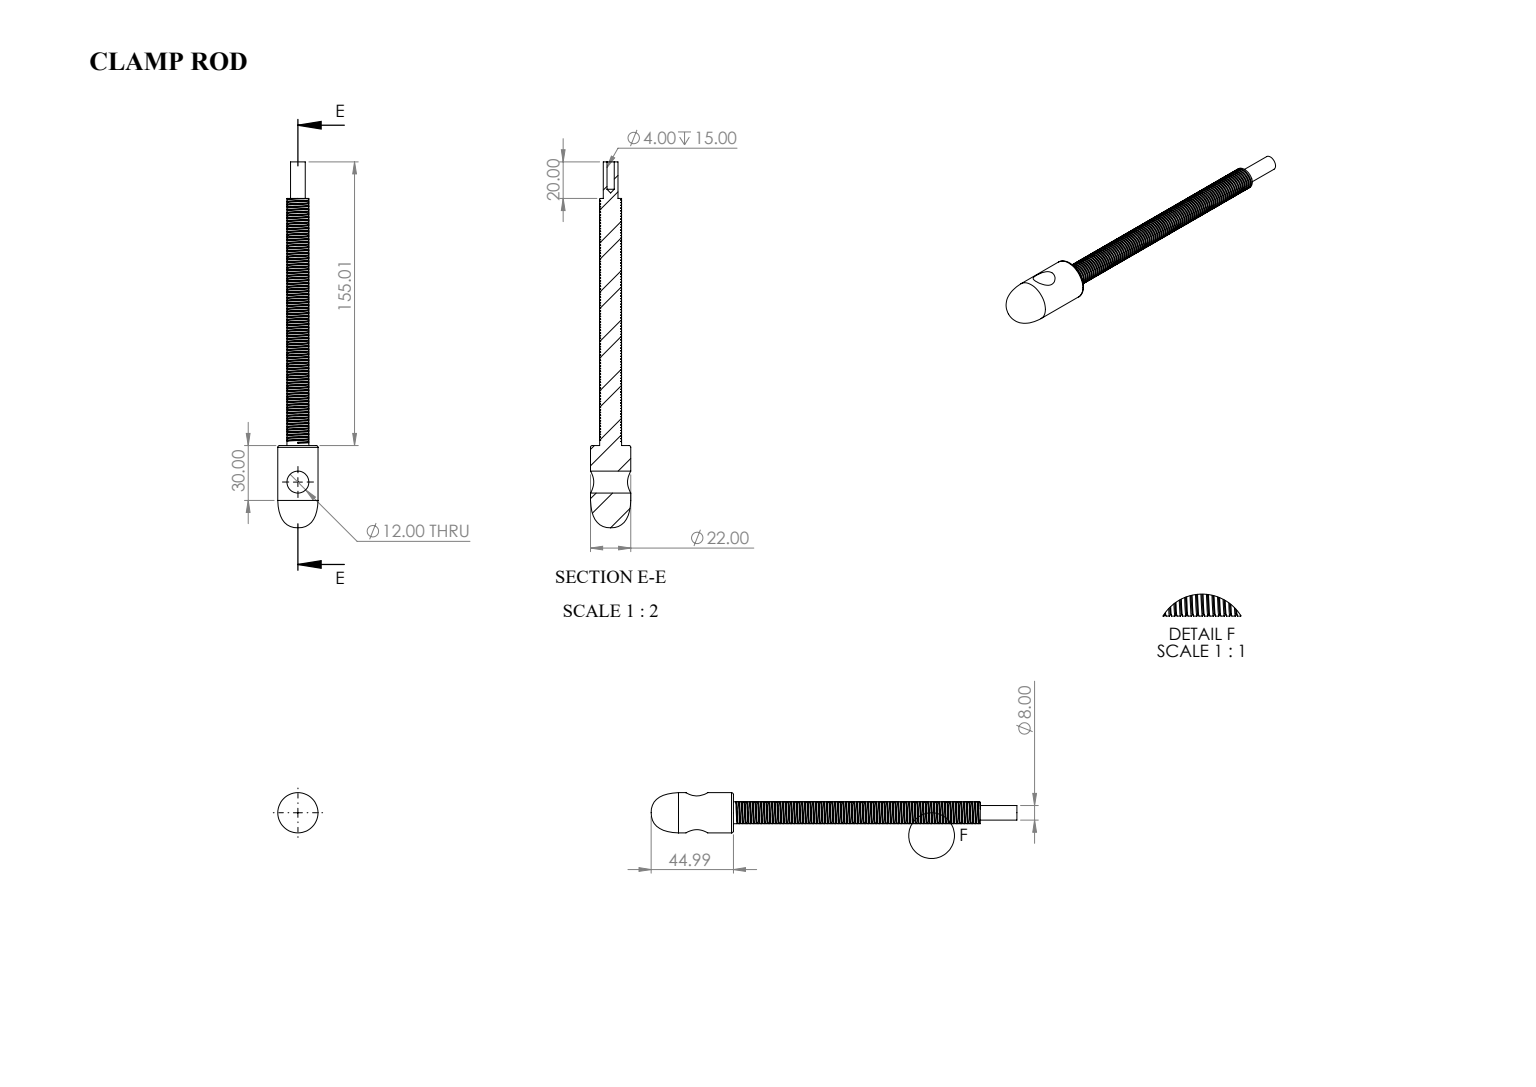
ISO-10303-21;
HEADER;
FILE_DESCRIPTION (('STEP AP214'),
    '1' );
FILE_NAME ('Clamp rod.step',
    '2026-10-07T06:38:26',
    ( '' ),
    ( '' ),
    'SwSTEP 2.0',
    'SolidWorks 2021',
    '' );
FILE_SCHEMA (( 'AUTOMOTIVE_DESIGN' ));
ENDSEC;

DATA;
#1=VERTEX_POINT ( 'NONE', #13580 ) ;
#5=ORIENTED_EDGE ( 'NONE', *, *, #19399, .F. ) ;
#6=CARTESIAN_POINT ( 'NONE',  ( -5.412658773652684552, -3.125000000000099920, -143.0669872981078470 ) ) ;
#10=CARTESIAN_POINT ( 'NONE',  ( 5.999999999999999112, 2.951592740943527306E-14, -151.5863248654052029 ) ) ;
#13=CARTESIAN_POINT ( 'NONE',  ( 3.464101615137757051, -5.999999999999979572, -171.3363248654052029 ) ) ;
#15=CARTESIAN_POINT ( 'NONE',  ( -5.412658773652739619, 3.124999999999975131, -63.18301270189225249 ) ) ;
#16=CARTESIAN_POINT ( 'NONE',  ( -5.999999999999963585, 1.780251999655701777E-13, -110.9136751345948255 ) ) ;
#18=DIRECTION ( 'NONE',  ( 1.000000000000000000, -5.551115123125774074E-17, 0.000000000000000000 ) ) ;
#21=CYLINDRICAL_SURFACE ( 'NONE', #16144, 11.00000000000001599 ) ;
#23=EDGE_CURVE ( 'NONE', #18475, #14303, #3726, .T. ) ;
#26=EDGE_LOOP ( 'NONE', ( #21447, #18277, #20127, #3460 ) ) ;
#27=CARTESIAN_POINT ( 'NONE',  ( -6.350852961085760029, -1.281975124255709124E-13, -55.12500000000003553 ) ) ;
#29=CARTESIAN_POINT ( 'NONE',  ( 6.000000000000000888, -1.859271017917181981E-14, -167.1636751345948255 ) ) ;
#30=CARTESIAN_POINT ( 'NONE',  ( -3.464101615137757051, -5.999999999999979572, -179.0863248654052313 ) ) ;
#34=CARTESIAN_POINT ( 'NONE',  ( -3.608439182435052128, -6.250000000000110134, -103.9419872981078328 ) ) ;
#36=CARTESIAN_POINT ( 'NONE',  ( -3.464101615137725076, 5.999999999999979572, -176.5863248654052313 ) ) ;
#37=VECTOR ( 'NONE', #4562, 1000.000000000000000 ) ;
#40=CARTESIAN_POINT ( 'NONE',  ( 3.175426480543072749, -5.500000000000105693, -138.6250000000000568 ) ) ;
#47=CARTESIAN_POINT ( 'NONE',  ( -3.175426480542816510, -5.500000000000057732, -66.87500000000002842 ) ) ;
#48=CARTESIAN_POINT ( 'NONE',  ( 0.000000000000000000, -5.999999999999991118, -81.46132486540524553 ) ) ;
#50=CARTESIAN_POINT ( 'NONE',  ( 3.608439182435180470, 6.249999999999982236, -80.05801270189219565 ) ) ;
#51=CARTESIAN_POINT ( 'NONE',  ( 5.196152422706629359, 3.000000000000002665, -140.0386751345948255 ) ) ;
#58=( BOUNDED_CURVE ( )  B_SPLINE_CURVE ( 2, ( #3111, #10057, #5114, #12242, #12386, #512, #17135, #26164, #2819 ),
 .UNSPECIFIED., .F., .T. ) 
 B_SPLINE_CURVE_WITH_KNOTS ( ( 3, 2, 2, 2, 3 ),
 ( 0.05277777777777781232, 0.05370370370370369795, 0.05555555555555558023, 0.05740740740740746251, 0.05833333333333334814 ),
 .UNSPECIFIED. ) 
 CURVE ( )  GEOMETRIC_REPRESENTATION_ITEM ( )  RATIONAL_B_SPLINE_CURVE ( ( 0.9330127018922194093, 0.9330127018922234061, 1.000000000000000000, 0.8660254037844388186, 1.000000000000000000, 0.8660254037844388186, 1.000000000000000000, 0.9330127018922194093, 0.9330127018922194093 ) ) 
 REPRESENTATION_ITEM ( '' )  );
#59=CARTESIAN_POINT ( 'NONE',  ( 4.763139720814407951, -2.749999999999988454, -149.0000000000000284 ) ) ;
#61=CARTESIAN_POINT ( 'NONE',  ( 3.175426480543072749, -5.500000000000105693, -138.6250000000000568 ) ) ;
#62=CARTESIAN_POINT ( 'NONE',  ( 3.608439182435180470, 6.249999999999982236, -164.0580127018922383 ) ) ;
#63=CARTESIAN_POINT ( 'NONE',  ( 0.000000000000000000, -5.999999999999991118, -148.9613248654052597 ) ) ;
#65=CARTESIAN_POINT ( 'NONE',  ( 6.350852961086080661, -9.614813431917819062E-14, -76.87500000000002842 ) ) ;
#67=CARTESIAN_POINT ( 'NONE',  ( -4.763139720814407951, 2.749999999999946709, -62.75000000000002842 ) ) ;
#68=CARTESIAN_POINT ( 'NONE',  ( -5.196152422706601826, 2.999999999999975131, -154.5386751345948539 ) ) ;
#70=CARTESIAN_POINT ( 'NONE',  ( 3.464101615137757051, -5.999999999999979572, -114.3363248654051745 ) ) ;
#71=CARTESIAN_POINT ( 'NONE',  ( -5.196152422706573404, -3.000000000000002665, -144.7113248654052313 ) ) ;
#74=CARTESIAN_POINT ( 'NONE',  ( -3.464101615137757051, -5.999999999999979572, -50.08632486540522422 ) ) ;
#75=CARTESIAN_POINT ( 'NONE',  ( 6.000000000000000888, -3.330669073875464691E-16, -7.560779664488942560E-35 ) ) ;
#78=ORIENTED_EDGE ( 'NONE', *, *, #7844, .T. ) ;
#82=CARTESIAN_POINT ( 'NONE',  ( -3.464101615137757051, -5.999999999999979572, -85.16367513459481131 ) ) ;
#84=VERTEX_POINT ( 'NONE', #7829 ) ;
#86=VECTOR ( 'NONE', #24008, 1000.000000000000114 ) ;
#87=VERTEX_POINT ( 'NONE', #29166 ) ;
#89=CARTESIAN_POINT ( 'NONE',  ( -6.350852961085760029, -1.281975124255709124E-13, -91.12500000000001421 ) ) ;
#90=CARTESIAN_POINT ( 'NONE',  ( -7.216878364870328078, 0.000000000000000000, -106.5580127018922525 ) ) ;
#91=VERTEX_POINT ( 'NONE', #21836 ) ;
#92=CARTESIAN_POINT ( 'NONE',  ( 5.959413262067462469, 9.246315551493085039, -24.19612909832622449 ) ) ;
#94=CIRCLE ( 'NONE', #6471, 2.000000000000003109 ) ;
#95=CARTESIAN_POINT ( 'NONE',  ( 3.464101615137757051, -5.999999999999979572, -63.33632486540521711 ) ) ;
#97=ADVANCED_FACE ( 'NONE', ( #784 ), #22288, .T. ) ;
#99=CARTESIAN_POINT ( 'NONE',  ( 4.763139720814407951, 2.750000000000002665, -169.7500000000000000 ) ) ;
#102=CARTESIAN_POINT ( 'NONE',  ( -4.763139720814407951, 2.749999999999946709, -151.2500000000000000 ) ) ;
#106=CARTESIAN_POINT ( 'NONE',  ( -2.775557561562891351E-14, -5.500000000000115463, -101.2500000000000000 ) ) ;
#109=CARTESIAN_POINT ( 'NONE',  ( 3.175426480543072749, 5.499999999999865885, -154.6250000000000853 ) ) ;
#110=CARTESIAN_POINT ( 'NONE',  ( -3.175426480542816510, 5.499999999999865885, -86.87500000000007105 ) ) ;
#113=ORIENTED_EDGE ( 'NONE', *, *, #22581, .F. ) ;
#120=ORIENTED_EDGE ( 'NONE', *, *, #127, .F. ) ;
#122=DIRECTION ( 'NONE',  ( -7.147005652999508048E-36, 5.642372883946980038E-36, 1.000000000000000000 ) ) ;
#124=VERTEX_POINT ( 'NONE', #14929 ) ;
#127=EDGE_CURVE ( 'NONE', #21812, #1827, #10033, .T. ) ;
#128=CARTESIAN_POINT ( 'NONE',  ( 4.763139720814407951, -2.749999999999988454, -109.9999999999999858 ) ) ;
#130=CARTESIAN_POINT ( 'NONE',  ( 3.175426480543072749, -5.500000000000105693, -150.6250000000000284 ) ) ;
#131=CARTESIAN_POINT ( 'NONE',  ( -5.412658773652684552, -3.125000000000099920, -130.4330127018922383 ) ) ;
#132=ORIENTED_EDGE ( 'NONE', *, *, #22296, .F. ) ;
#133=CARTESIAN_POINT ( 'NONE',  ( 0.000000000000000000, 0.000000000000000000, 0.000000000000000000 ) ) ;
#134=CARTESIAN_POINT ( 'NONE',  ( 3.608439182435180470, -6.249999999999997335, -171.1919872981078470 ) ) ;
#137=VERTEX_POINT ( 'NONE', #1215 ) ;
#141=CARTESIAN_POINT ( 'NONE',  ( -3.464101615137725076, 5.999999999999979572, -95.58632486540524553 ) ) ;
#143=CARTESIAN_POINT ( 'NONE',  ( -2.775557561562891351E-14, -5.500000000000115463, -180.7500000000000284 ) ) ;
#145=CARTESIAN_POINT ( 'NONE',  ( -5.412658773652739619, 3.124999999999975131, -178.6830127018922383 ) ) ;
#149=CARTESIAN_POINT ( 'NONE',  ( -6.350852961085760029, -1.281975124255709124E-13, -113.6249999999999858 ) ) ;
#152=VERTEX_POINT ( 'NONE', #29328 ) ;
#154=DIRECTION ( 'NONE',  ( -7.147005652999508048E-36, 5.642372883946980038E-36, 1.000000000000000000 ) ) ;
#155=CARTESIAN_POINT ( 'NONE',  ( 6.000000000000000888, 1.607695154586715303, -168.5966878364870354 ) ) ;
#156=CARTESIAN_POINT ( 'NONE',  ( 5.196152422706629359, 3.000000000000002665, -131.9613248654052313 ) ) ;
#157=( BOUNDED_CURVE ( )  B_SPLINE_CURVE ( 2, ( #10782, #15865, #1831, #11235, #29931, #22280, #26855, #27319, #5814 ),
 .UNSPECIFIED., .F., .T. ) 
 B_SPLINE_CURVE_WITH_KNOTS ( ( 3, 2, 2, 2, 3 ),
 ( 0.6750000000000000444, 0.6759259259259259300, 0.6777777777777778123, 0.6796296296296295836, 0.6805555555555554692 ),
 .UNSPECIFIED. ) 
 CURVE ( )  GEOMETRIC_REPRESENTATION_ITEM ( )  RATIONAL_B_SPLINE_CURVE ( ( 0.9330127018922194093, 0.9330127018922234061, 1.000000000000000000, 0.8660254037844388186, 1.000000000000000000, 0.8660254037844388186, 1.000000000000000000, 0.9330127018922234061, 0.9330127018922194093 ) ) 
 REPRESENTATION_ITEM ( '' )  );
#159=EDGE_LOOP ( 'NONE', ( #11290, #9356, #28132, #17982 ) ) ;
#170=CARTESIAN_POINT ( 'NONE',  ( 3.608439182435180470, -6.249999999999997335, -141.1919872981078186 ) ) ;
#177=CYLINDRICAL_SURFACE ( 'NONE', #16338, 6.000000000000000888 ) ;
#179=CARTESIAN_POINT ( 'NONE',  ( 3.464101615137852974, 5.999999999999884537, -146.8363248654052313 ) ) ;
#184=CARTESIAN_POINT ( 'NONE',  ( -4.763139720814407951, -2.750000000000016431, -58.00000000000004974 ) ) ;
#186=CYLINDRICAL_SURFACE ( 'NONE', #12466, 6.000000000000000888 ) ;
#190=CARTESIAN_POINT ( 'NONE',  ( -7.216878364870328078, 0.000000000000000000, -99.69198729810781856 ) ) ;
#194=CARTESIAN_POINT ( 'NONE',  ( -4.763139720814407951, 2.749999999999946709, -128.7500000000000284 ) ) ;
#197=EDGE_LOOP ( 'NONE', ( #23745, #2064, #9008, #12960 ) ) ;
#198=CARTESIAN_POINT ( 'NONE',  ( 6.000000000000052403, 1.607695154586625819, -163.5193375672974128 ) ) ;
#199=CARTESIAN_POINT ( 'NONE',  ( 0.000000000000000000, 5.499999999999991118, -67.50000000000000000 ) ) ;
#201=CARTESIAN_POINT ( 'NONE',  ( 2.775557561562891351E-14, 6.250000000000033751, -84.43301270189223828 ) ) ;
#202=CARTESIAN_POINT ( 'NONE',  ( 6.000000000000000888, -3.330669073875464691E-16, -7.560779664488942560E-35 ) ) ;
#203=CARTESIAN_POINT ( 'NONE',  ( 6.000000000000000888, 1.743066579297358182E-13, -113.1636751345948397 ) ) ;
#205=FACE_OUTER_BOUND ( 'NONE', #29290, .T. ) ;
#208=CARTESIAN_POINT ( 'NONE',  ( -3.175426480542816066, -5.500000000000057732, -144.8750000000000853 ) ) ;
#209=CARTESIAN_POINT ( 'NONE',  ( 5.196152422706629359, -2.999999999999988898, -105.2113248654052455 ) ) ;
#210=CARTESIAN_POINT ( 'NONE',  ( 3.608439182435180470, -6.249999999999997335, -155.5580127018922383 ) ) ;
#211=DIRECTION ( 'NONE',  ( 1.000000000000000000, -5.551115123125773458E-17, -1.260129944081490338E-35 ) ) ;
#212=DIRECTION ( 'NONE',  ( 1.000000000000000000, -5.551115123125774074E-17, 0.000000000000000000 ) ) ;
#213=CARTESIAN_POINT ( 'NONE',  ( -4.763139720814407951, 2.749999999999946709, -82.25000000000004263 ) ) ;
#214=CARTESIAN_POINT ( 'NONE',  ( 5.999999999999974243, 1.607695154586759934, -132.5966878364870354 ) ) ;
#215=CARTESIAN_POINT ( 'NONE',  ( -6.350852961085760029, -1.281975124255709124E-13, -67.12500000000002842 ) ) ;
#216=CARTESIAN_POINT ( 'NONE',  ( -5.999999999999971578, 1.607695154586715303, -154.4806624327026157 ) ) ;
#218=CARTESIAN_POINT ( 'NONE',  ( 0.000000000000000000, 0.000000000000000000, 0.000000000000000000 ) ) ;
#221=EDGE_CURVE ( 'NONE', #23969, #26551, #13207, .T. ) ;
#222=CARTESIAN_POINT ( 'NONE',  ( 6.000000000000000888, 1.743066579297358182E-13, -49.58632486540520290 ) ) ;
#225=DIRECTION ( 'NONE',  ( -7.147005652999508048E-36, 5.642372883946980038E-36, 1.000000000000000000 ) ) ;
#226=VERTEX_POINT ( 'NONE', #20904 ) ;
#229=CARTESIAN_POINT ( 'NONE',  ( -5.999999999999963585, 1.780251999655701777E-13, -62.91367513459483973 ) ) ;
#230=( BOUNDED_CURVE ( )  B_SPLINE_CURVE ( 2, ( #16660, #4488, #23098, #2488, #25984, #326, #16513, #12052, #16065 ),
 .UNSPECIFIED., .F., .T. ) 
 B_SPLINE_CURVE_WITH_KNOTS ( ( 3, 2, 2, 2, 3 ),
 ( 0.5083333333333334147, 0.5092592592592593004, 0.5111111111111110716, 0.5129629629629629539, 0.5138888888888888395 ),
 .UNSPECIFIED. ) 
 CURVE ( )  GEOMETRIC_REPRESENTATION_ITEM ( )  RATIONAL_B_SPLINE_CURVE ( ( 0.9330127018922194093, 0.9330127018922234061, 1.000000000000000000, 0.8660254037844388186, 1.000000000000000000, 0.8660254037844388186, 1.000000000000000000, 0.9330127018922234061, 0.9330127018922194093 ) ) 
 REPRESENTATION_ITEM ( '' )  );
#231=ADVANCED_FACE ( 'NONE', ( #13556 ), #6599, .F. ) ;
#233=CARTESIAN_POINT ( 'NONE',  ( 2.775557561562891351E-14, -6.250000000000061284, -151.8169872981078186 ) ) ;
#235=CARTESIAN_POINT ( 'NONE',  ( -2.775557561562891351E-14, -5.500000000000115463, -87.75000000000000000 ) ) ;
#236=CARTESIAN_POINT ( 'NONE',  ( -5.412658773652684552, -3.125000000000099920, -100.4330127018922525 ) ) ;
#237=( BOUNDED_CURVE ( )  B_SPLINE_CURVE ( 2, ( #7992, #5676, #24577, #27183, #10633, #12799, #20145, #15086, #3680 ),
 .UNSPECIFIED., .F., .F. ) 
 B_SPLINE_CURVE_WITH_KNOTS ( ( 3, 2, 2, 2, 3 ),
 ( 0.5416666666666667407, 0.5425925925925925153, 0.5444444444444445086, 0.5462962962962962798, 0.5472222222222222765 ),
 .UNSPECIFIED. ) 
 CURVE ( )  GEOMETRIC_REPRESENTATION_ITEM ( )  RATIONAL_B_SPLINE_CURVE ( ( 0.9330127018922194093, 0.9330127018922274029, 1.000000000000000000, 0.8660254037844388186, 1.000000000000000000, 0.8660254037844388186, 1.000000000000000000, 0.9330127018922154125, 0.9330127018922194093 ) ) 
 REPRESENTATION_ITEM ( '' )  );
#238=ORIENTED_EDGE ( 'NONE', *, *, #23310, .F. ) ;
#240=CARTESIAN_POINT ( 'NONE',  ( 3.175426480543072749, -5.500000000000105693, -167.1250000000000000 ) ) ;
#241=CARTESIAN_POINT ( 'NONE',  ( -5.999999999999962697, 3.323446944526963891E-14, -155.3363248654052313 ) ) ;
#243=CARTESIAN_POINT ( 'NONE',  ( -5.999999999999963585, 1.780251999655701777E-13, -68.33632486540521711 ) ) ;
#244=CARTESIAN_POINT ( 'NONE',  ( 6.350852961086080661, -9.614813431917819062E-14, -175.8750000000000284 ) ) ;
#247=CARTESIAN_POINT ( 'NONE',  ( -6.350852961085760029, -1.281975124255709124E-13, -158.6250000000000284 ) ) ;
#249=CARTESIAN_POINT ( 'NONE',  ( 0.000000000000000000, -5.999999999999991118, -103.9613248654052171 ) ) ;
#251=CARTESIAN_POINT ( 'NONE',  ( 6.350852961086080661, -9.614813431917819062E-14, -100.8749999999999858 ) ) ;
#254=CARTESIAN_POINT ( 'NONE',  ( 0.000000000000000000, 5.499999999999991118, -156.0000000000000284 ) ) ;
#255=CARTESIAN_POINT ( 'NONE',  ( 0.000000000000000000, 5.499999999999991118, -87.00000000000002842 ) ) ;
#264=LINE ( 'NONE', #7761, #2214 ) ;
#265=ORIENTED_EDGE ( 'NONE', *, *, #5075, .F. ) ;
#266=VECTOR ( 'NONE', #18330, 1000.000000000000000 ) ;
#267=FACE_OUTER_BOUND ( 'NONE', #28986, .T. ) ;
#268=DIRECTION ( 'NONE',  ( 1.000000000000000000, -5.551115123125773458E-17, -1.260129944081490338E-35 ) ) ;
#269=VERTEX_POINT ( 'NONE', #30248 ) ;
#270=EDGE_CURVE ( 'NONE', #5714, #18702, #21431, .T. ) ;
#271=EDGE_CURVE ( 'NONE', #137, #4894, #411, .T. ) ;
#272=ORIENTED_EDGE ( 'NONE', *, *, #28675, .F. ) ;
#275=CARTESIAN_POINT ( 'NONE',  ( 4.763139720814407951, -2.749999999999988454, -111.5000000000000426 ) ) ;
#277=CARTESIAN_POINT ( 'NONE',  ( -7.216878364870328078, 0.000000000000000000, -123.0580127018922667 ) ) ;
#280=CARTESIAN_POINT ( 'NONE',  ( 5.412658773652712085, -3.125000000000086153, -171.0669872981078186 ) ) ;
#282=CARTESIAN_POINT ( 'NONE',  ( -5.999999999999963585, 1.780251999655701777E-13, -95.91367513459483973 ) ) ;
#284=CARTESIAN_POINT ( 'NONE',  ( 1.170107792545981740, 5.489964307952348577, -180.0000000000000000 ) ) ;
#285=CARTESIAN_POINT ( 'NONE',  ( 6.000000000000052403, 1.607695154586625819, -138.0193375672974128 ) ) ;
#286=CARTESIAN_POINT ( 'NONE',  ( 3.175426480543072749, -5.500000000000105693, -176.1250000000000284 ) ) ;
#288=CARTESIAN_POINT ( 'NONE',  ( 5.412658773652712085, -3.125000000000086153, -173.4330127018922667 ) ) ;
#290=CARTESIAN_POINT ( 'NONE',  ( 6.000000000000000888, -1.859271017917181981E-14, -159.6636751345948539 ) ) ;
#291=CARTESIAN_POINT ( 'NONE',  ( 0.000000000000000000, 5.499999999999991118, -113.9999999999999858 ) ) ;
#293=CARTESIAN_POINT ( 'NONE',  ( 5.196152422706629359, 3.000000000000002665, -89.03867513459485394 ) ) ;
#297=FACE_OUTER_BOUND ( 'NONE', #159, .T. ) ;
#298=ADVANCED_FACE ( 'NONE', ( #18607 ), #22898, .T. ) ;
#300=FACE_OUTER_BOUND ( 'NONE', #4802, .T. ) ;
#301=ORIENTED_EDGE ( 'NONE', *, *, #25346, .T. ) ;
#303=CARTESIAN_POINT ( 'NONE',  ( -2.775557561562891351E-14, -5.500000000000115463, -177.7500000000000284 ) ) ;
#304=CARTESIAN_POINT ( 'NONE',  ( -5.999999999999919176, 1.607695154586804565, -109.4806624327025872 ) ) ;
#306=ADVANCED_FACE ( 'NONE', ( #6902 ), #3947, .F. ) ;
#309=ORIENTED_EDGE ( 'NONE', *, *, #13878, .F. ) ;
#310=CARTESIAN_POINT ( 'NONE',  ( 6.000000000000000888, 1.607695154586715303, -141.5966878364870354 ) ) ;
#312=AXIS2_PLACEMENT_3D ( 'NONE', #25231, #13938, #2374 ) ;
#313=CARTESIAN_POINT ( 'NONE',  ( 3.608439182435180470, -6.249999999999997335, -139.6919872981078470 ) ) ;
#316=CARTESIAN_POINT ( 'NONE',  ( 0.000000000000000000, -5.999999999999991118, -116.5386751345948113 ) ) ;
#320=CARTESIAN_POINT ( 'NONE',  ( -6.000000000000007105, -1.607695154586655129, -56.84668783648705670 ) ) ;
#321=CARTESIAN_POINT ( 'NONE',  ( -5.196152422706601826, 2.999999999999975131, -92.46132486540520290 ) ) ;
#322=CARTESIAN_POINT ( 'NONE',  ( -5.196152422706601826, 2.999999999999975131, -60.03867513459481842 ) ) ;
#323=CYLINDRICAL_SURFACE ( 'NONE', #17586, 6.000000000000000888 ) ;
#325=( BOUNDED_CURVE ( )  B_SPLINE_CURVE ( 2, ( #10202, #24450, #15442, #15117, #22321, #16023, #7867, #17427, #1256 ),
 .UNSPECIFIED., .F., .T. ) 
 B_SPLINE_CURVE_WITH_KNOTS ( ( 3, 2, 2, 2, 3 ),
 ( 0.9694444444444444420, 0.9703703703703703276, 0.9722222222222222099, 0.9740740740740740922, 0.9749999999999999778 ),
 .UNSPECIFIED. ) 
 CURVE ( )  GEOMETRIC_REPRESENTATION_ITEM ( )  RATIONAL_B_SPLINE_CURVE ( ( 0.9330127018922194093, 0.9330127018922194093, 1.000000000000000000, 0.8660254037844388186, 1.000000000000000000, 0.8660254037844388186, 1.000000000000000000, 0.9330127018922234061, 0.9330127018922194093 ) ) 
 REPRESENTATION_ITEM ( '' )  );
#326=CARTESIAN_POINT ( 'NONE',  ( -3.464101615137725076, 5.999999999999979572, -112.6636751345948113 ) ) ;
#330=CARTESIAN_POINT ( 'NONE',  ( 5.196152422706629359, 3.000000000000002665, -88.46132486540525974 ) ) ;
#331=DIRECTION ( 'NONE',  ( 1.000000000000000000, -5.551115123125773458E-17, -1.260129944081490338E-35 ) ) ;
#336=CARTESIAN_POINT ( 'NONE',  ( -5.412658773652684552, -3.125000000000099920, -107.0669872981078186 ) ) ;
#340=CARTESIAN_POINT ( 'NONE',  ( -2.775557561562891351E-14, -5.500000000000115463, -126.7500000000000284 ) ) ;
#341=VERTEX_POINT ( 'NONE', #2733 ) ;
#342=ORIENTED_EDGE ( 'NONE', *, *, #4463, .F. ) ;
#343=CARTESIAN_POINT ( 'NONE',  ( 0.000000000000000000, 5.999999999999977796, -163.2113248654052313 ) ) ;
#344=CARTESIAN_POINT ( 'NONE',  ( 6.350852961086080661, -9.614813431917819062E-14, -58.87500000000005684 ) ) ;
#345=CARTESIAN_POINT ( 'NONE',  ( 3.464101615137852974, 5.999999999999884537, -115.9136751345948255 ) ) ;
#347=CARTESIAN_POINT ( 'NONE',  ( -3.608439182435052128, -6.250000000000110134, -83.80801270189228092 ) ) ;
#353=CARTESIAN_POINT ( 'NONE',  ( 4.763139720814407951, 2.750000000000002665, -141.2500000000000000 ) ) ;
#356=CARTESIAN_POINT ( 'NONE',  ( -5.999999999999919176, 1.607695154586804565, -89.40331216351302146 ) ) ;
#357=CARTESIAN_POINT ( 'NONE',  ( -4.763139720814407951, -2.750000000000016431, -70.00000000000000000 ) ) ;
#361=CARTESIAN_POINT ( 'NONE',  ( 4.763139720814407951, -2.749999999999988454, -68.00000000000000000 ) ) ;
#375=CARTESIAN_POINT ( 'NONE',  ( 5.196152422706629359, -2.999999999999988898, -158.2886751345948824 ) ) ;
#376=CARTESIAN_POINT ( 'NONE',  ( 5.412658773652739619, 3.124999999999988898, -46.31698729810784698 ) ) ;
#378=CARTESIAN_POINT ( 'NONE',  ( -3.608439182435115633, 6.249999999999965361, -152.4419872981078186 ) ) ;
#380=CARTESIAN_POINT ( 'NONE',  ( 6.350852961086080661, -9.614813431917819062E-14, -93.37500000000001421 ) ) ;
#382=CARTESIAN_POINT ( 'NONE',  ( -5.999999999999963585, 8.134310703387671600E-14, -146.9136751345948255 ) ) ;
#384=EDGE_CURVE ( 'NONE', #3266, #22196, #14318, .T. ) ;
#385=CARTESIAN_POINT ( 'NONE',  ( 3.464101615137852974, 5.999999999999884537, -54.41367513459480421 ) ) ;
#388=CARTESIAN_POINT ( 'NONE',  ( 6.000000000000000888, -1.859271017917181981E-14, -58.58632486540521001 ) ) ;
#390=CARTESIAN_POINT ( 'NONE',  ( -6.350852961085760029, -1.281975124255709124E-13, -161.6250000000000284 ) ) ;
#391=CARTESIAN_POINT ( 'NONE',  ( 3.464101615137852974, 5.999999999999884537, -58.33632486540519579 ) ) ;
#393=CARTESIAN_POINT ( 'NONE',  ( 3.175426480543072749, 5.499999999999865885, -157.6250000000000000 ) ) ;
#395=CARTESIAN_POINT ( 'NONE',  ( -5.999999999999963585, 1.780251999655701777E-13, -52.41367513459481842 ) ) ;
#396=CARTESIAN_POINT ( 'NONE',  ( 4.763139720814407951, -2.749999999999988454, -104.0000000000000426 ) ) ;
#398=CARTESIAN_POINT ( 'NONE',  ( 4.763139720814407951, 2.750000000000002665, -85.75000000000000000 ) ) ;
#399=EDGE_CURVE ( 'NONE', #13073, #10035, #3539, .T. ) ;
#403=CARTESIAN_POINT ( 'NONE',  ( 6.000000000000000888, 1.743066579297358182E-13, -66.08632486540521711 ) ) ;
#405=DIRECTION ( 'NONE',  ( -7.147005652999508048E-36, 5.642372883946980038E-36, 1.000000000000000000 ) ) ;
#406=( BOUNDED_CURVE ( )  B_SPLINE_CURVE ( 2, ( #1039, #17971, #8566, #24843, #3636, #27284, #29442, #15202, #10435 ),
 .UNSPECIFIED., .F., .T. ) 
 B_SPLINE_CURVE_WITH_KNOTS ( ( 3, 2, 2, 2, 3 ),
 ( 0.7305555555555556246, 0.7314814814814813992, 0.7333333333333333925, 0.7351851851851851638, 0.7361111111111111605 ),
 .UNSPECIFIED. ) 
 CURVE ( )  GEOMETRIC_REPRESENTATION_ITEM ( )  RATIONAL_B_SPLINE_CURVE ( ( 0.9330127018922194093, 0.9330127018922274029, 1.000000000000000000, 0.8660254037844388186, 1.000000000000000000, 0.8660254037844388186, 1.000000000000000000, 0.9330127018922154125, 0.9330127018922194093 ) ) 
 REPRESENTATION_ITEM ( '' )  );
#407=VERTEX_POINT ( 'NONE', #16470 ) ;
#411=( BOUNDED_CURVE ( )  B_SPLINE_CURVE ( 2, ( #22599, #27778, #25320, #13714, #3980, #25172, #11559, #20749, #13403 ),
 .UNSPECIFIED., .F., .T. ) 
 B_SPLINE_CURVE_WITH_KNOTS ( ( 3, 2, 2, 2, 3 ),
 ( 0.7916666666666666297, 0.7925925925925926263, 0.7944444444444445086, 0.7962962962962962798, 0.7972222222222222765 ),
 .UNSPECIFIED. ) 
 CURVE ( )  GEOMETRIC_REPRESENTATION_ITEM ( )  RATIONAL_B_SPLINE_CURVE ( ( 0.9330127018922194093, 0.9330127018922154125, 1.000000000000000000, 0.8660254037844388186, 1.000000000000000000, 0.8660254037844388186, 1.000000000000000000, 0.9330127018922154125, 0.9330127018922194093 ) ) 
 REPRESENTATION_ITEM ( '' )  );
#415=CARTESIAN_POINT ( 'NONE',  ( -6.350852961085760029, -1.281975124255709124E-13, -116.6250000000000000 ) ) ;
#417=CARTESIAN_POINT ( 'NONE',  ( -7.216878364870328078, 0.000000000000000000, -126.0580127018922383 ) ) ;
#419=ORIENTED_EDGE ( 'NONE', *, *, #27844, .T. ) ;
#420=DIRECTION ( 'NONE',  ( -7.147005652999508048E-36, 5.642372883946980038E-36, 1.000000000000000000 ) ) ;
#421=CARTESIAN_POINT ( 'NONE',  ( -5.412658773652739619, 3.124999999999975131, -164.3169872981078470 ) ) ;
#424=EDGE_CURVE ( 'NONE', #5958, #13461, #21610, .T. ) ;
#425=ORIENTED_EDGE ( 'NONE', *, *, #2357, .T. ) ;
#429=CARTESIAN_POINT ( 'NONE',  ( -6.350852961085760029, -1.281975124255709124E-13, -178.1250000000000568 ) ) ;
#432=CARTESIAN_POINT ( 'NONE',  ( 5.412658773652712085, -3.125000000000086153, -180.9330127018922099 ) ) ;
#433=CARTESIAN_POINT ( 'NONE',  ( 3.464101615137852974, 5.999999999999884537, -76.33632486540521711 ) ) ;
#434=CARTESIAN_POINT ( 'NONE',  ( 6.000000000000000888, -1.859271017917181981E-14, -101.1636751345948397 ) ) ;
#435=CARTESIAN_POINT ( 'NONE',  ( 3.175426480543072749, 5.499999999999865885, -123.1250000000000426 ) ) ;
#437=CARTESIAN_POINT ( 'NONE',  ( 4.763139720814407951, -2.749999999999988454, -115.9999999999999858 ) ) ;
#442=CARTESIAN_POINT ( 'NONE',  ( -6.000000000000007105, -1.607695154586655129, -137.2693375672974412 ) ) ;
#445=CARTESIAN_POINT ( 'NONE',  ( -3.175426480542816066, -5.500000000000057732, -176.3750000000000284 ) ) ;
#447=CARTESIAN_POINT ( 'NONE',  ( 6.000000000000000888, -1.859271017917181981E-14, -110.1636751345948397 ) ) ;
#448=VERTEX_POINT ( 'NONE', #25798 ) ;
#449=CARTESIAN_POINT ( 'NONE',  ( 6.000000000000000888, 1.743066579297358182E-13, -77.16367513459482552 ) ) ;
#451=ORIENTED_EDGE ( 'NONE', *, *, #28247, .T. ) ;
#453=CARTESIAN_POINT ( 'NONE',  ( -5.999999999999919176, 1.607695154586804565, -84.90331216351302146 ) ) ;
#457=CARTESIAN_POINT ( 'NONE',  ( -7.216878364870328078, 0.000000000000000000, -131.1919872981078754 ) ) ;
#467=LINE ( 'NONE', #14635, #3548 ) ;
#469=PRESENTATION_STYLE_ASSIGNMENT (( #21238 ) ) ;
#471=DIRECTION ( 'NONE',  ( 1.000000000000000000, -5.551115123125773458E-17, -1.260129944081490338E-35 ) ) ;
#472=AXIS2_PLACEMENT_3D ( 'NONE', #8835, #8361, #29233 ) ;
#474=AXIS2_PLACEMENT_3D ( 'NONE', #15433, #6176, #10653 ) ;
#478=CARTESIAN_POINT ( 'NONE',  ( -5.196152422706601826, 2.999999999999975131, -62.46132486540523132 ) ) ;
#483=CARTESIAN_POINT ( 'NONE',  ( -5.412658773652739619, 3.124999999999975131, -107.3169872981078470 ) ) ;
#484=CARTESIAN_POINT ( 'NONE',  ( 0.000000000000000000, -5.999999999999991118, -50.53867513459481131 ) ) ;
#488=CARTESIAN_POINT ( 'NONE',  ( -4.763139720814407951, -2.750000000000016431, -128.5000000000000000 ) ) ;
#490=ORIENTED_EDGE ( 'NONE', *, *, #27090, .F. ) ;
#492=CARTESIAN_POINT ( 'NONE',  ( -4.763139720814407951, -2.750000000000016431, -58.00000000000004974 ) ) ;
#494=CARTESIAN_POINT ( 'NONE',  ( 3.464101615137757051, -5.999999999999979572, -179.4136751345948255 ) ) ;
#495=ADVANCED_FACE ( 'NONE', ( #14745 ), #24385, .T. ) ;
#496=CARTESIAN_POINT ( 'NONE',  ( -5.412658773652739619, 3.124999999999975131, -85.68301270189226670 ) ) ;
#497=( BOUNDED_CURVE ( )  B_SPLINE_CURVE ( 2, ( #1610, #24805, #8523, #10863, #3898, #11012, #30329, #18684, #16396 ),
 .UNSPECIFIED., .F., .T. ) 
 B_SPLINE_CURVE_WITH_KNOTS ( ( 3, 2, 2, 2, 3 ),
 ( 0.3027777777777777568, 0.3037037037037036979, 0.3055555555555555802, 0.3074074074074074070, 0.3083333333333333481 ),
 .UNSPECIFIED. ) 
 CURVE ( )  GEOMETRIC_REPRESENTATION_ITEM ( )  RATIONAL_B_SPLINE_CURVE ( ( 0.9330127018922194093, 0.9330127018922174109, 1.000000000000000000, 0.8660254037844388186, 1.000000000000000000, 0.8660254037844388186, 1.000000000000000000, 0.9330127018922174109, 0.9330127018922194093 ) ) 
 REPRESENTATION_ITEM ( '' )  );
#499=LINE ( 'NONE', #202, #6440 ) ;
#504=CARTESIAN_POINT ( 'NONE',  ( -3.175426480542816066, 5.499999999999865885, -137.8750000000000568 ) ) ;
#505=CARTESIAN_POINT ( 'NONE',  ( -5.999999999999963585, 1.780251999655701777E-13, -68.33632486540521711 ) ) ;
#506=CARTESIAN_POINT ( 'NONE',  ( 3.608439182435180470, 6.249999999999982236, -156.5580127018922383 ) ) ;
#509=CARTESIAN_POINT ( 'NONE',  ( 3.175426480543072749, -5.500000000000105693, -68.12500000000002842 ) ) ;
#510=CARTESIAN_POINT ( 'NONE',  ( 6.000000000000000888, 1.607695154586715303, -114.5966878364870496 ) ) ;
#511=CARTESIAN_POINT ( 'NONE',  ( 4.763139720814407951, -2.749999999999988454, -66.50000000000000000 ) ) ;
#512=CARTESIAN_POINT ( 'NONE',  ( 3.464101615137852974, 5.999999999999884537, -53.83632486540516737 ) ) ;
#514=CARTESIAN_POINT ( 'NONE',  ( 6.000000000000000888, -1.607695154586752384, -144.1533121635130215 ) ) ;
#516=CARTESIAN_POINT ( 'NONE',  ( 0.000000000000000000, 5.999999999999977796, -133.7886751345947971 ) ) ;
#518=DIRECTION ( 'NONE',  ( 1.000000000000000000, -5.551115123125773458E-17, -1.260129944081490338E-35 ) ) ;
#525=CARTESIAN_POINT ( 'NONE',  ( -4.763139720814407951, 2.749999999999946709, -176.7500000000000284 ) ) ;
#528=CARTESIAN_POINT ( 'NONE',  ( 5.412658773652712085, -3.125000000000086153, -151.5669872981077901 ) ) ;
#529=ORIENTED_EDGE ( 'NONE', *, *, #11929, .F. ) ;
#530=CARTESIAN_POINT ( 'NONE',  ( 0.000000000000000000, 5.499999999999991118, -79.50000000000001421 ) ) ;
#533=EDGE_CURVE ( 'NONE', #16758, #856, #5098, .T. ) ;
#534=CARTESIAN_POINT ( 'NONE',  ( 2.775557561562891351E-14, -6.250000000000061284, -98.68301270189222407 ) ) ;
#536=AXIS2_PLACEMENT_3D ( 'NONE', #24063, #9950, #268 ) ;
#537=CARTESIAN_POINT ( 'NONE',  ( 6.000000000000000888, 1.743066579297358182E-13, -99.08632486540518869 ) ) ;
#542=CARTESIAN_POINT ( 'NONE',  ( -6.350852961085760029, -1.281975124255709124E-13, -167.6249999999999716 ) ) ;
#544=CARTESIAN_POINT ( 'NONE',  ( -3.175426480542816510, -5.500000000000057732, -155.3750000000000000 ) ) ;
#545=CARTESIAN_POINT ( 'NONE',  ( -5.999999999999971578, 1.607695154586715303, -76.48066243270260145 ) ) ;
#546=CARTESIAN_POINT ( 'NONE',  ( -3.464101615137757051, -5.999999999999979572, -104.0863248654052171 ) ) ;
#548=CARTESIAN_POINT ( 'NONE',  ( -4.763139720814407951, 2.749999999999946709, -91.25000000000005684 ) ) ;
#549=CARTESIAN_POINT ( 'NONE',  ( -5.999999999999963585, 8.134310703387671600E-14, -125.3363248654052171 ) ) ;
#551=CARTESIAN_POINT ( 'NONE',  ( -4.763139720814407951, -2.750000000000016431, -89.50000000000002842 ) ) ;
#553=DIRECTION ( 'NONE',  ( -7.147005652999508048E-36, 5.642372883946980038E-36, 1.000000000000000000 ) ) ;
#559=FACE_OUTER_BOUND ( 'NONE', #25739, .T. ) ;
#561=CARTESIAN_POINT ( 'NONE',  ( 2.775557561562895769E-14, 11.00000000000000000, -14.99152654425661702 ) ) ;
#562=LINE ( 'NONE', #14722, #2515 ) ;
#563=VECTOR ( 'NONE', #154, 1000.000000000000000 ) ;
#565=EDGE_CURVE ( 'NONE', #10035, #23969, #28298, .T. ) ;
#567=VERTEX_POINT ( 'NONE', #2802 ) ;
#568=CARTESIAN_POINT ( 'NONE',  ( 6.350852961086080661, -9.614813431917819062E-14, -108.3750000000000426 ) ) ;
#570=EDGE_CURVE ( 'NONE', #16363, #15998, #499, .T. ) ;
#571=CARTESIAN_POINT ( 'NONE',  ( -5.412658773652739619, 3.124999999999975131, -124.6830127018922525 ) ) ;
#572=ORIENTED_EDGE ( 'NONE', *, *, #9855, .F. ) ;
#574=CARTESIAN_POINT ( 'NONE',  ( -3.608439182435115633, 6.249999999999965361, -164.4419872981078186 ) ) ;
#578=VECTOR ( 'NONE', #10743, 1000.000000000000000 ) ;
#579=CARTESIAN_POINT ( 'NONE',  ( -5.412658773652739619, 3.124999999999975131, -57.18301270189224539 ) ) ;
#580=ORIENTED_EDGE ( 'NONE', *, *, #270, .T. ) ;
#583=CARTESIAN_POINT ( 'NONE',  ( -4.763139720814407951, -2.750000000000016431, -175.0000000000000568 ) ) ;
#585=CARTESIAN_POINT ( 'NONE',  ( 0.000000000000000000, -5.999999999999991118, -112.9613248654052171 ) ) ;
#586=CARTESIAN_POINT ( 'NONE',  ( 2.775557561562891351E-14, 6.250000000000033751, -177.4330127018922667 ) ) ;
#589=CARTESIAN_POINT ( 'NONE',  ( 3.175426480543072749, 5.499999999999865885, -118.6250000000000284 ) ) ;
#590=CARTESIAN_POINT ( 'NONE',  ( -5.999999999999963585, 1.780251999655701777E-13, -48.83632486540521711 ) ) ;
#592=CARTESIAN_POINT ( 'NONE',  ( -4.763139720814407951, -2.750000000000016431, -113.5000000000000426 ) ) ;
#594=CARTESIAN_POINT ( 'NONE',  ( 0.000000000000000000, 5.999999999999977796, -88.78867513459486815 ) ) ;
#596=AXIS2_PLACEMENT_3D ( 'NONE', #27372, #17745, #27220 ) ;
#597=CARTESIAN_POINT ( 'NONE',  ( 6.000000000000000888, -1.859271017917181981E-14, -171.6636751345948539 ) ) ;
#602=CARTESIAN_POINT ( 'NONE',  ( 0.000000000000000000, 5.499999999999991118, -177.0000000000000568 ) ) ;
#603=EDGE_CURVE ( 'NONE', #26278, #3013, #9857, .T. ) ;
#606=CARTESIAN_POINT ( 'NONE',  ( -5.196152422706573404, -3.000000000000002665, -125.7886751345948539 ) ) ;
#607=ORIENTED_EDGE ( 'NONE', *, *, #14978, .T. ) ;
#614=CARTESIAN_POINT ( 'NONE',  ( 2.775557561562891351E-14, 6.250000000000033751, -134.5669872981078470 ) ) ;
#616=CARTESIAN_POINT ( 'NONE',  ( 3.464101615137852974, 5.999999999999884537, -130.9136751345948539 ) ) ;
#621=CARTESIAN_POINT ( 'NONE',  ( 6.000000000000000888, -1.859271017917181981E-14, -135.6636751345948255 ) ) ;
#629=LINE ( 'NONE', #14357, #14784 ) ;
#630=CARTESIAN_POINT ( 'NONE',  ( 4.763139720814407951, 2.750000000000002665, -139.7500000000000284 ) ) ;
#633=EDGE_LOOP ( 'NONE', ( #16313, #27975, #1968, #14002 ) ) ;
#634=CARTESIAN_POINT ( 'NONE',  ( 3.175426480543072749, -5.500000000000105693, -48.62500000000000711 ) ) ;
#635=CARTESIAN_POINT ( 'NONE',  ( -3.464101615137725076, 5.999999999999979572, -88.08632486540520290 ) ) ;
#636=CARTESIAN_POINT ( 'NONE',  ( -3.464101615137757051, -5.999999999999979572, -100.1636751345948113 ) ) ;
#637=STYLED_ITEM ( 'NONE', ( #9932 ), #15129 ) ;
#643=CARTESIAN_POINT ( 'NONE',  ( 7.216878364870455975, -6.409875621278545621E-14, -95.94198729810780435 ) ) ;
#646=CARTESIAN_POINT ( 'NONE',  ( 0.000000000000000000, 0.000000000000000000, 0.000000000000000000 ) ) ;
#648=CARTESIAN_POINT ( 'NONE',  ( -6.350852961085760029, -1.281975124255709124E-13, -130.1250000000000284 ) ) ;
#649=VECTOR ( 'NONE', #7995, 1000.000000000000000 ) ;
#650=ADVANCED_FACE ( 'NONE', ( #5702 ), #17888, .T. ) ;
#651=VERTEX_POINT ( 'NONE', #19847 ) ;
#655=CARTESIAN_POINT ( 'NONE',  ( 4.763139720814407951, -2.749999999999988454, -56.00000000000004974 ) ) ;
#656=DIRECTION ( 'NONE',  ( -7.147005652999508048E-36, 5.642372883946980038E-36, 1.000000000000000000 ) ) ;
#658=CARTESIAN_POINT ( 'NONE',  ( -7.216878364870328078, 0.000000000000000000, -82.55801270189220986 ) ) ;
#659=CARTESIAN_POINT ( 'NONE',  ( -6.000000000000000888, 1.067854986875958443E-15, 7.560779664488942560E-35 ) ) ;
#661=CARTESIAN_POINT ( 'NONE',  ( -5.196152422706601826, 2.999999999999975131, -79.53867513459483973 ) ) ;
#664=CARTESIAN_POINT ( 'NONE',  ( -4.763139720814407951, 2.749999999999946709, -136.2499999999999716 ) ) ;
#666=DIRECTION ( 'NONE',  ( -7.147005652999508048E-36, 5.642372883946980038E-36, 1.000000000000000000 ) ) ;
#667=CARTESIAN_POINT ( 'NONE',  ( 6.000000000000000888, 1.743066579297358182E-13, -51.66367513459483263 ) ) ;
#668=CARTESIAN_POINT ( 'NONE',  ( -2.775557561562891351E-14, -5.500000000000115463, -71.25000000000002842 ) ) ;
#669=CARTESIAN_POINT ( 'NONE',  ( 0.000000000000000000, 5.999999999999977796, -114.2886751345948397 ) ) ;
#670=CARTESIAN_POINT ( 'NONE',  ( 3.175426480543072749, 5.499999999999865885, -58.62499999999998579 ) ) ;
#671=LINE ( 'NONE', #12834, #5698 ) ;
#674=DIRECTION ( 'NONE',  ( 1.260129944081490070E-35, 5.642372883946978702E-36, 1.000000000000000000 ) ) ;
#677=CARTESIAN_POINT ( 'NONE',  ( -5.196152422706573404, -3.000000000000002665, -58.28867513459484684 ) ) ;
#681=DIRECTION ( 'NONE',  ( -7.147005652999508048E-36, 5.642372883946980038E-36, 1.000000000000000000 ) ) ;
#685=( BOUNDED_CURVE ( )  B_SPLINE_CURVE ( 2, ( #21379, #16796, #14490, #23827, #19664, #24717, #8270, #12486, #26695 ),
 .UNSPECIFIED., .F., .T. ) 
 B_SPLINE_CURVE_WITH_KNOTS ( ( 3, 2, 2, 2, 3 ),
 ( 0.9527777777777778345, 0.9537037037037037202, 0.9555555555555556024, 0.9574074074074073737, 0.9583333333333333703 ),
 .UNSPECIFIED. ) 
 CURVE ( )  GEOMETRIC_REPRESENTATION_ITEM ( )  RATIONAL_B_SPLINE_CURVE ( ( 0.9330127018922194093, 0.9330127018922234061, 1.000000000000000000, 0.8660254037844388186, 1.000000000000000000, 0.8660254037844388186, 1.000000000000000000, 0.9330127018922154125, 0.9330127018922194093 ) ) 
 REPRESENTATION_ITEM ( '' )  );
#686=CARTESIAN_POINT ( 'NONE',  ( 3.175426480543072749, -5.500000000000105693, -180.6250000000000284 ) ) ;
#688=VERTEX_POINT ( 'NONE', #17572 ) ;
#689=CARTESIAN_POINT ( 'NONE',  ( -6.350852961085760029, -1.281975124255709124E-13, -79.12500000000001421 ) ) ;
#690=CARTESIAN_POINT ( 'NONE',  ( 5.412658773652739619, 3.124999999999988898, -101.1830127018922241 ) ) ;
#693=CARTESIAN_POINT ( 'NONE',  ( -4.763139720814407951, 2.749999999999946709, -167.7500000000000000 ) ) ;
#697=CARTESIAN_POINT ( 'NONE',  ( -5.999999999999956479, -1.607695154586745057, -59.26933756729745539 ) ) ;
#700=CARTESIAN_POINT ( 'NONE',  ( 4.763139720814407951, -2.749999999999988454, -167.0000000000000284 ) ) ;
#701=CARTESIAN_POINT ( 'NONE',  ( 0.000000000000000000, -5.999999999999991118, -60.46132486540523132 ) ) ;
#702=CARTESIAN_POINT ( 'NONE',  ( -2.775557561562891351E-14, -5.500000000000115463, -150.7500000000000568 ) ) ;
#704=CARTESIAN_POINT ( 'NONE',  ( -5.196152422706573404, -3.000000000000002665, -52.28867513459483973 ) ) ;
#705=CARTESIAN_POINT ( 'NONE',  ( 3.175426480543072749, -5.500000000000105693, -98.12500000000004263 ) ) ;
#706=CARTESIAN_POINT ( 'NONE',  ( -3.175426480542816510, 5.499999999999865885, -89.87500000000001421 ) ) ;
#709=CARTESIAN_POINT ( 'NONE',  ( 0.000000000000000000, -5.999999999999991118, -136.0386751345948255 ) ) ;
#712=CARTESIAN_POINT ( 'NONE',  ( 6.000000000000000888, -1.859271017917181981E-14, -88.58632486540523132 ) ) ;
#713=EDGE_CURVE ( 'NONE', #28274, #9960, #8962, .T. ) ;
#716=EDGE_CURVE ( 'NONE', #15617, #21702, #27616, .T. ) ;
#718=CARTESIAN_POINT ( 'NONE',  ( 6.000000000000000888, -3.330669073875464691E-16, -7.560779664488942560E-35 ) ) ;
#719=CYLINDRICAL_SURFACE ( 'NONE', #14325, 4.000000000000004441 ) ;
#721=EDGE_LOOP ( 'NONE', ( #24132, #26615, #12517, #1556 ) ) ;
#723=ORIENTED_EDGE ( 'NONE', *, *, #24077, .F. ) ;
#724=CARTESIAN_POINT ( 'NONE',  ( -4.763139720814407951, 2.749999999999946709, -106.2500000000000142 ) ) ;
#726=CARTESIAN_POINT ( 'NONE',  ( 2.775557561562891351E-14, -6.250000000000061284, -122.6830127018922525 ) ) ;
#727=ORIENTED_EDGE ( 'NONE', *, *, #26320, .T. ) ;
#728=CARTESIAN_POINT ( 'NONE',  ( 6.000000000000000888, 1.743066579297358182E-13, -111.6636751345948255 ) ) ;
#729=CARTESIAN_POINT ( 'NONE',  ( 3.608439182435180470, 6.249999999999982236, -157.1919872981078470 ) ) ;
#733=VECTOR ( 'NONE', #24203, 1000.000000000000000 ) ;
#734=( BOUNDED_CURVE ( )  B_SPLINE_CURVE ( 2, ( #7930, #21493, #12589, #26656, #9808, #28516, #7487, #16897, #14586 ),
 .UNSPECIFIED., .F., .F. ) 
 B_SPLINE_CURVE_WITH_KNOTS ( ( 3, 2, 2, 2, 3 ),
 ( 0.8361111111111110272, 0.8370370370370370239, 0.8388888888888889062, 0.8407407407407407884, 0.8416666666666666741 ),
 .UNSPECIFIED. ) 
 CURVE ( )  GEOMETRIC_REPRESENTATION_ITEM ( )  RATIONAL_B_SPLINE_CURVE ( ( 0.9330127018922194093, 0.9330127018922154125, 1.000000000000000000, 0.8660254037844388186, 1.000000000000000000, 0.8660254037844388186, 1.000000000000000000, 0.9330127018922194093, 0.9330127018922194093 ) ) 
 REPRESENTATION_ITEM ( '' )  );
#735=CARTESIAN_POINT ( 'NONE',  ( 2.775557561562891351E-14, -6.250000000000061284, -61.18301270189224539 ) ) ;
#740=FACE_OUTER_BOUND ( 'NONE', #21778, .T. ) ;
#742=CARTESIAN_POINT ( 'NONE',  ( -5.999999999999963585, -1.487416814333745711E-14, -113.3363248654052029 ) ) ;
#743=CARTESIAN_POINT ( 'NONE',  ( -7.216878364870328078, 0.000000000000000000, -166.5580127018922383 ) ) ;
#744=CARTESIAN_POINT ( 'NONE',  ( 0.000000000000000000, 0.000000000000000000, 0.000000000000000000 ) ) ;
#747=CARTESIAN_POINT ( 'NONE',  ( 4.763139720814407951, 2.750000000000002665, -115.7500000000000142 ) ) ;
#748=CARTESIAN_POINT ( 'NONE',  ( -4.763139720814407951, -2.750000000000016431, -114.9999999999999858 ) ) ;
#749=CARTESIAN_POINT ( 'NONE',  ( -5.999999999999963585, -1.487416814333745711E-14, -88.41367513459482552 ) ) ;
#750=VERTEX_POINT ( 'NONE', #6178 ) ;
#753=CARTESIAN_POINT ( 'NONE',  ( 3.464101615137852974, 5.999999999999884537, -109.3363248654052313 ) ) ;
#754=ADVANCED_FACE ( 'NONE', ( #3547 ), #12979, .T. ) ;
#761=CARTESIAN_POINT ( 'NONE',  ( 5.196152422706629359, 3.000000000000002665, -144.5386751345948539 ) ) ;
#766=AXIS2_PLACEMENT_3D ( 'NONE', #22355, #13325, #29562 ) ;
#768=CARTESIAN_POINT ( 'NONE',  ( -3.608439182435115633, 6.249999999999965361, -131.4419872981078470 ) ) ;
#770=CARTESIAN_POINT ( 'NONE',  ( 6.000000000000000888, -1.859271017917181981E-14, -84.08632486540520290 ) ) ;
#771=CARTESIAN_POINT ( 'NONE',  ( -5.999999999999963585, 8.134310703387671600E-14, -116.9136751345948539 ) ) ;
#774=DIRECTION ( 'NONE',  ( -7.147005652999508048E-36, 5.642372883946980038E-36, 1.000000000000000000 ) ) ;
#776=( BOUNDED_CURVE ( )  B_SPLINE_CURVE ( 2, ( #18217, #4046, #8982, #16240, #3741, #13175, #17921, #22513, #27535 ),
 .UNSPECIFIED., .F., .T. ) 
 B_SPLINE_CURVE_WITH_KNOTS ( ( 3, 2, 2, 2, 3 ),
 ( 0.7249999999999999778, 0.7259259259259259744, 0.7277777777777777457, 0.7296296296296296280, 0.7305555555555556246 ),
 .UNSPECIFIED. ) 
 CURVE ( )  GEOMETRIC_REPRESENTATION_ITEM ( )  RATIONAL_B_SPLINE_CURVE ( ( 0.9330127018922194093, 0.9330127018922154125, 1.000000000000000000, 0.8660254037844388186, 1.000000000000000000, 0.8660254037844388186, 1.000000000000000000, 0.9330127018922154125, 0.9330127018922194093 ) ) 
 REPRESENTATION_ITEM ( '' )  );
#781=CARTESIAN_POINT ( 'NONE',  ( 6.000000000000052403, -1.607695154586662678, -162.1533121635129646 ) ) ;
#784=FACE_OUTER_BOUND ( 'NONE', #24987, .T. ) ;
#785=CARTESIAN_POINT ( 'NONE',  ( 6.350852961086080661, -9.614813431917819062E-14, -138.3750000000000568 ) ) ;
#787=ORIENTED_EDGE ( 'NONE', *, *, #30306, .T. ) ;
#788=CARTESIAN_POINT ( 'NONE',  ( -6.000000000000000888, 1.067854986875958443E-15, 7.560779664488942560E-35 ) ) ;
#793=DIRECTION ( 'NONE',  ( -7.147005652999508048E-36, 5.642372883946980038E-36, 1.000000000000000000 ) ) ;
#794=CARTESIAN_POINT ( 'NONE',  ( 2.775557561562891351E-14, -6.250000000000061284, -91.81698729810783277 ) ) ;
#798=CARTESIAN_POINT ( 'NONE',  ( -4.763139720814407951, -2.750000000000016431, -130.0000000000000000 ) ) ;
#799=VERTEX_POINT ( 'NONE', #16 ) ;
#803=CARTESIAN_POINT ( 'NONE',  ( -3.175426480542816510, 5.499999999999865885, -53.87500000000003553 ) ) ;
#804=CARTESIAN_POINT ( 'NONE',  ( -6.000000000000007105, -1.607695154586655129, -51.76933756729743408 ) ) ;
#805=CARTESIAN_POINT ( 'NONE',  ( 3.682280293032525798, 10.37087330740121516, -29.75307074678472219 ) ) ;
#806=CARTESIAN_POINT ( 'NONE',  ( -3.608439182435052128, -6.250000000000110134, -73.30801270189222407 ) ) ;
#808=CARTESIAN_POINT ( 'NONE',  ( 0.000000000000000000, 0.000000000000000000, -183.0000000000000000 ) ) ;
#810=CARTESIAN_POINT ( 'NONE',  ( 3.175426480543072749, -5.500000000000105693, -141.6250000000000000 ) ) ;
#812=CARTESIAN_POINT ( 'NONE',  ( -7.216878364870328078, 0.000000000000000000, -156.0580127018922383 ) ) ;
#813=CARTESIAN_POINT ( 'NONE',  ( 0.000000000000000000, 5.499999999999991118, -70.50000000000000000 ) ) ;
#814=ADVANCED_FACE ( 'NONE', ( #25673 ), #14053, .T. ) ;
#815=CARTESIAN_POINT ( 'NONE',  ( -6.350852961085760029, -1.281975124255709124E-13, -61.12500000000000711 ) ) ;
#819=CARTESIAN_POINT ( 'NONE',  ( 6.000000000000000888, 7.762456499804234384E-14, -127.5863248654052171 ) ) ;
#820=VECTOR ( 'NONE', #10037, 1000.000000000000000 ) ;
#823=ORIENTED_EDGE ( 'NONE', *, *, #13344, .F. ) ;
#828=CARTESIAN_POINT ( 'NONE',  ( 3.175426480543072749, -5.500000000000105693, -177.6250000000000284 ) ) ;
#830=CARTESIAN_POINT ( 'NONE',  ( 2.775557561562891351E-14, 6.250000000000033751, -155.5669872981078186 ) ) ;
#832=CARTESIAN_POINT ( 'NONE',  ( 3.175426480543072749, 5.499999999999865885, -79.62500000000002842 ) ) ;
#837=CARTESIAN_POINT ( 'NONE',  ( 2.676951800742168933E-14, -11.00000000000000000, -19.00000000000002132 ) ) ;
#839=CARTESIAN_POINT ( 'NONE',  ( -2.775557561562891351E-14, -5.500000000000115463, -162.7500000000000000 ) ) ;
#840=CARTESIAN_POINT ( 'NONE',  ( -5.999999999999963585, 1.780251999655701777E-13, -70.41367513459482552 ) ) ;
#841=CARTESIAN_POINT ( 'NONE',  ( 3.175426480543072749, -5.500000000000105693, -144.6250000000000000 ) ) ;
#843=CARTESIAN_POINT ( 'NONE',  ( 3.175426480543072749, 5.499999999999865885, -91.62500000000001421 ) ) ;
#844=LINE ( 'NONE', #12869, #23611 ) ;
#846=( BOUNDED_CURVE ( )  B_SPLINE_CURVE ( 2, ( #18304, #29786, #27617, #4440, #13865, #23205, #26380, #5028, #14738 ),
 .UNSPECIFIED., .F., .F. ) 
 B_SPLINE_CURVE_WITH_KNOTS ( ( 3, 2, 2, 2, 3 ),
 ( 0.7694444444444443754, 0.7703703703703703720, 0.7722222222222222543, 0.7740740740740741366, 0.7750000000000000222 ),
 .UNSPECIFIED. ) 
 CURVE ( )  GEOMETRIC_REPRESENTATION_ITEM ( )  RATIONAL_B_SPLINE_CURVE ( ( 0.9330127018922194093, 0.9330127018922154125, 1.000000000000000000, 0.8660254037844388186, 1.000000000000000000, 0.8660254037844388186, 1.000000000000000000, 0.9330127018922194093, 0.9330127018922194093 ) ) 
 REPRESENTATION_ITEM ( '' )  );
#847=CARTESIAN_POINT ( 'NONE',  ( -6.350852961085760029, -1.281975124255709124E-13, -82.12500000000004263 ) ) ;
#848=CARTESIAN_POINT ( 'NONE',  ( -3.464101615137725076, 5.999999999999979572, -143.5863248654052029 ) ) ;
#853=ORIENTED_EDGE ( 'NONE', *, *, #6435, .T. ) ;
#854=DIRECTION ( 'NONE',  ( -7.147005652999508048E-36, 5.642372883946980038E-36, 1.000000000000000000 ) ) ;
#855=CARTESIAN_POINT ( 'NONE',  ( 0.000000000000000000, 0.000000000000000000, 0.000000000000000000 ) ) ;
#856=VERTEX_POINT ( 'NONE', #23833 ) ;
#859=ORIENTED_EDGE ( 'NONE', *, *, #13108, .T. ) ;
#860=CARTESIAN_POINT ( 'NONE',  ( -6.350852961085760029, -1.281975124255709124E-13, -109.1250000000000426 ) ) ;
#862=CARTESIAN_POINT ( 'NONE',  ( 7.216878364870455975, -6.409875621278545621E-14, -123.8080127018922099 ) ) ;
#863=CARTESIAN_POINT ( 'NONE',  ( -3.464101615137725076, 5.999999999999979572, -111.1636751345948113 ) ) ;
#864=CARTESIAN_POINT ( 'NONE',  ( -5.412658773652684552, -3.125000000000099920, -158.0669872981078754 ) ) ;
#866=VECTOR ( 'NONE', #30376, 1000.000000000000000 ) ;
#869=ADVANCED_FACE ( 'NONE', ( #2769 ), #23688, .T. ) ;
#870=CARTESIAN_POINT ( 'NONE',  ( 3.608439182435180470, 6.249999999999982236, -56.05801270189221697 ) ) ;
#873=EDGE_CURVE ( 'NONE', #26117, #9617, #18488, .T. ) ;
#875=CARTESIAN_POINT ( 'NONE',  ( 0.000000000000000000, 5.999999999999977796, -137.7113248654052029 ) ) ;
#876=CARTESIAN_POINT ( 'NONE',  ( 3.175426480543072749, -5.500000000000105693, -173.1250000000000284 ) ) ;
#879=CARTESIAN_POINT ( 'NONE',  ( 7.216878364870455975, -6.409875621278545621E-14, -167.3080127018922951 ) ) ;
#882=CARTESIAN_POINT ( 'NONE',  ( -3.175426480542816066, 5.499999999999865885, -119.8750000000000284 ) ) ;
#884=CARTESIAN_POINT ( 'NONE',  ( -2.775557561562891351E-14, -5.500000000000115463, -105.7500000000000142 ) ) ;
#885=CARTESIAN_POINT ( 'NONE',  ( -5.196152422706601826, 2.999999999999975131, -100.5386751345947971 ) ) ;
#889=CARTESIAN_POINT ( 'NONE',  ( -5.999999999999963585, 1.780251999655701777E-13, -104.3363248654052313 ) ) ;
#890=CARTESIAN_POINT ( 'NONE',  ( 0.000000000000000000, 5.999999999999977796, -86.71132486540523132 ) ) ;
#891=VERTEX_POINT ( 'NONE', #3355 ) ;
#892=CARTESIAN_POINT ( 'NONE',  ( 5.196152422706629359, -2.999999999999988898, -126.7886751345948539 ) ) ;
#893=CARTESIAN_POINT ( 'NONE',  ( -7.216878364870328078, 0.000000000000000000, -84.69198729810781856 ) ) ;
#899=VERTEX_POINT ( 'NONE', #10460 ) ;
#900=CARTESIAN_POINT ( 'NONE',  ( 5.412658773652712085, -3.125000000000086153, -127.5669872981078328 ) ) ;
#904=EDGE_LOOP ( 'NONE', ( #7851, #19174, #4581, #7003 ) ) ;
#907=EDGE_CURVE ( 'NONE', #26173, #21329, #8122, .T. ) ;
#908=CYLINDRICAL_SURFACE ( 'NONE', #11806, 6.000000000000000888 ) ;
#911=CARTESIAN_POINT ( 'NONE',  ( -3.464101615137757051, -5.999999999999979572, -47.08632486540521001 ) ) ;
#912=CARTESIAN_POINT ( 'NONE',  ( 2.775557561562891351E-14, 6.250000000000033751, -68.56698729810784698 ) ) ;
#916=CARTESIAN_POINT ( 'NONE',  ( -3.175426480542816510, -5.500000000000057732, -135.8750000000000284 ) ) ;
#921=CARTESIAN_POINT ( 'NONE',  ( -4.763139720814407951, 2.749999999999946709, -47.75000000000001421 ) ) ;
#923=CARTESIAN_POINT ( 'NONE',  ( -6.000000000000000888, 1.067854986875958443E-15, 7.560779664488942560E-35 ) ) ;
#928=CARTESIAN_POINT ( 'NONE',  ( -7.216878364870328078, 0.000000000000000000, -95.19198729810780435 ) ) ;
#933=EDGE_CURVE ( 'NONE', #5714, #6341, #12785, .T. ) ;
#934=( BOUNDED_CURVE ( )  B_SPLINE_CURVE ( 2, ( #21772, #10103, #29104, #3305, #19474, #12731, #22070, #10405, #17478 ),
 .UNSPECIFIED., .F., .T. ) 
 B_SPLINE_CURVE_WITH_KNOTS ( ( 3, 2, 2, 2, 3 ),
 ( 0.7305555555555556246, 0.7314814814814815103, 0.7333333333333332815, 0.7351851851851851638, 0.7361111111111110494 ),
 .UNSPECIFIED. ) 
 CURVE ( )  GEOMETRIC_REPRESENTATION_ITEM ( )  RATIONAL_B_SPLINE_CURVE ( ( 0.9330127018922194093, 0.9330127018922234061, 1.000000000000000000, 0.8660254037844388186, 1.000000000000000000, 0.8660254037844388186, 1.000000000000000000, 0.9330127018922234061, 0.9330127018922194093 ) ) 
 REPRESENTATION_ITEM ( '' )  );
#936=ORIENTED_EDGE ( 'NONE', *, *, #2428, .F. ) ;
#938=CARTESIAN_POINT ( 'NONE',  ( -4.763139720814407951, -2.750000000000016431, -56.49999999999999289 ) ) ;
#939=AXIS2_PLACEMENT_3D ( 'NONE', #2581, #2142, #18442 ) ;
#941=FACE_OUTER_BOUND ( 'NONE', #3694, .T. ) ;
#942=CARTESIAN_POINT ( 'NONE',  ( -5.412658773652739619, 3.124999999999975131, -78.18301270189220986 ) ) ;
#946=DIRECTION ( 'NONE',  ( -7.147005652999508048E-36, 5.642372883946980038E-36, 1.000000000000000000 ) ) ;
#947=CARTESIAN_POINT ( 'NONE',  ( 0.000000000000000000, 5.999999999999977796, -104.7113248654052455 ) ) ;
#948=CARTESIAN_POINT ( 'NONE',  ( 3.175426480543072749, -5.500000000000105693, -129.6250000000000284 ) ) ;
#951=CARTESIAN_POINT ( 'NONE',  ( 5.196152422706629359, 3.000000000000002665, -51.53867513459481131 ) ) ;
#952=CARTESIAN_POINT ( 'NONE',  ( -3.175426480542816066, 5.499999999999865885, -71.87500000000000000 ) ) ;
#954=CARTESIAN_POINT ( 'NONE',  ( 6.350852961086080661, -9.614813431917819062E-14, -55.87500000000003553 ) ) ;
#956=VERTEX_POINT ( 'NONE', #3206 ) ;
#959=CARTESIAN_POINT ( 'NONE',  ( 0.000000000000000000, 5.999999999999977796, -97.78867513459482552 ) ) ;
#961=CARTESIAN_POINT ( 'NONE',  ( -5.999999999999963585, -1.487416814333745711E-14, -167.9136751345948255 ) ) ;
#967=AXIS2_PLACEMENT_3D ( 'NONE', #10942, #18012, #27929 ) ;
#968=ADVANCED_FACE ( 'NONE', ( #1786 ), #908, .T. ) ;
#969=CYLINDRICAL_SURFACE ( 'NONE', #5964, 6.000000000000000888 ) ;
#970=CARTESIAN_POINT ( 'NONE',  ( -3.175426480542816510, -5.500000000000057732, -176.3750000000000284 ) ) ;
#972=CARTESIAN_POINT ( 'NONE',  ( -5.412658773652739619, 3.124999999999975131, -147.8169872981078186 ) ) ;
#974=CARTESIAN_POINT ( 'NONE',  ( 4.763139720814407951, 2.750000000000002665, -82.74999999999998579 ) ) ;
#975=ADVANCED_FACE ( 'NONE', ( #5513 ), #10306, .T. ) ;
#976=CARTESIAN_POINT ( 'NONE',  ( 2.775557561562891351E-14, 6.250000000000033751, -91.93301270189225249 ) ) ;
#982=DIRECTION ( 'NONE',  ( 1.000000000000000000, -5.551115123125773458E-17, -1.260129944081490338E-35 ) ) ;
#985=CARTESIAN_POINT ( 'NONE',  ( 4.763139720814407951, -2.749999999999988454, -165.4999999999999716 ) ) ;
#987=CARTESIAN_POINT ( 'NONE',  ( 3.175426480543072749, 5.499999999999865885, -145.6250000000000284 ) ) ;
#989=CARTESIAN_POINT ( 'NONE',  ( 0.000000000000000000, 0.000000000000000000, 0.000000000000000000 ) ) ;
#990=CARTESIAN_POINT ( 'NONE',  ( -3.175426480542816066, 5.499999999999865885, -94.37500000000002842 ) ) ;
#992=CARTESIAN_POINT ( 'NONE',  ( 0.000000000000000000, 5.499999999999991118, -78.00000000000001421 ) ) ;
#993=CARTESIAN_POINT ( 'NONE',  ( 0.000000000000000000, 0.000000000000000000, 0.000000000000000000 ) ) ;
#994=CARTESIAN_POINT ( 'NONE',  ( 6.000000000000000888, -1.607695154586752384, -72.15331216351299304 ) ) ;
#995=CARTESIAN_POINT ( 'NONE',  ( 6.000000000000052403, -1.607695154586662678, -108.1533121635129362 ) ) ;
#1002=CARTESIAN_POINT ( 'NONE',  ( 6.000000000000000888, 1.743066579297358182E-13, -78.66367513459482552 ) ) ;
#1010=CARTESIAN_POINT ( 'NONE',  ( -2.775557561562891351E-14, -5.500000000000115463, -102.7500000000000142 ) ) ;
#1012=CARTESIAN_POINT ( 'NONE',  ( 7.216878364870455975, -6.409875621278545621E-14, -116.3080127018922383 ) ) ;
#1015=CARTESIAN_POINT ( 'NONE',  ( 3.464101615137852974, 5.999999999999884537, -111.4136751345948113 ) ) ;
#1016=CARTESIAN_POINT ( 'NONE',  ( -3.608439182435115633, 6.249999999999965361, -158.4419872981077901 ) ) ;
#1018=CARTESIAN_POINT ( 'NONE',  ( -5.196152422706601826, 2.999999999999975131, -63.03867513459482552 ) ) ;
#1019=CARTESIAN_POINT ( 'NONE',  ( -3.608439182435115633, 6.249999999999965361, -60.30801270189223118 ) ) ;
#1021=DIRECTION ( 'NONE',  ( -7.147005652999508048E-36, 5.642372883946980038E-36, 1.000000000000000000 ) ) ;
#1022=( BOUNDED_CURVE ( )  B_SPLINE_CURVE ( 2, ( #24795, #13319, #10381, #3742, #29082, #17457, #26771, #1446, #29558 ),
 .UNSPECIFIED., .F., .F. ) 
 B_SPLINE_CURVE_WITH_KNOTS ( ( 3, 2, 2, 2, 3 ),
 ( 0.2249999999999999778, 0.2259259259259259189, 0.2277777777777777735, 0.2296296296296296280, 0.2305555555555555691 ),
 .UNSPECIFIED. ) 
 CURVE ( )  GEOMETRIC_REPRESENTATION_ITEM ( )  RATIONAL_B_SPLINE_CURVE ( ( 0.9330127018922196314, 0.9330127018922185211, 1.000000000000000000, 0.8660254037844388186, 1.000000000000000000, 0.8660254037844388186, 1.000000000000000000, 0.9330127018922184101, 0.9330127018922194093 ) ) 
 REPRESENTATION_ITEM ( '' )  );
#1023=CARTESIAN_POINT ( 'NONE',  ( -5.196152422706573404, -3.000000000000002665, -56.78867513459484684 ) ) ;
#1024=CARTESIAN_POINT ( 'NONE',  ( -5.999999999999963585, 1.780251999655701777E-13, -62.33632486540522422 ) ) ;
#1026=CARTESIAN_POINT ( 'NONE',  ( 4.763139720814407951, -2.749999999999988454, -174.5000000000000000 ) ) ;
#1029=CARTESIAN_POINT ( 'NONE',  ( -3.608439182435115633, 6.249999999999965361, -165.3080127018922667 ) ) ;
#1030=CARTESIAN_POINT ( 'NONE',  ( 6.000000000000000888, -3.330669073875464691E-16, -7.560779664488942560E-35 ) ) ;
#1032=CARTESIAN_POINT ( 'NONE',  ( 6.350852961086080661, -9.614813431917819062E-14, -112.8750000000000568 ) ) ;
#1034=CARTESIAN_POINT ( 'NONE',  ( 3.175426480543072749, -5.500000000000105693, -102.6250000000000000 ) ) ;
#1037=CARTESIAN_POINT ( 'NONE',  ( -5.999999999999963585, 1.780251999655701777E-13, -112.4136751345948255 ) ) ;
#1039=CARTESIAN_POINT ( 'NONE',  ( -5.999999999999963585, 8.134310703387671600E-14, -144.8363248654052029 ) ) ;
#1041=ORIENTED_EDGE ( 'NONE', *, *, #16511, .T. ) ;
#1043=DIRECTION ( 'NONE',  ( -7.147005652999508048E-36, 5.642372883946980038E-36, 1.000000000000000000 ) ) ;
#1046=CARTESIAN_POINT ( 'NONE',  ( -3.175426480542816510, 5.499999999999865885, -160.3750000000000000 ) ) ;
#1047=CARTESIAN_POINT ( 'NONE',  ( -3.464101615137725076, 5.999999999999979572, -65.58632486540523132 ) ) ;
#1050=CARTESIAN_POINT ( 'NONE',  ( 2.775557561562891351E-14, 6.250000000000033751, -85.06698729810780435 ) ) ;
#1052=CARTESIAN_POINT ( 'NONE',  ( 6.000000000000052403, -1.607695154586662678, -102.7306624327026014 ) ) ;
#1060=CARTESIAN_POINT ( 'NONE',  ( 5.412658773652712085, -3.125000000000086153, -141.9330127018922383 ) ) ;
#1061=ORIENTED_EDGE ( 'NONE', *, *, #15386, .T. ) ;
#1063=CARTESIAN_POINT ( 'NONE',  ( 2.775557561562891351E-14, -6.250000000000061284, -130.8169872981078186 ) ) ;
#1064=CARTESIAN_POINT ( 'NONE',  ( 6.000000000000000888, -1.607695154586752384, -135.1533121635129646 ) ) ;
#1065=CARTESIAN_POINT ( 'NONE',  ( 6.000000000000000888, 1.743066579297358182E-13, -50.16367513459482552 ) ) ;
#1072=CARTESIAN_POINT ( 'NONE',  ( 3.464101615137852974, 5.999999999999884537, -46.33632486540520290 ) ) ;
#1073=CARTESIAN_POINT ( 'NONE',  ( -5.412658773652739619, 3.124999999999975131, -65.31698729810780435 ) ) ;
#1074=VECTOR ( 'NONE', #6895, 1000.000000000000000 ) ;
#1075=CARTESIAN_POINT ( 'NONE',  ( 3.608439182435180470, 6.249999999999982236, -55.19198729810779724 ) ) ;
#1078=DIRECTION ( 'NONE',  ( -7.147005652999508048E-36, 5.642372883946980038E-36, 1.000000000000000000 ) ) ;
#1079=CARTESIAN_POINT ( 'NONE',  ( -3.175426480542816510, -5.500000000000057732, -131.3750000000000000 ) ) ;
#1081=ORIENTED_EDGE ( 'NONE', *, *, #14582, .F. ) ;
#1085=CARTESIAN_POINT ( 'NONE',  ( 6.000000000000000888, 7.762456499804235646E-14, -128.1636751345948539 ) ) ;
#1086=VERTEX_POINT ( 'NONE', #10382 ) ;
#1088=LINE ( 'NONE', #8141, #5633 ) ;
#1091=LINE ( 'NONE', #16959, #11184 ) ;
#1095=FACE_OUTER_BOUND ( 'NONE', #24456, .T. ) ;
#1098=CARTESIAN_POINT ( 'NONE',  ( -4.763139720814407951, -2.750000000000016431, -50.49999999999998579 ) ) ;
#1100=FACE_OUTER_BOUND ( 'NONE', #19908, .T. ) ;
#1102=CARTESIAN_POINT ( 'NONE',  ( 0.000000000000000000, 5.999999999999977796, -169.2113248654052313 ) ) ;
#1105=CARTESIAN_POINT ( 'NONE',  ( -4.763139720814407951, -2.750000000000016431, -128.5000000000000000 ) ) ;
#1108=CARTESIAN_POINT ( 'NONE',  ( 4.763139720814407951, 2.750000000000002665, -60.25000000000002842 ) ) ;
#1109=CARTESIAN_POINT ( 'NONE',  ( -6.350852961085760029, -1.281975124255709124E-13, -53.62500000000002842 ) ) ;
#1110=ORIENTED_EDGE ( 'NONE', *, *, #6647, .T. ) ;
#1114=CARTESIAN_POINT ( 'NONE',  ( 6.000000000000052403, -1.607695154586662678, -98.23066243270257303 ) ) ;
#1117=EDGE_CURVE ( 'NONE', #22297, #28019, #20626, .T. ) ;
#1122=EDGE_LOOP ( 'NONE', ( #29042, #12206, #2437, #3414 ) ) ;
#1123=CARTESIAN_POINT ( 'NONE',  ( 6.350852961086080661, -9.614813431917819062E-14, -147.3750000000000284 ) ) ;
#1124=CARTESIAN_POINT ( 'NONE',  ( -5.412658773652684552, -3.125000000000099920, -50.06698729810782567 ) ) ;
#1126=EDGE_LOOP ( 'NONE', ( #23177, #6889, #6796, #29307 ) ) ;
#1127=CARTESIAN_POINT ( 'NONE',  ( -5.412658773652739619, 3.124999999999975131, -150.8169872981078186 ) ) ;
#1128=CARTESIAN_POINT ( 'NONE',  ( -4.763139720814407951, -2.750000000000016431, -71.50000000000001421 ) ) ;
#1129=CARTESIAN_POINT ( 'NONE',  ( 3.608439182435180470, -6.249999999999997335, -97.05801270189228092 ) ) ;
#1131=CARTESIAN_POINT ( 'NONE',  ( -3.464101615137757051, -5.999999999999979572, -96.58632486540517448 ) ) ;
#1132=LINE ( 'NONE', #5889, #21951 ) ;
#1133=CARTESIAN_POINT ( 'NONE',  ( -5.999999999999963585, 1.780251999655701777E-13, -98.33632486540520290 ) ) ;
#1135=CARTESIAN_POINT ( 'NONE',  ( 3.175426480543072749, 5.499999999999865885, -157.6250000000000284 ) ) ;
#1136=CARTESIAN_POINT ( 'NONE',  ( 0.000000000000000000, 0.000000000000000000, -185.0000000000000000 ) ) ;
#1137=CARTESIAN_POINT ( 'NONE',  ( 6.350852961086080661, -9.614813431917819062E-14, -150.3749999999999716 ) ) ;
#1138=DIRECTION ( 'NONE',  ( -7.147005652999508048E-36, 5.642372883946980038E-36, 1.000000000000000000 ) ) ;
#1142=CARTESIAN_POINT ( 'NONE',  ( 3.175426480543072749, -5.500000000000105693, -92.12500000000002842 ) ) ;
#1144=CARTESIAN_POINT ( 'NONE',  ( -4.763139720814407951, 2.749999999999946709, -77.74999999999998579 ) ) ;
#1145=CARTESIAN_POINT ( 'NONE',  ( -3.464101615137725076, 5.999999999999979572, -164.5863248654051745 ) ) ;
#1146=CARTESIAN_POINT ( 'NONE',  ( 6.000000000000000888, 1.743066579297358182E-13, -108.0863248654051745 ) ) ;
#1147=CYLINDRICAL_SURFACE ( 'NONE', #12388, 6.000000000000000888 ) ;
#1149=CARTESIAN_POINT ( 'NONE',  ( 5.196152422706629359, 3.000000000000002665, -134.9613248654052313 ) ) ;
#1150=CARTESIAN_POINT ( 'NONE',  ( 5.999999999999993783, 1.607695154586726627, -174.5966878364870638 ) ) ;
#1151=EDGE_CURVE ( 'NONE', #14341, #27647, #10219, .T. ) ;
#1152=ORIENTED_EDGE ( 'NONE', *, *, #25660, .T. ) ;
#1154=VERTEX_POINT ( 'NONE', #12860 ) ;
#1157=CARTESIAN_POINT ( 'NONE',  ( -3.175426480542816510, -5.500000000000057732, -102.8750000000000142 ) ) ;
#1158=DIRECTION ( 'NONE',  ( -7.147005652999508048E-36, 5.642372883946980038E-36, 1.000000000000000000 ) ) ;
#1159=CARTESIAN_POINT ( 'NONE',  ( -7.216878364870328078, 0.000000000000000000, -117.0580127018922383 ) ) ;
#1161=DIRECTION ( 'NONE',  ( 1.000000000000000000, -5.551115123125773458E-17, -1.260129944081490338E-35 ) ) ;
#1164=CARTESIAN_POINT ( 'NONE',  ( -5.412658773652739619, 3.124999999999975131, -52.68301270189223828 ) ) ;
#1166=CARTESIAN_POINT ( 'NONE',  ( -5.999999999999919176, 1.607695154586804565, -167.4033121635129930 ) ) ;
#1167=CARTESIAN_POINT ( 'NONE',  ( 6.000000000000000000, 2.951592740943527306E-14, -162.0863248654052029 ) ) ;
#1169=CARTESIAN_POINT ( 'NONE',  ( 4.763139720814407951, -2.749999999999988454, -167.0000000000000284 ) ) ;
#1172=CARTESIAN_POINT ( 'NONE',  ( 3.608439182435180470, 6.249999999999982236, -167.0580127018922383 ) ) ;
#1173=CARTESIAN_POINT ( 'NONE',  ( 5.196152422706629359, 3.000000000000002665, -48.53867513459481131 ) ) ;
#1174=EDGE_CURVE ( 'NONE', #6115, #21171, #17488, .T. ) ;
#1175=CARTESIAN_POINT ( 'NONE',  ( -3.175426480542816066, 5.499999999999865885, -116.8750000000000000 ) ) ;
#1177=CARTESIAN_POINT ( 'NONE',  ( -6.350852961085760029, -1.281975124255709124E-13, -104.6250000000000142 ) ) ;
#1179=CARTESIAN_POINT ( 'NONE',  ( 6.000000000000052403, -1.607695154586662678, -87.15331216351297883 ) ) ;
#1181=ORIENTED_EDGE ( 'NONE', *, *, #24077, .T. ) ;
#1183=CARTESIAN_POINT ( 'NONE',  ( -6.000000000000000888, 1.067854986875958443E-15, 7.560779664488942560E-35 ) ) ;
#1186=ADVANCED_FACE ( 'NONE', ( #6969 ), #23283, .T. ) ;
#1187=EDGE_LOOP ( 'NONE', ( #5977, #17515, #27970, #21972 ) ) ;
#1188=CARTESIAN_POINT ( 'NONE',  ( 4.763139720814407951, 2.750000000000002665, -160.7500000000000568 ) ) ;
#1189=CARTESIAN_POINT ( 'NONE',  ( -5.999999999999962697, 3.323446944526963891E-14, -155.9136751345948255 ) ) ;
#1190=CARTESIAN_POINT ( 'NONE',  ( 2.775557561562891351E-14, 6.250000000000033751, -80.56698729810784698 ) ) ;
#1191=CARTESIAN_POINT ( 'NONE',  ( 5.196152422706629359, -2.999999999999988898, -129.2113248654052029 ) ) ;
#1198=ORIENTED_EDGE ( 'NONE', *, *, #12923, .F. ) ;
#1199=CARTESIAN_POINT ( 'NONE',  ( -7.216878364870328078, 0.000000000000000000, -126.6919872981078186 ) ) ;
#1200=CARTESIAN_POINT ( 'NONE',  ( 6.350852961086080661, -9.614813431917819062E-14, -169.8750000000000568 ) ) ;
#1201=ORIENTED_EDGE ( 'NONE', *, *, #28205, .T. ) ;
#1205=( BOUNDED_CURVE ( )  B_SPLINE_CURVE ( 2, ( #1262, #8493, #17587, #15285, #1422, #13444, #20183, #10673, #29680 ),
 .UNSPECIFIED., .F., .T. ) 
 B_SPLINE_CURVE_WITH_KNOTS ( ( 3, 2, 2, 2, 3 ),
 ( 0.9472222222222221877, 0.9481481481481481843, 0.9499999999999999556, 0.9518518518518518379, 0.9527777777777778345 ),
 .UNSPECIFIED. ) 
 CURVE ( )  GEOMETRIC_REPRESENTATION_ITEM ( )  RATIONAL_B_SPLINE_CURVE ( ( 0.9330127018922194093, 0.9330127018922154125, 1.000000000000000000, 0.8660254037844388186, 1.000000000000000000, 0.8660254037844388186, 1.000000000000000000, 0.9330127018922154125, 0.9330127018922194093 ) ) 
 REPRESENTATION_ITEM ( '' )  );
#1211=CARTESIAN_POINT ( 'NONE',  ( -3.608439182435115633, 6.249999999999965361, -66.94198729810787540 ) ) ;
#1212=CARTESIAN_POINT ( 'NONE',  ( 2.775557561562891351E-14, 6.250000000000033751, -56.56698729810783277 ) ) ;
#1214=ADVANCED_FACE ( 'NONE', ( #11475 ), #20499, .T. ) ;
#1215=CARTESIAN_POINT ( 'NONE',  ( 6.000000000000000000, 2.951592740943527306E-14, -153.0863248654052029 ) ) ;
#1216=CARTESIAN_POINT ( 'NONE',  ( -3.175426480542816510, 5.499999999999865885, -125.8749999999999858 ) ) ;
#1218=CARTESIAN_POINT ( 'NONE',  ( -5.196152422706601826, 2.999999999999975131, -166.5386751345948539 ) ) ;
#1222=AXIS2_PLACEMENT_3D ( 'NONE', #19173, #2861, #23774 ) ;
#1223=CARTESIAN_POINT ( 'NONE',  ( -5.999999999999963585, 1.780251999655701777E-13, -68.33632486540521711 ) ) ;
#1227=CARTESIAN_POINT ( 'NONE',  ( 3.464101615137757051, -5.999999999999979572, -147.9136751345947971 ) ) ;
#1228=EDGE_LOOP ( 'NONE', ( #5885, #18243, #10727, #28847 ) ) ;
#1230=CYLINDRICAL_SURFACE ( 'NONE', #23312, 6.000000000000000888 ) ;
#1231=CARTESIAN_POINT ( 'NONE',  ( 7.216878364870455975, -6.409875621278545621E-14, -94.44198729810780435 ) ) ;
#1235=VERTEX_POINT ( 'NONE', #8834 ) ;
#1240=VECTOR ( 'NONE', #11493, 1000.000000000000000 ) ;
#1241=CARTESIAN_POINT ( 'NONE',  ( -2.775557561562891351E-14, -5.500000000000115463, -50.25000000000001421 ) ) ;
#1243=CARTESIAN_POINT ( 'NONE',  ( -5.999999999999963585, -1.487416814333745711E-14, -134.9136751345948255 ) ) ;
#1245=CARTESIAN_POINT ( 'NONE',  ( -5.412658773652684552, -3.125000000000099920, -71.93301270189222407 ) ) ;
#1246=DIRECTION ( 'NONE',  ( 1.000000000000000000, -5.551115123125773458E-17, -1.260129944081490338E-35 ) ) ;
#1250=( BOUNDED_CURVE ( )  B_SPLINE_CURVE ( 2, ( #18450, #23048, #27922, #4439, #25639, #4288, #22892, #16464, #25793 ),
 .UNSPECIFIED., .F., .F. ) 
 B_SPLINE_CURVE_WITH_KNOTS ( ( 3, 2, 2, 2, 3 ),
 ( 0.6416666666666666075, 0.6425925925925926041, 0.6444444444444443754, 0.6462962962962963687, 0.6472222222222221433 ),
 .UNSPECIFIED. ) 
 CURVE ( )  GEOMETRIC_REPRESENTATION_ITEM ( )  RATIONAL_B_SPLINE_CURVE ( ( 0.9330127018922194093, 0.9330127018922154125, 1.000000000000000000, 0.8660254037844388186, 1.000000000000000000, 0.8660254037844388186, 1.000000000000000000, 0.9330127018922274029, 0.9330127018922194093 ) ) 
 REPRESENTATION_ITEM ( '' )  );
#1251=CARTESIAN_POINT ( 'NONE',  ( 3.464101615137757051, -5.999999999999979572, -152.4136751345947971 ) ) ;
#1252=ADVANCED_FACE ( 'NONE', ( #6513 ), #13620, .T. ) ;
#1253=CARTESIAN_POINT ( 'NONE',  ( -5.999999999999963585, 1.780251999655701777E-13, -104.3363248654052313 ) ) ;
#1255=CARTESIAN_POINT ( 'NONE',  ( -4.763139720814407951, 2.749999999999946709, -128.7500000000000284 ) ) ;
#1256=CARTESIAN_POINT ( 'NONE',  ( -5.999999999999963585, 3.021315404115421074E-15, -177.8363248654052029 ) ) ;
#1257=CARTESIAN_POINT ( 'NONE',  ( -6.000000000000000888, 1.067854986875958443E-15, 7.560779664488942560E-35 ) ) ;
#1259=VECTOR ( 'NONE', #23001, 1000.000000000000000 ) ;
#1260=CARTESIAN_POINT ( 'NONE',  ( -4.763139720814407951, -2.750000000000016431, -67.00000000000000000 ) ) ;
#1261=CARTESIAN_POINT ( 'NONE',  ( -3.175426480542816510, 5.499999999999865885, -58.37500000000004974 ) ) ;
#1262=CARTESIAN_POINT ( 'NONE',  ( 6.000000000000001776, 5.345404176511898156E-15, -174.0863248654052597 ) ) ;
#1263=ORIENTED_EDGE ( 'NONE', *, *, #10873, .F. ) ;
#1266=CARTESIAN_POINT ( 'NONE',  ( 0.000000000000000000, 0.000000000000000000, 0.000000000000000000 ) ) ;
#1273=CARTESIAN_POINT ( 'NONE',  ( 5.999999999999949374, -1.607695154586841868, -121.6533121635130215 ) ) ;
#1274=ORIENTED_EDGE ( 'NONE', *, *, #7037, .T. ) ;
#1276=CARTESIAN_POINT ( 'NONE',  ( 0.000000000000000000, 5.499999999999991118, -145.5000000000000284 ) ) ;
#1277=CARTESIAN_POINT ( 'NONE',  ( 2.775557561562891351E-14, -6.250000000000061284, -48.31698729810784698 ) ) ;
#1280=CARTESIAN_POINT ( 'NONE',  ( 2.775557561562891351E-14, 6.250000000000033751, -146.5669872981077901 ) ) ;
#1281=CARTESIAN_POINT ( 'NONE',  ( -3.175426480542816510, -5.500000000000057732, -71.37499999999997158 ) ) ;
#1282=CARTESIAN_POINT ( 'NONE',  ( -5.412658773652684552, -3.125000000000099920, -91.43301270189225249 ) ) ;
#1283=CARTESIAN_POINT ( 'NONE',  ( -3.035671606378273601, -10.57820549248702413, -19.81012201018820207 ) ) ;
#1285=DIRECTION ( 'NONE',  ( -7.147005652999508048E-36, 5.642372883946980038E-36, 1.000000000000000000 ) ) ;
#1287=CARTESIAN_POINT ( 'NONE',  ( 6.000000000000000888, 1.743066579297358182E-13, -64.58632486540520290 ) ) ;
#1290=CARTESIAN_POINT ( 'NONE',  ( 4.763139720814407951, 2.750000000000002665, -154.7500000000000568 ) ) ;
#1292=CARTESIAN_POINT ( 'NONE',  ( -2.775557561562891351E-14, -5.500000000000115463, -147.7500000000000568 ) ) ;
#1293=CARTESIAN_POINT ( 'NONE',  ( -2.846577545692754452, 4.964493094582011601, -180.0000000000000568 ) ) ;
#1294=CARTESIAN_POINT ( 'NONE',  ( 4.763139720814407951, -2.749999999999988454, -83.00000000000001421 ) ) ;
#1297=CARTESIAN_POINT ( 'NONE',  ( -2.775557561562891351E-14, -5.500000000000115463, -84.74999999999998579 ) ) ;
#1299=CARTESIAN_POINT ( 'NONE',  ( 0.000000000000000000, 0.000000000000000000, 0.000000000000000000 ) ) ;
#1304=CARTESIAN_POINT ( 'NONE',  ( -5.999999999999962697, 3.323446944526963891E-14, -149.9136751345948255 ) ) ;
#1307=CARTESIAN_POINT ( 'NONE',  ( 0.000000000000000000, 0.000000000000000000, 0.000000000000000000 ) ) ;
#1308=ORIENTED_EDGE ( 'NONE', *, *, #3958, .T. ) ;
#1311=CARTESIAN_POINT ( 'NONE',  ( 5.196152422706629359, 3.000000000000002665, -80.96132486540518869 ) ) ;
#1313=ORIENTED_EDGE ( 'NONE', *, *, #1406, .F. ) ;
#1315=EDGE_LOOP ( 'NONE', ( #26283, #787, #24719, #15620 ) ) ;
#1316=ADVANCED_FACE ( 'NONE', ( #205 ), #7283, .T. ) ;
#1317=CARTESIAN_POINT ( 'NONE',  ( 3.175426480543072749, -5.500000000000105693, -99.62500000000007105 ) ) ;
#1318=AXIS2_PLACEMENT_3D ( 'NONE', #14407, #23448, #7138 ) ;
#1320=CARTESIAN_POINT ( 'NONE',  ( 3.608439182435180470, -6.249999999999997335, -112.0580127018922241 ) ) ;
#1321=ORIENTED_EDGE ( 'NONE', *, *, #25861, .F. ) ;
#1322=CARTESIAN_POINT ( 'NONE',  ( -5.196152422706601826, 2.999999999999975131, -140.4613248654052029 ) ) ;
#1324=CARTESIAN_POINT ( 'NONE',  ( -7.216878364870328078, 0.000000000000000000, -52.55801270189219565 ) ) ;
#1328=EDGE_CURVE ( 'NONE', #891, #6568, #7854, .T. ) ;
#1329=DIRECTION ( 'NONE',  ( -7.147005652999508048E-36, 5.642372883946980038E-36, 1.000000000000000000 ) ) ;
#1332=CARTESIAN_POINT ( 'NONE',  ( -4.763139720814407951, -2.750000000000016431, -172.0000000000000284 ) ) ;
#1334=CARTESIAN_POINT ( 'NONE',  ( -3.464101615137757051, -5.999999999999979572, -158.0863248654051461 ) ) ;
#1335=CARTESIAN_POINT ( 'NONE',  ( -3.608439182435052128, -6.250000000000110134, -169.3080127018922383 ) ) ;
#1337=CARTESIAN_POINT ( 'NONE',  ( 3.175426480543072749, -5.500000000000105693, -108.6250000000000426 ) ) ;
#1339=CARTESIAN_POINT ( 'NONE',  ( 6.350852961086080661, -9.614813431917819062E-14, -105.3750000000000142 ) ) ;
#1342=AXIS2_PLACEMENT_3D ( 'NONE', #6536, #15958, #2095 ) ;
#1343=ORIENTED_EDGE ( 'NONE', *, *, #17804, .T. ) ;
#1345=CARTESIAN_POINT ( 'NONE',  ( -5.196152422706573404, -3.000000000000002665, -90.71132486540523132 ) ) ;
#1350=CARTESIAN_POINT ( 'NONE',  ( -5.412658773652739619, 3.124999999999975131, -84.81698729810783277 ) ) ;
#1353=EDGE_LOOP ( 'NONE', ( #22306, #16440, #26957, #9386 ) ) ;
#1354=LINE ( 'NONE', #15056, #20895 ) ;
#1355=VECTOR ( 'NONE', #18169, 1000.000000000000000 ) ;
#1356=EDGE_LOOP ( 'NONE', ( #20099, #18143, #1741, #23491 ) ) ;
#1357=VERTEX_POINT ( 'NONE', #28452 ) ;
#1360=CARTESIAN_POINT ( 'NONE',  ( -6.350852961085760029, -1.281975124255709124E-13, -119.6250000000000142 ) ) ;
#1361=CARTESIAN_POINT ( 'NONE',  ( 5.412658773652739619, 3.124999999999988898, -138.6830127018922099 ) ) ;
#1364=CARTESIAN_POINT ( 'NONE',  ( 3.608439182435180470, -6.249999999999997335, -120.1919872981077901 ) ) ;
#1366=CARTESIAN_POINT ( 'NONE',  ( 3.175426480543072749, 5.499999999999865885, -175.6250000000000284 ) ) ;
#1371=EDGE_CURVE ( 'NONE', #2905, #26686, #29456, .T. ) ;
#1372=CARTESIAN_POINT ( 'NONE',  ( -3.464101615137725076, 5.999999999999979572, -148.0863248654052029 ) ) ;
#1374=CARTESIAN_POINT ( 'NONE',  ( 6.000000000000000888, -1.607695154586752384, -54.73066243270260856 ) ) ;
#1376=CARTESIAN_POINT ( 'NONE',  ( 5.412658773652739619, 3.124999999999988898, -68.81698729810781856 ) ) ;
#1377=CARTESIAN_POINT ( 'NONE',  ( -5.412658773652684552, -3.125000000000099920, -57.56698729810783277 ) ) ;
#1378=CARTESIAN_POINT ( 'NONE',  ( 6.000000000000000888, -1.859271017917181981E-14, -120.6636751345948255 ) ) ;
#1379=CARTESIAN_POINT ( 'NONE',  ( -5.196152422706573404, -3.000000000000002665, -64.28867513459479710 ) ) ;
#1380=CARTESIAN_POINT ( 'NONE',  ( 0.000000000000000000, 5.999999999999977796, -55.78867513459484684 ) ) ;
#1382=CARTESIAN_POINT ( 'NONE',  ( -4.763139720814407951, -2.750000000000016431, -128.5000000000000000 ) ) ;
#1383=ORIENTED_EDGE ( 'NONE', *, *, #1753, .T. ) ;
#1387=CARTESIAN_POINT ( 'NONE',  ( 5.196152422706629359, 3.000000000000002665, -130.4613248654051745 ) ) ;
#1388=CARTESIAN_POINT ( 'NONE',  ( 6.000000000000000888, -3.330669073875464691E-16, -7.560779664488942560E-35 ) ) ;
#1392=CARTESIAN_POINT ( 'NONE',  ( 2.775557561562891351E-14, -6.250000000000061284, -112.8169872981078470 ) ) ;
#1394=( BOUNDED_CURVE ( )  B_SPLINE_CURVE ( 2, ( #16594, #11373, #23336, #27901, #20870, #28206, #23487, #25288, #6875 ),
 .UNSPECIFIED., .F., .T. ) 
 B_SPLINE_CURVE_WITH_KNOTS ( ( 3, 2, 2, 2, 3 ),
 ( 0.2916666666666666297, 0.2925925925925926263, 0.2944444444444443976, 0.2962962962962962798, 0.2972222222222222765 ),
 .UNSPECIFIED. ) 
 CURVE ( )  GEOMETRIC_REPRESENTATION_ITEM ( )  RATIONAL_B_SPLINE_CURVE ( ( 0.9330127018922194093, 0.9330127018922154125, 1.000000000000000000, 0.8660254037844388186, 1.000000000000000000, 0.8660254037844388186, 1.000000000000000000, 0.9330127018922154125, 0.9330127018922194093 ) ) 
 REPRESENTATION_ITEM ( '' )  );
#1397=EDGE_LOOP ( 'NONE', ( #6849, #11106, #18173, #7701 ) ) ;
#1398=CYLINDRICAL_SURFACE ( 'NONE', #13043, 6.000000000000000888 ) ;
#1402=CARTESIAN_POINT ( 'NONE',  ( -5.999999999999971578, 1.607695154586715303, -80.98066243270260145 ) ) ;
#1403=CARTESIAN_POINT ( 'NONE',  ( -2.775557561562891351E-14, -5.500000000000115463, -48.75000000000001421 ) ) ;
#1404=CARTESIAN_POINT ( 'NONE',  ( 6.000000000000000888, 1.743066579297358182E-13, -90.08632486540521711 ) ) ;
#1406=EDGE_CURVE ( 'NONE', #15772, #19941, #28840, .T. ) ;
#1408=CARTESIAN_POINT ( 'NONE',  ( 5.412658773652712085, -3.125000000000086153, -75.93301270189223828 ) ) ;
#1413=CARTESIAN_POINT ( 'NONE',  ( -5.999999999999963585, 1.780251999655701777E-13, -83.33632486540520290 ) ) ;
#1416=CARTESIAN_POINT ( 'NONE',  ( 3.175426480543072749, 5.499999999999865885, -135.1250000000000284 ) ) ;
#1418=CARTESIAN_POINT ( 'NONE',  ( -5.412658773652739619, 3.124999999999975131, -148.6830127018922099 ) ) ;
#1420=ORIENTED_EDGE ( 'NONE', *, *, #26541, .T. ) ;
#1421=CARTESIAN_POINT ( 'NONE',  ( 3.175426480543072749, 5.499999999999865885, -60.12500000000000000 ) ) ;
#1422=CARTESIAN_POINT ( 'NONE',  ( 0.000000000000000000, -5.999999999999991118, -174.4613248654052313 ) ) ;
#1423=ORIENTED_EDGE ( 'NONE', *, *, #29948, .F. ) ;
#1426=CARTESIAN_POINT ( 'NONE',  ( -5.999999999999956479, -1.607695154586745057, -118.3466878364870496 ) ) ;
#1434=EDGE_CURVE ( 'NONE', #2600, #448, #13380, .T. ) ;
#1435=CARTESIAN_POINT ( 'NONE',  ( -4.763139720814407951, -2.750000000000016431, -142.0000000000000284 ) ) ;
#1438=CARTESIAN_POINT ( 'NONE',  ( -3.608439182435052128, -6.250000000000110134, -48.44198729810783277 ) ) ;
#1441=CARTESIAN_POINT ( 'NONE',  ( -4.763139720814407951, 2.749999999999946709, -73.25000000000004263 ) ) ;
#1443=CARTESIAN_POINT ( 'NONE',  ( 2.775557561562891351E-14, -6.250000000000061284, -97.18301270189222407 ) ) ;
#1444=CARTESIAN_POINT ( 'NONE',  ( -3.979146954363663724, -10.25926384964412641, -20.49296196285819249 ) ) ;
#1445=CARTESIAN_POINT ( 'NONE',  ( 0.000000000000000000, 5.999999999999977796, -106.7886751345948397 ) ) ;
#1446=CARTESIAN_POINT ( 'NONE',  ( 6.000000000000014211, -1.607695154586730180, -150.7306624327026157 ) ) ;
#1447=CARTESIAN_POINT ( 'NONE',  ( 3.464101615137757051, -5.999999999999979572, -86.41367513459481131 ) ) ;
#1449=CARTESIAN_POINT ( 'NONE',  ( 4.763139720814407951, 2.750000000000002665, -153.2500000000000000 ) ) ;
#1451=DIRECTION ( 'NONE',  ( -7.147005652999508048E-36, 5.642372883946980038E-36, 1.000000000000000000 ) ) ;
#1453=AXIS2_PLACEMENT_3D ( 'NONE', #14881, #1021, #3029 ) ;
#1454=CARTESIAN_POINT ( 'NONE',  ( -6.350852961085760029, -1.281975124255709124E-13, -86.62500000000000000 ) ) ;
#1455=DIRECTION ( 'NONE',  ( 1.000000000000000000, -5.551115123125773458E-17, -1.260129944081490338E-35 ) ) ;
#1456=CARTESIAN_POINT ( 'NONE',  ( 3.175426480543072749, -5.500000000000105693, -84.62499999999998579 ) ) ;
#1457=CARTESIAN_POINT ( 'NONE',  ( 6.000000000000000888, 1.743066579297358182E-13, -74.16367513459483973 ) ) ;
#1463=EDGE_LOOP ( 'NONE', ( #15726, #20603, #7769, #24062 ) ) ;
#1467=EDGE_CURVE ( 'NONE', #28105, #1357, #29526, .T. ) ;
#1471=CARTESIAN_POINT ( 'NONE',  ( -4.763139720814407951, 2.749999999999946709, -97.25000000000000000 ) ) ;
#1472=AXIS2_PLACEMENT_3D ( 'NONE', #1633, #30044, #4389 ) ;
#1473=CARTESIAN_POINT ( 'NONE',  ( 5.196152422706629359, 3.000000000000002665, -96.53867513459479710 ) ) ;
#1474=CARTESIAN_POINT ( 'NONE',  ( 5.412658773652712085, -3.125000000000086153, -114.9330127018922667 ) ) ;
#1476=CARTESIAN_POINT ( 'NONE',  ( 6.000000000000000888, 7.762456499804235646E-14, -117.0863248654052171 ) ) ;
#1479=DIRECTION ( 'NONE',  ( -7.147005652999508048E-36, 5.642372883946980038E-36, 1.000000000000000000 ) ) ;
#1480=CARTESIAN_POINT ( 'NONE',  ( -5.412658773652684552, -3.125000000000099920, -52.43301270189226670 ) ) ;
#1482=CARTESIAN_POINT ( 'NONE',  ( 5.196152422706629359, 3.000000000000002665, -160.4613248654052029 ) ) ;
#1483=( BOUNDED_CURVE ( )  B_SPLINE_CURVE ( 2, ( #26051, #4994, #14427, #23764, #21461, #391, #9782, #2846, #28786 ),
 .UNSPECIFIED., .F., .T. ) 
 B_SPLINE_CURVE_WITH_KNOTS ( ( 3, 2, 2, 2, 3 ),
 ( 0.08611111111111113825, 0.08703703703703702388, 0.08888888888888890616, 0.09074074074074078844, 0.09166666666666667407 ),
 .UNSPECIFIED. ) 
 CURVE ( )  GEOMETRIC_REPRESENTATION_ITEM ( )  RATIONAL_B_SPLINE_CURVE ( ( 0.9330127018922194093, 0.9330127018922234061, 1.000000000000000000, 0.8660254037844388186, 1.000000000000000000, 0.8660254037844388186, 1.000000000000000000, 0.9330127018922194093, 0.9330127018922194093 ) ) 
 REPRESENTATION_ITEM ( '' )  );
#1486=CARTESIAN_POINT ( 'NONE',  ( 0.000000000000000000, 5.499999999999991118, -166.4999999999999716 ) ) ;
#1488=CARTESIAN_POINT ( 'NONE',  ( -6.350852961085760029, -1.281975124255709124E-13, -110.6249999999999716 ) ) ;
#1490=CARTESIAN_POINT ( 'NONE',  ( 0.000000000000000000, 5.499999999999991118, -106.5000000000000426 ) ) ;
#1496=VECTOR ( 'NONE', #7971, 1000.000000000000000 ) ;
#1498=DIRECTION ( 'NONE',  ( 1.000000000000000000, -5.551115123125773458E-17, -1.260129944081490338E-35 ) ) ;
#1500=CARTESIAN_POINT ( 'NONE',  ( 4.763139720814407951, -2.749999999999988454, -158.0000000000000284 ) ) ;
#1502=CARTESIAN_POINT ( 'NONE',  ( 2.775557561562891351E-14, -6.250000000000061284, -79.81698729810781856 ) ) ;
#1504=ORIENTED_EDGE ( 'NONE', *, *, #4500, .T. ) ;
#1505=FACE_OUTER_BOUND ( 'NONE', #16602, .T. ) ;
#1508=EDGE_LOOP ( 'NONE', ( #12148, #15683, #3081, #29216 ) ) ;
#1510=CARTESIAN_POINT ( 'NONE',  ( 3.175426480543072749, -5.500000000000105693, -119.1250000000000142 ) ) ;
#1511=CARTESIAN_POINT ( 'NONE',  ( 3.608439182435180470, -6.249999999999997335, -137.5580127018922099 ) ) ;
#1512=ORIENTED_EDGE ( 'NONE', *, *, #19591, .F. ) ;
#1514=CARTESIAN_POINT ( 'NONE',  ( -5.412658773652739619, 3.124999999999975131, -123.8169872981078612 ) ) ;
#1515=CARTESIAN_POINT ( 'NONE',  ( 2.775557561562891351E-14, -6.250000000000061284, -175.8169872981077901 ) ) ;
#1516=CARTESIAN_POINT ( 'NONE',  ( -3.175426480542816510, 5.499999999999865885, -169.3750000000000853 ) ) ;
#1519=ORIENTED_EDGE ( 'NONE', *, *, #17212, .T. ) ;
#1525=CARTESIAN_POINT ( 'NONE',  ( 6.000000000000000888, -1.859271017917181981E-14, -46.58632486540520290 ) ) ;
#1527=CARTESIAN_POINT ( 'NONE',  ( 5.412658773652739619, 3.124999999999988898, -65.81698729810780435 ) ) ;
#1528=CARTESIAN_POINT ( 'NONE',  ( -5.412658773652739619, 3.124999999999975131, -54.81698729810779724 ) ) ;
#1530=CARTESIAN_POINT ( 'NONE',  ( -4.763139720814407951, -2.750000000000016431, -52.00000000000004263 ) ) ;
#1531=CARTESIAN_POINT ( 'NONE',  ( -5.999999999999971578, 1.607695154586715303, -55.48066243270262987 ) ) ;
#1533=CARTESIAN_POINT ( 'NONE',  ( -6.350852961085760029, -1.281975124255709124E-13, -133.1250000000000284 ) ) ;
#1538=EDGE_CURVE ( 'NONE', #9651, #18552, #14062, .T. ) ;
#1539=( BOUNDED_CURVE ( )  B_SPLINE_CURVE ( 2, ( #28814, #7630, #26217, #3313, #14875, #22080, #10113, #21930, #17040 ),
 .UNSPECIFIED., .F., .F. ) 
 B_SPLINE_CURVE_WITH_KNOTS ( ( 3, 2, 2, 2, 3 ),
 ( 0.8916666666666666075, 0.8925925925925926041, 0.8944444444444444864, 0.8962962962962962576, 0.8972222222222222543 ),
 .UNSPECIFIED. ) 
 CURVE ( )  GEOMETRIC_REPRESENTATION_ITEM ( )  RATIONAL_B_SPLINE_CURVE ( ( 0.9330127018922194093, 0.9330127018922154125, 1.000000000000000000, 0.8660254037844388186, 1.000000000000000000, 0.8660254037844388186, 1.000000000000000000, 0.9330127018922154125, 0.9330127018922194093 ) ) 
 REPRESENTATION_ITEM ( '' )  );
#1540=CARTESIAN_POINT ( 'NONE',  ( 6.000000000000000888, -1.859271017917181981E-14, -58.58632486540521001 ) ) ;
#1541=DIRECTION ( 'NONE',  ( 1.000000000000000000, -5.551115123125773458E-17, -1.260129944081490338E-35 ) ) ;
#1543=ORIENTED_EDGE ( 'NONE', *, *, #25275, .T. ) ;
#1545=CARTESIAN_POINT ( 'NONE',  ( -5.999999999999963585, -1.487416814333745711E-14, -71.33632486540521711 ) ) ;
#1547=CARTESIAN_POINT ( 'NONE',  ( -5.412658773652739619, 3.124999999999975131, -119.3169872981078043 ) ) ;
#1551=EDGE_CURVE ( 'NONE', #30268, #2318, #19624, .T. ) ;
#1554=DIRECTION ( 'NONE',  ( 1.000000000000000000, -5.551115123125773458E-17, -1.260129944081490338E-35 ) ) ;
#1556=ORIENTED_EDGE ( 'NONE', *, *, #13694, .F. ) ;
#1558=ORIENTED_EDGE ( 'NONE', *, *, #20639, .T. ) ;
#1560=CARTESIAN_POINT ( 'NONE',  ( -6.350852961085760029, -1.281975124255709124E-13, -50.62500000000001421 ) ) ;
#1563=CARTESIAN_POINT ( 'NONE',  ( -5.999999999999956479, -1.607695154586745057, -80.26933756729744118 ) ) ;
#1564=CARTESIAN_POINT ( 'NONE',  ( 5.412658773652712085, -3.125000000000086153, -65.43301270189222407 ) ) ;
#1570=CARTESIAN_POINT ( 'NONE',  ( 6.000000000000000888, -1.859271017917181981E-14, -93.66367513459481131 ) ) ;
#1571=CARTESIAN_POINT ( 'NONE',  ( 3.175426480543072749, -5.500000000000105693, -134.1250000000000284 ) ) ;
#1572=CARTESIAN_POINT ( 'NONE',  ( 2.775557561562891351E-14, 6.250000000000033751, -148.9330127018922383 ) ) ;
#1576=CARTESIAN_POINT ( 'NONE',  ( 3.175426480543072749, 5.499999999999865885, -61.62500000000001421 ) ) ;
#1577=CARTESIAN_POINT ( 'NONE',  ( 0.000000000000000000, -5.999999999999991118, -76.96132486540518869 ) ) ;
#1579=ORIENTED_EDGE ( 'NONE', *, *, #3648, .F. ) ;
#1585=ADVANCED_FACE ( 'NONE', ( #6941 ), #16360, .T. ) ;
#1586=( BOUNDED_CURVE ( )  B_SPLINE_CURVE ( 2, ( #26131, #21396, #7254, #25986, #4931, #14362, #2634, #12054, #7541 ),
 .UNSPECIFIED., .F., .T. ) 
 B_SPLINE_CURVE_WITH_KNOTS ( ( 3, 2, 2, 2, 3 ),
 ( 0.4472222222222221877, 0.4481481481481481843, 0.4499999999999999556, 0.4518518518518518379, 0.4527777777777778345 ),
 .UNSPECIFIED. ) 
 CURVE ( )  GEOMETRIC_REPRESENTATION_ITEM ( )  RATIONAL_B_SPLINE_CURVE ( ( 0.9330127018922194093, 0.9330127018922154125, 1.000000000000000000, 0.8660254037844388186, 1.000000000000000000, 0.8660254037844388186, 1.000000000000000000, 0.9330127018922154125, 0.9330127018922194093 ) ) 
 REPRESENTATION_ITEM ( '' )  );
#1587=EDGE_CURVE ( 'NONE', #23232, #688, #22775, .T. ) ;
#1591=ORIENTED_EDGE ( 'NONE', *, *, #11046, .F. ) ;
#1592=CARTESIAN_POINT ( 'NONE',  ( -2.775557561562891351E-14, -5.500000000000115463, -149.2500000000000000 ) ) ;
#1593=ORIENTED_EDGE ( 'NONE', *, *, #12719, .F. ) ;
#1596=CARTESIAN_POINT ( 'NONE',  ( -4.763139720814407951, 2.749999999999946709, -76.25000000000004263 ) ) ;
#1598=CARTESIAN_POINT ( 'NONE',  ( -5.412658773652739619, 3.124999999999975131, -90.18301270189222407 ) ) ;
#1599=( GEOMETRIC_REPRESENTATION_CONTEXT ( 3 ) GLOBAL_UNCERTAINTY_ASSIGNED_CONTEXT ( ( #9739 ) ) GLOBAL_UNIT_ASSIGNED_CONTEXT ( ( #1638, #26049, #7009 ) ) REPRESENTATION_CONTEXT ( 'NONE', 'WORKASPACE' ) );
#1600=DIRECTION ( 'NONE',  ( -7.147005652999508048E-36, 5.642372883946980038E-36, 1.000000000000000000 ) ) ;
#1605=CARTESIAN_POINT ( 'NONE',  ( 4.763139720814407951, 2.750000000000002665, -156.2500000000000000 ) ) ;
#1607=CARTESIAN_POINT ( 'NONE',  ( -3.847734726282651341, 4.353436196510543255, -179.9999999999999716 ) ) ;
#1608=EDGE_CURVE ( 'NONE', #11104, #7154, #629, .T. ) ;
#1609=CARTESIAN_POINT ( 'NONE',  ( 4.763139720814407951, -2.749999999999988454, -84.50000000000001421 ) ) ;
#1610=CARTESIAN_POINT ( 'NONE',  ( -5.999999999999963585, 8.134310703387671600E-14, -140.9136751345947971 ) ) ;
#1611=CARTESIAN_POINT ( 'NONE',  ( -3.175426480542816510, -5.500000000000057732, -74.37500000000000000 ) ) ;
#1613=CARTESIAN_POINT ( 'NONE',  ( 0.000000000000000000, -5.999999999999991118, -120.4613248654052313 ) ) ;
#1615=CARTESIAN_POINT ( 'NONE',  ( -5.196152422706573404, -3.000000000000002665, -108.7113248654052455 ) ) ;
#1616=CARTESIAN_POINT ( 'NONE',  ( 0.000000000000000000, -5.999999999999991118, -149.5386751345948539 ) ) ;
#1620=EDGE_CURVE ( 'NONE', #1154, #14874, #25896, .T. ) ;
#1621=CARTESIAN_POINT ( 'NONE',  ( 5.999999999999949374, 1.607695154586804565, -75.59668783648704959 ) ) ;
#1625=ORIENTED_EDGE ( 'NONE', *, *, #20597, .F. ) ;
#1627=CARTESIAN_POINT ( 'NONE',  ( -3.175426480542816510, -5.500000000000057732, -101.3750000000000000 ) ) ;
#1629=CARTESIAN_POINT ( 'NONE',  ( 5.999999999999949374, 1.607695154586804565, -96.59668783648702117 ) ) ;
#1630=CARTESIAN_POINT ( 'NONE',  ( 7.216878364870455975, -6.409875621278545621E-14, -113.3080127018922241 ) ) ;
#1631=AXIS2_PLACEMENT_3D ( 'NONE', #14570, #21174, #9946 ) ;
#1632=CARTESIAN_POINT ( 'NONE',  ( 5.196152422706629359, 3.000000000000002665, -140.9613248654052597 ) ) ;
#1633=CARTESIAN_POINT ( 'NONE',  ( 5.551115123125782702E-14, 1.999999999999890754, -200.0000000000000000 ) ) ;
#1634=CARTESIAN_POINT ( 'NONE',  ( 3.464101615137757051, -5.999999999999979572, -143.4136751345948255 ) ) ;
#1635=CARTESIAN_POINT ( 'NONE',  ( 5.412658773652712085, -3.125000000000086153, -51.93301270189220986 ) ) ;
#1638=( LENGTH_UNIT ( ) NAMED_UNIT ( * ) SI_UNIT ( .MILLI., .METRE. ) );
#1640=CARTESIAN_POINT ( 'NONE',  ( 5.196152422706629359, 3.000000000000002665, -136.4613248654051745 ) ) ;
#1641=CARTESIAN_POINT ( 'NONE',  ( -3.175426480542816510, 5.499999999999865885, -161.8750000000000568 ) ) ;
#1644=ADVANCED_FACE ( 'NONE', ( #11569 ), #25657, .T. ) ;
#1645=CARTESIAN_POINT ( 'NONE',  ( 6.350852961086080661, -9.614813431917819062E-14, -109.8750000000000426 ) ) ;
#1647=CARTESIAN_POINT ( 'NONE',  ( 6.000000000000026645, -1.607695154586707753, -122.2306624327026014 ) ) ;
#1649=CARTESIAN_POINT ( 'NONE',  ( 0.000000000000000000, 5.499999999999991118, -99.00000000000002842 ) ) ;
#1650=CARTESIAN_POINT ( 'NONE',  ( -5.999999999999962697, 3.323446944526963891E-14, -151.4136751345948255 ) ) ;
#1658=EDGE_LOOP ( 'NONE', ( #28483, #28368, #823, #7689 ) ) ;
#1659=LINE ( 'NONE', #27591, #6925 ) ;
#1662=CARTESIAN_POINT ( 'NONE',  ( 3.608439182435180470, 6.249999999999982236, -89.69198729810783277 ) ) ;
#1663=CARTESIAN_POINT ( 'NONE',  ( 6.000000000000000888, 7.762456499804234384E-14, -129.0863248654052029 ) ) ;
#1665=CARTESIAN_POINT ( 'NONE',  ( -3.978158145384737221, 10.25965056898454009, -29.50791791133369912 ) ) ;
#1666=CARTESIAN_POINT ( 'NONE',  ( 3.175426480543072749, 5.499999999999865885, -151.6250000000000284 ) ) ;
#1669=CARTESIAN_POINT ( 'NONE',  ( -2.775557561562891351E-14, -5.500000000000115463, -125.2500000000000284 ) ) ;
#1670=( BOUNDED_CURVE ( )  B_SPLINE_CURVE ( 2, ( #12028, #23816, #21367, #16488, #25814, #9694, #28398, #21524, #449 ),
 .UNSPECIFIED., .F., .T. ) 
 B_SPLINE_CURVE_WITH_KNOTS ( ( 3, 2, 2, 2, 3 ),
 ( 0.7694444444444443754, 0.7703703703703703720, 0.7722222222222222543, 0.7740740740740740256, 0.7750000000000000222 ),
 .UNSPECIFIED. ) 
 CURVE ( )  GEOMETRIC_REPRESENTATION_ITEM ( )  RATIONAL_B_SPLINE_CURVE ( ( 0.9330127018922194093, 0.9330127018922154125, 1.000000000000000000, 0.8660254037844388186, 1.000000000000000000, 0.8660254037844388186, 1.000000000000000000, 0.9330127018922154125, 0.9330127018922194093 ) ) 
 REPRESENTATION_ITEM ( '' )  );
#1671=CARTESIAN_POINT ( 'NONE',  ( 7.216878364870455975, -6.409875621278545621E-14, -138.8080127018922667 ) ) ;
#1672=VERTEX_POINT ( 'NONE', #27635 ) ;
#1673=CARTESIAN_POINT ( 'NONE',  ( 6.000000000000000000, 2.951592740943527306E-14, -156.6636751345948255 ) ) ;
#1674=CARTESIAN_POINT ( 'NONE',  ( -5.412658773652739619, 3.124999999999975131, -120.8169872981078612 ) ) ;
#1675=CARTESIAN_POINT ( 'NONE',  ( 7.216878364870455975, -6.409875621278545621E-14, -178.4419872981078470 ) ) ;
#1676=CARTESIAN_POINT ( 'NONE',  ( -4.763139720814407951, 2.749999999999946709, -172.2500000000000000 ) ) ;
#1678=LINE ( 'NONE', #14418, #25045 ) ;
#1683=CARTESIAN_POINT ( 'NONE',  ( -5.999999999999963585, -1.487416814333745711E-14, -128.3363248654052029 ) ) ;
#1684=DIRECTION ( 'NONE',  ( -7.147005652999508048E-36, 5.642372883946980038E-36, 1.000000000000000000 ) ) ;
#1685=CARTESIAN_POINT ( 'NONE',  ( 3.608439182435180470, -6.249999999999997335, -76.69198729810784698 ) ) ;
#1686=CARTESIAN_POINT ( 'NONE',  ( 5.412658773652712085, -3.125000000000086153, -60.06698729810783277 ) ) ;
#1687=CARTESIAN_POINT ( 'NONE',  ( -3.464101615137757051, -5.999999999999979572, -121.1636751345947829 ) ) ;
#1688=CARTESIAN_POINT ( 'NONE',  ( -6.350852961085760029, -1.281975124255709124E-13, -49.12500000000000711 ) ) ;
#1692=CARTESIAN_POINT ( 'NONE',  ( 4.763139720814407951, 2.750000000000002665, -127.7500000000000284 ) ) ;
#1693=CARTESIAN_POINT ( 'NONE',  ( -5.196152422706601826, 2.999999999999975131, -50.46132486540522422 ) ) ;
#1695=CARTESIAN_POINT ( 'NONE',  ( -6.000000000000060396, -1.607695154586566089, -119.2693375672974554 ) ) ;
#1698=CARTESIAN_POINT ( 'NONE',  ( 6.000000000000000888, -1.607695154586752384, -147.7306624327026157 ) ) ;
#1699=VERTEX_POINT ( 'NONE', #6614 ) ;
#1703=CARTESIAN_POINT ( 'NONE',  ( -5.412658773652739619, 3.124999999999975131, -116.3169872981078043 ) ) ;
#1705=CARTESIAN_POINT ( 'NONE',  ( 6.000000000000000888, -1.859271017917181981E-14, -135.6636751345948255 ) ) ;
#1707=DIRECTION ( 'NONE',  ( -7.147005652999508048E-36, 5.642372883946980038E-36, 1.000000000000000000 ) ) ;
#1712=EDGE_CURVE ( 'NONE', #16735, #152, #4458, .T. ) ;
#1713=CARTESIAN_POINT ( 'NONE',  ( 4.763139720814407951, -2.749999999999988454, -47.00000000000004263 ) ) ;
#1717=CARTESIAN_POINT ( 'NONE',  ( 5.412658773652712085, -3.125000000000086153, -66.93301270189222407 ) ) ;
#1719=CARTESIAN_POINT ( 'NONE',  ( 0.000000000000000000, 0.000000000000000000, 0.000000000000000000 ) ) ;
#1726=CARTESIAN_POINT ( 'NONE',  ( -6.350852961085760029, -1.281975124255709124E-13, -124.1250000000000426 ) ) ;
#1728=ORIENTED_EDGE ( 'NONE', *, *, #3030, .F. ) ;
#1729=CARTESIAN_POINT ( 'NONE',  ( 6.350852961086080661, -9.614813431917819062E-14, -64.87500000000001421 ) ) ;
#1730=CARTESIAN_POINT ( 'NONE',  ( 0.000000000000000000, 5.999999999999977796, -124.2113248654052029 ) ) ;
#1731=CYLINDRICAL_SURFACE ( 'NONE', #14058, 6.000000000000000888 ) ;
#1733=VECTOR ( 'NONE', #1707, 1000.000000000000000 ) ;
#1736=CARTESIAN_POINT ( 'NONE',  ( 6.000000000000000888, 7.762456499804235646E-14, -119.1636751345948113 ) ) ;
#1740=CARTESIAN_POINT ( 'NONE',  ( 6.350852961086080661, -9.614813431917819062E-14, -144.3750000000000568 ) ) ;
#1741=ORIENTED_EDGE ( 'NONE', *, *, #4930, .T. ) ;
#1743=ORIENTED_EDGE ( 'NONE', *, *, #5754, .F. ) ;
#1745=CARTESIAN_POINT ( 'NONE',  ( 4.763139720814407951, -2.749999999999988454, -72.50000000000001421 ) ) ;
#1747=CARTESIAN_POINT ( 'NONE',  ( -7.216878364870328078, 0.000000000000000000, -88.55801270189223828 ) ) ;
#1749=CARTESIAN_POINT ( 'NONE',  ( -3.677985992802528692, -10.37237449091587038, -20.24368265486285168 ) ) ;
#1750=CARTESIAN_POINT ( 'NONE',  ( 6.000000000000000888, 1.743066579297358182E-13, -107.1636751345948539 ) ) ;
#1753=EDGE_CURVE ( 'NONE', #6341, #1235, #24733, .T. ) ;
#1755=( BOUNDED_CURVE ( )  B_SPLINE_CURVE ( 2, ( #27471, #3832, #22448, #22601, #16026, #4300, #10791, #6447, #13718 ),
 .UNSPECIFIED., .F., .T. ) 
 B_SPLINE_CURVE_WITH_KNOTS ( ( 3, 2, 2, 2, 3 ),
 ( 0.3194444444444444753, 0.3203703703703703609, 0.3222222222222222432, 0.3240740740740740700, 0.3250000000000000111 ),
 .UNSPECIFIED. ) 
 CURVE ( )  GEOMETRIC_REPRESENTATION_ITEM ( )  RATIONAL_B_SPLINE_CURVE ( ( 0.9330127018922194093, 0.9330127018922214077, 1.000000000000000000, 0.8660254037844388186, 1.000000000000000000, 0.8660254037844388186, 1.000000000000000000, 0.9330127018922194093, 0.9330127018922194093 ) ) 
 REPRESENTATION_ITEM ( '' )  );
#1756=CARTESIAN_POINT ( 'NONE',  ( 3.175426480543072749, 5.499999999999865885, -153.1250000000000853 ) ) ;
#1760=CARTESIAN_POINT ( 'NONE',  ( -4.763139720814407951, -2.750000000000016431, -88.00000000000002842 ) ) ;
#1761=CARTESIAN_POINT ( 'NONE',  ( -4.763139720814407951, 2.749999999999946709, -74.75000000000004263 ) ) ;
#1763=CARTESIAN_POINT ( 'NONE',  ( -5.999999999999963585, 1.780251999655701777E-13, -51.83632486540522422 ) ) ;
#1765=CARTESIAN_POINT ( 'NONE',  ( -5.999999999999956479, -1.607695154586745057, -76.34668783648700696 ) ) ;
#1768=CARTESIAN_POINT ( 'NONE',  ( 5.999999999999974243, 1.607695154586759934, -119.0966878364870354 ) ) ;
#1769=CARTESIAN_POINT ( 'NONE',  ( -5.196152422706601826, 2.999999999999975131, -134.4613248654051745 ) ) ;
#1770=CARTESIAN_POINT ( 'NONE',  ( 6.000000000000000888, -3.330669073875464691E-16, -7.560779664488942560E-35 ) ) ;
#1775=CARTESIAN_POINT ( 'NONE',  ( -3.464101615137725076, 5.999999999999979572, -157.0863248654051745 ) ) ;
#1780=CARTESIAN_POINT ( 'NONE',  ( 4.763139720814407951, -2.749999999999988454, -101.0000000000000284 ) ) ;
#1781=LINE ( 'NONE', #29587, #20442 ) ;
#1782=CARTESIAN_POINT ( 'NONE',  ( 3.608439182435180470, 6.249999999999982236, -104.0580127018922383 ) ) ;
#1784=CARTESIAN_POINT ( 'NONE',  ( -3.175426480542816510, 5.499999999999865885, -163.3750000000000568 ) ) ;
#1785=CARTESIAN_POINT ( 'NONE',  ( 5.412658773652712085, -3.125000000000086153, -53.43301270189226670 ) ) ;
#1786=FACE_OUTER_BOUND ( 'NONE', #8972, .T. ) ;
#1787=ORIENTED_EDGE ( 'NONE', *, *, #19661, .F. ) ;
#1788=EDGE_CURVE ( 'NONE', #688, #9162, #25493, .T. ) ;
#1789=CARTESIAN_POINT ( 'NONE',  ( 0.000000000000000000, 0.000000000000000000, 0.000000000000000000 ) ) ;
#1790=CARTESIAN_POINT ( 'NONE',  ( 6.350852961086080661, -9.614813431917819062E-14, -159.3750000000000284 ) ) ;
#1794=CARTESIAN_POINT ( 'NONE',  ( 4.763139720814407951, -2.749999999999988454, -105.5000000000000426 ) ) ;
#1797=CARTESIAN_POINT ( 'NONE',  ( 3.175426480543072749, -5.500000000000105693, -101.1250000000000000 ) ) ;
#1799=CARTESIAN_POINT ( 'NONE',  ( -3.464101615137725076, 5.999999999999979572, -162.1636751345948824 ) ) ;
#1801=VERTEX_POINT ( 'NONE', #30414 ) ;
#1809=CARTESIAN_POINT ( 'NONE',  ( -3.608439182435115633, 6.249999999999965361, -89.44198729810784698 ) ) ;
#1812=CARTESIAN_POINT ( 'NONE',  ( 5.196152422706629359, -2.999999999999988898, -65.28867513459479710 ) ) ;
#1814=ORIENTED_EDGE ( 'NONE', *, *, #25969, .F. ) ;
#1816=ORIENTED_EDGE ( 'NONE', *, *, #5303, .T. ) ;
#1818=CARTESIAN_POINT ( 'NONE',  ( -2.775557561562891351E-14, -5.500000000000115463, -117.7500000000000284 ) ) ;
#1821=CARTESIAN_POINT ( 'NONE',  ( 2.775557561562891351E-14, -6.250000000000061284, -128.6830127018922383 ) ) ;
#1822=ORIENTED_EDGE ( 'NONE', *, *, #29117, .T. ) ;
#1824=CARTESIAN_POINT ( 'NONE',  ( -5.412658773652684552, -3.125000000000099920, -126.5669872981078328 ) ) ;
#1825=CARTESIAN_POINT ( 'NONE',  ( -5.412658773652684552, -3.125000000000099920, -176.0669872981078186 ) ) ;
#1827=VERTEX_POINT ( 'NONE', #9692 ) ;
#1830=DIRECTION ( 'NONE',  ( -7.147005652999508048E-36, 5.642372883946980038E-36, 1.000000000000000000 ) ) ;
#1831=CARTESIAN_POINT ( 'NONE',  ( 5.196152422706629359, 3.000000000000002665, -90.53867513459485394 ) ) ;
#1836=CARTESIAN_POINT ( 'NONE',  ( -3.608439182435052128, -6.250000000000110134, -72.44198729810781856 ) ) ;
#1837=CARTESIAN_POINT ( 'NONE',  ( 3.608439182435180470, -6.249999999999997335, -58.69198729810781856 ) ) ;
#1839=CARTESIAN_POINT ( 'NONE',  ( -3.175426480542816510, -5.500000000000057732, -48.87500000000001421 ) ) ;
#1841=DIRECTION ( 'NONE',  ( -1.000000000000000000, 5.551115123125774690E-17, 0.000000000000000000 ) ) ;
#1843=CARTESIAN_POINT ( 'NONE',  ( 0.000000000000000000, 5.499999999999991118, -118.5000000000000568 ) ) ;
#1845=ORIENTED_EDGE ( 'NONE', *, *, #4106, .T. ) ;
#1847=CARTESIAN_POINT ( 'NONE',  ( 6.000000000000000888, 7.762456499804234384E-14, -123.0863248654052313 ) ) ;
#1849=ORIENTED_EDGE ( 'NONE', *, *, #13796, .T. ) ;
#1852=CARTESIAN_POINT ( 'NONE',  ( -3.608439182435052128, -6.250000000000110134, -117.4419872981078328 ) ) ;
#1853=CARTESIAN_POINT ( 'NONE',  ( -6.000000000000007105, -1.607695154586655129, -110.2693375672973986 ) ) ;
#1861=EDGE_CURVE ( 'NONE', #21664, #269, #5048, .T. ) ;
#1862=CARTESIAN_POINT ( 'NONE',  ( 5.412658773652739619, 3.124999999999988898, -149.8169872981078186 ) ) ;
#1863=ORIENTED_EDGE ( 'NONE', *, *, #20873, .T. ) ;
#1869=CARTESIAN_POINT ( 'NONE',  ( -3.608439182435115633, 6.249999999999965361, -67.80801270189226670 ) ) ;
#1871=CARTESIAN_POINT ( 'NONE',  ( 3.464101615137852974, 5.999999999999884537, -177.4136751345947971 ) ) ;
#1872=CYLINDRICAL_SURFACE ( 'NONE', #16767, 6.000000000000000888 ) ;
#1873=CARTESIAN_POINT ( 'NONE',  ( 3.464101615137757051, -5.999999999999979572, -155.4136751345947687 ) ) ;
#1877=CARTESIAN_POINT ( 'NONE',  ( 4.763139720814407951, 2.750000000000002665, -126.2500000000000284 ) ) ;
#1880=ORIENTED_EDGE ( 'NONE', *, *, #14063, .T. ) ;
#1881=CARTESIAN_POINT ( 'NONE',  ( 6.350852961086080661, -9.614813431917819062E-14, -58.87500000000004974 ) ) ;
#1882=CARTESIAN_POINT ( 'NONE',  ( 3.464101615137757051, -5.999999999999979572, -153.9136751345947971 ) ) ;
#1883=CARTESIAN_POINT ( 'NONE',  ( 6.000000000000000888, 1.743066579297358182E-13, -70.58632486540523132 ) ) ;
#1884=CARTESIAN_POINT ( 'NONE',  ( 6.000000000000014211, -1.607695154586730180, -162.7306624327026725 ) ) ;
#1885=EDGE_LOOP ( 'NONE', ( #8262, #17030, #26038, #26441 ) ) ;
#1894=CARTESIAN_POINT ( 'NONE',  ( 6.350852961086080661, -9.614813431917819062E-14, -139.8750000000000568 ) ) ;
#1895=EDGE_CURVE ( 'NONE', #29849, #22223, #25723, .T. ) ;
#1899=CARTESIAN_POINT ( 'NONE',  ( 0.000000000000000000, 5.499999999999991118, -69.00000000000000000 ) ) ;
#1900=CARTESIAN_POINT ( 'NONE',  ( -5.196152422706573404, -3.000000000000002665, -164.7886751345948255 ) ) ;
#1901=CARTESIAN_POINT ( 'NONE',  ( 7.216878364870455975, -6.409875621278545621E-14, -90.80801270189223828 ) ) ;
#1904=CARTESIAN_POINT ( 'NONE',  ( -3.464101615137725076, 5.999999999999979572, -106.6636751345948397 ) ) ;
#1906=CARTESIAN_POINT ( 'NONE',  ( 0.000000000000000000, 0.000000000000000000, 0.000000000000000000 ) ) ;
#1909=CARTESIAN_POINT ( 'NONE',  ( 3.175426480543072749, -5.500000000000105693, -144.6250000000000000 ) ) ;
#1911=CARTESIAN_POINT ( 'NONE',  ( -6.350852961085760029, -1.281975124255709124E-13, -142.1250000000000000 ) ) ;
#1912=CARTESIAN_POINT ( 'NONE',  ( 5.412658773652739619, 3.124999999999988898, -159.6830127018922099 ) ) ;
#1913=DIRECTION ( 'NONE',  ( 1.000000000000000000, -5.551115123125773458E-17, -1.260129944081490338E-35 ) ) ;
#1914=CYLINDRICAL_SURFACE ( 'NONE', #18404, 6.000000000000000888 ) ;
#1915=CARTESIAN_POINT ( 'NONE',  ( 4.763139720814407951, -2.749999999999988454, -77.00000000000001421 ) ) ;
#1917=CARTESIAN_POINT ( 'NONE',  ( -3.175426480542816510, 5.499999999999865885, -73.37500000000000000 ) ) ;
#1918=CARTESIAN_POINT ( 'NONE',  ( 0.000000000000000000, 0.000000000000000000, 0.000000000000000000 ) ) ;
#1919=DIRECTION ( 'NONE',  ( -7.147005652999508048E-36, 5.642372883946980038E-36, 1.000000000000000000 ) ) ;
#1920=DIRECTION ( 'NONE',  ( -7.147005652999508048E-36, 5.642372883946980038E-36, 1.000000000000000000 ) ) ;
#1921=EDGE_CURVE ( 'NONE', #12335, #28542, #1586, .T. ) ;
#1925=EDGE_CURVE ( 'NONE', #28690, #12627, #5379, .T. ) ;
#1926=CARTESIAN_POINT ( 'NONE',  ( 5.196152422706629359, 3.000000000000002665, -55.46132486540522422 ) ) ;
#1932=CARTESIAN_POINT ( 'NONE',  ( -3.464101615137757051, -5.999999999999979572, -157.1636751345947971 ) ) ;
#1933=CARTESIAN_POINT ( 'NONE',  ( -5.999999999999963585, 0.000000000000000000, -179.3363248654052313 ) ) ;
#1939=CARTESIAN_POINT ( 'NONE',  ( -4.763139720814407951, 2.749999999999946709, -95.75000000000000000 ) ) ;
#1941=CARTESIAN_POINT ( 'NONE',  ( 7.216878364870455975, -6.409875621278545621E-14, -105.8080127018922525 ) ) ;
#1944=CARTESIAN_POINT ( 'NONE',  ( -2.775557561562891351E-14, -5.500000000000115463, -162.7500000000000000 ) ) ;
#1945=CARTESIAN_POINT ( 'NONE',  ( 1.581364418632522639, -10.89278420593270447, -30.80148057605385503 ) ) ;
#1946=AXIS2_PLACEMENT_3D ( 'NONE', #13470, #19888, #10701 ) ;
#1948=CYLINDRICAL_SURFACE ( 'NONE', #24486, 6.000000000000000888 ) ;
#1949=CYLINDRICAL_SURFACE ( 'NONE', #13935, 6.000000000000000888 ) ;
#1951=CARTESIAN_POINT ( 'NONE',  ( -2.775557561562891351E-14, -5.500000000000115463, -174.7500000000000284 ) ) ;
#1953=CARTESIAN_POINT ( 'NONE',  ( 4.763139720814407951, 2.750000000000002665, -159.2500000000000000 ) ) ;
#1956=CARTESIAN_POINT ( 'NONE',  ( -4.763139720814407951, 2.749999999999946709, -112.2500000000000142 ) ) ;
#1957=CYLINDRICAL_SURFACE ( 'NONE', #10992, 6.000000000000000888 ) ;
#1959=CARTESIAN_POINT ( 'NONE',  ( 3.175426480543072749, 5.499999999999865885, -96.12500000000004263 ) ) ;
#1962=ORIENTED_EDGE ( 'NONE', *, *, #10188, .T. ) ;
#1965=EDGE_CURVE ( 'NONE', #20877, #1086, #237, .T. ) ;
#1968=ORIENTED_EDGE ( 'NONE', *, *, #5524, .F. ) ;
#1970=CARTESIAN_POINT ( 'NONE',  ( 3.608439182435180470, -6.249999999999997335, -90.19198729810784698 ) ) ;
#1976=CARTESIAN_POINT ( 'NONE',  ( 6.350852961086080661, -9.614813431917819062E-14, -120.3750000000000142 ) ) ;
#1978=CARTESIAN_POINT ( 'NONE',  ( -5.412658773652684552, -3.125000000000099920, -131.9330127018922383 ) ) ;
#1981=CARTESIAN_POINT ( 'NONE',  ( 5.412658773652712085, -3.125000000000086153, -166.5669872981078186 ) ) ;
#1982=CARTESIAN_POINT ( 'NONE',  ( -5.412658773652739619, 3.124999999999975131, -177.8169872981077901 ) ) ;
#1983=CARTESIAN_POINT ( 'NONE',  ( 5.196152422706629359, 3.000000000000002665, -147.5386751345948539 ) ) ;
#1984=VERTEX_POINT ( 'NONE', #1540 ) ;
#1990=CARTESIAN_POINT ( 'NONE',  ( 7.216878364870455975, -6.409875621278545621E-14, -74.94198729810783277 ) ) ;
#1991=CARTESIAN_POINT ( 'NONE',  ( 5.412658773652712085, -3.125000000000086153, -61.56698729810783277 ) ) ;
#1992=CARTESIAN_POINT ( 'NONE',  ( 5.999999999999949374, 1.607695154586804565, -111.0193375672974270 ) ) ;
#1993=CARTESIAN_POINT ( 'NONE',  ( 3.175426480543072749, -5.500000000000105693, -50.12500000000001421 ) ) ;
#1994=CARTESIAN_POINT ( 'NONE',  ( 5.196152422706629359, 3.000000000000002665, -103.4613248654052171 ) ) ;
#1998=CARTESIAN_POINT ( 'NONE',  ( 3.175426480543072749, 5.499999999999865885, -124.6250000000000426 ) ) ;
#1999=CARTESIAN_POINT ( 'NONE',  ( -3.175426480542816510, 5.499999999999865885, -155.8750000000000000 ) ) ;
#2004=EDGE_CURVE ( 'NONE', #15491, #16271, #6300, .T. ) ;
#2007=VECTOR ( 'NONE', #20605, 1000.000000000000000 ) ;
#2010=CARTESIAN_POINT ( 'NONE',  ( 5.196152422706629359, -2.999999999999988898, -114.7886751345948397 ) ) ;
#2012=CARTESIAN_POINT ( 'NONE',  ( -5.412658773652684552, -3.125000000000099920, -119.0669872981078328 ) ) ;
#2013=CARTESIAN_POINT ( 'NONE',  ( 0.000000000000000000, -5.999999999999991118, -176.5386751345948824 ) ) ;
#2014=ADVANCED_FACE ( 'NONE', ( #5994 ), #15569, .T. ) ;
#2016=EDGE_LOOP ( 'NONE', ( #10257, #16667, #23258, #28613 ) ) ;
#2017=ORIENTED_EDGE ( 'NONE', *, *, #19492, .F. ) ;
#2018=CYLINDRICAL_SURFACE ( 'NONE', #13549, 6.000000000000000888 ) ;
#2022=CARTESIAN_POINT ( 'NONE',  ( 5.412658773652712085, -3.125000000000086153, -150.0669872981078470 ) ) ;
#2028=CARTESIAN_POINT ( 'NONE',  ( -5.196152422706573404, -3.000000000000002665, -137.7886751345947971 ) ) ;
#2029=CARTESIAN_POINT ( 'NONE',  ( 5.412658773652712085, -3.125000000000086153, -71.43301270189222407 ) ) ;
#2033=CARTESIAN_POINT ( 'NONE',  ( -3.464101615137757051, -5.999999999999979572, -161.0863248654052313 ) ) ;
#2034=CARTESIAN_POINT ( 'NONE',  ( 5.196152422706629359, -2.999999999999988898, -146.2886751345948824 ) ) ;
#2036=CARTESIAN_POINT ( 'NONE',  ( 6.000000000000000888, -3.330669073875464691E-16, -7.560779664488942560E-35 ) ) ;
#2038=CARTESIAN_POINT ( 'NONE',  ( 6.000000000000000888, -3.330669073875464691E-16, -7.560779664488942560E-35 ) ) ;
#2039=( BOUNDED_CURVE ( )  B_SPLINE_CURVE ( 2, ( #2859, #12280, #17173, #23772, #5304, #24059, #4862, #5450, #14858 ),
 .UNSPECIFIED., .F., .T. ) 
 B_SPLINE_CURVE_WITH_KNOTS ( ( 3, 2, 2, 2, 3 ),
 ( 0.4083333333333333259, 0.4092592592592592671, 0.4111111111111110938, 0.4129629629629629761, 0.4138888888888888618 ),
 .UNSPECIFIED. ) 
 CURVE ( )  GEOMETRIC_REPRESENTATION_ITEM ( )  RATIONAL_B_SPLINE_CURVE ( ( 0.9330127018922194093, 0.9330127018922194093, 1.000000000000000000, 0.8660254037844388186, 1.000000000000000000, 0.8660254037844388186, 1.000000000000000000, 0.9330127018922214077, 0.9330127018922194093 ) ) 
 REPRESENTATION_ITEM ( '' )  );
#2040=CARTESIAN_POINT ( 'NONE',  ( 6.350852961086080661, -9.614813431917819062E-14, -120.3750000000000426 ) ) ;
#2042=CARTESIAN_POINT ( 'NONE',  ( 2.775557561562891351E-14, 6.250000000000033751, -142.9330127018922383 ) ) ;
#2047=CARTESIAN_POINT ( 'NONE',  ( 3.175426480543072749, 5.499999999999865885, -58.62499999999999289 ) ) ;
#2048=DIRECTION ( 'NONE',  ( -7.147005652999508048E-36, 5.642372883946980038E-36, 1.000000000000000000 ) ) ;
#2050=EDGE_CURVE ( 'NONE', #30268, #19941, #19982, .T. ) ;
#2052=ORIENTED_EDGE ( 'NONE', *, *, #20488, .F. ) ;
#2061=VERTEX_POINT ( 'NONE', #13408 ) ;
#2063=CARTESIAN_POINT ( 'NONE',  ( -6.350852961085760029, -1.281975124255709124E-13, -136.1250000000000568 ) ) ;
#2064=ORIENTED_EDGE ( 'NONE', *, *, #12820, .T. ) ;
#2067=CARTESIAN_POINT ( 'NONE',  ( -3.175426480542816510, -5.500000000000057732, -63.87500000000001421 ) ) ;
#2075=CARTESIAN_POINT ( 'NONE',  ( 3.175426480543072749, 5.499999999999865885, -147.1250000000000284 ) ) ;
#2077=CARTESIAN_POINT ( 'NONE',  ( -7.216878364870328078, 0.000000000000000000, -157.5580127018922383 ) ) ;
#2078=CARTESIAN_POINT ( 'NONE',  ( -4.763139720814407951, 2.749999999999946709, -76.25000000000004263 ) ) ;
#2080=CARTESIAN_POINT ( 'NONE',  ( 3.175426480543072749, 5.499999999999865885, -76.62500000000001421 ) ) ;
#2082=CARTESIAN_POINT ( 'NONE',  ( -5.999999999999963585, -1.487416814333745711E-14, -154.4136751345947971 ) ) ;
#2084=CARTESIAN_POINT ( 'NONE',  ( -5.999999999999963585, -1.487416814333745711E-14, -88.41367513459482552 ) ) ;
#2085=DIRECTION ( 'NONE',  ( -7.147005652999508048E-36, 5.642372883946980038E-36, 1.000000000000000000 ) ) ;
#2088=CARTESIAN_POINT ( 'NONE',  ( 3.464101615137852974, 5.999999999999884537, -55.33632486540524553 ) ) ;
#2090=CARTESIAN_POINT ( 'NONE',  ( 6.000000000000000888, 1.743066579297358182E-13, -86.16367513459481131 ) ) ;
#2091=ORIENTED_EDGE ( 'NONE', *, *, #27334, .F. ) ;
#2095=DIRECTION ( 'NONE',  ( 1.000000000000000000, -5.551115123125773458E-17, -1.260129944081490338E-35 ) ) ;
#2096=VERTEX_POINT ( 'NONE', #1223 ) ;
#2097=ORIENTED_EDGE ( 'NONE', *, *, #10762, .T. ) ;
#2098=VERTEX_POINT ( 'NONE', #29334 ) ;
#2099=CARTESIAN_POINT ( 'NONE',  ( -3.175426480542816510, 5.499999999999865885, -89.87500000000001421 ) ) ;
#2100=CARTESIAN_POINT ( 'NONE',  ( 5.412658773652739619, 3.124999999999988898, -107.1830127018922383 ) ) ;
#2101=CARTESIAN_POINT ( 'NONE',  ( -6.000000000000000888, 1.067854986875958443E-15, 7.560779664488942560E-35 ) ) ;
#2102=CARTESIAN_POINT ( 'NONE',  ( -5.999999999999919176, 1.607695154586804565, -51.90331216351300725 ) ) ;
#2104=CARTESIAN_POINT ( 'NONE',  ( 3.175426480543072749, -5.500000000000105693, -165.6250000000000000 ) ) ;
#2105=CARTESIAN_POINT ( 'NONE',  ( 5.380679364423385458, -9.595766763449143255, -27.68326114948592931 ) ) ;
#2106=ORIENTED_EDGE ( 'NONE', *, *, #26530, .F. ) ;
#2108=DIRECTION ( 'NONE',  ( -7.147005652999508048E-36, 5.642372883946980038E-36, 1.000000000000000000 ) ) ;
#2110=CARTESIAN_POINT ( 'NONE',  ( 3.175426480543072749, -5.500000000000105693, -174.6250000000000284 ) ) ;
#2112=CARTESIAN_POINT ( 'NONE',  ( 3.175426480543072749, -5.500000000000105693, -162.6250000000000284 ) ) ;
#2114=CARTESIAN_POINT ( 'NONE',  ( 3.175426480543072749, 5.499999999999865885, -100.6250000000000000 ) ) ;
#2115=DIRECTION ( 'NONE',  ( -7.147005652999508048E-36, 5.642372883946980038E-36, 1.000000000000000000 ) ) ;
#2117=CARTESIAN_POINT ( 'NONE',  ( -3.175426480542816510, -5.500000000000057732, -99.87500000000000000 ) ) ;
#2124=DIRECTION ( 'NONE',  ( -7.147005652999508048E-36, 5.642372883946980038E-36, 1.000000000000000000 ) ) ;
#2128=CARTESIAN_POINT ( 'NONE',  ( -5.999999999999963585, 1.780251999655701777E-13, -111.8363248654052313 ) ) ;
#2137=CARTESIAN_POINT ( 'NONE',  ( 3.175426480543072749, 5.499999999999865885, -115.6250000000000142 ) ) ;
#2140=CARTESIAN_POINT ( 'NONE',  ( 3.608439182435180470, 6.249999999999982236, -134.0580127018922667 ) ) ;
#2141=ORIENTED_EDGE ( 'NONE', *, *, #8869, .T. ) ;
#2142=DIRECTION ( 'NONE',  ( -7.147005652999508048E-36, 5.642372883946980038E-36, 1.000000000000000000 ) ) ;
#2143=CARTESIAN_POINT ( 'NONE',  ( -3.608439182435115633, 6.249999999999965361, -165.9419872981078186 ) ) ;
#2144=CARTESIAN_POINT ( 'NONE',  ( -5.412658773652684552, -3.125000000000099920, -180.5669872981078186 ) ) ;
#2150=CARTESIAN_POINT ( 'NONE',  ( 5.511802646651305260, 2.338480655312030976, -180.0000000000001705 ) ) ;
#2153=CARTESIAN_POINT ( 'NONE',  ( -3.608439182435052128, -6.250000000000110134, -73.94198729810781856 ) ) ;
#2154=CARTESIAN_POINT ( 'NONE',  ( 3.608439182435180470, -6.249999999999997335, -60.19198729810783277 ) ) ;
#2155=CARTESIAN_POINT ( 'NONE',  ( -3.175426480542816510, 5.499999999999865885, -47.87500000000000000 ) ) ;
#2157=CARTESIAN_POINT ( 'NONE',  ( -3.464101615137757051, -5.999999999999979572, -123.5863248654051745 ) ) ;
#2158=CARTESIAN_POINT ( 'NONE',  ( 0.000000000000000000, -5.999999999999991118, -53.53867513459481842 ) ) ;
#2160=CARTESIAN_POINT ( 'NONE',  ( 4.763139720814407951, -2.749999999999988454, -119.0000000000000000 ) ) ;
#2164=VECTOR ( 'NONE', #17817, 1000.000000000000000 ) ;
#2166=CARTESIAN_POINT ( 'NONE',  ( -5.999999999999963585, 1.780251999655701777E-13, -95.33632486540520290 ) ) ;
#2169=CARTESIAN_POINT ( 'NONE',  ( -6.000000000000000888, 1.067854986875958443E-15, 7.560779664488942560E-35 ) ) ;
#2171=CARTESIAN_POINT ( 'NONE',  ( 7.216878364870455975, -6.409875621278545621E-14, -109.4419872981078043 ) ) ;
#2173=ORIENTED_EDGE ( 'NONE', *, *, #8544, .T. ) ;
#2174=CARTESIAN_POINT ( 'NONE',  ( -5.999999999999982236, -1.607695154586700426, -142.3466878364870354 ) ) ;
#2176=CARTESIAN_POINT ( 'NONE',  ( 3.608439182435180470, 6.249999999999982236, -136.1919872981078470 ) ) ;
#2183=CARTESIAN_POINT ( 'NONE',  ( -5.412658773652739619, 3.124999999999975131, -70.68301270189225249 ) ) ;
#2185=CARTESIAN_POINT ( 'NONE',  ( 5.196152422706629359, -2.999999999999988898, -124.7113248654052597 ) ) ;
#2186=CARTESIAN_POINT ( 'NONE',  ( 5.196152422706629359, -2.999999999999988898, -69.78867513459485394 ) ) ;
#2191=EDGE_CURVE ( 'NONE', #28056, #407, #21075, .T. ) ;
#2192=CARTESIAN_POINT ( 'NONE',  ( 6.350852961086080661, -9.614813431917819062E-14, -123.3750000000000000 ) ) ;
#2194=CARTESIAN_POINT ( 'NONE',  ( 5.412658773652712085, -3.125000000000086153, -144.9330127018922383 ) ) ;
#2196=CYLINDRICAL_SURFACE ( 'NONE', #4313, 6.000000000000000888 ) ;
#2198=CARTESIAN_POINT ( 'NONE',  ( 4.763139720814407951, -2.749999999999988454, -56.00000000000004974 ) ) ;
#2199=CARTESIAN_POINT ( 'NONE',  ( 3.464101615137852974, 5.999999999999884537, -124.3363248654051603 ) ) ;
#2200=CARTESIAN_POINT ( 'NONE',  ( 6.000000000000000888, 1.607695154586715303, -63.01933756729744829 ) ) ;
#2202=ORIENTED_EDGE ( 'NONE', *, *, #12275, .F. ) ;
#2205=AXIS2_PLACEMENT_3D ( 'NONE', #28868, #27023, #14927 ) ;
#2206=CARTESIAN_POINT ( 'NONE',  ( 5.412658773652739619, 3.124999999999988898, -103.3169872981078470 ) ) ;
#2211=CARTESIAN_POINT ( 'NONE',  ( -6.350852961085760029, -1.281975124255709124E-13, -134.6250000000000284 ) ) ;
#2214=VECTOR ( 'NONE', #405, 1000.000000000000000 ) ;
#2215=CARTESIAN_POINT ( 'NONE',  ( -4.763139720814407951, -2.750000000000016431, -62.50000000000000000 ) ) ;
#2226=( BOUNDED_CURVE ( )  B_SPLINE_CURVE ( 2, ( #19868, #5871, #8175, #28611, #3261, #17140, #17593, #7579, #15292 ),
 .UNSPECIFIED., .F., .T. ) 
 B_SPLINE_CURVE_WITH_KNOTS ( ( 3, 2, 2, 2, 3 ),
 ( 0.3138888888888888840, 0.3148148148148147696, 0.3166666666666666519, 0.3185185185185185341, 0.3194444444444445308 ),
 .UNSPECIFIED. ) 
 CURVE ( )  GEOMETRIC_REPRESENTATION_ITEM ( )  RATIONAL_B_SPLINE_CURVE ( ( 0.9330127018922194093, 0.9330127018922194093, 1.000000000000000000, 0.8660254037844388186, 1.000000000000000000, 0.8660254037844388186, 1.000000000000000000, 0.9330127018922154125, 0.9330127018922194093 ) ) 
 REPRESENTATION_ITEM ( '' )  );
#2227=CARTESIAN_POINT ( 'NONE',  ( 3.175426480543072749, -5.500000000000105693, -152.1250000000000284 ) ) ;
#2229=CIRCLE ( 'NONE', #11578, 4.000000000000003553 ) ;
#2230=CARTESIAN_POINT ( 'NONE',  ( -3.175426480542816510, 5.499999999999865885, -134.8750000000000000 ) ) ;
#2231=CARTESIAN_POINT ( 'NONE',  ( -5.412658773652684552, -3.125000000000099920, -164.9330127018922667 ) ) ;
#2232=FACE_OUTER_BOUND ( 'NONE', #13224, .T. ) ;
#2233=CARTESIAN_POINT ( 'NONE',  ( 3.175426480543072749, -5.500000000000105693, -80.12500000000002842 ) ) ;
#2234=CARTESIAN_POINT ( 'NONE',  ( -3.999999999999997335, 7.119033245839719993E-16, -180.0000000000000568 ) ) ;
#2235=CARTESIAN_POINT ( 'NONE',  ( 6.350852961086080661, -9.614813431917819062E-14, -76.87500000000000000 ) ) ;
#2236=CARTESIAN_POINT ( 'NONE',  ( -3.464101615137757051, -5.999999999999979572, -156.5863248654052313 ) ) ;
#2238=CARTESIAN_POINT ( 'NONE',  ( -3.464101615137757051, -5.999999999999979572, -88.16367513459482552 ) ) ;
#2251=VERTEX_POINT ( 'NONE', #8774 ) ;
#2255=CARTESIAN_POINT ( 'NONE',  ( 4.763139720814407951, -2.749999999999988454, -87.50000000000002842 ) ) ;
#2257=CARTESIAN_POINT ( 'NONE',  ( 3.608439182435180470, -6.249999999999997335, -109.0580127018921957 ) ) ;
#2258=ORIENTED_EDGE ( 'NONE', *, *, #21716, .F. ) ;
#2261=CARTESIAN_POINT ( 'NONE',  ( -6.000000000000007105, -1.607695154586655129, -63.76933756729744118 ) ) ;
#2263=CARTESIAN_POINT ( 'NONE',  ( 5.196152422706629359, 3.000000000000002665, -93.53867513459479710 ) ) ;
#2264=CARTESIAN_POINT ( 'NONE',  ( -4.763139720814407951, -2.750000000000016431, -169.0000000000000284 ) ) ;
#2265=CARTESIAN_POINT ( 'NONE',  ( 3.175426480543072749, -5.500000000000105693, -156.6250000000000000 ) ) ;
#2269=CARTESIAN_POINT ( 'NONE',  ( -3.175426480542816066, -5.500000000000057732, -104.3750000000000142 ) ) ;
#2270=CARTESIAN_POINT ( 'NONE',  ( -5.196152422706601826, 2.999999999999975131, -87.03867513459483973 ) ) ;
#2271=CARTESIAN_POINT ( 'NONE',  ( -2.775557561562891351E-14, -5.500000000000115463, -101.2500000000000000 ) ) ;
#2277=CARTESIAN_POINT ( 'NONE',  ( -3.464101615137757051, -5.999999999999979572, -161.6636751345947687 ) ) ;
#2283=CARTESIAN_POINT ( 'NONE',  ( -5.999999999999919176, 1.607695154586804565, -111.9033121635129930 ) ) ;
#2286=CARTESIAN_POINT ( 'NONE',  ( 6.000000000000000888, -3.330669073875464691E-16, -7.560779664488942560E-35 ) ) ;
#2290=CARTESIAN_POINT ( 'NONE',  ( 0.000000000000000000, 5.499999999999991118, -115.5000000000000426 ) ) ;
#2293=CARTESIAN_POINT ( 'NONE',  ( -3.608439182435115633, 6.249999999999965361, -130.8080127018922383 ) ) ;
#2296=CARTESIAN_POINT ( 'NONE',  ( 3.608439182435180470, -6.249999999999997335, -172.6919872981078470 ) ) ;
#2302=CARTESIAN_POINT ( 'NONE',  ( 2.846577545700131662, 4.964493094578525501, -180.0000000000000000 ) ) ;
#2303=DIRECTION ( 'NONE',  ( 1.000000000000000000, -5.551115123125774690E-17, 0.000000000000000000 ) ) ;
#2306=CARTESIAN_POINT ( 'NONE',  ( 5.412658773652739619, 3.124999999999988898, -176.1830127018922383 ) ) ;
#2308=CARTESIAN_POINT ( 'NONE',  ( -6.000000000000007105, -1.607695154586655129, -48.76933756729741987 ) ) ;
#2309=LINE ( 'NONE', #21350, #4504 ) ;
#2310=CARTESIAN_POINT ( 'NONE',  ( 4.763139720814407951, 2.750000000000002665, -124.7500000000000284 ) ) ;
#2311=CARTESIAN_POINT ( 'NONE',  ( 6.000000000000000888, -1.859271017917181981E-14, -146.1636751345948255 ) ) ;
#2315=LINE ( 'NONE', #28389, #563 ) ;
#2316=CARTESIAN_POINT ( 'NONE',  ( 5.196152422706629359, 3.000000000000002665, -105.5386751345948113 ) ) ;
#2317=( BOUNDED_CURVE ( )  B_SPLINE_CURVE ( 2, ( #20901, #19496, #28826, #7787, #585, #12753, #3178, #9820, #742 ),
 .UNSPECIFIED., .F., .T. ) 
 B_SPLINE_CURVE_WITH_KNOTS ( ( 3, 2, 2, 2, 3 ),
 ( 0.4916666666666665853, 0.4925925925925925819, 0.4944444444444444642, 0.4962962962962963465, 0.4972222222222222321 ),
 .UNSPECIFIED. ) 
 CURVE ( )  GEOMETRIC_REPRESENTATION_ITEM ( )  RATIONAL_B_SPLINE_CURVE ( ( 0.9330127018922194093, 0.9330127018922154125, 1.000000000000000000, 0.8660254037844388186, 1.000000000000000000, 0.8660254037844388186, 1.000000000000000000, 0.9330127018922194093, 0.9330127018922194093 ) ) 
 REPRESENTATION_ITEM ( '' )  );
#2318=VERTEX_POINT ( 'NONE', #2166 ) ;
#2321=CARTESIAN_POINT ( 'NONE',  ( 5.196152422706629359, 3.000000000000002665, -122.0386751345948824 ) ) ;
#2322=EDGE_CURVE ( 'NONE', #91, #5714, #22225, .T. ) ;
#2323=CARTESIAN_POINT ( 'NONE',  ( 2.775557561562891351E-14, -6.250000000000061284, -108.3169872981077901 ) ) ;
#2325=ORIENTED_EDGE ( 'NONE', *, *, #17767, .F. ) ;
#2326=CYLINDRICAL_SURFACE ( 'NONE', #16772, 6.000000000000000888 ) ;
#2331=EDGE_CURVE ( 'NONE', #3077, #26117, #7501, .T. ) ;
#2333=CARTESIAN_POINT ( 'NONE',  ( 7.216878364870455975, -6.409875621278545621E-14, -136.4419872981077901 ) ) ;
#2334=CARTESIAN_POINT ( 'NONE',  ( -5.999999999999963585, 8.134310703387671600E-14, -146.9136751345948255 ) ) ;
#2337=CARTESIAN_POINT ( 'NONE',  ( 5.196152422706629359, -2.999999999999988898, -171.2113248654052313 ) ) ;
#2338=CARTESIAN_POINT ( 'NONE',  ( 5.412658773652739619, 3.124999999999988898, -57.68301270189224539 ) ) ;
#2341=CARTESIAN_POINT ( 'NONE',  ( 3.464101615137757051, -5.999999999999979572, -124.8363248654051745 ) ) ;
#2345=CARTESIAN_POINT ( 'NONE',  ( 0.000000000000000000, 5.999999999999977796, -115.2113248654052029 ) ) ;
#2348=CARTESIAN_POINT ( 'NONE',  ( 6.000000000000000888, 1.743066579297358182E-13, -75.08632486540521711 ) ) ;
#2351=CARTESIAN_POINT ( 'NONE',  ( 4.763139720814407951, 2.750000000000002665, -55.75000000000002132 ) ) ;
#2353=CARTESIAN_POINT ( 'NONE',  ( 5.196152422706629359, 3.000000000000002665, -121.4613248654052313 ) ) ;
#2357=EDGE_CURVE ( 'NONE', #28820, #11352, #22041, .T. ) ;
#2358=CARTESIAN_POINT ( 'NONE',  ( -5.412658773652684552, -3.125000000000099920, -104.0669872981078186 ) ) ;
#2362=EDGE_LOOP ( 'NONE', ( #28718, #15523, #16232, #7841 ) ) ;
#2363=( BOUNDED_CURVE ( )  B_SPLINE_CURVE ( 2, ( #10930, #20279, #29469, #24718, #15225, #15066, #3351, #19809, #15549 ),
 .UNSPECIFIED., .F., .F. ) 
 B_SPLINE_CURVE_WITH_KNOTS ( ( 3, 2, 2, 2, 3 ),
 ( 0.008333333333333414750, 0.009259259259259300379, 0.01111111111111107164, 0.01296296296296295392, 0.01388888888888883955 ),
 .UNSPECIFIED. ) 
 CURVE ( )  GEOMETRIC_REPRESENTATION_ITEM ( )  RATIONAL_B_SPLINE_CURVE ( ( 0.9330127018922194093, 0.9330127018922234061, 1.000000000000000000, 0.8660254037844388186, 1.000000000000000000, 0.8660254037844388186, 1.000000000000000000, 0.9330127018922234061, 0.9330127018922194093 ) ) 
 REPRESENTATION_ITEM ( '' )  );
#2365=CARTESIAN_POINT ( 'NONE',  ( -4.763139720814407951, -2.750000000000016431, -139.0000000000000000 ) ) ;
#2369=CARTESIAN_POINT ( 'NONE',  ( 4.763139720814407951, 2.750000000000002665, -67.75000000000002842 ) ) ;
#2371=CARTESIAN_POINT ( 'NONE',  ( -3.608439182435052128, -6.250000000000110134, -80.80801270189226670 ) ) ;
#2374=DIRECTION ( 'NONE',  ( 1.000000000000000000, -5.551115123125773458E-17, -1.260129944081490338E-35 ) ) ;
#2376=CARTESIAN_POINT ( 'NONE',  ( -3.175426480542816066, -5.500000000000057732, -146.3750000000000284 ) ) ;
#2378=CARTESIAN_POINT ( 'NONE',  ( 0.000000000000000000, 5.499999999999991118, -133.5000000000000000 ) ) ;
#2379=CARTESIAN_POINT ( 'NONE',  ( -3.608439182435115633, 6.249999999999965361, -162.3080127018922667 ) ) ;
#2380=CARTESIAN_POINT ( 'NONE',  ( 3.464101615137757051, -5.999999999999979572, -148.8363248654051176 ) ) ;
#2381=CARTESIAN_POINT ( 'NONE',  ( 3.175426480543072749, 5.499999999999865885, -75.12500000000000000 ) ) ;
#2382=CARTESIAN_POINT ( 'NONE',  ( -6.350852961085760029, -1.281975124255709124E-13, -62.62500000000001421 ) ) ;
#2385=EDGE_CURVE ( 'NONE', #22196, #4423, #17948, .T. ) ;
#2388=CARTESIAN_POINT ( 'NONE',  ( -3.464101615137757051, -5.999999999999979572, -98.08632486540524553 ) ) ;
#2389=EDGE_CURVE ( 'NONE', #15666, #14341, #19074, .T. ) ;
#2393=DIRECTION ( 'NONE',  ( -7.147005652999508048E-36, 5.642372883946980038E-36, 1.000000000000000000 ) ) ;
#2395=ORIENTED_EDGE ( 'NONE', *, *, #10585, .T. ) ;
#2396=( BOUNDED_CURVE ( )  B_SPLINE_CURVE ( 2, ( #17510, #29751, #3936, #6257, #20394, #8728, #27433, #13223, #6402 ),
 .UNSPECIFIED., .F., .T. ) 
 B_SPLINE_CURVE_WITH_KNOTS ( ( 3, 2, 2, 2, 3 ),
 ( 0.7361111111111110494, 0.7370370370370370461, 0.7388888888888889284, 0.7407407407407406996, 0.7416666666666666963 ),
 .UNSPECIFIED. ) 
 CURVE ( )  GEOMETRIC_REPRESENTATION_ITEM ( )  RATIONAL_B_SPLINE_CURVE ( ( 0.9330127018922194093, 0.9330127018922154125, 1.000000000000000000, 0.8660254037844388186, 1.000000000000000000, 0.8660254037844388186, 1.000000000000000000, 0.9330127018922154125, 0.9330127018922194093 ) ) 
 REPRESENTATION_ITEM ( '' )  );
#2399=VERTEX_POINT ( 'NONE', #14897 ) ;
#2400=CARTESIAN_POINT ( 'NONE',  ( -3.175426480542816510, 5.499999999999865885, -88.37500000000000000 ) ) ;
#2401=CARTESIAN_POINT ( 'NONE',  ( 7.216878364870455975, -6.409875621278545621E-14, -107.3080127018922525 ) ) ;
#2402=( BOUNDED_CURVE ( )  B_SPLINE_CURVE ( 2, ( #16114, #4073, #22834, #1775, #11179, #29879, #8858, #13806, #18241 ),
 .UNSPECIFIED., .F., .T. ) 
 B_SPLINE_CURVE_WITH_KNOTS ( ( 3, 2, 2, 2, 3 ),
 ( 0.8194444444444444198, 0.8203703703703704164, 0.8222222222222221877, 0.8240740740740740700, 0.8249999999999999556 ),
 .UNSPECIFIED. ) 
 CURVE ( )  GEOMETRIC_REPRESENTATION_ITEM ( )  RATIONAL_B_SPLINE_CURVE ( ( 0.9330127018922194093, 0.9330127018922154125, 1.000000000000000000, 0.8660254037844388186, 1.000000000000000000, 0.8660254037844388186, 1.000000000000000000, 0.9330127018922234061, 0.9330127018922194093 ) ) 
 REPRESENTATION_ITEM ( '' )  );
#2403=ORIENTED_EDGE ( 'NONE', *, *, #30161, .F. ) ;
#2406=CARTESIAN_POINT ( 'NONE',  ( -6.350852961085760029, -1.281975124255709124E-13, -163.1249999999999716 ) ) ;
#2407=CARTESIAN_POINT ( 'NONE',  ( -5.412658773652739619, 3.124999999999975131, -48.18301270189223828 ) ) ;
#2409=SURFACE_SIDE_STYLE ('',( #14424 ) ) ;
#2410=CARTESIAN_POINT ( 'NONE',  ( -3.175426480542816066, -5.500000000000057732, -170.3750000000000853 ) ) ;
#2412=CARTESIAN_POINT ( 'NONE',  ( 4.763139720814407951, 2.750000000000002665, -151.7500000000000568 ) ) ;
#2414=CARTESIAN_POINT ( 'NONE',  ( 0.000000000000000000, 5.499999999999991118, -103.5000000000000426 ) ) ;
#2417=CARTESIAN_POINT ( 'NONE',  ( 4.763139720814407951, 2.750000000000002665, -87.25000000000005684 ) ) ;
#2424=DIRECTION ( 'NONE',  ( -7.147005652999508048E-36, 5.642372883946980038E-36, 1.000000000000000000 ) ) ;
#2428=EDGE_CURVE ( 'NONE', #1801, #26144, #4898, .T. ) ;
#2431=CARTESIAN_POINT ( 'NONE',  ( 0.000000000000000000, 0.000000000000000000, 0.000000000000000000 ) ) ;
#2433=ORIENTED_EDGE ( 'NONE', *, *, #19492, .T. ) ;
#2434=LINE ( 'NONE', #2286, #3664 ) ;
#2435=ORIENTED_EDGE ( 'NONE', *, *, #25003, .T. ) ;
#2437=ORIENTED_EDGE ( 'NONE', *, *, #24781, .F. ) ;
#2438=CARTESIAN_POINT ( 'NONE',  ( 3.175426480543072749, -5.500000000000105693, -110.1249999999999858 ) ) ;
#2439=AXIS2_PLACEMENT_3D ( 'NONE', #3544, #5700, #21859 ) ;
#2441=CARTESIAN_POINT ( 'NONE',  ( -7.216878364870328078, 0.000000000000000000, -129.0580127018922383 ) ) ;
#2442=ORIENTED_EDGE ( 'NONE', *, *, #8844, .T. ) ;
#2445=CARTESIAN_POINT ( 'NONE',  ( 7.216878364870455975, -6.409875621278545621E-14, -167.9419872981078186 ) ) ;
#2449=CARTESIAN_POINT ( 'NONE',  ( 3.106370373199874635, 4.832402510089593761, -180.0000000000001421 ) ) ;
#2451=CARTESIAN_POINT ( 'NONE',  ( 6.350852961086080661, -9.614813431917819062E-14, -178.8750000000000284 ) ) ;
#2453=CARTESIAN_POINT ( 'NONE',  ( -3.608439182435115633, 6.249999999999965361, -177.3080127018922383 ) ) ;
#2455=CARTESIAN_POINT ( 'NONE',  ( -4.763139720814407951, -2.750000000000016431, -111.9999999999999858 ) ) ;
#2457=CARTESIAN_POINT ( 'NONE',  ( 6.000000000000052403, 1.607695154586625819, -154.5193375672974128 ) ) ;
#2458=VERTEX_POINT ( 'NONE', #21359 ) ;
#2463=EDGE_CURVE ( 'NONE', #15491, #21222, #25343, .T. ) ;
#2467=CARTESIAN_POINT ( 'NONE',  ( -5.196152422706573404, -3.000000000000002665, -176.7886751345948539 ) ) ;
#2468=CARTESIAN_POINT ( 'NONE',  ( -5.196152422706573404, -3.000000000000002665, -95.78867513459482552 ) ) ;
#2469=LINE ( 'NONE', #25959, #11347 ) ;
#2470=ORIENTED_EDGE ( 'NONE', *, *, #27046, .F. ) ;
#2471=ORIENTED_EDGE ( 'NONE', *, *, #25251, .T. ) ;
#2472=LINE ( 'NONE', #4467, #26239 ) ;
#2474=CARTESIAN_POINT ( 'NONE',  ( 2.775557561562891351E-14, 6.250000000000033751, -137.5669872981077901 ) ) ;
#2477=CARTESIAN_POINT ( 'NONE',  ( -5.196152422706573404, -3.000000000000002665, -171.7113248654052029 ) ) ;
#2480=CARTESIAN_POINT ( 'NONE',  ( -5.999999999999963585, 8.134310703387671600E-14, -125.3363248654052171 ) ) ;
#2482=CARTESIAN_POINT ( 'NONE',  ( 0.000000000000000000, -5.999999999999991118, -139.9613248654052313 ) ) ;
#2483=ADVANCED_FACE ( 'NONE', ( #14608 ), #23961, .T. ) ;
#2485=SURFACE_SIDE_STYLE ('',( #2629 ) ) ;
#2487=( BOUNDED_CURVE ( )  B_SPLINE_CURVE ( 2, ( #15246, #5831, #13114, #3837, #29493, #13265, #24578, #7839, #12957 ),
 .UNSPECIFIED., .F., .T. ) 
 B_SPLINE_CURVE_WITH_KNOTS ( ( 3, 2, 2, 2, 3 ),
 ( 0.3750000000000000000, 0.3759259259259258856, 0.3777777777777777679, 0.3796296296296296502, 0.3805555555555555358 ),
 .UNSPECIFIED. ) 
 CURVE ( )  GEOMETRIC_REPRESENTATION_ITEM ( )  RATIONAL_B_SPLINE_CURVE ( ( 0.9330127018922194093, 0.9330127018922194093, 1.000000000000000000, 0.8660254037844388186, 1.000000000000000000, 0.8660254037844388186, 1.000000000000000000, 0.9330127018922234061, 0.9330127018922194093 ) ) 
 REPRESENTATION_ITEM ( '' )  );
#2488=CARTESIAN_POINT ( 'NONE',  ( 3.464101615137852974, 5.999999999999884537, -112.9136751345948255 ) ) ;
#2489=ORIENTED_EDGE ( 'NONE', *, *, #4182, .T. ) ;
#2490=CARTESIAN_POINT ( 'NONE',  ( 0.000000000000000000, 5.499999999999991118, -52.49999999999999289 ) ) ;
#2491=CARTESIAN_POINT ( 'NONE',  ( -5.999999999999971578, 1.607695154586715303, -87.90331216351300725 ) ) ;
#2495=CARTESIAN_POINT ( 'NONE',  ( 2.775557561562891351E-14, 6.250000000000033751, -100.0669872981078186 ) ) ;
#2497=CARTESIAN_POINT ( 'NONE',  ( 6.000000000000000888, 1.743066579297358182E-13, -77.16367513459483973 ) ) ;
#2499=CARTESIAN_POINT ( 'NONE',  ( -3.175426480542816510, 5.499999999999865885, -139.3750000000000568 ) ) ;
#2502=CARTESIAN_POINT ( 'NONE',  ( 5.196152422706629359, 3.000000000000002665, -163.4613248654052029 ) ) ;
#2503=CARTESIAN_POINT ( 'NONE',  ( 4.763139720814407951, -2.749999999999988454, -69.50000000000000000 ) ) ;
#2505=CARTESIAN_POINT ( 'NONE',  ( -5.999999999999919176, 1.607695154586804565, -65.98066243270258724 ) ) ;
#2506=CARTESIAN_POINT ( 'NONE',  ( -7.216878364870328078, 0.000000000000000000, -84.05801270189220986 ) ) ;
#2510=CARTESIAN_POINT ( 'NONE',  ( 5.999999999999949374, -1.607695154586841868, -175.6533121635130215 ) ) ;
#2511=VECTOR ( 'NONE', #12672, 1000.000000000000114 ) ;
#2513=CARTESIAN_POINT ( 'NONE',  ( -3.175426480542816066, 5.499999999999865885, -149.8750000000000000 ) ) ;
#2515=VECTOR ( 'NONE', #21031, 1000.000000000000000 ) ;
#2516=CARTESIAN_POINT ( 'NONE',  ( -5.412658773652739619, 3.124999999999975131, -162.1830127018922951 ) ) ;
#2517=CARTESIAN_POINT ( 'NONE',  ( -5.999999999999962697, 3.323446944526963260E-14, -149.3363248654052313 ) ) ;
#2518=VECTOR ( 'NONE', #14237, 1000.000000000000000 ) ;
#2519=CARTESIAN_POINT ( 'NONE',  ( -3.175426480542816066, 5.499999999999865885, -82.37500000000002842 ) ) ;
#2520=CARTESIAN_POINT ( 'NONE',  ( 3.464101615137852974, 5.999999999999884537, -85.91367513459482552 ) ) ;
#2522=CARTESIAN_POINT ( 'NONE',  ( -2.775557561562891351E-14, -5.500000000000115463, -63.75000000000002842 ) ) ;
#2530=( BOUNDED_CURVE ( )  B_SPLINE_CURVE ( 2, ( #10038, #19415, #14235, #28146, #14088, #25860, #4806, #2505, #15109 ),
 .UNSPECIFIED., .F., .F. ) 
 B_SPLINE_CURVE_WITH_KNOTS ( ( 3, 2, 2, 2, 3 ),
 ( 0.8527777777777778567, 0.8537037037037037424, 0.8555555555555555136, 0.8574074074074073959, 0.8583333333333332815 ),
 .UNSPECIFIED. ) 
 CURVE ( )  GEOMETRIC_REPRESENTATION_ITEM ( )  RATIONAL_B_SPLINE_CURVE ( ( 0.9330127018922194093, 0.9330127018922234061, 1.000000000000000000, 0.8660254037844388186, 1.000000000000000000, 0.8660254037844388186, 1.000000000000000000, 0.9330127018922234061, 0.9330127018922194093 ) ) 
 REPRESENTATION_ITEM ( '' )  );
#2533=CARTESIAN_POINT ( 'NONE',  ( 6.000000000000000888, -3.330669073875464691E-16, -7.560779664488942560E-35 ) ) ;
#2534=VERTEX_POINT ( 'NONE', #18231 ) ;
#2536=CARTESIAN_POINT ( 'NONE',  ( 6.000000000000000888, -1.859271017917181981E-14, -141.0863248654052029 ) ) ;
#2537=B_SPLINE_CURVE_WITH_KNOTS ( 'NONE', 3,
 ( #11703, #25638, #284, #14312, #27770, #2302, #2449, #6590, #6747, #16463, #21200, #18302, #7052, #16318, #2150, #16013 ),
 .UNSPECIFIED., .F., .F.,
 ( 4, 2, 2, 2, 2, 2, 2, 4 ),
 ( 0.000000000000000000, 0.001747794382755240477, 0.002621691574132859522, 0.003495588765510479218, 0.004369485956888098481, 0.005243383148265719045, 0.006117280339643340475, 0.006991177531020960172 ),
 .UNSPECIFIED. ) ;
#2539=CARTESIAN_POINT ( 'NONE',  ( 6.350852961086080661, -9.614813431917819062E-14, -153.3750000000000000 ) ) ;
#2540=DIRECTION ( 'NONE',  ( -7.147005652999508048E-36, 5.642372883946980038E-36, 1.000000000000000000 ) ) ;
#2543=ORIENTED_EDGE ( 'NONE', *, *, #603, .T. ) ;
#2544=CARTESIAN_POINT ( 'NONE',  ( 4.763139720814407951, -2.749999999999988454, -89.00000000000002842 ) ) ;
#2545=CARTESIAN_POINT ( 'NONE',  ( 7.216878364870455975, -6.409875621278545621E-14, -101.3080127018922525 ) ) ;
#2547=EDGE_CURVE ( 'NONE', #226, #17900, #28486, .T. ) ;
#2549=CARTESIAN_POINT ( 'NONE',  ( -3.464101615137757051, -5.999999999999979572, -68.08632486540523132 ) ) ;
#2550=CARTESIAN_POINT ( 'NONE',  ( 4.763139720814407951, 2.750000000000002665, -171.2500000000000000 ) ) ;
#2551=CARTESIAN_POINT ( 'NONE',  ( 5.196152422706629359, -2.999999999999988898, -80.28867513459481131 ) ) ;
#2552=CARTESIAN_POINT ( 'NONE',  ( -6.350852961085760029, -1.281975124255709124E-13, -154.1250000000000568 ) ) ;
#2554=CARTESIAN_POINT ( 'NONE',  ( 4.763139720814407951, -2.749999999999988454, -99.50000000000002842 ) ) ;
#2556=CARTESIAN_POINT ( 'NONE',  ( 0.000000000000000000, 5.999999999999977796, -59.71132486540520290 ) ) ;
#2557=EDGE_CURVE ( 'NONE', #84, #21073, #12765, .T. ) ;
#2558=CARTESIAN_POINT ( 'NONE',  ( -4.763139720814407951, -2.750000000000016431, -155.5000000000000284 ) ) ;
#2559=CARTESIAN_POINT ( 'NONE',  ( -3.175426480542816510, 5.499999999999865885, -91.37500000000001421 ) ) ;
#2564=UNCERTAINTY_MEASURE_WITH_UNIT (LENGTH_MEASURE( 1.000000000000000082E-05 ), #28419, 'distance_accuracy_value', 'NONE');
#2566=CARTESIAN_POINT ( 'NONE',  ( 5.196152422706629359, -2.999999999999988898, -66.21132486540520290 ) ) ;
#2574=CARTESIAN_POINT ( 'NONE',  ( -3.464101615137757051, -5.999999999999979572, -141.5863248654052029 ) ) ;
#2576=ORIENTED_EDGE ( 'NONE', *, *, #30089, .T. ) ;
#2577=CARTESIAN_POINT ( 'NONE',  ( 4.763139720814407951, -2.749999999999988454, -117.5000000000000426 ) ) ;
#2579=CARTESIAN_POINT ( 'NONE',  ( 7.216878364870455975, -6.409875621278545621E-14, -120.8080127018921957 ) ) ;
#2581=CARTESIAN_POINT ( 'NONE',  ( 0.000000000000000000, 0.000000000000000000, 0.000000000000000000 ) ) ;
#2582=CARTESIAN_POINT ( 'NONE',  ( 3.608439182435180470, 6.249999999999982236, -169.1919872981078186 ) ) ;
#2586=ORIENTED_EDGE ( 'NONE', *, *, #28158, .F. ) ;
#2588=EDGE_CURVE ( 'NONE', #14973, #8441, #16177, .T. ) ;
#2589=DIRECTION ( 'NONE',  ( -7.147005652999508048E-36, 5.642372883946980038E-36, 1.000000000000000000 ) ) ;
#2590=LINE ( 'NONE', #28666, #30003 ) ;
#2591=CARTESIAN_POINT ( 'NONE',  ( -4.763139720814407951, 2.749999999999946709, -176.7500000000000284 ) ) ;
#2593=CARTESIAN_POINT ( 'NONE',  ( -7.216878364870328078, 0.000000000000000000, -174.0580127018922667 ) ) ;
#2597=CARTESIAN_POINT ( 'NONE',  ( -2.775557561562891351E-14, -5.500000000000115463, -113.2500000000000142 ) ) ;
#2598=CARTESIAN_POINT ( 'NONE',  ( 5.630955349231442142, 2.071796769705314123, -180.0000000000000568 ) ) ;
#2599=CARTESIAN_POINT ( 'NONE',  ( 6.000000000000000888, 1.607695154586715303, -101.0966878364870638 ) ) ;
#2600=VERTEX_POINT ( 'NONE', #889 ) ;
#2604=CARTESIAN_POINT ( 'NONE',  ( -6.000000000000023093, 1.607695154586625819, -131.4033121635129930 ) ) ;
#2606=ORIENTED_EDGE ( 'NONE', *, *, #11414, .F. ) ;
#2608=CARTESIAN_POINT ( 'NONE',  ( 6.000000000000000888, -3.330669073875464691E-16, -7.560779664488942560E-35 ) ) ;
#2609=CARTESIAN_POINT ( 'NONE',  ( 5.196152422706629359, 3.000000000000002665, -108.5386751345948113 ) ) ;
#2612=CARTESIAN_POINT ( 'NONE',  ( -5.999999999999963585, -1.487416814333745711E-14, -80.33632486540523132 ) ) ;
#2614=ORIENTED_EDGE ( 'NONE', *, *, #3229, .F. ) ;
#2616=( BOUNDED_SURFACE ( )  B_SPLINE_SURFACE ( 2, 3, ( 
 ( #15747, #13432, #6483, #25204 ),
 ( #4167, #13591, #8159, #26892 ),
 ( #15273, #24601, #3551, #10658 ) ),
 .UNSPECIFIED., .F., .F., .F. ) 
 B_SPLINE_SURFACE_WITH_KNOTS ( ( 3, 3 ),
 ( 4, 4 ),
 ( 0.000000000000000000, 1.000000000000000000 ),
 ( 0.000000000000000000, 1.000000000000000000 ),
 .UNSPECIFIED. ) 
 GEOMETRIC_REPRESENTATION_ITEM ( )  RATIONAL_B_SPLINE_SURFACE ( (
 ( 1.000000000000000000, 0.3333333333333334259, 0.3333333333333334259, 1.000000000000000000),
 ( 1.000000000000000000, 0.3333333333333334259, 0.3333333333333334259, 1.000000000000000000),
 ( 1.000000000000000000, 0.3333333333333334259, 0.3333333333333334259, 1.000000000000000000) ) ) 
 REPRESENTATION_ITEM ( '' )  SURFACE ( )  );
#2618=CARTESIAN_POINT ( 'NONE',  ( -3.608439182435052128, -6.250000000000110134, -141.4419872981078186 ) ) ;
#2619=CARTESIAN_POINT ( 'NONE',  ( 6.000000000000001776, 5.345404176511898156E-15, -174.6636751345948539 ) ) ;
#2621=CARTESIAN_POINT ( 'NONE',  ( 0.000000000000000000, 5.999999999999977796, -129.2886751345947971 ) ) ;
#2628=CARTESIAN_POINT ( 'NONE',  ( 5.999999999999949374, 1.607695154586804565, -60.59668783648704249 ) ) ;
#2629=SURFACE_STYLE_FILL_AREA ( #23545 ) ;
#2632=CARTESIAN_POINT ( 'NONE',  ( 5.999999999999988454, 1.607695154586737729, -149.0966878364870922 ) ) ;
#2634=CARTESIAN_POINT ( 'NONE',  ( -5.196152422706573404, -3.000000000000002665, -107.2113248654052455 ) ) ;
#2635=CARTESIAN_POINT ( 'NONE',  ( 6.000000000000000888, 7.762456499804234384E-14, -132.6636751345948539 ) ) ;
#2636=CARTESIAN_POINT ( 'NONE',  ( -5.999999999999919176, 1.607695154586804565, -120.9033121635129930 ) ) ;
#2642=CARTESIAN_POINT ( 'NONE',  ( -5.412658773652739619, 3.124999999999975131, -101.3169872981078470 ) ) ;
#2643=CARTESIAN_POINT ( 'NONE',  ( 0.000000000000000000, 5.999999999999977796, -176.7113248654052029 ) ) ;
#2647=CARTESIAN_POINT ( 'NONE',  ( -6.350852961085760029, -1.281975124255709124E-13, -131.6250000000000284 ) ) ;
#2649=CARTESIAN_POINT ( 'NONE',  ( 6.350852961086080661, -9.614813431917819062E-14, -57.37500000000004974 ) ) ;
#2650=CARTESIAN_POINT ( 'NONE',  ( 6.000000000000000888, -1.859271017917181981E-14, -116.1636751345948255 ) ) ;
#2651=DIRECTION ( 'NONE',  ( -7.147005652999508048E-36, 5.642372883946980038E-36, 1.000000000000000000 ) ) ;
#2652=CARTESIAN_POINT ( 'NONE',  ( 5.412658773652739619, 3.124999999999988898, -86.18301270189220986 ) ) ;
#2653=( BOUNDED_CURVE ( )  B_SPLINE_CURVE ( 2, ( #2904, #7662, #2468, #11884, #9384, #28547, #28252, #4905, #4762 ),
 .UNSPECIFIED., .F., .T. ) 
 B_SPLINE_CURVE_WITH_KNOTS ( ( 3, 2, 2, 2, 3 ),
 ( 0.6361111111111110716, 0.6370370370370370683, 0.6388888888888888395, 0.6407407407407407218, 0.6416666666666667185 ),
 .UNSPECIFIED. ) 
 CURVE ( )  GEOMETRIC_REPRESENTATION_ITEM ( )  RATIONAL_B_SPLINE_CURVE ( ( 0.9330127018922194093, 0.9330127018922154125, 1.000000000000000000, 0.8660254037844388186, 1.000000000000000000, 0.8660254037844388186, 1.000000000000000000, 0.9330127018922154125, 0.9330127018922194093 ) ) 
 REPRESENTATION_ITEM ( '' )  );
#2656=CARTESIAN_POINT ( 'NONE',  ( -3.464101615137725076, 5.999999999999979572, -139.6636751345947971 ) ) ;
#2659=CARTESIAN_POINT ( 'NONE',  ( 3.175426480543072749, 5.499999999999865885, -144.1250000000000000 ) ) ;
#2661=CARTESIAN_POINT ( 'NONE',  ( -5.412658773652684552, -3.125000000000099920, -154.4330127018922383 ) ) ;
#2662=CARTESIAN_POINT ( 'NONE',  ( 0.000000000000000000, 5.999999999999977796, -116.7113248654052597 ) ) ;
#2664=CARTESIAN_POINT ( 'NONE',  ( 3.175426480543072749, 5.499999999999865885, -69.12500000000002842 ) ) ;
#2666=CARTESIAN_POINT ( 'NONE',  ( 3.175426480543072749, 5.499999999999865885, -61.62500000000000000 ) ) ;
#2667=CARTESIAN_POINT ( 'NONE',  ( 0.000000000000000000, -5.999999999999991118, -148.0386751345948539 ) ) ;
#2674=EDGE_LOOP ( 'NONE', ( #27119, #10105, #17595, #4465 ) ) ;
#2679=CARTESIAN_POINT ( 'NONE',  ( 5.999999999999949374, 1.607695154586804565, -64.51933756729744118 ) ) ;
#2680=CARTESIAN_POINT ( 'NONE',  ( 3.175426480543072749, -5.500000000000105693, -179.1250000000000568 ) ) ;
#2682=VERTEX_POINT ( 'NONE', #19250 ) ;
#2684=CARTESIAN_POINT ( 'NONE',  ( -6.350852961085760029, -1.281975124255709124E-13, -86.62499999999998579 ) ) ;
#2685=TOROIDAL_SURFACE ( 'NONE', #10053, 9.999999999999998224, 1.000000000000000000 ) ;
#2687=ORIENTED_EDGE ( 'NONE', *, *, #11577, .T. ) ;
#2691=CARTESIAN_POINT ( 'NONE',  ( -5.999999999999963585, 1.780251999655701777E-13, -94.41367513459482552 ) ) ;
#2692=CARTESIAN_POINT ( 'NONE',  ( 4.509628467067703816, -10.03401783428612326, -21.03762154299058906 ) ) ;
#2693=CARTESIAN_POINT ( 'NONE',  ( 5.196152422706629359, -2.999999999999988898, -67.71132486540520290 ) ) ;
#2694=CARTESIAN_POINT ( 'NONE',  ( -4.763139720814407951, -2.750000000000016431, -166.0000000000000284 ) ) ;
#2695=CARTESIAN_POINT ( 'NONE',  ( 6.000000000000000888, -1.607695154586752384, -80.23066243270258724 ) ) ;
#2696=CARTESIAN_POINT ( 'NONE',  ( -6.350852961085760029, -1.281975124255709124E-13, -152.6250000000000568 ) ) ;
#2698=CARTESIAN_POINT ( 'NONE',  ( -3.464101615137757051, -5.999999999999979572, -52.16367513459485394 ) ) ;
#2699=( BOUNDED_CURVE ( )  B_SPLINE_CURVE ( 2, ( #8153, #26887, #20000, #5400, #29352, #22310, #24759, #24594, #24440 ),
 .UNSPECIFIED., .F., .F. ) 
 B_SPLINE_CURVE_WITH_KNOTS ( ( 3, 2, 2, 2, 3 ),
 ( 0.9027777777777777901, 0.9037037037037036757, 0.9055555555555555580, 0.9074074074074074403, 0.9083333333333333259 ),
 .UNSPECIFIED. ) 
 CURVE ( )  GEOMETRIC_REPRESENTATION_ITEM ( )  RATIONAL_B_SPLINE_CURVE ( ( 0.9330127018922194093, 0.9330127018922194093, 1.000000000000000000, 0.8660254037844388186, 1.000000000000000000, 0.8660254037844388186, 1.000000000000000000, 0.9330127018922194093, 0.9330127018922194093 ) ) 
 REPRESENTATION_ITEM ( '' )  );
#2701=CARTESIAN_POINT ( 'NONE',  ( -2.775557561562891351E-14, -5.500000000000115463, -89.25000000000005684 ) ) ;
#2703=CARTESIAN_POINT ( 'NONE',  ( 0.000000000000000000, 0.000000000000000000, 0.000000000000000000 ) ) ;
#2707=CARTESIAN_POINT ( 'NONE',  ( 6.000000000000000888, 7.762456499804235646E-14, -129.6636751345948255 ) ) ;
#2708=VERTEX_POINT ( 'NONE', #12651 ) ;
#2709=AXIS2_PLACEMENT_3D ( 'NONE', #5352, #16637, #5203 ) ;
#2710=CARTESIAN_POINT ( 'NONE',  ( 6.000000000000000888, 7.762456499804235646E-14, -117.6636751345948255 ) ) ;
#2712=EDGE_CURVE ( 'NONE', #11265, #20245, #26137, .T. ) ;
#2713=ORIENTED_EDGE ( 'NONE', *, *, #3850, .T. ) ;
#2717=CARTESIAN_POINT ( 'NONE',  ( -3.175426480542816510, -5.500000000000057732, -110.3750000000000426 ) ) ;
#2720=CARTESIAN_POINT ( 'NONE',  ( -3.608439182435052128, -6.250000000000110134, -125.8080127018922383 ) ) ;
#2723=CARTESIAN_POINT ( 'NONE',  ( 2.775557561562891351E-14, 6.250000000000033751, -158.5669872981078186 ) ) ;
#2727=CARTESIAN_POINT ( 'NONE',  ( 2.799076333356274106E-14, 11.00000000000000000, -19.00000000000002132 ) ) ;
#2728=CARTESIAN_POINT ( 'NONE',  ( -4.763139720814407951, 2.749999999999946709, -181.2500000000000284 ) ) ;
#2731=CARTESIAN_POINT ( 'NONE',  ( 3.608439182435180470, 6.249999999999982236, -176.0580127018922667 ) ) ;
#2732=DIRECTION ( 'NONE',  ( 1.000000000000000000, -5.551115123125773458E-17, -1.260129944081490338E-35 ) ) ;
#2733=CARTESIAN_POINT ( 'NONE',  ( -5.999999999999962697, 3.323446944526963891E-14, -161.9136751345948539 ) ) ;
#2734=CARTESIAN_POINT ( 'NONE',  ( -2.775557561562891351E-14, -5.500000000000115463, -123.7500000000000284 ) ) ;
#2737=CARTESIAN_POINT ( 'NONE',  ( -3.175426480542816510, 5.499999999999865885, -113.8750000000000000 ) ) ;
#2739=CARTESIAN_POINT ( 'NONE',  ( 5.196152422706629359, 3.000000000000002665, -101.0386751345948539 ) ) ;
#2744=CARTESIAN_POINT ( 'NONE',  ( -3.464101615137725076, 5.999999999999979572, -168.1636751345948255 ) ) ;
#2746=PLANE ( 'NONE',  #8076 ) ;
#2748=CARTESIAN_POINT ( 'NONE',  ( 6.000000000000000888, 1.743066579297358182E-13, -87.08632486540520290 ) ) ;
#2751=CARTESIAN_POINT ( 'NONE',  ( -4.763139720814407951, 2.749999999999946709, -179.7500000000000284 ) ) ;
#2754=ORIENTED_EDGE ( 'NONE', *, *, #10445, .T. ) ;
#2757=ORIENTED_EDGE ( 'NONE', *, *, #23319, .T. ) ;
#2762=CARTESIAN_POINT ( 'NONE',  ( 5.412658773652712085, -3.125000000000086153, -129.0669872981078470 ) ) ;
#2765=VERTEX_POINT ( 'NONE', #24889 ) ;
#2769=FACE_OUTER_BOUND ( 'NONE', #17397, .T. ) ;
#2772=CARTESIAN_POINT ( 'NONE',  ( 6.000000000000052403, -1.607695154586662678, -99.15331216351297883 ) ) ;
#2773=CARTESIAN_POINT ( 'NONE',  ( 5.196152422706629359, 3.000000000000002665, -146.9613248654052597 ) ) ;
#2775=( NAMED_UNIT ( * ) PLANE_ANGLE_UNIT ( ) SI_UNIT ( $, .RADIAN. ) );
#2780=CARTESIAN_POINT ( 'NONE',  ( 3.175426480543072749, 5.499999999999865885, -48.12500000000000000 ) ) ;
#2783=EDGE_LOOP ( 'NONE', ( #3660, #529, #9080, #20842 ) ) ;
#2788=CARTESIAN_POINT ( 'NONE',  ( -3.608439182435052128, -6.250000000000110134, -100.9419872981078186 ) ) ;
#2789=CARTESIAN_POINT ( 'NONE',  ( -5.999999999999971578, 1.607695154586715303, -172.4806624327026157 ) ) ;
#2790=ADVANCED_FACE ( 'NONE', ( #26875 ), #1230, .T. ) ;
#2794=AXIS2_PLACEMENT_3D ( 'NONE', #3371, #24884, #24425 ) ;
#2795=CARTESIAN_POINT ( 'NONE',  ( 0.000000000000000000, 5.499999999999991118, -127.5000000000000568 ) ) ;
#2798=CARTESIAN_POINT ( 'NONE',  ( 0.000000000000000000, 5.499999999999991118, -60.00000000000005684 ) ) ;
#2799=CARTESIAN_POINT ( 'NONE',  ( 3.464101615137757051, -5.999999999999979572, -81.33632486540523132 ) ) ;
#2801=CARTESIAN_POINT ( 'NONE',  ( 2.775557561562891351E-14, 6.250000000000033751, -82.93301270189223828 ) ) ;
#2802=CARTESIAN_POINT ( 'NONE',  ( 2.775557561562891351E-14, 10.99999999999998224, -31.00000000000002842 ) ) ;
#2804=CARTESIAN_POINT ( 'NONE',  ( 5.999999999999999112, 2.951592740943527306E-14, -150.0863248654052313 ) ) ;
#2806=LINE ( 'NONE', #9896, #23463 ) ;
#2807=CARTESIAN_POINT ( 'NONE',  ( 5.999999999999949374, 1.607695154586804565, -61.51933756729744118 ) ) ;
#2809=CARTESIAN_POINT ( 'NONE',  ( -4.763139720814407951, 2.749999999999946709, -140.7500000000000284 ) ) ;
#2811=CARTESIAN_POINT ( 'NONE',  ( -5.412658773652739619, 3.124999999999975131, -150.1830127018922667 ) ) ;
#2812=CARTESIAN_POINT ( 'NONE',  ( -5.999999999999963585, -1.487416814333745711E-14, -101.3363248654052171 ) ) ;
#2813=VECTOR ( 'NONE', #2540, 1000.000000000000000 ) ;
#2815=EDGE_CURVE ( 'NONE', #2765, #25369, #27340, .T. ) ;
#2816=CARTESIAN_POINT ( 'NONE',  ( -4.763139720814407951, -2.750000000000016431, -68.50000000000000000 ) ) ;
#2817=CARTESIAN_POINT ( 'NONE',  ( -5.999999999999963585, 1.780251999655701777E-13, -85.41367513459483973 ) ) ;
#2818=CARTESIAN_POINT ( 'NONE',  ( -2.775557561562891351E-14, -5.500000000000115463, -68.25000000000002842 ) ) ;
#2819=CARTESIAN_POINT ( 'NONE',  ( 6.000000000000000888, -1.859271017917181981E-14, -54.08632486540521001 ) ) ;
#2823=CARTESIAN_POINT ( 'NONE',  ( -5.999999999999971578, 1.607695154586715303, -133.4806624327025872 ) ) ;
#2824=CARTESIAN_POINT ( 'NONE',  ( 6.000000000000000888, -1.607695154586752384, -147.1533121635130215 ) ) ;
#2826=ADVANCED_FACE ( 'NONE', ( #6159 ), #2685, .T. ) ;
#2829=VECTOR ( 'NONE', #21429, 1000.000000000000000 ) ;
#2833=CARTESIAN_POINT ( 'NONE',  ( -2.775557561562891351E-14, -5.500000000000115463, -177.7500000000000284 ) ) ;
#2836=CARTESIAN_POINT ( 'NONE',  ( -4.763139720814407951, 2.749999999999946709, -83.74999999999998579 ) ) ;
#2837=CARTESIAN_POINT ( 'NONE',  ( -5.412658773652684552, -3.125000000000099920, -98.93301270189225249 ) ) ;
#2839=MECHANICAL_DESIGN_GEOMETRIC_PRESENTATION_REPRESENTATION('',(#24414),#25396);
#2840=CARTESIAN_POINT ( 'NONE',  ( -5.999999999999963585, -1.487416814333745711E-14, -128.3363248654052029 ) ) ;
#2845=CARTESIAN_POINT ( 'NONE',  ( -3.175426480542816066, 5.499999999999865885, -166.3750000000000568 ) ) ;
#2846=CARTESIAN_POINT ( 'NONE',  ( 6.000000000000000888, 1.607695154586715303, -58.51933756729743408 ) ) ;
#2847=COLOUR_RGB ( '', 0.40784314, 0.44705882, 0.49803922) ;
#2848=CARTESIAN_POINT ( 'NONE',  ( 3.175426480543072749, 5.499999999999865885, -154.6250000000000853 ) ) ;
#2849=EDGE_CURVE ( 'NONE', #9948, #12840, #10858, .T. ) ;
#2850=CARTESIAN_POINT ( 'NONE',  ( -3.464101615137725076, 5.999999999999979572, -76.66367513459483973 ) ) ;
#2853=CARTESIAN_POINT ( 'NONE',  ( 0.000000000000000000, 5.499999999999991118, -96.00000000000002842 ) ) ;
#2855=CARTESIAN_POINT ( 'NONE',  ( -4.763139720814407951, 2.749999999999946709, -88.25000000000005684 ) ) ;
#2859=CARTESIAN_POINT ( 'NONE',  ( 6.000000000000000888, -1.859271017917181981E-14, -126.6636751345948397 ) ) ;
#2860=EDGE_CURVE ( 'NONE', #23232, #25957, #1088, .T. ) ;
#2861=DIRECTION ( 'NONE',  ( -7.147005652999508048E-36, 5.642372883946980038E-36, 1.000000000000000000 ) ) ;
#2862=ORIENTED_EDGE ( 'NONE', *, *, #14815, .T. ) ;
#2863=SURFACE_STYLE_USAGE ( .BOTH. , #14573 ) ;
#2869=CARTESIAN_POINT ( 'NONE',  ( 3.175426480543072749, 5.499999999999865885, -106.6250000000000284 ) ) ;
#2871=CARTESIAN_POINT ( 'NONE',  ( 6.350852961086080661, -9.614813431917819062E-14, -150.3749999999999716 ) ) ;
#2872=CARTESIAN_POINT ( 'NONE',  ( 5.412658773652739619, 3.124999999999988898, -122.1830127018922525 ) ) ;
#2875=CARTESIAN_POINT ( 'NONE',  ( -5.196152422706601826, 2.999999999999975131, -111.0386751345948113 ) ) ;
#2876=CARTESIAN_POINT ( 'NONE',  ( -3.608439182435115633, 6.249999999999965361, -159.9419872981077901 ) ) ;
#2879=CARTESIAN_POINT ( 'NONE',  ( 5.412658773652739619, 3.124999999999988898, -60.68301270189224539 ) ) ;
#2880=ORIENTED_EDGE ( 'NONE', *, *, #17113, .T. ) ;
#2881=CARTESIAN_POINT ( 'NONE',  ( 6.000000000000000888, -1.859271017917181981E-14, -168.0863248654052029 ) ) ;
#2882=CARTESIAN_POINT ( 'NONE',  ( -0.4007817556719547869, 11.00000000000000711, -19.00000000000001066 ) ) ;
#2884=CARTESIAN_POINT ( 'NONE',  ( -4.763139720814407951, 2.749999999999946709, -175.2500000000000284 ) ) ;
#2886=CARTESIAN_POINT ( 'NONE',  ( 5.196152422706629359, 3.000000000000002665, -100.4613248654052171 ) ) ;
#2887=CARTESIAN_POINT ( 'NONE',  ( -5.412658773652684552, -3.125000000000099920, -179.9330127018922099 ) ) ;
#2889=EDGE_CURVE ( 'NONE', #9651, #8975, #3687, .T. ) ;
#2890=CARTESIAN_POINT ( 'NONE',  ( -5.999999999999963585, 1.780251999655701777E-13, -48.83632486540521711 ) ) ;
#2891=CARTESIAN_POINT ( 'NONE',  ( 4.763139720814407951, 2.750000000000002665, -118.7500000000000284 ) ) ;
#2892=CARTESIAN_POINT ( 'NONE',  ( 0.000000000000000000, 5.999999999999977796, -84.28867513459481131 ) ) ;
#2893=CARTESIAN_POINT ( 'NONE',  ( -3.175426480542816510, 5.499999999999865885, -116.8750000000000142 ) ) ;
#2897=LINE ( 'NONE', #19205, #8416 ) ;
#2898=CARTESIAN_POINT ( 'NONE',  ( 3.464101615137757051, -5.999999999999979572, -55.83632486540525264 ) ) ;
#2901=CARTESIAN_POINT ( 'NONE',  ( -5.196152422706573404, -3.000000000000002665, -126.7113248654052597 ) ) ;
#2904=CARTESIAN_POINT ( 'NONE',  ( -5.999999999999963585, 1.780251999655701777E-13, -95.91367513459483973 ) ) ;
#2905=VERTEX_POINT ( 'NONE', #27261 ) ;
#2906=ORIENTED_EDGE ( 'NONE', *, *, #6480, .T. ) ;
#2910=CARTESIAN_POINT ( 'NONE',  ( -7.216878364870328078, 0.000000000000000000, -128.1919872981078186 ) ) ;
#2913=CARTESIAN_POINT ( 'NONE',  ( -3.464101615137757051, -5.999999999999979572, -116.6636751345947545 ) ) ;
#2918=( BOUNDED_CURVE ( )  B_SPLINE_CURVE ( 2, ( #18115, #17820, #13222, #24692, #15369, #1799, #6401, #8245, #8565 ),
 .UNSPECIFIED., .F., .T. ) 
 B_SPLINE_CURVE_WITH_KNOTS ( ( 3, 2, 2, 2, 3 ),
 ( 0.1416666666666666907, 0.1425925925925926041, 0.1444444444444444309, 0.1462962962962962854, 0.1472222222222221988 ),
 .UNSPECIFIED. ) 
 CURVE ( )  GEOMETRIC_REPRESENTATION_ITEM ( )  RATIONAL_B_SPLINE_CURVE ( ( 0.9330127018922194093, 0.9330127018922204085, 1.000000000000000000, 0.8660254037844388186, 1.000000000000000000, 0.8660254037844388186, 1.000000000000000000, 0.9330127018922205195, 0.9330127018922196314 ) ) 
 REPRESENTATION_ITEM ( '' )  );
#2921=CARTESIAN_POINT ( 'NONE',  ( 6.000000000000052403, -1.607695154586662678, -139.6533121635129930 ) ) ;
#2922=CARTESIAN_POINT ( 'NONE',  ( 5.196152422706629359, -2.999999999999988898, -69.21132486540521711 ) ) ;
#2925=CARTESIAN_POINT ( 'NONE',  ( -5.196152422706573404, -3.000000000000002665, -143.2113248654052313 ) ) ;
#2927=CARTESIAN_POINT ( 'NONE',  ( -6.350852961085760029, -1.281975124255709124E-13, -136.1250000000000568 ) ) ;
#2929=VERTEX_POINT ( 'NONE', #24959 ) ;
#2932=ADVANCED_FACE ( 'NONE', ( #29724 ), #12887, .T. ) ;
#2934=VERTEX_POINT ( 'NONE', #3608 ) ;
#2937=CARTESIAN_POINT ( 'NONE',  ( -3.608439182435115633, 6.249999999999965361, -95.44198729810779014 ) ) ;
#2938=CARTESIAN_POINT ( 'NONE',  ( 0.000000000000000000, 0.000000000000000000, 0.000000000000000000 ) ) ;
#2943=CARTESIAN_POINT ( 'NONE',  ( 0.000000000000000000, 5.499999999999991118, -126.0000000000000000 ) ) ;
#2947=CARTESIAN_POINT ( 'NONE',  ( -5.196152422706601826, 2.999999999999975131, -96.03867513459485394 ) ) ;
#2948=CARTESIAN_POINT ( 'NONE',  ( -4.763139720814407951, 2.749999999999946709, -55.25000000000002132 ) ) ;
#2951=CARTESIAN_POINT ( 'NONE',  ( 3.035671606378345100, 10.57820549248699926, -19.81012201018821273 ) ) ;
#2952=CARTESIAN_POINT ( 'NONE',  ( -5.412658773652739619, 3.124999999999975131, -81.18301270189220986 ) ) ;
#2953=CARTESIAN_POINT ( 'NONE',  ( -5.999999999999971578, 1.607695154586715303, -168.9033121635130215 ) ) ;
#2958=EDGE_CURVE ( 'NONE', #14503, #25740, #14966, .T. ) ;
#2959=CARTESIAN_POINT ( 'NONE',  ( 3.175426480543072749, 5.499999999999865885, -136.6250000000000568 ) ) ;
#2961=CARTESIAN_POINT ( 'NONE',  ( -3.608439182435115633, 6.249999999999965361, -151.8080127018922383 ) ) ;
#2963=CARTESIAN_POINT ( 'NONE',  ( 3.175426480543072749, 5.499999999999865885, -67.62500000000002842 ) ) ;
#2964=CARTESIAN_POINT ( 'NONE',  ( -4.763139720814407951, -2.750000000000016431, -61.00000000000000000 ) ) ;
#2971=AXIS2_PLACEMENT_3D ( 'NONE', #1906, #11313, #30010 ) ;
#2977=CARTESIAN_POINT ( 'NONE',  ( -3.175426480542816510, -5.500000000000057732, -179.3750000000000568 ) ) ;
#2979=CARTESIAN_POINT ( 'NONE',  ( -5.412658773652739619, 3.124999999999975131, -153.8169872981078186 ) ) ;
#2981=CARTESIAN_POINT ( 'NONE',  ( -3.175426480542816510, 5.499999999999865885, -83.87500000000004263 ) ) ;
#2983=CARTESIAN_POINT ( 'NONE',  ( 2.775557561562891351E-14, -6.250000000000061284, -100.1830127018922241 ) ) ;
#2987=CARTESIAN_POINT ( 'NONE',  ( 3.175426480543072749, 5.499999999999865885, -168.1250000000000000 ) ) ;
#2989=CARTESIAN_POINT ( 'NONE',  ( 4.754775042825850839, -9.920200456738756500, -21.33539821540183468 ) ) ;
#2992=CARTESIAN_POINT ( 'NONE',  ( 3.175426480543072749, -5.500000000000105693, -162.6250000000000568 ) ) ;
#2993=CARTESIAN_POINT ( 'NONE',  ( -3.464101615137725076, 5.999999999999979572, -161.5863248654051745 ) ) ;
#2994=CARTESIAN_POINT ( 'NONE',  ( 3.175426480543072749, -5.500000000000105693, -146.1250000000000000 ) ) ;
#2996=CARTESIAN_POINT ( 'NONE',  ( -3.175426480542816066, -5.500000000000057732, -96.87499999999997158 ) ) ;
#2997=CARTESIAN_POINT ( 'NONE',  ( 6.000000000000000888, -1.859271017917181981E-14, -126.0863248654052171 ) ) ;
#2998=( BOUNDED_CURVE ( )  B_SPLINE_CURVE ( 2, ( #16258, #9148, #11645, #11492, #25411, #13487, #27403, #9300, #13958 ),
 .UNSPECIFIED., .F., .F. ) 
 B_SPLINE_CURVE_WITH_KNOTS ( ( 3, 2, 2, 2, 3 ),
 ( 0.6416666666666667185, 0.6425925925925926041, 0.6444444444444444864, 0.6462962962962962576, 0.6472222222222221433 ),
 .UNSPECIFIED. ) 
 CURVE ( )  GEOMETRIC_REPRESENTATION_ITEM ( )  RATIONAL_B_SPLINE_CURVE ( ( 0.9330127018922194093, 0.9330127018922234061, 1.000000000000000000, 0.8660254037844388186, 1.000000000000000000, 0.8660254037844388186, 1.000000000000000000, 0.9330127018922234061, 0.9330127018922194093 ) ) 
 REPRESENTATION_ITEM ( '' )  );
#2999=CARTESIAN_POINT ( 'NONE',  ( -2.775557561562891351E-14, -5.500000000000115463, -92.25000000000000000 ) ) ;
#3001=CARTESIAN_POINT ( 'NONE',  ( -5.999999999999971578, 1.607695154586715303, -143.4033121635129930 ) ) ;
#3006=CARTESIAN_POINT ( 'NONE',  ( -6.000000000000000888, 1.067854986875958443E-15, 7.560779664488942560E-35 ) ) ;
#3008=ORIENTED_EDGE ( 'NONE', *, *, #7985, .T. ) ;
#3009=CARTESIAN_POINT ( 'NONE',  ( 5.196152422706629359, 3.000000000000002665, -179.0386751345948255 ) ) ;
#3013=VERTEX_POINT ( 'NONE', #26956 ) ;
#3014=ORIENTED_EDGE ( 'NONE', *, *, #8120, .T. ) ;
#3015=VECTOR ( 'NONE', #25712, 1000.000000000000000 ) ;
#3018=CARTESIAN_POINT ( 'NONE',  ( -2.775557561562891351E-14, -5.500000000000115463, -104.2500000000000142 ) ) ;
#3020=CARTESIAN_POINT ( 'NONE',  ( -3.608439182435052128, -6.250000000000110134, -121.3080127018921957 ) ) ;
#3022=CARTESIAN_POINT ( 'NONE',  ( -5.999999999999963585, -1.487416814333745711E-14, -118.4136751345948255 ) ) ;
#3023=CARTESIAN_POINT ( 'NONE',  ( 2.775557561562891351E-14, -6.250000000000061284, -157.8169872981078470 ) ) ;
#3027=CARTESIAN_POINT ( 'NONE',  ( -3.608439182435115633, 6.249999999999965361, -57.30801270189221697 ) ) ;
#3029=DIRECTION ( 'NONE',  ( 1.000000000000000000, -5.551115123125773458E-17, -1.260129944081490338E-35 ) ) ;
#3030=EDGE_CURVE ( 'NONE', #26278, #3569, #25738, .T. ) ;
#3031=CARTESIAN_POINT ( 'NONE',  ( -1.384933631640781648, 10.91424797897492560, -19.15860252534411146 ) ) ;
#3032=CARTESIAN_POINT ( 'NONE',  ( 6.000000000000000888, 7.762456499804234384E-14, -138.0863248654051745 ) ) ;
#3033=CARTESIAN_POINT ( 'NONE',  ( -3.175426480542816510, 5.499999999999865885, -178.3750000000000568 ) ) ;
#3036=CARTESIAN_POINT ( 'NONE',  ( 5.412658773652712085, -3.125000000000086153, -167.4330127018922667 ) ) ;
#3039=CARTESIAN_POINT ( 'NONE',  ( -4.763139720814407951, 2.749999999999946709, -119.7500000000000284 ) ) ;
#3040=CARTESIAN_POINT ( 'NONE',  ( -3.464101615137725076, 5.999999999999979572, -84.16367513459481131 ) ) ;
#3041=CARTESIAN_POINT ( 'NONE',  ( 4.763139720814407951, 2.750000000000002665, -112.7500000000000142 ) ) ;
#3043=CARTESIAN_POINT ( 'NONE',  ( -5.999999999999971578, 1.607695154586715303, -88.48066243270262987 ) ) ;
#3044=ORIENTED_EDGE ( 'NONE', *, *, #4067, .T. ) ;
#3048=ORIENTED_EDGE ( 'NONE', *, *, #16099, .T. ) ;
#3050=CARTESIAN_POINT ( 'NONE',  ( -3.175426480542816066, -5.500000000000057732, -179.3750000000000568 ) ) ;
#3051=EDGE_LOOP ( 'NONE', ( #14605, #23100, #26807, #9998 ) ) ;
#3053=VERTEX_POINT ( 'NONE', #28024 ) ;
#3055=CARTESIAN_POINT ( 'NONE',  ( 0.000000000000000000, 5.999999999999977796, -85.21132486540523132 ) ) ;
#3057=EDGE_CURVE ( 'NONE', #15338, #12734, #21000, .T. ) ;
#3058=ORIENTED_EDGE ( 'NONE', *, *, #22847, .F. ) ;
#3059=CARTESIAN_POINT ( 'NONE',  ( -3.608439182435052128, -6.250000000000110134, -130.9419872981078470 ) ) ;
#3060=LINE ( 'NONE', #26114, #29914 ) ;
#3061=CARTESIAN_POINT ( 'NONE',  ( 5.999999999999949374, 1.607695154586804565, -50.09668783648704249 ) ) ;
#3062=CYLINDRICAL_SURFACE ( 'NONE', #17718, 6.000000000000000888 ) ;
#3063=VERTEX_POINT ( 'NONE', #13495 ) ;
#3066=CARTESIAN_POINT ( 'NONE',  ( -5.196152422706573404, -3.000000000000002665, -92.21132486540523132 ) ) ;
#3067=CARTESIAN_POINT ( 'NONE',  ( 0.000000000000000000, 0.000000000000000000, 0.000000000000000000 ) ) ;
#3068=EDGE_CURVE ( 'NONE', #14517, #16677, #19282, .T. ) ;
#3070=CARTESIAN_POINT ( 'NONE',  ( -5.999999999999971578, 1.607695154586715303, -92.40331216351296462 ) ) ;
#3071=DIRECTION ( 'NONE',  ( -7.147005652999508048E-36, 5.642372883946980038E-36, 1.000000000000000000 ) ) ;
#3072=DIRECTION ( 'NONE',  ( -7.147005652999508048E-36, 5.642372883946980038E-36, 1.000000000000000000 ) ) ;
#3073=CARTESIAN_POINT ( 'NONE',  ( 6.000000000000000888, 1.743066579297358182E-13, -56.16367513459481842 ) ) ;
#3074=CARTESIAN_POINT ( 'NONE',  ( -5.999999999999956479, -1.607695154586745057, -143.2693375672974696 ) ) ;
#3075=CARTESIAN_POINT ( 'NONE',  ( 3.175426480543072749, 5.499999999999865885, -133.6250000000000284 ) ) ;
#3076=AXIS2_PLACEMENT_3D ( 'NONE', #3148, #19322, #7615 ) ;
#3077=VERTEX_POINT ( 'NONE', #27410 ) ;
#3078=CARTESIAN_POINT ( 'NONE',  ( 0.000000000000000000, 5.499999999999991118, -49.49999999999998579 ) ) ;
#3081=ORIENTED_EDGE ( 'NONE', *, *, #15845, .F. ) ;
#3083=CARTESIAN_POINT ( 'NONE',  ( -3.608439182435052128, -6.250000000000110134, -91.94198729810786119 ) ) ;
#3084=CARTESIAN_POINT ( 'NONE',  ( -3.464101615137757051, -5.999999999999979572, -78.58632486540523132 ) ) ;
#3086=ADVANCED_FACE ( 'NONE', ( #6376 ), #9310, .T. ) ;
#3087=CARTESIAN_POINT ( 'NONE',  ( -6.350852961085760029, -1.281975124255709124E-13, -133.1250000000000284 ) ) ;
#3088=( BOUNDED_CURVE ( )  B_SPLINE_CURVE ( 2, ( #25106, #6224, #13485, #15643, #18087, #15485, #5905, #20515, #3760 ),
 .UNSPECIFIED., .F., .T. ) 
 B_SPLINE_CURVE_WITH_KNOTS ( ( 3, 2, 2, 2, 3 ),
 ( 0.5750000000000000666, 0.5759259259259259522, 0.5777777777777777235, 0.5796296296296296058, 0.5805555555555554914 ),
 .UNSPECIFIED. ) 
 CURVE ( )  GEOMETRIC_REPRESENTATION_ITEM ( )  RATIONAL_B_SPLINE_CURVE ( ( 0.9330127018922194093, 0.9330127018922234061, 1.000000000000000000, 0.8660254037844388186, 1.000000000000000000, 0.8660254037844388186, 1.000000000000000000, 0.9330127018922234061, 0.9330127018922194093 ) ) 
 REPRESENTATION_ITEM ( '' )  );
#3092=CARTESIAN_POINT ( 'NONE',  ( 5.196152422706629359, -2.999999999999988898, -82.71132486540521711 ) ) ;
#3093=CARTESIAN_POINT ( 'NONE',  ( -3.175426480542816510, -5.500000000000057732, -59.37500000000005684 ) ) ;
#3094=CARTESIAN_POINT ( 'NONE',  ( -5.999999999999963585, -1.487416814333745711E-14, -101.9136751345948397 ) ) ;
#3095=CARTESIAN_POINT ( 'NONE',  ( 6.000000000000000888, 1.743066579297358182E-13, -62.16367513459481131 ) ) ;
#3096=EDGE_CURVE ( 'NONE', #2061, #14641, #6515, .T. ) ;
#3097=CARTESIAN_POINT ( 'NONE',  ( 5.412658773652739619, 3.124999999999988898, -74.18301270189225249 ) ) ;
#3098=PRODUCT_DEFINITION_FORMATION_WITH_SPECIFIED_SOURCE ( 'ANY', '', #30020, .NOT_KNOWN. ) ;
#3100=DIRECTION ( 'NONE',  ( -7.147005652999508048E-36, 5.642372883946980038E-36, 1.000000000000000000 ) ) ;
#3103=CARTESIAN_POINT ( 'NONE',  ( -4.763139720814407951, -2.750000000000016431, -142.0000000000000284 ) ) ;
#3105=CARTESIAN_POINT ( 'NONE',  ( -3.608439182435115633, 6.249999999999965361, -156.3080127018922383 ) ) ;
#3108=CARTESIAN_POINT ( 'NONE',  ( -4.763139720814407951, -2.750000000000016431, -71.50000000000001421 ) ) ;
#3109=CARTESIAN_POINT ( 'NONE',  ( 6.000000000000000888, 1.743066579297358182E-13, -104.1636751345948397 ) ) ;
#3110=CARTESIAN_POINT ( 'NONE',  ( -6.350852961085760029, -1.281975124255709124E-13, -59.62500000000000000 ) ) ;
#3111=CARTESIAN_POINT ( 'NONE',  ( -5.999999999999963585, 1.780251999655701777E-13, -53.33632486540522422 ) ) ;
#3114=VECTOR ( 'NONE', #27005, 1000.000000000000000 ) ;
#3121=ORIENTED_EDGE ( 'NONE', *, *, #22620, .F. ) ;
#3123=EDGE_CURVE ( 'NONE', #22623, #8626, #2402, .T. ) ;
#3124=ADVANCED_FACE ( 'NONE', ( #4380 ), #27557, .T. ) ;
#3125=CARTESIAN_POINT ( 'NONE',  ( -4.763139720814407951, -2.750000000000016431, -178.0000000000000568 ) ) ;
#3127=CARTESIAN_POINT ( 'NONE',  ( 5.412658773652712085, -3.125000000000086153, -153.0669872981078470 ) ) ;
#3129=CARTESIAN_POINT ( 'NONE',  ( 0.000000000000000000, 5.499999999999991118, -78.00000000000001421 ) ) ;
#3130=CARTESIAN_POINT ( 'NONE',  ( 3.608439182435180470, 6.249999999999982236, -102.5580127018922383 ) ) ;
#3131=VERTEX_POINT ( 'NONE', #25256 ) ;
#3134=CARTESIAN_POINT ( 'NONE',  ( 3.027755249632174461, -10.58056329815971175, -19.80527582512398155 ) ) ;
#3137=CARTESIAN_POINT ( 'NONE',  ( -3.175426480542816066, -5.500000000000057732, -165.8750000000000568 ) ) ;
#3139=CARTESIAN_POINT ( 'NONE',  ( -6.350852961085760029, -1.281975124255709124E-13, -146.6250000000000284 ) ) ;
#3142=CARTESIAN_POINT ( 'NONE',  ( 4.763139720814407951, -2.749999999999988454, -95.00000000000002842 ) ) ;
#3144=CARTESIAN_POINT ( 'NONE',  ( 6.350852961086080661, -9.614813431917819062E-14, -78.37500000000001421 ) ) ;
#3145=CARTESIAN_POINT ( 'NONE',  ( 3.464101615137852974, 5.999999999999884537, -143.8363248654052029 ) ) ;
#3148=CARTESIAN_POINT ( 'NONE',  ( 0.000000000000000000, 0.000000000000000000, 0.000000000000000000 ) ) ;
#3151=ORIENTED_EDGE ( 'NONE', *, *, #19399, .T. ) ;
#3157=ORIENTED_EDGE ( 'NONE', *, *, #5433, .T. ) ;
#3161=CARTESIAN_POINT ( 'NONE',  ( 4.763139720814407951, -2.749999999999988454, -102.5000000000000284 ) ) ;
#3163=CARTESIAN_POINT ( 'NONE',  ( -5.412658773652739619, 3.124999999999975131, -126.1830127018922525 ) ) ;
#3166=CARTESIAN_POINT ( 'NONE',  ( 7.216878364870455975, -6.409875621278545621E-14, -160.4419872981077901 ) ) ;
#3170=CARTESIAN_POINT ( 'NONE',  ( 3.608439182435180470, 6.249999999999982236, -62.05801270189223828 ) ) ;
#3171=ORIENTED_EDGE ( 'NONE', *, *, #23133, .F. ) ;
#3173=( BOUNDED_CURVE ( )  B_SPLINE_CURVE ( 2, ( #7581, #12249, #23744, #21285, #28322, #26027, #26317, #26172, #23882 ),
 .UNSPECIFIED., .F., .T. ) 
 B_SPLINE_CURVE_WITH_KNOTS ( ( 3, 2, 2, 2, 3 ),
 ( 0.2694444444444444309, 0.2703703703703703720, 0.2722222222222221988, 0.2740740740740740811, 0.2750000000000000222 ),
 .UNSPECIFIED. ) 
 CURVE ( )  GEOMETRIC_REPRESENTATION_ITEM ( )  RATIONAL_B_SPLINE_CURVE ( ( 0.9330127018922194093, 0.9330127018922174109, 1.000000000000000000, 0.8660254037844388186, 1.000000000000000000, 0.8660254037844388186, 1.000000000000000000, 0.9330127018922174109, 0.9330127018922194093 ) ) 
 REPRESENTATION_ITEM ( '' )  );
#3174=CARTESIAN_POINT ( 'NONE',  ( -5.999486246981926563, 9.219878802943876295, -25.40874315777524117 ) ) ;
#3176=CARTESIAN_POINT ( 'NONE',  ( -2.775557561562891351E-14, -5.500000000000115463, -168.7500000000000000 ) ) ;
#3178=CARTESIAN_POINT ( 'NONE',  ( -5.196152422706573404, -3.000000000000002665, -113.2113248654051887 ) ) ;
#3179=CARTESIAN_POINT ( 'NONE',  ( 5.412658773652712085, -3.125000000000086153, -168.9330127018922099 ) ) ;
#3182=CARTESIAN_POINT ( 'NONE',  ( 3.175426480543072749, -5.500000000000105693, -117.6250000000000284 ) ) ;
#3183=CARTESIAN_POINT ( 'NONE',  ( -6.350852961085760029, -1.281975124255709124E-13, -103.1250000000000000 ) ) ;
#3191=CARTESIAN_POINT ( 'NONE',  ( 0.000000000000000000, -5.999999999999991118, -127.0386751345948255 ) ) ;
#3192=CARTESIAN_POINT ( 'NONE',  ( 7.216878364870455975, -6.409875621278545621E-14, -83.94198729810781856 ) ) ;
#3195=EDGE_CURVE ( 'NONE', #25601, #18584, #29039, .T. ) ;
#3196=VERTEX_POINT ( 'NONE', #5539 ) ;
#3198=ORIENTED_EDGE ( 'NONE', *, *, #30089, .F. ) ;
#3200=CARTESIAN_POINT ( 'NONE',  ( -5.412658773652684552, -3.125000000000099920, -128.0669872981078470 ) ) ;
#3201=CARTESIAN_POINT ( 'NONE',  ( 0.000000000000000000, 5.999999999999977796, -49.78867513459483973 ) ) ;
#3205=CARTESIAN_POINT ( 'NONE',  ( 3.464101615137757051, -5.999999999999979572, -138.9136751345947971 ) ) ;
#3206=CARTESIAN_POINT ( 'NONE',  ( -5.999999999999963585, 8.134310703387671600E-14, -136.4136751345948255 ) ) ;
#3208=CARTESIAN_POINT ( 'NONE',  ( -3.464101615137757051, -5.999999999999979572, -99.58632486540520290 ) ) ;
#3214=CARTESIAN_POINT ( 'NONE',  ( 6.000000000000000888, 7.762456499804234384E-14, -128.1636751345948539 ) ) ;
#3215=DIRECTION ( 'NONE',  ( 1.000000000000000000, -5.551115123125773458E-17, -1.260129944081490338E-35 ) ) ;
#3217=CARTESIAN_POINT ( 'NONE',  ( 0.000000000000000000, 5.999999999999977796, -173.7113248654052029 ) ) ;
#3219=CARTESIAN_POINT ( 'NONE',  ( 6.350852961086080661, -9.614813431917819062E-14, -49.87500000000000711 ) ) ;
#3227=CARTESIAN_POINT ( 'NONE',  ( 3.608439182435180470, 6.249999999999982236, -97.19198729810780435 ) ) ;
#3228=CARTESIAN_POINT ( 'NONE',  ( 5.196152422706629359, -2.999999999999988898, -50.28867513459483973 ) ) ;
#3229=EDGE_CURVE ( 'NONE', #22623, #9072, #16562, .T. ) ;
#3233=AXIS2_PLACEMENT_3D ( 'NONE', #2703, #553, #16882 ) ;
#3237=CARTESIAN_POINT ( 'NONE',  ( -6.350852961085760029, -1.281975124255709124E-13, -58.12500000000005684 ) ) ;
#3240=CARTESIAN_POINT ( 'NONE',  ( 0.000000000000000000, 5.999999999999977796, -67.78867513459485394 ) ) ;
#3243=CARTESIAN_POINT ( 'NONE',  ( 0.000000000000000000, 0.000000000000000000, 0.000000000000000000 ) ) ;
#3245=CARTESIAN_POINT ( 'NONE',  ( -5.999999999999956479, -1.607695154586745057, -168.7693375672974128 ) ) ;
#3247=CARTESIAN_POINT ( 'NONE',  ( 4.763139720814407951, -2.749999999999988454, -143.0000000000000284 ) ) ;
#3249=CARTESIAN_POINT ( 'NONE',  ( 7.216878364870455975, -6.409875621278545621E-14, -153.8080127018922099 ) ) ;
#3251=CARTESIAN_POINT ( 'NONE',  ( 0.000000000000000000, 5.999999999999977796, -67.21132486540520290 ) ) ;
#3253=CARTESIAN_POINT ( 'NONE',  ( 4.763139720814407951, -2.749999999999988454, -74.00000000000001421 ) ) ;
#3254=CARTESIAN_POINT ( 'NONE',  ( -4.763139720814407951, 2.749999999999946709, -53.75000000000002132 ) ) ;
#3256=VERTEX_POINT ( 'NONE', #229 ) ;
#3261=CARTESIAN_POINT ( 'NONE',  ( 0.000000000000000000, -5.999999999999991118, -88.96132486540520290 ) ) ;
#3264=( BOUNDED_CURVE ( )  B_SPLINE_CURVE ( 2, ( #17857, #18151, #29937, #13553, #27621, #8283, #25317, #8602, #4134 ),
 .UNSPECIFIED., .F., .T. ) 
 B_SPLINE_CURVE_WITH_KNOTS ( ( 3, 2, 2, 2, 3 ),
 ( 0.08055555555555556080, 0.08148148148148148806, 0.08333333333333332871, 0.08518518518518518323, 0.08611111111111111049 ),
 .UNSPECIFIED. ) 
 CURVE ( )  GEOMETRIC_REPRESENTATION_ITEM ( )  RATIONAL_B_SPLINE_CURVE ( ( 0.9330127018922194093, 0.9330127018922194093, 1.000000000000000000, 0.8660254037844388186, 1.000000000000000000, 0.8660254037844388186, 1.000000000000000000, 0.9330127018922194093, 0.9330127018922194093 ) ) 
 REPRESENTATION_ITEM ( '' )  );
#3265=ADVANCED_FACE ( 'NONE', ( #25212 ), #2196, .T. ) ;
#3266=VERTEX_POINT ( 'NONE', #11600 ) ;
#3270=CARTESIAN_POINT ( 'NONE',  ( -3.464101615137757051, -5.999999999999979572, -102.5863248654052171 ) ) ;
#3271=CARTESIAN_POINT ( 'NONE',  ( -3.175426480542816510, -5.500000000000057732, -177.8750000000000568 ) ) ;
#3274=CARTESIAN_POINT ( 'NONE',  ( -5.412658773652684552, -3.125000000000099920, -147.5669872981077901 ) ) ;
#3275=ORIENTED_EDGE ( 'NONE', *, *, #6016, .T. ) ;
#3276=CARTESIAN_POINT ( 'NONE',  ( -6.350852961085760029, -1.281975124255709124E-13, -85.12499999999998579 ) ) ;
#3278=CARTESIAN_POINT ( 'NONE',  ( 5.412658773652739619, 3.124999999999988898, -92.18301270189222407 ) ) ;
#3279=CARTESIAN_POINT ( 'NONE',  ( -3.464101615137725076, 5.999999999999979572, -175.6636751345948539 ) ) ;
#3281=DIRECTION ( 'NONE',  ( 1.000000000000000000, -5.551115123125773458E-17, -1.260129944081490338E-35 ) ) ;
#3285=CARTESIAN_POINT ( 'NONE',  ( -4.763139720814407951, -2.750000000000016431, -167.4999999999999716 ) ) ;
#3286=LINE ( 'NONE', #12712, #12391 ) ;
#3287=CARTESIAN_POINT ( 'NONE',  ( 4.763139720814407951, 2.750000000000002665, -150.2500000000000000 ) ) ;
#3288=DIRECTION ( 'NONE',  ( 1.000000000000000000, -5.551115123125773458E-17, -1.260129944081490338E-35 ) ) ;
#3289=EDGE_CURVE ( 'NONE', #8702, #19684, #9255, .T. ) ;
#3290=CARTESIAN_POINT ( 'NONE',  ( -3.175426480542816066, 5.499999999999865885, -97.37499999999997158 ) ) ;
#3293=CARTESIAN_POINT ( 'NONE',  ( -3.175426480542816510, 5.499999999999865885, -80.87500000000002842 ) ) ;
#3296=CARTESIAN_POINT ( 'NONE',  ( 0.000000000000000000, 5.999999999999977796, -64.78867513459485394 ) ) ;
#3298=CARTESIAN_POINT ( 'NONE',  ( 0.000000000000000000, 0.000000000000000000, 0.000000000000000000 ) ) ;
#3299=CARTESIAN_POINT ( 'NONE',  ( -3.464101615137725076, 5.999999999999979572, -128.5863248654052029 ) ) ;
#3301=EDGE_CURVE ( 'NONE', #17475, #9162, #15810, .T. ) ;
#3302=CARTESIAN_POINT ( 'NONE',  ( 0.000000000000000000, 5.999999999999977796, -78.28867513459481131 ) ) ;
#3303=ORIENTED_EDGE ( 'NONE', *, *, #18154, .T. ) ;
#3304=CARTESIAN_POINT ( 'NONE',  ( 3.464101615137852974, 5.999999999999884537, -73.33632486540520290 ) ) ;
#3305=CARTESIAN_POINT ( 'NONE',  ( 3.464101615137852974, 5.999999999999884537, -82.91367513459479710 ) ) ;
#3306=CARTESIAN_POINT ( 'NONE',  ( 6.000000000000000888, -1.859271017917181981E-14, -115.5863248654052171 ) ) ;
#3308=ORIENTED_EDGE ( 'NONE', *, *, #5000, .T. ) ;
#3310=CARTESIAN_POINT ( 'NONE',  ( 3.175426480543072749, 5.499999999999865885, -102.1250000000000142 ) ) ;
#3311=CARTESIAN_POINT ( 'NONE',  ( 3.608439182435180470, 6.249999999999982236, -119.0580127018922667 ) ) ;
#3313=CARTESIAN_POINT ( 'NONE',  ( -3.464101615137757051, -5.999999999999979572, -61.16367513459483263 ) ) ;
#3314=CARTESIAN_POINT ( 'NONE',  ( -5.412658773652739619, 3.124999999999975131, -159.8169872981078470 ) ) ;
#3315=CARTESIAN_POINT ( 'NONE',  ( -6.000000000000000888, 1.067854986875958443E-15, 7.560779664488942560E-35 ) ) ;
#3317=CARTESIAN_POINT ( 'NONE',  ( 7.216878364870455975, -6.409875621278545621E-14, -62.30801270189223828 ) ) ;
#3319=CARTESIAN_POINT ( 'NONE',  ( -5.196152422706601826, 2.999999999999975131, -117.0386751345948682 ) ) ;
#3320=CARTESIAN_POINT ( 'NONE',  ( -5.999999999999963585, 1.780251999655701777E-13, -98.91367513459483973 ) ) ;
#3321=CARTESIAN_POINT ( 'NONE',  ( -5.801553858104669281, 9.346157964213334779, -26.58091173639826366 ) ) ;
#3322=LINE ( 'NONE', #22240, #578 ) ;
#3323=CARTESIAN_POINT ( 'NONE',  ( 6.350852961086080661, -9.614813431917819062E-14, -169.8750000000000568 ) ) ;
#3326=CARTESIAN_POINT ( 'NONE',  ( 2.775557561562891351E-14, 6.250000000000033751, -169.9330127018922099 ) ) ;
#3330=CARTESIAN_POINT ( 'NONE',  ( 3.175426480543072749, 5.499999999999865885, -117.1249999999999858 ) ) ;
#3332=ADVANCED_FACE ( 'NONE', ( #17656 ), #17361, .T. ) ;
#3333=CARTESIAN_POINT ( 'NONE',  ( 4.763139720814407951, -2.749999999999988454, -108.5000000000000426 ) ) ;
#3339=ORIENTED_EDGE ( 'NONE', *, *, #12241, .F. ) ;
#3340=CARTESIAN_POINT ( 'NONE',  ( 3.175426480543072749, -5.500000000000105693, -161.1250000000000284 ) ) ;
#3341=CARTESIAN_POINT ( 'NONE',  ( -5.196152422706601826, 2.999999999999975131, -156.0386751345948539 ) ) ;
#3342=CARTESIAN_POINT ( 'NONE',  ( -5.412658773652684552, -3.125000000000099920, -81.56698729810784698 ) ) ;
#3343=ORIENTED_EDGE ( 'NONE', *, *, #28060, .T. ) ;
#3344=DIRECTION ( 'NONE',  ( -7.147005652999508048E-36, 5.642372883946980038E-36, 1.000000000000000000 ) ) ;
#3347=( BOUNDED_CURVE ( )  B_SPLINE_CURVE ( 2, ( #2311, #14324, #30405, #9374, #16626, #9530, #4893, #29943, #8923 ),
 .UNSPECIFIED., .F., .T. ) 
 B_SPLINE_CURVE_WITH_KNOTS ( ( 3, 2, 2, 2, 3 ),
 ( 0.2638888888888888951, 0.2648148148148148362, 0.2666666666666666630, 0.2685185185185185452, 0.2694444444444444309 ),
 .UNSPECIFIED. ) 
 CURVE ( )  GEOMETRIC_REPRESENTATION_ITEM ( )  RATIONAL_B_SPLINE_CURVE ( ( 0.9330127018922194093, 0.9330127018922194093, 1.000000000000000000, 0.8660254037844388186, 1.000000000000000000, 0.8660254037844388186, 1.000000000000000000, 0.9330127018922214077, 0.9330127018922194093 ) ) 
 REPRESENTATION_ITEM ( '' )  );
#3349=CARTESIAN_POINT ( 'NONE',  ( 3.608439182435180470, -6.249999999999997335, -133.6919872981078470 ) ) ;
#3350=DIRECTION ( 'NONE',  ( -7.147005652999508048E-36, 5.642372883946980038E-36, 1.000000000000000000 ) ) ;
#3351=CARTESIAN_POINT ( 'NONE',  ( 5.196152422706629359, 3.000000000000002665, -47.96132486540521711 ) ) ;
#3355=CARTESIAN_POINT ( 'NONE',  ( -5.999999999999963585, 1.780251999655701777E-13, -60.83632486540522422 ) ) ;
#3358=CARTESIAN_POINT ( 'NONE',  ( 0.000000000000000000, -5.999999999999991118, -55.03867513459481842 ) ) ;
#3360=CARTESIAN_POINT ( 'NONE',  ( 3.608439182435180470, -6.249999999999997335, -69.19198729810781856 ) ) ;
#3361=CARTESIAN_POINT ( 'NONE',  ( -3.608439182435052128, -6.250000000000110134, -51.44198729810784698 ) ) ;
#3362=CARTESIAN_POINT ( 'NONE',  ( -5.999999999999956479, -1.607695154586745057, -128.8466878364870354 ) ) ;
#3366=CARTESIAN_POINT ( 'NONE',  ( 4.763139720814407951, -2.749999999999988454, -129.5000000000000000 ) ) ;
#3367=CARTESIAN_POINT ( 'NONE',  ( 0.000000000000000000, 0.000000000000000000, 0.000000000000000000 ) ) ;
#3369=CARTESIAN_POINT ( 'NONE',  ( 3.464101615137852974, 5.999999999999884537, -173.8363248654051461 ) ) ;
#3371=CARTESIAN_POINT ( 'NONE',  ( 0.000000000000000000, 0.000000000000000000, 0.000000000000000000 ) ) ;
#3376=ORIENTED_EDGE ( 'NONE', *, *, #22189, .F. ) ;
#3380=CARTESIAN_POINT ( 'NONE',  ( 2.775557561562891351E-14, 6.250000000000033751, -97.06698729810780435 ) ) ;
#3381=CARTESIAN_POINT ( 'NONE',  ( 3.464101615137757051, -5.999999999999979572, -50.41367513459484684 ) ) ;
#3387=CARTESIAN_POINT ( 'NONE',  ( 5.196152422706629359, 3.000000000000002665, -81.53867513459483973 ) ) ;
#3389=CARTESIAN_POINT ( 'NONE',  ( 6.350852961086080661, -9.614813431917819062E-14, -52.87500000000002132 ) ) ;
#3392=CARTESIAN_POINT ( 'NONE',  ( 0.000000000000000000, -5.999999999999991118, -51.46132486540522422 ) ) ;
#3393=CARTESIAN_POINT ( 'NONE',  ( -3.608439182435115633, 6.249999999999965361, -73.80801270189223828 ) ) ;
#3394=CARTESIAN_POINT ( 'NONE',  ( 0.000000000000000000, -5.999999999999991118, -172.9613248654052313 ) ) ;
#3397=( BOUNDED_CURVE ( )  B_SPLINE_CURVE ( 2, ( #3704, #20464, #10821, #22931, #8637, #18041, #13590, #13289, #20172 ),
 .UNSPECIFIED., .F., .F. ) 
 B_SPLINE_CURVE_WITH_KNOTS ( ( 3, 2, 2, 2, 3 ),
 ( 0.02499999999999999445, 0.02592592592592592518, 0.02777777777777777624, 0.02962962962962963076, 0.03055555555555556149 ),
 .UNSPECIFIED. ) 
 CURVE ( )  GEOMETRIC_REPRESENTATION_ITEM ( )  RATIONAL_B_SPLINE_CURVE ( ( 0.9330127018922195203, 0.9330127018922190762, 1.000000000000000000, 0.8660254037844388186, 1.000000000000000000, 0.8660254037844388186, 1.000000000000000000, 0.9330127018922189652, 0.9330127018922194093 ) ) 
 REPRESENTATION_ITEM ( '' )  );
#3398=VECTOR ( 'NONE', #15561, 1000.000000000000000 ) ;
#3399=CARTESIAN_POINT ( 'NONE',  ( -5.999999999999968026, -1.607695154586722186, -152.8466878364870070 ) ) ;
#3400=CARTESIAN_POINT ( 'NONE',  ( 0.000000000000000000, 0.000000000000000000, 0.000000000000000000 ) ) ;
#3401=CARTESIAN_POINT ( 'NONE',  ( 3.464101615137757051, -5.999999999999979572, -93.91367513459479710 ) ) ;
#3403=CARTESIAN_POINT ( 'NONE',  ( -3.175426480542816066, 5.499999999999865885, -134.8750000000000284 ) ) ;
#3405=CARTESIAN_POINT ( 'NONE',  ( -7.216878364870328078, 0.000000000000000000, -148.5580127018922667 ) ) ;
#3406=DIRECTION ( 'NONE',  ( 1.000000000000000000, -5.551115123125773458E-17, -1.260129944081490338E-35 ) ) ;
#3407=CARTESIAN_POINT ( 'NONE',  ( 4.763139720814407951, -2.749999999999988454, -62.00000000000000000 ) ) ;
#3408=CARTESIAN_POINT ( 'NONE',  ( 4.763139720814407951, -2.749999999999988454, -56.00000000000004974 ) ) ;
#3413=CARTESIAN_POINT ( 'NONE',  ( 6.000000000000000888, 1.743066579297358182E-13, -98.16367513459481131 ) ) ;
#3414=ORIENTED_EDGE ( 'NONE', *, *, #1861, .F. ) ;
#3418=CARTESIAN_POINT ( 'NONE',  ( 0.000000000000000000, 5.499999999999991118, -147.0000000000000284 ) ) ;
#3421=CARTESIAN_POINT ( 'NONE',  ( 5.412658773652739619, 3.124999999999988898, -151.3169872981078186 ) ) ;
#3423=CARTESIAN_POINT ( 'NONE',  ( -3.175426480542816510, 5.499999999999865885, -80.87500000000002842 ) ) ;
#3424=CARTESIAN_POINT ( 'NONE',  ( 7.216878364870455975, -6.409875621278545621E-14, -93.80801270189219565 ) ) ;
#3432=CARTESIAN_POINT ( 'NONE',  ( -3.175426480542816066, -5.500000000000057732, -152.3749999999999716 ) ) ;
#3433=LINE ( 'NONE', #19739, #6166 ) ;
#3434=CARTESIAN_POINT ( 'NONE',  ( 4.763139720814407951, -2.749999999999988454, -146.0000000000000284 ) ) ;
#3436=CARTESIAN_POINT ( 'NONE',  ( 4.763139720814407951, -2.749999999999988454, -96.50000000000002842 ) ) ;
#3437=CARTESIAN_POINT ( 'NONE',  ( -3.175426480542816510, 5.499999999999865885, -77.87500000000001421 ) ) ;
#3440=CYLINDRICAL_SURFACE ( 'NONE', #16706, 6.000000000000000888 ) ;
#3442=FACE_OUTER_BOUND ( 'NONE', #24095, .T. ) ;
#3445=DIRECTION ( 'NONE',  ( -7.147005652999508048E-36, 5.642372883946980038E-36, 1.000000000000000000 ) ) ;
#3455=ORIENTED_EDGE ( 'NONE', *, *, #271, .F. ) ;
#3457=CARTESIAN_POINT ( 'NONE',  ( 6.350852961086080661, -9.614813431917819062E-14, -103.8750000000000000 ) ) ;
#3458=CARTESIAN_POINT ( 'NONE',  ( -5.196152422706573404, -3.000000000000002665, -89.78867513459488237 ) ) ;
#3459=CARTESIAN_POINT ( 'NONE',  ( -5.412658773652684552, -3.125000000000099920, -115.4330127018922099 ) ) ;
#3460=ORIENTED_EDGE ( 'NONE', *, *, #8067, .F. ) ;
#3461=CARTESIAN_POINT ( 'NONE',  ( 0.000000000000000000, 0.000000000000000000, 0.000000000000000000 ) ) ;
#3464=CARTESIAN_POINT ( 'NONE',  ( 2.775557561562891351E-14, 6.250000000000033751, -52.93301270189220986 ) ) ;
#3466=CARTESIAN_POINT ( 'NONE',  ( 5.999999999999974243, 1.607695154586759934, -117.5966878364870354 ) ) ;
#3469=CARTESIAN_POINT ( 'NONE',  ( -5.999999999999963585, 8.134310703387671600E-14, -135.8363248654052597 ) ) ;
#3471=CARTESIAN_POINT ( 'NONE',  ( -3.175426480542816510, -5.500000000000057732, -167.3750000000000568 ) ) ;
#3473=CARTESIAN_POINT ( 'NONE',  ( -5.999999999999919176, 1.607695154586804565, -107.4033121635130072 ) ) ;
#3474=CARTESIAN_POINT ( 'NONE',  ( 5.412658773652739619, 3.124999999999988898, -170.1830127018922383 ) ) ;
#3476=VECTOR ( 'NONE', #12338, 1000.000000000000000 ) ;
#3477=CARTESIAN_POINT ( 'NONE',  ( 6.350852961086080661, -9.614813431917819062E-14, -117.3750000000000000 ) ) ;
#3478=CARTESIAN_POINT ( 'NONE',  ( 6.000000000000000888, -3.330669073875464691E-16, -7.560779664488942560E-35 ) ) ;
#3479=CARTESIAN_POINT ( 'NONE',  ( -2.775557561562891351E-14, -5.500000000000115463, -107.2500000000000142 ) ) ;
#3482=CARTESIAN_POINT ( 'NONE',  ( -3.464101615137757051, -5.999999999999979572, -84.58632486540520290 ) ) ;
#3489=CARTESIAN_POINT ( 'NONE',  ( 6.000000000000000888, 1.743066579297358182E-13, -71.16367513459481131 ) ) ;
#3490=DIRECTION ( 'NONE',  ( 1.000000000000000000, -5.551115123125774074E-17, -1.260129944081490070E-35 ) ) ;
#3491=VERTEX_POINT ( 'NONE', #19901 ) ;
#3492=CARTESIAN_POINT ( 'NONE',  ( -4.763139720814407951, 2.749999999999946709, -161.7500000000000568 ) ) ;
#3493=AXIS2_PLACEMENT_3D ( 'NONE', #16183, #20439, #18161 ) ;
#3495=CARTESIAN_POINT ( 'NONE',  ( -5.412658773652739619, 3.124999999999975131, -78.81698729810781856 ) ) ;
#3496=CARTESIAN_POINT ( 'NONE',  ( -5.196152422706573404, -3.000000000000002665, -97.28867513459482552 ) ) ;
#3497=ORIENTED_EDGE ( 'NONE', *, *, #20101, .T. ) ;
#3498=CARTESIAN_POINT ( 'NONE',  ( -5.999999999999963585, -1.487416814333745711E-14, -143.9136751345948255 ) ) ;
#3499=VERTEX_POINT ( 'NONE', #28945 ) ;
#3503=CARTESIAN_POINT ( 'NONE',  ( 2.775557561562891351E-14, -6.250000000000061284, -139.1830127018922667 ) ) ;
#3506=CARTESIAN_POINT ( 'NONE',  ( 3.608439182435180470, -6.249999999999997335, -124.6919872981078043 ) ) ;
#3508=CARTESIAN_POINT ( 'NONE',  ( -6.350852961085760029, -1.281975124255709124E-13, -173.6250000000000284 ) ) ;
#3510=ORIENTED_EDGE ( 'NONE', *, *, #21687, .T. ) ;
#3512=CARTESIAN_POINT ( 'NONE',  ( -3.464101615137725076, 5.999999999999979572, -135.1636751345948539 ) ) ;
#3513=CARTESIAN_POINT ( 'NONE',  ( 6.000000000000000888, -1.859271017917181981E-14, -172.5863248654052029 ) ) ;
#3514=DIRECTION ( 'NONE',  ( -7.147005652999508048E-36, 5.642372883946980038E-36, 1.000000000000000000 ) ) ;
#3516=CARTESIAN_POINT ( 'NONE',  ( 6.000000000000000888, 1.743066579297358182E-13, -107.1636751345948539 ) ) ;
#3518=CARTESIAN_POINT ( 'NONE',  ( 5.412658773652712085, -3.125000000000086153, -70.56698729810784698 ) ) ;
#3521=CARTESIAN_POINT ( 'NONE',  ( -5.196152422706601826, 2.999999999999975131, -127.5386751345948255 ) ) ;
#3522=CARTESIAN_POINT ( 'NONE',  ( 4.763139720814407951, -2.749999999999988454, -131.0000000000000000 ) ) ;
#3523=FACE_OUTER_BOUND ( 'NONE', #3529, .T. ) ;
#3524=ORIENTED_EDGE ( 'NONE', *, *, #14977, .T. ) ;
#3525=CARTESIAN_POINT ( 'NONE',  ( -5.999999999999944933, 1.607695154586759934, -131.9806624327025872 ) ) ;
#3528=CARTESIAN_POINT ( 'NONE',  ( 5.196152422706629359, -2.999999999999988898, -99.78867513459482552 ) ) ;
#3529=EDGE_LOOP ( 'NONE', ( #21935, #4451, #1512, #24034 ) ) ;
#3531=CARTESIAN_POINT ( 'NONE',  ( 0.000000000000000000, 0.000000000000000000, -43.99152654425658682 ) ) ;
#3532=CARTESIAN_POINT ( 'NONE',  ( -5.412658773652739619, 3.124999999999975131, -93.81698729810783277 ) ) ;
#3539=( BOUNDED_CURVE ( )  B_SPLINE_CURVE ( 2, ( #14600, #18914, #21349, #9368, #9975, #23952, #21508, #2308, #2890 ),
 .UNSPECIFIED., .F., .F. ) 
 B_SPLINE_CURVE_WITH_KNOTS ( ( 3, 2, 2, 2, 3 ),
 ( 0.01388888888888883955, 0.01481481481481483620, 0.01666666666666671848, 0.01851851851851848973, 0.01944444444444448639 ),
 .UNSPECIFIED. ) 
 CURVE ( )  GEOMETRIC_REPRESENTATION_ITEM ( )  RATIONAL_B_SPLINE_CURVE ( ( 0.9330127018922194093, 0.9330127018922154125, 1.000000000000000000, 0.8660254037844388186, 1.000000000000000000, 0.8660254037844388186, 1.000000000000000000, 0.9330127018922154125, 0.9330127018922194093 ) ) 
 REPRESENTATION_ITEM ( '' )  );
#3541=CARTESIAN_POINT ( 'NONE',  ( -3.464101615137725076, 5.999999999999979572, -81.16367513459479710 ) ) ;
#3542=CARTESIAN_POINT ( 'NONE',  ( -6.350852961085760029, -1.281975124255709124E-13, -52.12500000000002132 ) ) ;
#3544=CARTESIAN_POINT ( 'NONE',  ( 0.000000000000000000, 0.000000000000000000, 0.000000000000000000 ) ) ;
#3545=CARTESIAN_POINT ( 'NONE',  ( 3.464101615137852974, 5.999999999999884537, -61.91367513459483263 ) ) ;
#3546=CARTESIAN_POINT ( 'NONE',  ( -7.216878364870328078, 0.000000000000000000, -75.05801270189223828 ) ) ;
#3547=FACE_OUTER_BOUND ( 'NONE', #721, .T. ) ;
#3548=VECTOR ( 'NONE', #26567, 1000.000000000000000 ) ;
#3550=DIRECTION ( 'NONE',  ( -7.147005652999508048E-36, 5.642372883946980038E-36, 1.000000000000000000 ) ) ;
#3551=CARTESIAN_POINT ( 'NONE',  ( 0.000000000000000000, 0.000000000000000000, 0.000000000000000000 ) ) ;
#3552=CARTESIAN_POINT ( 'NONE',  ( 0.000000000000000000, 5.999999999999977796, -79.78867513459486815 ) ) ;
#3553=CYLINDRICAL_SURFACE ( 'NONE', #16780, 6.000000000000000888 ) ;
#3555=CARTESIAN_POINT ( 'NONE',  ( -2.775557561562891351E-14, -5.500000000000115463, -128.2500000000000284 ) ) ;
#3559=CARTESIAN_POINT ( 'NONE',  ( -4.763139720814407951, 2.749999999999946709, -62.75000000000002842 ) ) ;
#3561=CARTESIAN_POINT ( 'NONE',  ( 6.350852961086080661, -9.614813431917819062E-14, -60.37500000000000000 ) ) ;
#3564=CARTESIAN_POINT ( 'NONE',  ( -5.999999999999963585, -1.487416814333745711E-14, -118.4136751345948255 ) ) ;
#3565=ADVANCED_FACE ( 'NONE', ( #28638 ), #7609, .T. ) ;
#3566=CARTESIAN_POINT ( 'NONE',  ( -6.000000000000007105, -1.607695154586655129, -104.8466878364870212 ) ) ;
#3569=VERTEX_POINT ( 'NONE', #24054 ) ;
#3571=DIRECTION ( 'NONE',  ( -7.147005652999508048E-36, 5.642372883946980038E-36, 1.000000000000000000 ) ) ;
#3573=CARTESIAN_POINT ( 'NONE',  ( 3.175426480543072749, -5.500000000000105693, -149.1250000000000284 ) ) ;
#3575=CARTESIAN_POINT ( 'NONE',  ( -7.216878364870328078, 0.000000000000000000, -50.19198729810784698 ) ) ;
#3577=ORIENTED_EDGE ( 'NONE', *, *, #20951, .T. ) ;
#3578=CARTESIAN_POINT ( 'NONE',  ( 5.412658773652712085, -3.125000000000086153, -148.5669872981077901 ) ) ;
#3579=CARTESIAN_POINT ( 'NONE',  ( -6.350852961085760029, -1.281975124255709124E-13, -73.12500000000005684 ) ) ;
#3581=CARTESIAN_POINT ( 'NONE',  ( 3.608439182435180470, -6.249999999999997335, -91.05801270189225249 ) ) ;
#3583=CARTESIAN_POINT ( 'NONE',  ( -1.595708107228580142, -10.89084870836962970, -30.79786109011545392 ) ) ;
#3584=CARTESIAN_POINT ( 'NONE',  ( 3.464101615137757051, -5.999999999999979572, -96.33632486540517448 ) ) ;
#3586=CARTESIAN_POINT ( 'NONE',  ( 6.000000000000000888, 1.743066579297358182E-13, -99.08632486540518869 ) ) ;
#3587=CARTESIAN_POINT ( 'NONE',  ( -2.775557561562891351E-14, -5.500000000000115463, -153.7500000000000568 ) ) ;
#3588=FACE_OUTER_BOUND ( 'NONE', #13778, .T. ) ;
#3589=CARTESIAN_POINT ( 'NONE',  ( -6.350852961085760029, -1.281975124255709124E-13, -149.6250000000000568 ) ) ;
#3592=UNCERTAINTY_MEASURE_WITH_UNIT (LENGTH_MEASURE( 1.000000000000000082E-05 ), #15981, 'distance_accuracy_value', 'NONE');
#3593=CARTESIAN_POINT ( 'NONE',  ( -3.175426480542816066, -5.500000000000057732, -83.37500000000004263 ) ) ;
#3596=CARTESIAN_POINT ( 'NONE',  ( 0.000000000000000000, 5.499999999999991118, -81.00000000000001421 ) ) ;
#3597=CARTESIAN_POINT ( 'NONE',  ( 5.196152422706629359, -2.999999999999988898, -74.28867513459481131 ) ) ;
#3600=CARTESIAN_POINT ( 'NONE',  ( 5.196152422706629359, -2.999999999999988898, -149.2886751345948824 ) ) ;
#3607=CARTESIAN_POINT ( 'NONE',  ( -5.999999999999963585, -1.487416814333745711E-14, -80.33632486540523132 ) ) ;
#3608=CARTESIAN_POINT ( 'NONE',  ( 6.000000000000000888, 1.743066579297358182E-13, -66.66367513459481131 ) ) ;
#3610=ADVANCED_FACE ( 'NONE', ( #22979 ), #13480, .T. ) ;
#3612=CARTESIAN_POINT ( 'NONE',  ( -6.350852961085760029, -1.281975124255709124E-13, -94.12500000000004263 ) ) ;
#3613=CARTESIAN_POINT ( 'NONE',  ( 0.000000000000000000, 0.000000000000000000, 0.000000000000000000 ) ) ;
#3614=CARTESIAN_POINT ( 'NONE',  ( 2.775557561562891351E-14, -6.250000000000061284, -112.1830127018922383 ) ) ;
#3615=EDGE_LOOP ( 'NONE', ( #10910, #25155, #29145, #21063 ) ) ;
#3618=CARTESIAN_POINT ( 'NONE',  ( 3.608439182435180470, 6.249999999999982236, -50.05801270189224539 ) ) ;
#3625=CARTESIAN_POINT ( 'NONE',  ( 4.763139720814407951, 2.750000000000002665, -172.7500000000000284 ) ) ;
#3627=CARTESIAN_POINT ( 'NONE',  ( 5.196152422706629359, -2.999999999999988898, -157.7113248654052313 ) ) ;
#3628=CARTESIAN_POINT ( 'NONE',  ( 2.775557561562891351E-14, -6.250000000000061284, -172.1830127018922383 ) ) ;
#3629=CARTESIAN_POINT ( 'NONE',  ( 3.464101615137852974, 5.999999999999884537, -48.41367513459483263 ) ) ;
#3630=CARTESIAN_POINT ( 'NONE',  ( 4.763139720814407951, -2.749999999999988454, -108.5000000000000426 ) ) ;
#3631=CARTESIAN_POINT ( 'NONE',  ( 0.000000000000000000, 0.000000000000000000, 0.000000000000000000 ) ) ;
#3632=CARTESIAN_POINT ( 'NONE',  ( -4.763139720814407951, -2.750000000000016431, -106.0000000000000426 ) ) ;
#3635=SURFACE_SIDE_STYLE ('',( #4099 ) ) ;
#3636=CARTESIAN_POINT ( 'NONE',  ( 0.000000000000000000, 5.999999999999977796, -145.2113248654052313 ) ) ;
#3638=DIRECTION ( 'NONE',  ( 1.000000000000000000, -5.551115123125773458E-17, -1.260129944081490338E-35 ) ) ;
#3641=EDGE_LOOP ( 'NONE', ( #20645, #16995, #11387, #21182 ) ) ;
#3642=CARTESIAN_POINT ( 'NONE',  ( 3.175426480543072749, 5.499999999999865885, -160.6250000000000284 ) ) ;
#3643=CARTESIAN_POINT ( 'NONE',  ( 5.999999999999949374, 1.607695154586804565, -66.01933756729745539 ) ) ;
#3645=CARTESIAN_POINT ( 'NONE',  ( -3.608439182435052128, -6.250000000000110134, -82.94198729810780435 ) ) ;
#3646=CARTESIAN_POINT ( 'NONE',  ( -3.464101615137757051, -5.999999999999979572, -97.16367513459481131 ) ) ;
#3648=EDGE_CURVE ( 'NONE', #9719, #9700, #9501, .T. ) ;
#3653=CARTESIAN_POINT ( 'NONE',  ( 6.350852961086080661, -9.614813431917819062E-14, -132.3750000000000284 ) ) ;
#3654=CARTESIAN_POINT ( 'NONE',  ( -3.608439182435052128, -6.250000000000110134, -139.3080127018922667 ) ) ;
#3656=CARTESIAN_POINT ( 'NONE',  ( 6.000000000000052403, -1.607695154586662678, -57.15331216351299304 ) ) ;
#3657=CARTESIAN_POINT ( 'NONE',  ( -7.216878364870328078, 0.000000000000000000, -120.6919872981078043 ) ) ;
#3659=CARTESIAN_POINT ( 'NONE',  ( 4.763139720814407951, 2.750000000000002665, -171.2500000000000000 ) ) ;
#3660=ORIENTED_EDGE ( 'NONE', *, *, #19184, .F. ) ;
#3663=CARTESIAN_POINT ( 'NONE',  ( 3.464101615137757051, -5.999999999999979572, -117.3363248654052171 ) ) ;
#3664=VECTOR ( 'NONE', #21183, 1000.000000000000000 ) ;
#3668=CARTESIAN_POINT ( 'NONE',  ( 3.608439182435180470, 6.249999999999982236, -64.19198729810784698 ) ) ;
#3669=CARTESIAN_POINT ( 'NONE',  ( 7.216878364870455975, -6.409875621278545621E-14, -52.44198729810779014 ) ) ;
#3674=CARTESIAN_POINT ( 'NONE',  ( -4.763139720814407951, 2.749999999999946709, -133.2500000000000284 ) ) ;
#3675=CARTESIAN_POINT ( 'NONE',  ( 0.000000000000000000, 5.999999999999977796, -50.71132486540519579 ) ) ;
#3676=ORIENTED_EDGE ( 'NONE', *, *, #30129, .T. ) ;
#3677=CARTESIAN_POINT ( 'NONE',  ( -5.999999999999963585, 8.134310703387671600E-14, -131.9136751345948255 ) ) ;
#3678=AXIS2_PLACEMENT_3D ( 'NONE', #5600, #15002, #22213 ) ;
#3679=EDGE_CURVE ( 'NONE', #26998, #26866, #22364, .T. ) ;
#3680=CARTESIAN_POINT ( 'NONE',  ( 6.000000000000000888, -1.859271017917181981E-14, -120.0863248654052313 ) ) ;
#3681=CARTESIAN_POINT ( 'NONE',  ( -5.999999999999963585, 8.134310703387671600E-14, -129.8363248654052313 ) ) ;
#3682=ADVANCED_FACE ( 'NONE', ( #24948 ), #29571, .T. ) ;
#3683=VERTEX_POINT ( 'NONE', #20056 ) ;
#3685=CARTESIAN_POINT ( 'NONE',  ( -5.412658773652684552, -3.125000000000099920, -113.0669872981078186 ) ) ;
#3687=CIRCLE ( 'NONE', #23822, 2.000000000000003109 ) ;
#3691=ORIENTED_EDGE ( 'NONE', *, *, #21983, .F. ) ;
#3692=FACE_OUTER_BOUND ( 'NONE', #2674, .T. ) ;
#3694=EDGE_LOOP ( 'NONE', ( #5564, #3803, #18937, #9323 ) ) ;
#3697=CARTESIAN_POINT ( 'NONE',  ( -3.175426480542816510, -5.500000000000057732, -50.37500000000001421 ) ) ;
#3699=CARTESIAN_POINT ( 'NONE',  ( -5.999999999999963585, 1.780251999655701777E-13, -51.83632486540522422 ) ) ;
#3700=CARTESIAN_POINT ( 'NONE',  ( -3.464101615137725076, 5.999999999999979572, -61.66367513459484684 ) ) ;
#3701=CARTESIAN_POINT ( 'NONE',  ( -3.608439182435115633, 6.249999999999965361, -78.30801270189225249 ) ) ;
#3704=CARTESIAN_POINT ( 'NONE',  ( -5.999999999999963585, 3.021315404115420679E-15, -178.4136751345947971 ) ) ;
#3709=CARTESIAN_POINT ( 'NONE',  ( 4.763139720814407951, 2.750000000000002665, -133.7500000000000284 ) ) ;
#3710=CARTESIAN_POINT ( 'NONE',  ( 0.000000000000000000, 5.999999999999977796, -68.71132486540520290 ) ) ;
#3711=CARTESIAN_POINT ( 'NONE',  ( -5.412658773652684552, -3.125000000000099920, -146.9330127018922383 ) ) ;
#3713=CARTESIAN_POINT ( 'NONE',  ( 6.000000000000001776, 5.345404176511898156E-15, -178.5863248654052313 ) ) ;
#3714=ORIENTED_EDGE ( 'NONE', *, *, #29804, .F. ) ;
#3715=EDGE_CURVE ( 'NONE', #1086, #15338, #17134, .T. ) ;
#3716=CARTESIAN_POINT ( 'NONE',  ( -4.763139720814407951, 2.749999999999946709, -59.75000000000002842 ) ) ;
#3718=CARTESIAN_POINT ( 'NONE',  ( 5.999999999999949374, 1.607695154586804565, -70.51933756729742697 ) ) ;
#3719=( BOUNDED_CURVE ( )  B_SPLINE_CURVE ( 2, ( #25015, #5812, #22278, #22738, #29317, #8275, #6589, #27919, #29930 ),
 .UNSPECIFIED., .F., .F. ) 
 B_SPLINE_CURVE_WITH_KNOTS ( ( 3, 2, 2, 2, 3 ),
 ( 0.1305555555555555636, 0.1314814814814814770, 0.1333333333333333315, 0.1351851851851851860, 0.1361111111111110994 ),
 .UNSPECIFIED. ) 
 CURVE ( )  GEOMETRIC_REPRESENTATION_ITEM ( )  RATIONAL_B_SPLINE_CURVE ( ( 0.9330127018922194093, 0.9330127018922204085, 1.000000000000000000, 0.8660254037844388186, 1.000000000000000000, 0.8660254037844388186, 1.000000000000000000, 0.9330127018922205195, 0.9330127018922196314 ) ) 
 REPRESENTATION_ITEM ( '' )  );
#3721=CARTESIAN_POINT ( 'NONE',  ( -5.196152422706573404, -3.000000000000002665, -163.2886751345948255 ) ) ;
#3725=CARTESIAN_POINT ( 'NONE',  ( 2.775557561562891351E-14, 5.874999999999977796, -46.28349364905393060 ) ) ;
#3726=( BOUNDED_CURVE ( )  B_SPLINE_CURVE ( 2, ( #17392, #29021, #10313, #17859, #22444, #27177, #7986, #22135, #8454 ),
 .UNSPECIFIED., .F., .T. ) 
 B_SPLINE_CURVE_WITH_KNOTS ( ( 3, 2, 2, 2, 3 ),
 ( 0.2083333333333333703, 0.2092592592592592560, 0.2111111111111111382, 0.2129629629629629095, 0.2138888888888887951 ),
 .UNSPECIFIED. ) 
 CURVE ( )  GEOMETRIC_REPRESENTATION_ITEM ( )  RATIONAL_B_SPLINE_CURVE ( ( 0.9330127018922194093, 0.9330127018922234061, 1.000000000000000000, 0.8660254037844388186, 1.000000000000000000, 0.8660254037844388186, 1.000000000000000000, 0.9330127018922234061, 0.9330127018922194093 ) ) 
 REPRESENTATION_ITEM ( '' )  );
#3731=CARTESIAN_POINT ( 'NONE',  ( 4.763139720814407951, -2.749999999999988454, -144.5000000000000284 ) ) ;
#3736=CARTESIAN_POINT ( 'NONE',  ( 4.763139720814407951, -2.749999999999988454, -71.00000000000001421 ) ) ;
#3738=CARTESIAN_POINT ( 'NONE',  ( 3.608439182435180470, 6.249999999999982236, -93.55801270189226670 ) ) ;
#3740=EDGE_CURVE ( 'NONE', #10931, #10419, #25540, .T. ) ;
#3741=CARTESIAN_POINT ( 'NONE',  ( 0.000000000000000000, -5.999999999999991118, -83.53867513459483973 ) ) ;
#3742=CARTESIAN_POINT ( 'NONE',  ( -3.464101615137757051, -5.999999999999979572, -151.1636751345947971 ) ) ;
#3743=CARTESIAN_POINT ( 'NONE',  ( -5.196152422706601826, 2.999999999999975131, -98.46132486540520290 ) ) ;
#3744=CARTESIAN_POINT ( 'NONE',  ( 0.000000000000000000, -5.999999999999991118, -64.96132486540523132 ) ) ;
#3746=CARTESIAN_POINT ( 'NONE',  ( 0.000000000000000000, 5.499999999999991118, -159.0000000000000284 ) ) ;
#3751=CARTESIAN_POINT ( 'NONE',  ( -3.175426480542816066, 5.499999999999865885, -89.87500000000001421 ) ) ;
#3755=CARTESIAN_POINT ( 'NONE',  ( 0.000000000000000000, 5.499999999999991118, -82.50000000000001421 ) ) ;
#3756=EDGE_CURVE ( 'NONE', #10765, #8441, #14401, .T. ) ;
#3760=CARTESIAN_POINT ( 'NONE',  ( -5.999999999999963585, 1.780251999655701777E-13, -103.4136751345948255 ) ) ;
#3763=CARTESIAN_POINT ( 'NONE',  ( -5.999999999999971578, 1.607695154586715303, -134.4033121635129930 ) ) ;
#3772=CARTESIAN_POINT ( 'NONE',  ( -3.175426480542816510, 5.499999999999865885, -100.3750000000000000 ) ) ;
#3773=CARTESIAN_POINT ( 'NONE',  ( -5.196152422706601826, 2.999999999999975131, -70.53867513459482552 ) ) ;
#3774=CARTESIAN_POINT ( 'NONE',  ( 2.775557561562891351E-14, 6.250000000000033751, -118.9330127018922667 ) ) ;
#3776=CARTESIAN_POINT ( 'NONE',  ( 0.000000000000000000, 5.999999999999977796, -91.78867513459482552 ) ) ;
#3778=EDGE_CURVE ( 'NONE', #29507, #22623, #11684, .T. ) ;
#3780=CARTESIAN_POINT ( 'NONE',  ( -3.608439182435052128, -6.250000000000110134, -55.30801270189220276 ) ) ;
#3784=CARTESIAN_POINT ( 'NONE',  ( -4.763139720814407951, 2.749999999999946709, -172.2500000000000000 ) ) ;
#3788=CARTESIAN_POINT ( 'NONE',  ( 0.000000000000000000, 5.499999999999991118, -110.9999999999999858 ) ) ;
#3791=CARTESIAN_POINT ( 'NONE',  ( -4.763139720814407951, -2.750000000000016431, -107.5000000000000426 ) ) ;
#3793=VERTEX_POINT ( 'NONE', #15124 ) ;
#3798=CARTESIAN_POINT ( 'NONE',  ( -5.999999999999963585, -1.487416814333745711E-14, -134.3363248654052313 ) ) ;
#3801=CARTESIAN_POINT ( 'NONE',  ( 3.608439182435180470, 6.249999999999982236, -79.19198729810786119 ) ) ;
#3802=CARTESIAN_POINT ( 'NONE',  ( 3.464101615137757051, -5.999999999999979572, -102.9136751345948255 ) ) ;
#3803=ORIENTED_EDGE ( 'NONE', *, *, #23220, .F. ) ;
#3804=CARTESIAN_POINT ( 'NONE',  ( -5.196152422706573404, -3.000000000000002665, -75.71132486540521711 ) ) ;
#3807=CARTESIAN_POINT ( 'NONE',  ( 4.763139720814407951, 2.750000000000002665, -124.7500000000000284 ) ) ;
#3808=( BOUNDED_CURVE ( )  B_SPLINE_CURVE ( 2, ( #15377, #8739, #8257, #5957, #27294, #3802, #24704, #1052, #15847 ),
 .UNSPECIFIED., .F., .F. ) 
 B_SPLINE_CURVE_WITH_KNOTS ( ( 3, 2, 2, 2, 3 ),
 ( 0.5805555555555554914, 0.5814814814814814881, 0.5833333333333333703, 0.5851851851851851416, 0.5861111111111111382 ),
 .UNSPECIFIED. ) 
 CURVE ( )  GEOMETRIC_REPRESENTATION_ITEM ( )  RATIONAL_B_SPLINE_CURVE ( ( 0.9330127018922194093, 0.9330127018922154125, 1.000000000000000000, 0.8660254037844388186, 1.000000000000000000, 0.8660254037844388186, 1.000000000000000000, 0.9330127018922154125, 0.9330127018922194093 ) ) 
 REPRESENTATION_ITEM ( '' )  );
#3809=CARTESIAN_POINT ( 'NONE',  ( 2.775557561562891351E-14, -6.250000000000061284, -142.1830127018922667 ) ) ;
#3812=CARTESIAN_POINT ( 'NONE',  ( 2.775557561562891351E-14, 6.250000000000033751, -122.5669872981078328 ) ) ;
#3815=CARTESIAN_POINT ( 'NONE',  ( 3.175426480543072749, 5.499999999999865885, -169.6250000000000000 ) ) ;
#3818=ORIENTED_EDGE ( 'NONE', *, *, #23282, .T. ) ;
#3821=CARTESIAN_POINT ( 'NONE',  ( -5.999999999999971578, 1.607695154586715303, -170.9806624327026157 ) ) ;
#3824=CARTESIAN_POINT ( 'NONE',  ( -7.216878364870328078, 0.000000000000000000, -68.19198729810780435 ) ) ;
#3825=CARTESIAN_POINT ( 'NONE',  ( -5.412658773652684552, -3.125000000000099920, -56.06698729810782567 ) ) ;
#3827=CARTESIAN_POINT ( 'NONE',  ( -2.775557561562891351E-14, -5.500000000000115463, -48.75000000000001421 ) ) ;
#3829=EDGE_CURVE ( 'NONE', #14180, #19519, #58, .T. ) ;
#3830=CARTESIAN_POINT ( 'NONE',  ( 4.763139720814407951, 2.750000000000002665, -130.7500000000000284 ) ) ;
#3832=CARTESIAN_POINT ( 'NONE',  ( 5.999999999999974243, 1.607695154586759934, -138.5966878364870354 ) ) ;
#3837=CARTESIAN_POINT ( 'NONE',  ( -3.464101615137725076, 5.999999999999979572, -97.08632486540518869 ) ) ;
#3839=ORIENTED_EDGE ( 'NONE', *, *, #24312, .T. ) ;
#3841=CARTESIAN_POINT ( 'NONE',  ( 6.000000000000000888, -1.607695154586752384, -109.6533121635129930 ) ) ;
#3844=CARTESIAN_POINT ( 'NONE',  ( 0.000000000000000000, 0.000000000000000000, 0.000000000000000000 ) ) ;
#3850=EDGE_CURVE ( 'NONE', #25854, #8489, #671, .T. ) ;
#3853=CARTESIAN_POINT ( 'NONE',  ( 6.000000000000000888, -1.859271017917181981E-14, -166.5863248654052029 ) ) ;
#3854=CARTESIAN_POINT ( 'NONE',  ( 7.216878364870455975, -6.409875621278545621E-14, -71.30801270189220986 ) ) ;
#3856=CARTESIAN_POINT ( 'NONE',  ( 0.000000000000000000, 0.000000000000000000, 0.000000000000000000 ) ) ;
#3858=( BOUNDED_CURVE ( )  B_SPLINE_CURVE ( 2, ( #15504, #17641, #15660, #26964, #3776, #3921, #13350, #4080, #5925 ),
 .UNSPECIFIED., .F., .F. ) 
 B_SPLINE_CURVE_WITH_KNOTS ( ( 3, 2, 2, 2, 3 ),
 ( 0.6638888888888889728, 0.6648148148148148584, 0.6666666666666666297, 0.6685185185185185119, 0.6694444444444443976 ),
 .UNSPECIFIED. ) 
 CURVE ( )  GEOMETRIC_REPRESENTATION_ITEM ( )  RATIONAL_B_SPLINE_CURVE ( ( 0.9330127018922194093, 0.9330127018922234061, 1.000000000000000000, 0.8660254037844388186, 1.000000000000000000, 0.8660254037844388186, 1.000000000000000000, 0.9330127018922234061, 0.9330127018922194093 ) ) 
 REPRESENTATION_ITEM ( '' )  );
#3860=CARTESIAN_POINT ( 'NONE',  ( -3.175426480542816066, -5.500000000000057732, -135.8750000000000284 ) ) ;
#3862=CARTESIAN_POINT ( 'NONE',  ( 2.775557561562891351E-14, -6.250000000000061284, -148.1830127018922667 ) ) ;
#3863=CARTESIAN_POINT ( 'NONE',  ( -6.000000000000000888, 1.067854986875958443E-15, 7.560779664488942560E-35 ) ) ;
#3866=CARTESIAN_POINT ( 'NONE',  ( -4.763139720814407951, -2.750000000000016431, -65.50000000000000000 ) ) ;
#3867=FACE_OUTER_BOUND ( 'NONE', #24961, .T. ) ;
#3869=CARTESIAN_POINT ( 'NONE',  ( -5.999999999999962697, 3.323446944526963891E-14, -163.4136751345948539 ) ) ;
#3874=FACE_OUTER_BOUND ( 'NONE', #1463, .T. ) ;
#3877=CARTESIAN_POINT ( 'NONE',  ( 6.000000000000000888, 7.762456499804234384E-14, -121.5863248654052455 ) ) ;
#3879=CARTESIAN_POINT ( 'NONE',  ( -3.175426480542816510, -5.500000000000057732, -147.8750000000000284 ) ) ;
#3881=VERTEX_POINT ( 'NONE', #14675 ) ;
#3882=CARTESIAN_POINT ( 'NONE',  ( -2.775557561562891351E-14, -5.500000000000115463, -69.75000000000002842 ) ) ;
#3884=EDGE_CURVE ( 'NONE', #22716, #18315, #14027, .T. ) ;
#3885=CARTESIAN_POINT ( 'NONE',  ( 5.412658773652712085, -3.125000000000086153, -93.93301270189225249 ) ) ;
#3886=CARTESIAN_POINT ( 'NONE',  ( -5.959413262067409178, -9.246315551493122342, -24.19612909832621384 ) ) ;
#3890=CARTESIAN_POINT ( 'NONE',  ( -3.464101615137757051, -5.999999999999979572, -65.08632486540523132 ) ) ;
#3892=( BOUNDED_CURVE ( )  B_SPLINE_CURVE ( 2, ( #27737, #25439, #4403, #13671, #9331, #9174, #27431, #18416, #16289 ),
 .UNSPECIFIED., .F., .T. ) 
 B_SPLINE_CURVE_WITH_KNOTS ( ( 3, 2, 2, 2, 3 ),
 ( 0.1138888888888888867, 0.1148148148148148140, 0.1166666666666666685, 0.1185185185185185230, 0.1194444444444444503 ),
 .UNSPECIFIED. ) 
 CURVE ( )  GEOMETRIC_REPRESENTATION_ITEM ( )  RATIONAL_B_SPLINE_CURVE ( ( 0.9330127018922194093, 0.9330127018922194093, 1.000000000000000000, 0.8660254037844388186, 1.000000000000000000, 0.8660254037844388186, 1.000000000000000000, 0.9330127018922189652, 0.9330127018922194093 ) ) 
 REPRESENTATION_ITEM ( '' )  );
#3893=CARTESIAN_POINT ( 'NONE',  ( -4.763139720814407951, -2.750000000000016431, -154.0000000000000284 ) ) ;
#3894=DIRECTION ( 'NONE',  ( 1.000000000000000000, -5.551115123125773458E-17, -1.260129944081490338E-35 ) ) ;
#3895=CARTESIAN_POINT ( 'NONE',  ( -0.5896198263027827569, 5.540201351793362150, -180.0000000000000853 ) ) ;
#3897=CARTESIAN_POINT ( 'NONE',  ( -2.775557561562891351E-14, -5.500000000000115463, -84.74999999999998579 ) ) ;
#3898=CARTESIAN_POINT ( 'NONE',  ( 0.000000000000000000, -5.999999999999991118, -140.5386751345948255 ) ) ;
#3899=FACE_OUTER_BOUND ( 'NONE', #20079, .T. ) ;
#3900=CARTESIAN_POINT ( 'NONE',  ( 3.175426480543072749, -5.500000000000105693, -71.12500000000004263 ) ) ;
#3903=DIRECTION ( 'NONE',  ( 1.000000000000000000, -5.551115123125773458E-17, -1.260129944081490338E-35 ) ) ;
#3907=CARTESIAN_POINT ( 'NONE',  ( 0.000000000000000000, 5.999999999999977796, -55.21132486540525264 ) ) ;
#3915=ORIENTED_EDGE ( 'NONE', *, *, #12634, .F. ) ;
#3916=CARTESIAN_POINT ( 'NONE',  ( -2.775557561562891351E-14, -5.500000000000115463, -93.75000000000000000 ) ) ;
#3917=CARTESIAN_POINT ( 'NONE',  ( -5.999999999999963585, 1.780251999655701777E-13, -70.41367513459482552 ) ) ;
#3918=EDGE_CURVE ( 'NONE', #4112, #15998, #11871, .T. ) ;
#3919=CARTESIAN_POINT ( 'NONE',  ( -5.412658773652739619, 3.124999999999975131, -114.1830127018922383 ) ) ;
#3920=ORIENTED_EDGE ( 'NONE', *, *, #11751, .F. ) ;
#3921=CARTESIAN_POINT ( 'NONE',  ( -3.464101615137725076, 5.999999999999979572, -91.66367513459485394 ) ) ;
#3922=FACE_OUTER_BOUND ( 'NONE', #17373, .T. ) ;
#3923=CARTESIAN_POINT ( 'NONE',  ( 5.196152422706629359, -2.999999999999988898, -143.2886751345948255 ) ) ;
#3924=AXIS2_PLACEMENT_3D ( 'NONE', #28870, #1078, #24421 ) ;
#3925=CARTESIAN_POINT ( 'NONE',  ( -7.216878364870328078, 0.000000000000000000, -51.05801270189225249 ) ) ;
#3928=CARTESIAN_POINT ( 'NONE',  ( -3.464101615137757051, -5.999999999999979572, -62.08632486540521711 ) ) ;
#3929=CARTESIAN_POINT ( 'NONE',  ( -4.763139720814407951, -2.750000000000016431, -161.5000000000000284 ) ) ;
#3931=CARTESIAN_POINT ( 'NONE',  ( 0.000000000000000000, 5.999999999999977796, -107.7113248654052455 ) ) ;
#3933=CARTESIAN_POINT ( 'NONE',  ( -4.763139720814407951, -2.750000000000016431, -94.00000000000002842 ) ) ;
#3934=CARTESIAN_POINT ( 'NONE',  ( -5.196152422706601826, 2.999999999999975131, -151.5386751345948539 ) ) ;
#3935=FILL_AREA_STYLE ('',( #10588 ) ) ;
#3936=CARTESIAN_POINT ( 'NONE',  ( -5.196152422706573404, -3.000000000000002665, -82.28867513459481131 ) ) ;
#3944=CARTESIAN_POINT ( 'NONE',  ( 4.763139720814407951, 2.750000000000002665, -162.2500000000000000 ) ) ;
#3945=CARTESIAN_POINT ( 'NONE',  ( 6.000000000000000888, -1.859271017917181981E-14, -169.5863248654052029 ) ) ;
#3947=CONICAL_SURFACE ( 'NONE', #4922, 1000.000000000000682, 0.7853981633974479459 ) ;
#3949=CARTESIAN_POINT ( 'NONE',  ( -5.412658773652684552, -3.125000000000099920, -87.56698729810786119 ) ) ;
#3952=CARTESIAN_POINT ( 'NONE',  ( -2.691259848637789442, 10.67213569177517840, -30.37695071776534661 ) ) ;
#3954=ORIENTED_EDGE ( 'NONE', *, *, #21438, .F. ) ;
#3957=CARTESIAN_POINT ( 'NONE',  ( 3.175426480543072749, 5.499999999999865885, -123.1250000000000426 ) ) ;
#3958=EDGE_CURVE ( 'NONE', #28373, #16384, #1205, .T. ) ;
#3959=VERTEX_POINT ( 'NONE', #24919 ) ;
#3961=CARTESIAN_POINT ( 'NONE',  ( 3.608439182435180470, 6.249999999999982236, -121.1919872981077901 ) ) ;
#3962=CARTESIAN_POINT ( 'NONE',  ( -5.412658773652684552, -3.125000000000099920, -174.5669872981078186 ) ) ;
#3963=CARTESIAN_POINT ( 'NONE',  ( 3.175426480543072749, 5.499999999999865885, -172.6250000000000000 ) ) ;
#3966=AXIS2_PLACEMENT_3D ( 'NONE', #3243, #946, #17730 ) ;
#3967=VERTEX_POINT ( 'NONE', #15606 ) ;
#3970=CARTESIAN_POINT ( 'NONE',  ( 5.196152422706629359, -2.999999999999988898, -117.2113248654052029 ) ) ;
#3975=CARTESIAN_POINT ( 'NONE',  ( -3.608439182435115633, 6.249999999999965361, -69.94198729810781856 ) ) ;
#3976=CARTESIAN_POINT ( 'NONE',  ( 2.775557561562891351E-14, -6.250000000000061284, -54.31698729810785409 ) ) ;
#3977=CARTESIAN_POINT ( 'NONE',  ( -5.999999999999919176, 1.607695154586804565, -110.4033121635129788 ) ) ;
#3978=CARTESIAN_POINT ( 'NONE',  ( 6.350852961086080661, -9.614813431917819062E-14, -46.87500000000000000 ) ) ;
#3980=CARTESIAN_POINT ( 'NONE',  ( 0.000000000000000000, -5.999999999999991118, -153.4613248654052029 ) ) ;
#3981=CARTESIAN_POINT ( 'NONE',  ( -4.763139720814407951, 2.749999999999946709, -131.7500000000000284 ) ) ;
#3984=CARTESIAN_POINT ( 'NONE',  ( 3.464101615137852974, 5.999999999999884537, -157.9136751345947971 ) ) ;
#3985=DIRECTION ( 'NONE',  ( -7.147005652999508048E-36, 5.642372883946980038E-36, 1.000000000000000000 ) ) ;
#3986=FACE_OUTER_BOUND ( 'NONE', #3641, .T. ) ;
#3987=( BOUNDED_CURVE ( )  B_SPLINE_CURVE ( 2, ( #21009, #14130, #29888, #95, #16426, #18864, #28037, #2261, #11351 ),
 .UNSPECIFIED., .F., .F. ) 
 B_SPLINE_CURVE_WITH_KNOTS ( ( 3, 2, 2, 2, 3 ),
 ( 0.1250000000000000000, 0.1259259259259258856, 0.1277777777777777679, 0.1296296296296296502, 0.1305555555555556468 ),
 .UNSPECIFIED. ) 
 CURVE ( )  GEOMETRIC_REPRESENTATION_ITEM ( )  RATIONAL_B_SPLINE_CURVE ( ( 0.9330127018922194093, 0.9330127018922194093, 1.000000000000000000, 0.8660254037844388186, 1.000000000000000000, 0.8660254037844388186, 1.000000000000000000, 0.9330127018922154125, 0.9330127018922194093 ) ) 
 REPRESENTATION_ITEM ( '' )  );
#3994=CARTESIAN_POINT ( 'NONE',  ( -5.412658773652684552, -3.125000000000099920, -114.5669872981078186 ) ) ;
#3995=CIRCLE ( 'NONE', #17759, 11.00000000000001599 ) ;
#3997=( BOUNDED_CURVE ( )  B_SPLINE_CURVE ( 2, ( #2650, #24003, #19414, #345, #18976, #9586, #14521, #12226, #28145 ),
 .UNSPECIFIED., .F., .T. ) 
 B_SPLINE_CURVE_WITH_KNOTS ( ( 3, 2, 2, 2, 3 ),
 ( 0.4861111111111111049, 0.4870370370370370461, 0.4888888888888888729, 0.4907407407407407551, 0.4916666666666666408 ),
 .UNSPECIFIED. ) 
 CURVE ( )  GEOMETRIC_REPRESENTATION_ITEM ( )  RATIONAL_B_SPLINE_CURVE ( ( 0.9330127018922194093, 0.9330127018922194093, 1.000000000000000000, 0.8660254037844388186, 1.000000000000000000, 0.8660254037844388186, 1.000000000000000000, 0.9330127018922214077, 0.9330127018922194093 ) ) 
 REPRESENTATION_ITEM ( '' )  );
#3999=ORIENTED_EDGE ( 'NONE', *, *, #21874, .T. ) ;
#4003=EDGE_CURVE ( 'NONE', #17334, #2061, #10672, .T. ) ;
#4008=CARTESIAN_POINT ( 'NONE',  ( -2.775557561562891351E-14, -5.500000000000115463, -51.75000000000002132 ) ) ;
#4012=CARTESIAN_POINT ( 'NONE',  ( 3.608439182435180470, 6.249999999999982236, -69.55801270189228092 ) ) ;
#4015=FACE_OUTER_BOUND ( 'NONE', #28181, .T. ) ;
#4018=CARTESIAN_POINT ( 'NONE',  ( -3.175426480542816066, -5.500000000000057732, -131.3750000000000284 ) ) ;
#4019=CARTESIAN_POINT ( 'NONE',  ( 3.608439182435180470, 6.249999999999982236, -143.0580127018922667 ) ) ;
#4022=CARTESIAN_POINT ( 'NONE',  ( -3.175426480542816066, -5.500000000000057732, -63.87500000000001421 ) ) ;
#4023=DIRECTION ( 'NONE',  ( -7.147005652999508048E-36, 5.642372883946980038E-36, 1.000000000000000000 ) ) ;
#4024=CARTESIAN_POINT ( 'NONE',  ( 6.000000000000000888, 1.743066579297358182E-13, -76.58632486540521711 ) ) ;
#4038=CARTESIAN_POINT ( 'NONE',  ( 3.175426480543072749, 5.499999999999865885, -144.1250000000000000 ) ) ;
#4041=CARTESIAN_POINT ( 'NONE',  ( -2.775557561562891351E-14, -5.500000000000115463, -75.75000000000004263 ) ) ;
#4042=CARTESIAN_POINT ( 'NONE',  ( -6.000000000000000888, 1.067854986875958443E-15, 7.560779664488942560E-35 ) ) ;
#4043=CARTESIAN_POINT ( 'NONE',  ( -5.412658773652684552, -3.125000000000099920, -88.43301270189223828 ) ) ;
#4045=CARTESIAN_POINT ( 'NONE',  ( -0.4044047236350920005, -11.00000000000001243, -31.00000000000003908 ) ) ;
#4046=CARTESIAN_POINT ( 'NONE',  ( -6.000000000000007105, -1.607695154586655129, -83.84668783648703538 ) ) ;
#4047=DIRECTION ( 'NONE',  ( -7.147005652999508048E-36, 5.642372883946980038E-36, 1.000000000000000000 ) ) ;
#4050=CARTESIAN_POINT ( 'NONE',  ( -4.763139720814407951, -2.750000000000016431, -158.5000000000000284 ) ) ;
#4052=LINE ( 'NONE', #30019, #17923 ) ;
#4053=CARTESIAN_POINT ( 'NONE',  ( 0.000000000000000000, 5.499999999999991118, -88.50000000000002842 ) ) ;
#4056=CARTESIAN_POINT ( 'NONE',  ( -3.175426480542816510, 5.499999999999865885, -70.37500000000004263 ) ) ;
#4057=AXIS2_PLACEMENT_3D ( 'NONE', #27772, #11396, #11554 ) ;
#4059=CARTESIAN_POINT ( 'NONE',  ( 5.196152422706629359, 3.000000000000002665, -164.9613248654052029 ) ) ;
#4060=CARTESIAN_POINT ( 'NONE',  ( 6.000000000000000888, -3.330669073875464691E-16, -7.560779664488942560E-35 ) ) ;
#4065=FACE_OUTER_BOUND ( 'NONE', #11416, .T. ) ;
#4067=EDGE_CURVE ( 'NONE', #15286, #18931, #28652, .T. ) ;
#4071=DIRECTION ( 'NONE',  ( 1.000000000000000000, -5.551115123125774690E-17, 0.000000000000000000 ) ) ;
#4073=CARTESIAN_POINT ( 'NONE',  ( -6.000000000000023093, 1.607695154586625819, -156.9033121635130215 ) ) ;
#4074=VERTEX_POINT ( 'NONE', #7100 ) ;
#4076=CARTESIAN_POINT ( 'NONE',  ( 3.175426480543072749, -5.500000000000105693, -96.62500000000004263 ) ) ;
#4077=CARTESIAN_POINT ( 'NONE',  ( 6.000000000000000888, -3.330669073875464691E-16, -7.560779664488942560E-35 ) ) ;
#4078=( BOUNDED_CURVE ( )  B_SPLINE_CURVE ( 2, ( #3607, #12429, #12581, #21923, #15170, #14864, #1311, #8218, #26503 ),
 .UNSPECIFIED., .F., .T. ) 
 B_SPLINE_CURVE_WITH_KNOTS ( ( 3, 2, 2, 2, 3 ),
 ( 0.2527777777777777679, 0.2537037037037036535, 0.2555555555555555358, 0.2574074074074074181, 0.2583333333333333037 ),
 .UNSPECIFIED. ) 
 CURVE ( )  GEOMETRIC_REPRESENTATION_ITEM ( )  RATIONAL_B_SPLINE_CURVE ( ( 0.9330127018922194093, 0.9330127018922194093, 1.000000000000000000, 0.8660254037844388186, 1.000000000000000000, 0.8660254037844388186, 1.000000000000000000, 0.9330127018922234061, 0.9330127018922194093 ) ) 
 REPRESENTATION_ITEM ( '' )  );
#4079=CARTESIAN_POINT ( 'NONE',  ( 3.608439182435180470, -6.249999999999997335, -106.0580127018922525 ) ) ;
#4080=CARTESIAN_POINT ( 'NONE',  ( -5.999999999999919176, 1.607695154586804565, -91.48066243270262987 ) ) ;
#4081=CARTESIAN_POINT ( 'NONE',  ( 0.000000000000000000, 0.000000000000000000, 0.000000000000000000 ) ) ;
#4084=CARTESIAN_POINT ( 'NONE',  ( 3.175426480543072749, -5.500000000000105693, -164.1249999999999716 ) ) ;
#4085=CARTESIAN_POINT ( 'NONE',  ( 2.775557561562891351E-14, 6.250000000000033751, -51.43301270189226670 ) ) ;
#4088=CARTESIAN_POINT ( 'NONE',  ( -9.999999999999998224, 1.868746227032927028E-15, -44.99152654425658682 ) ) ;
#4090=CARTESIAN_POINT ( 'NONE',  ( -5.196152422706573404, -3.000000000000002665, -62.21132486540520290 ) ) ;
#4091=CARTESIAN_POINT ( 'NONE',  ( -3.175426480542816510, -5.500000000000057732, -159.8750000000000284 ) ) ;
#4093=DIRECTION ( 'NONE',  ( -7.147005652999508048E-36, 5.642372883946980038E-36, 1.000000000000000000 ) ) ;
#4094=CARTESIAN_POINT ( 'NONE',  ( -3.175426480542816066, 5.499999999999865885, -110.8750000000000426 ) ) ;
#4097=CARTESIAN_POINT ( 'NONE',  ( -3.175426480542816510, -5.500000000000057732, -93.87500000000002842 ) ) ;
#4099=SURFACE_STYLE_FILL_AREA ( #3935 ) ;
#4101=ORIENTED_EDGE ( 'NONE', *, *, #17077, .F. ) ;
#4106=EDGE_CURVE ( 'NONE', #4711, #16677, #8966, .T. ) ;
#4108=CARTESIAN_POINT ( 'NONE',  ( 2.775557561562891351E-14, 6.250000000000033751, -89.56698729810786119 ) ) ;
#4110=ORIENTED_EDGE ( 'NONE', *, *, #3068, .T. ) ;
#4112=VERTEX_POINT ( 'NONE', #27672 ) ;
#4115=CARTESIAN_POINT ( 'NONE',  ( -4.763139720814407951, -2.750000000000016431, -118.0000000000000000 ) ) ;
#4117=CARTESIAN_POINT ( 'NONE',  ( -3.608439182435115633, 6.249999999999965361, -141.3080127018922099 ) ) ;
#4119=CARTESIAN_POINT ( 'NONE',  ( 6.000000000000000888, 1.743066579297358182E-13, -57.66367513459481842 ) ) ;
#4120=CARTESIAN_POINT ( 'NONE',  ( 5.412658773652739619, 3.124999999999988898, -124.3169872981078043 ) ) ;
#4121=CARTESIAN_POINT ( 'NONE',  ( 3.608439182435180470, 6.249999999999982236, -178.1919872981078470 ) ) ;
#4124=VERTEX_POINT ( 'NONE', #25989 ) ;
#4126=CYLINDRICAL_SURFACE ( 'NONE', #5875, 6.000000000000000888 ) ;
#4131=CARTESIAN_POINT ( 'NONE',  ( -7.216878364870328078, 0.000000000000000000, -74.19198729810783277 ) ) ;
#4132=CARTESIAN_POINT ( 'NONE',  ( 3.608439182435180470, -6.249999999999997335, -63.19198729810784698 ) ) ;
#4134=CARTESIAN_POINT ( 'NONE',  ( 6.000000000000000888, -1.859271017917181981E-14, -170.1636751345948539 ) ) ;
#4135=CARTESIAN_POINT ( 'NONE',  ( 4.763139720814407951, 2.750000000000002665, -49.75000000000001421 ) ) ;
#4137=CARTESIAN_POINT ( 'NONE',  ( 5.196152422706629359, -2.999999999999988898, -47.28867513459483973 ) ) ;
#4138=CARTESIAN_POINT ( 'NONE',  ( 6.350852961086080661, -9.614813431917819062E-14, -118.8750000000000142 ) ) ;
#4141=CARTESIAN_POINT ( 'NONE',  ( 3.464101615137757051, -5.999999999999979572, -118.8363248654052171 ) ) ;
#4146=EDGE_CURVE ( 'NONE', #16363, #4876, #13840, .T. ) ;
#4147=ORIENTED_EDGE ( 'NONE', *, *, #4283, .T. ) ;
#4149=DIRECTION ( 'NONE',  ( 1.000000000000000000, -5.551115123125773458E-17, -1.260129944081490338E-35 ) ) ;
#4151=CARTESIAN_POINT ( 'NONE',  ( -3.608439182435115633, 6.249999999999965361, -111.9419872981078186 ) ) ;
#4152=CARTESIAN_POINT ( 'NONE',  ( -3.464101615137757051, -5.999999999999979572, -54.58632486540518158 ) ) ;
#4153=EDGE_LOOP ( 'NONE', ( #23060, #23566, #28693, #23317 ) ) ;
#4154=ORIENTED_EDGE ( 'NONE', *, *, #17380, .T. ) ;
#4157=CARTESIAN_POINT ( 'NONE',  ( 2.775557561562891351E-14, 6.250000000000033751, -148.0669872981078470 ) ) ;
#4158=ORIENTED_EDGE ( 'NONE', *, *, #6293, .F. ) ;
#4159=CARTESIAN_POINT ( 'NONE',  ( -3.464101615137725076, 5.999999999999979572, -151.0863248654051745 ) ) ;
#4161=CARTESIAN_POINT ( 'NONE',  ( 3.464101615137852974, 5.999999999999884537, -120.4136751345947829 ) ) ;
#4163=CARTESIAN_POINT ( 'NONE',  ( 3.608439182435180470, -6.249999999999997335, -68.55801270189226670 ) ) ;
#4167=CARTESIAN_POINT ( 'NONE',  ( 4.325218075994005005E-32, 10.49588505988223375, 3.091235803958481245E-67 ) ) ;
#4168=CARTESIAN_POINT ( 'NONE',  ( 6.000000000000000888, -1.859271017917181981E-14, -146.1636751345948255 ) ) ;
#4169=VECTOR ( 'NONE', #11840, 1000.000000000000000 ) ;
#4170=EDGE_CURVE ( 'NONE', #18931, #137, #25162, .T. ) ;
#4173=( BOUNDED_CURVE ( )  B_SPLINE_CURVE ( 2, ( #6484, #27811, #18639, #9095, #27960, #11117, #29824, #20935, #6784 ),
 .UNSPECIFIED., .F., .F. ) 
 B_SPLINE_CURVE_WITH_KNOTS ( ( 3, 2, 2, 2, 3 ),
 ( 0.1194444444444444503, 0.1203703703703703637, 0.1222222222222222182, 0.1240740740740740727, 0.1249999999999999861 ),
 .UNSPECIFIED. ) 
 CURVE ( )  GEOMETRIC_REPRESENTATION_ITEM ( )  RATIONAL_B_SPLINE_CURVE ( ( 0.9330127018922194093, 0.9330127018922198534, 1.000000000000000000, 0.8660254037844388186, 1.000000000000000000, 0.8660254037844388186, 1.000000000000000000, 0.9330127018922198534, 0.9330127018922194093 ) ) 
 REPRESENTATION_ITEM ( '' )  );
#4174=CARTESIAN_POINT ( 'NONE',  ( -4.763139720814407951, -2.750000000000016431, -121.0000000000000000 ) ) ;
#4175=CYLINDRICAL_SURFACE ( 'NONE', #5805, 6.000000000000000888 ) ;
#4177=DIRECTION ( 'NONE',  ( 1.000000000000000000, -5.551115123125773458E-17, -1.260129944081490338E-35 ) ) ;
#4180=CARTESIAN_POINT ( 'NONE',  ( -3.175426480542816066, -5.500000000000057732, -53.37500000000002842 ) ) ;
#4182=EDGE_CURVE ( 'NONE', #3683, #18704, #23414, .T. ) ;
#4183=CARTESIAN_POINT ( 'NONE',  ( 0.000000000000000000, 0.000000000000000000, 0.000000000000000000 ) ) ;
#4185=EDGE_CURVE ( 'NONE', #26400, #27302, #26507, .T. ) ;
#4186=CARTESIAN_POINT ( 'NONE',  ( 6.000000000000000888, -1.859271017917181981E-14, -171.0863248654052029 ) ) ;
#4193=ORIENTED_EDGE ( 'NONE', *, *, #18370, .T. ) ;
#4194=CARTESIAN_POINT ( 'NONE',  ( -3.175426480542816510, -5.500000000000057732, -137.3750000000000568 ) ) ;
#4196=VERTEX_POINT ( 'NONE', #29139 ) ;
#4197=CARTESIAN_POINT ( 'NONE',  ( 3.175426480543072749, -5.500000000000105693, -75.62500000000000000 ) ) ;
#4200=CARTESIAN_POINT ( 'NONE',  ( -3.031145847945085681, -10.57562584360016800, -30.18173774084352345 ) ) ;
#4203=CARTESIAN_POINT ( 'NONE',  ( -5.999999999999963585, -1.487416814333745711E-14, -106.4136751345948113 ) ) ;
#4207=CARTESIAN_POINT ( 'NONE',  ( 6.350852961086080661, -9.614813431917819062E-14, -151.8749999999999716 ) ) ;
#4208=CARTESIAN_POINT ( 'NONE',  ( -6.000000000000000888, 1.067854986875958443E-15, 7.560779664488942560E-35 ) ) ;
#4209=CARTESIAN_POINT ( 'NONE',  ( -3.608439182435115633, 6.249999999999965361, -157.8080127018922383 ) ) ;
#4211=MECHANICAL_DESIGN_GEOMETRIC_PRESENTATION_REPRESENTATION('',(#8718),#25292);
#4212=CARTESIAN_POINT ( 'NONE',  ( -3.175426480542816066, 5.499999999999865885, -83.87500000000004263 ) ) ;
#4213=ADVANCED_FACE ( 'NONE', ( #4678 ), #14110, .T. ) ;
#4214=CARTESIAN_POINT ( 'NONE',  ( 0.000000000000000000, 5.499999999999991118, -76.50000000000001421 ) ) ;
#4222=CARTESIAN_POINT ( 'NONE',  ( 6.000000000000000888, 1.743066579297358182E-13, -55.58632486540519579 ) ) ;
#4224=CARTESIAN_POINT ( 'NONE',  ( -5.999999999999963585, 9.296355089585909904E-15, -169.4136751345948539 ) ) ;
#4227=CARTESIAN_POINT ( 'NONE',  ( -5.999999999999963585, 1.780251999655701777E-13, -109.4136751345948113 ) ) ;
#4229=DIRECTION ( 'NONE',  ( -7.147005652999508048E-36, 5.642372883946980038E-36, 1.000000000000000000 ) ) ;
#4230=ORIENTED_EDGE ( 'NONE', *, *, #10693, .F. ) ;
#4231=ORIENTED_EDGE ( 'NONE', *, *, #22296, .T. ) ;
#4232=ORIENTED_EDGE ( 'NONE', *, *, #20711, .F. ) ;
#4233=CARTESIAN_POINT ( 'NONE',  ( -3.175426480542816510, -5.500000000000057732, -98.37500000000000000 ) ) ;
#4234=CARTESIAN_POINT ( 'NONE',  ( 2.775557561562891351E-14, -6.250000000000061284, -106.1830127018922383 ) ) ;
#4239=CARTESIAN_POINT ( 'NONE',  ( 6.000000000000000888, -1.607695154586752384, -105.7306624327026299 ) ) ;
#4241=CARTESIAN_POINT ( 'NONE',  ( -5.196152422706601826, 2.999999999999975131, -159.9613248654052597 ) ) ;
#4244=CARTESIAN_POINT ( 'NONE',  ( 4.763139720814407951, 2.750000000000002665, -166.7500000000000000 ) ) ;
#4247=CARTESIAN_POINT ( 'NONE',  ( 3.175426480543072749, -5.500000000000105693, -110.1249999999999716 ) ) ;
#4250=CARTESIAN_POINT ( 'NONE',  ( -3.175426480542816510, 5.499999999999865885, -98.87499999999998579 ) ) ;
#4264=CARTESIAN_POINT ( 'NONE',  ( -7.216878364870328078, 0.000000000000000000, -86.19198729810781856 ) ) ;
#4266=VECTOR ( 'NONE', #4794, 1000.000000000000000 ) ;
#4268=( BOUNDED_CURVE ( )  B_SPLINE_CURVE ( 2, ( #28977, #24382, #28669, #23949, #14597, #7644, #19196, #28525, #17053 ),
 .UNSPECIFIED., .F., .T. ) 
 B_SPLINE_CURVE_WITH_KNOTS ( ( 3, 2, 2, 2, 3 ),
 ( 0.09166666666666666019, 0.09259259259259258745, 0.09444444444444444198, 0.09629629629629629650, 0.09722222222222222376 ),
 .UNSPECIFIED. ) 
 CURVE ( )  GEOMETRIC_REPRESENTATION_ITEM ( )  RATIONAL_B_SPLINE_CURVE ( ( 0.9330127018922194093, 0.9330127018922189652, 1.000000000000000000, 0.8660254037844388186, 1.000000000000000000, 0.8660254037844388186, 1.000000000000000000, 0.9330127018922194093, 0.9330127018922194093 ) ) 
 REPRESENTATION_ITEM ( '' )  );
#4269=ORIENTED_EDGE ( 'NONE', *, *, #11894, .F. ) ;
#4272=ORIENTED_EDGE ( 'NONE', *, *, #10270, .F. ) ;
#4273=CARTESIAN_POINT ( 'NONE',  ( -3.175426480542816510, -5.500000000000057732, -122.3749999999999716 ) ) ;
#4275=CARTESIAN_POINT ( 'NONE',  ( 7.216878364870455975, -6.409875621278545621E-14, -129.8080127018922383 ) ) ;
#4276=ORIENTED_EDGE ( 'NONE', *, *, #3068, .F. ) ;
#4277=CARTESIAN_POINT ( 'NONE',  ( -5.999999999999963585, 1.780251999655701777E-13, -57.83632486540521711 ) ) ;
#4278=CARTESIAN_POINT ( 'NONE',  ( -5.412658773652684552, -3.125000000000099920, -171.5669872981078186 ) ) ;
#4279=CARTESIAN_POINT ( 'NONE',  ( 2.775557561562891351E-14, -6.250000000000061284, -174.3169872981078470 ) ) ;
#4282=LINE ( 'NONE', #20419, #12813 ) ;
#4283=EDGE_CURVE ( 'NONE', #28542, #27987, #9608, .T. ) ;
#4287=CARTESIAN_POINT ( 'NONE',  ( -5.999999999999963585, 1.780251999655701777E-13, -95.33632486540520290 ) ) ;
#4288=CARTESIAN_POINT ( 'NONE',  ( 3.464101615137852974, 5.999999999999884537, -133.3363248654052313 ) ) ;
#4291=CARTESIAN_POINT ( 'NONE',  ( -3.608439182435115633, 6.249999999999965361, -75.94198729810784698 ) ) ;
#4292=CARTESIAN_POINT ( 'NONE',  ( 5.412658773652739619, 3.124999999999988898, -58.31698729810786119 ) ) ;
#4293=CARTESIAN_POINT ( 'NONE',  ( 0.000000000000000000, 5.499999999999991118, -52.49999999999999289 ) ) ;
#4295=CARTESIAN_POINT ( 'NONE',  ( -5.999999999999963585, 1.780251999655701777E-13, -47.91367513459483973 ) ) ;
#4297=CARTESIAN_POINT ( 'NONE',  ( -5.999999999999963585, 1.780251999655701777E-13, -63.83632486540523132 ) ) ;
#4298=CARTESIAN_POINT ( 'NONE',  ( 6.350852961086080661, -9.614813431917819062E-14, -120.3750000000000142 ) ) ;
#4299=CARTESIAN_POINT ( 'NONE',  ( -2.775557561562891351E-14, -5.500000000000115463, -156.7500000000000568 ) ) ;
#4300=CARTESIAN_POINT ( 'NONE',  ( -3.464101615137725076, 5.999999999999979572, -138.1636751345948824 ) ) ;
#4302=EDGE_LOOP ( 'NONE', ( #26549, #17154, #853, #5721 ) ) ;
#4304=DIRECTION ( 'NONE',  ( 1.000000000000000000, -5.551115123125773458E-17, -1.260129944081490338E-35 ) ) ;
#4306=EDGE_LOOP ( 'NONE', ( #23629, #17186, #10557, #7384 ) ) ;
#4310=CARTESIAN_POINT ( 'NONE',  ( -7.216878364870328078, 0.000000000000000000, -111.6919872981078186 ) ) ;
#4313=AXIS2_PLACEMENT_3D ( 'NONE', #9104, #16914, #4177 ) ;
#4314=ORIENTED_EDGE ( 'NONE', *, *, #6293, .T. ) ;
#4317=CARTESIAN_POINT ( 'NONE',  ( 5.412658773652739619, 3.124999999999988898, -50.81698729810779724 ) ) ;
#4318=COLOUR_RGB ( '', 0.66274510, 0.83137255, 0.94901961) ;
#4319=ORIENTED_EDGE ( 'NONE', *, *, #3289, .F. ) ;
#4320=CARTESIAN_POINT ( 'NONE',  ( -5.412658773652684552, -3.125000000000099920, -149.0669872981078470 ) ) ;
#4323=CARTESIAN_POINT ( 'NONE',  ( 7.216878364870455975, -6.409875621278545621E-14, -65.30801270189225249 ) ) ;
#4326=CARTESIAN_POINT ( 'NONE',  ( -5.196152422706573404, -3.000000000000002665, -125.2113248654052029 ) ) ;
#4327=CARTESIAN_POINT ( 'NONE',  ( -3.464101615137757051, -5.999999999999979572, -70.16367513459481131 ) ) ;
#4328=CARTESIAN_POINT ( 'NONE',  ( 0.000000000000000000, -5.999999999999991118, -155.5386751345948539 ) ) ;
#4331=CARTESIAN_POINT ( 'NONE',  ( -6.000000000000007105, -1.607695154586655129, -95.26933756729739855 ) ) ;
#4332=CARTESIAN_POINT ( 'NONE',  ( 4.763139720814407951, -2.749999999999988454, -120.5000000000000568 ) ) ;
#4335=CARTESIAN_POINT ( 'NONE',  ( 3.175426480543072749, -5.500000000000105693, -53.12500000000002842 ) ) ;
#4336=CARTESIAN_POINT ( 'NONE',  ( -3.464101615137725076, 5.999999999999979572, -70.08632486540525974 ) ) ;
#4337=VERTEX_POINT ( 'NONE', #25731 ) ;
#4341=EDGE_CURVE ( 'NONE', #29376, #12844, #30183, .T. ) ;
#4342=CARTESIAN_POINT ( 'NONE',  ( -3.175426480542816510, 5.499999999999865885, -140.8750000000000568 ) ) ;
#4346=CARTESIAN_POINT ( 'NONE',  ( -3.175426480542816510, -5.500000000000057732, -62.37500000000001421 ) ) ;
#4348=( BOUNDED_CURVE ( )  B_SPLINE_CURVE ( 2, ( #12914, #6110, #5786, #22710, #20259, #8094, #29605, #22103, #24986 ),
 .UNSPECIFIED., .F., .T. ) 
 B_SPLINE_CURVE_WITH_KNOTS ( ( 3, 2, 2, 2, 3 ),
 ( 0.5305555555555555580, 0.5314814814814814437, 0.5333333333333333259, 0.5351851851851852082, 0.5361111111111110938 ),
 .UNSPECIFIED. ) 
 CURVE ( )  GEOMETRIC_REPRESENTATION_ITEM ( )  RATIONAL_B_SPLINE_CURVE ( ( 0.9330127018922194093, 0.9330127018922194093, 1.000000000000000000, 0.8660254037844388186, 1.000000000000000000, 0.8660254037844388186, 1.000000000000000000, 0.9330127018922194093, 0.9330127018922194093 ) ) 
 REPRESENTATION_ITEM ( '' )  );
#4349=CARTESIAN_POINT ( 'NONE',  ( -7.216878364870328078, 0.000000000000000000, -90.05801270189223828 ) ) ;
#4350=EDGE_CURVE ( 'NONE', #19051, #14937, #21283, .T. ) ;
#4354=CARTESIAN_POINT ( 'NONE',  ( 5.999999999999999112, 2.951592740943527306E-14, -150.6636751345948539 ) ) ;
#4357=( BOUNDED_CURVE ( )  B_SPLINE_CURVE ( 2, ( #8143, #21848, #17408, #10179, #5685, #3084, #10329, #28727, #28581 ),
 .UNSPECIFIED., .F., .T. ) 
 B_SPLINE_CURVE_WITH_KNOTS ( ( 3, 2, 2, 2, 3 ),
 ( 0.2361111111111110494, 0.2370370370370370461, 0.2388888888888889284, 0.2407407407407406996, 0.2416666666666666963 ),
 .UNSPECIFIED. ) 
 CURVE ( )  GEOMETRIC_REPRESENTATION_ITEM ( )  RATIONAL_B_SPLINE_CURVE ( ( 0.9330127018922194093, 0.9330127018922154125, 1.000000000000000000, 0.8660254037844388186, 1.000000000000000000, 0.8660254037844388186, 1.000000000000000000, 0.9330127018922154125, 0.9330127018922194093 ) ) 
 REPRESENTATION_ITEM ( '' )  );
#4358=CARTESIAN_POINT ( 'NONE',  ( 6.350852961086080661, -9.614813431917819062E-14, -150.3749999999999716 ) ) ;
#4360=CARTESIAN_POINT ( 'NONE',  ( 3.175426480543072749, -5.500000000000105693, -141.6250000000000000 ) ) ;
#4361=CARTESIAN_POINT ( 'NONE',  ( -3.608439182435052128, -6.250000000000110134, -163.3080127018922667 ) ) ;
#4363=CARTESIAN_POINT ( 'NONE',  ( 6.000000000000000888, 1.743066579297358182E-13, -49.58632486540520290 ) ) ;
#4364=CARTESIAN_POINT ( 'NONE',  ( 4.763139720814407951, -2.749999999999988454, -80.00000000000001421 ) ) ;
#4366=CARTESIAN_POINT ( 'NONE',  ( -3.175426480542816510, 5.499999999999865885, -74.87500000000000000 ) ) ;
#4367=CARTESIAN_POINT ( 'NONE',  ( 0.000000000000000000, 5.999999999999977796, -154.7886751345948255 ) ) ;
#4371=CARTESIAN_POINT ( 'NONE',  ( -5.999999999999963585, -1.487416814333745711E-14, -118.4136751345948255 ) ) ;
#4380=FACE_OUTER_BOUND ( 'NONE', #28546, .T. ) ;
#4381=ORIENTED_EDGE ( 'NONE', *, *, #17113, .F. ) ;
#4384=CARTESIAN_POINT ( 'NONE',  ( -4.763139720814407951, -2.750000000000016431, -91.00000000000002842 ) ) ;
#4385=EDGE_CURVE ( 'NONE', #15456, #21925, #24186, .T. ) ;
#4386=CARTESIAN_POINT ( 'NONE',  ( -5.412658773652739619, 3.124999999999975131, -111.1830127018922383 ) ) ;
#4387=EDGE_CURVE ( 'NONE', #12154, #87, #4547, .T. ) ;
#4389=DIRECTION ( 'NONE',  ( 1.000000000000000000, -5.551115123125774074E-17, -1.260129944081490070E-35 ) ) ;
#4391=CARTESIAN_POINT ( 'NONE',  ( 4.513192036456002754, -10.03241344175769534, -28.95831720094627926 ) ) ;
#4393=CARTESIAN_POINT ( 'NONE',  ( 0.000000000000000000, 5.999999999999977796, -46.78867513459483973 ) ) ;
#4396=CARTESIAN_POINT ( 'NONE',  ( -3.175426480542816066, 5.499999999999865885, -173.8750000000000568 ) ) ;
#4398=CARTESIAN_POINT ( 'NONE',  ( 6.350852961086080661, -9.614813431917819062E-14, -163.8750000000000284 ) ) ;
#4400=VECTOR ( 'NONE', #3514, 1000.000000000000000 ) ;
#4401=( BOUNDED_CURVE ( )  B_SPLINE_CURVE ( 2, ( #23507, #11861, #27771, #6748, #21201, #9523, #16168, #25473, #13863 ),
 .UNSPECIFIED., .F., .F. ) 
 B_SPLINE_CURVE_WITH_KNOTS ( ( 3, 2, 2, 2, 3 ),
 ( 0.3305555555555555469, 0.3314814814814814881, 0.3333333333333333148, 0.3351851851851851971, 0.3361111111111110827 ),
 .UNSPECIFIED. ) 
 CURVE ( )  GEOMETRIC_REPRESENTATION_ITEM ( )  RATIONAL_B_SPLINE_CURVE ( ( 0.9330127018922194093, 0.9330127018922194093, 1.000000000000000000, 0.8660254037844388186, 1.000000000000000000, 0.8660254037844388186, 1.000000000000000000, 0.9330127018922214077, 0.9330127018922194093 ) ) 
 REPRESENTATION_ITEM ( '' )  );
#4402=CARTESIAN_POINT ( 'NONE',  ( 3.175426480543072749, -5.500000000000105693, -102.6250000000000142 ) ) ;
#4403=CARTESIAN_POINT ( 'NONE',  ( -5.196152422706573404, -3.000000000000002665, -166.2886751345948255 ) ) ;
#4404=CARTESIAN_POINT ( 'NONE',  ( 6.350852961086080661, -9.614813431917819062E-14, -96.37499999999997158 ) ) ;
#4410=CARTESIAN_POINT ( 'NONE',  ( 6.000000000000000888, 1.607695154586715303, -130.5193375672974128 ) ) ;
#4412=LINE ( 'NONE', #11683, #13537 ) ;
#4414=CARTESIAN_POINT ( 'NONE',  ( -3.464101615137757051, -5.999999999999979572, -170.0863248654051745 ) ) ;
#4416=CARTESIAN_POINT ( 'NONE',  ( 2.775557561562891351E-14, -6.250000000000061284, -85.81698729810783277 ) ) ;
#4419=CARTESIAN_POINT ( 'NONE',  ( 3.464101615137757051, -5.999999999999979572, -65.41367513459485394 ) ) ;
#4423=VERTEX_POINT ( 'NONE', #961 ) ;
#4424=CARTESIAN_POINT ( 'NONE',  ( -2.775557561562891351E-14, -5.500000000000115463, -123.7500000000000284 ) ) ;
#4426=EDGE_CURVE ( 'NONE', #16190, #6115, #16992, .T. ) ;
#4427=CARTESIAN_POINT ( 'NONE',  ( 5.412658773652739619, 3.124999999999988898, -129.6830127018922667 ) ) ;
#4430=CARTESIAN_POINT ( 'NONE',  ( 3.608439182435180470, 6.249999999999982236, -170.6919872981078470 ) ) ;
#4431=CARTESIAN_POINT ( 'NONE',  ( 5.412658773652712085, -3.125000000000086153, -177.0669872981078186 ) ) ;
#4438=DIRECTION ( 'NONE',  ( 1.000000000000000000, -5.551115123125773458E-17, -1.260129944081490338E-35 ) ) ;
#4439=CARTESIAN_POINT ( 'NONE',  ( -3.464101615137725076, 5.999999999999979572, -133.0863248654052313 ) ) ;
#4440=CARTESIAN_POINT ( 'NONE',  ( 3.464101615137757051, -5.999999999999979572, -150.3363248654051176 ) ) ;
#4442=CARTESIAN_POINT ( 'NONE',  ( 5.412658773652712085, -3.125000000000086153, -73.56698729810784698 ) ) ;
#4443=CARTESIAN_POINT ( 'NONE',  ( -5.412658773652684552, -3.125000000000099920, -60.56698729810783277 ) ) ;
#4444=CARTESIAN_POINT ( 'NONE',  ( -4.763139720814407951, 2.749999999999946709, -49.25000000000001421 ) ) ;
#4447=CARTESIAN_POINT ( 'NONE',  ( -5.999999999999963585, 1.780251999655701777E-13, -53.91367513459482552 ) ) ;
#4448=CARTESIAN_POINT ( 'NONE',  ( 3.175426480543072749, -5.500000000000105693, -117.6250000000000284 ) ) ;
#4451=ORIENTED_EDGE ( 'NONE', *, *, #26909, .T. ) ;
#4453=CARTESIAN_POINT ( 'NONE',  ( -5.999999999999963585, 1.780251999655701777E-13, -104.9136751345948255 ) ) ;
#4454=( BOUNDED_CURVE ( )  B_SPLINE_CURVE ( 2, ( #4869, #9508, #23640, #18894, #16305, #16452, #14300, #28063, #11846 ),
 .UNSPECIFIED., .F., .T. ) 
 B_SPLINE_CURVE_WITH_KNOTS ( ( 3, 2, 2, 2, 3 ),
 ( 0.04722222222222216548, 0.04814814814814816213, 0.05000000000000004441, 0.05185185185185181567, 0.05277777777777781232 ),
 .UNSPECIFIED. ) 
 CURVE ( )  GEOMETRIC_REPRESENTATION_ITEM ( )  RATIONAL_B_SPLINE_CURVE ( ( 0.9330127018922194093, 0.9330127018922154125, 1.000000000000000000, 0.8660254037844388186, 1.000000000000000000, 0.8660254037844388186, 1.000000000000000000, 0.9330127018922154125, 0.9330127018922194093 ) ) 
 REPRESENTATION_ITEM ( '' )  );
#4455=AXIS2_PLACEMENT_3D ( 'NONE', #4661, #4516, #29855 ) ;
#4456=ORIENTED_EDGE ( 'NONE', *, *, #1406, .T. ) ;
#4458=LINE ( 'NONE', #18775, #2007 ) ;
#4460=CARTESIAN_POINT ( 'NONE',  ( -3.608439182435115633, 6.249999999999965361, -107.4419872981077901 ) ) ;
#4462=FACE_OUTER_BOUND ( 'NONE', #12535, .T. ) ;
#4463=EDGE_CURVE ( 'NONE', #17549, #16378, #20073, .T. ) ;
#4465=ORIENTED_EDGE ( 'NONE', *, *, #20957, .F. ) ;
#4467=CARTESIAN_POINT ( 'NONE',  ( 6.000000000000000888, -3.330669073875464691E-16, -7.560779664488942560E-35 ) ) ;
#4470=CARTESIAN_POINT ( 'NONE',  ( 3.608439182435180470, 6.249999999999982236, -140.6919872981078470 ) ) ;
#4475=CARTESIAN_POINT ( 'NONE',  ( 3.608439182435180470, 6.249999999999982236, -71.05801270189222407 ) ) ;
#4478=CARTESIAN_POINT ( 'NONE',  ( 0.000000000000000000, 0.000000000000000000, -185.0000000000000000 ) ) ;
#4479=CARTESIAN_POINT ( 'NONE',  ( 0.000000000000000000, 0.000000000000000000, 0.000000000000000000 ) ) ;
#4485=CARTESIAN_POINT ( 'NONE',  ( 4.763139720814407951, 2.750000000000002665, -121.7500000000000284 ) ) ;
#4486=CARTESIAN_POINT ( 'NONE',  ( -5.999999999999963585, -1.487416814333745711E-14, -92.91367513459482552 ) ) ;
#4487=CARTESIAN_POINT ( 'NONE',  ( -5.412658773652684552, -3.125000000000099920, -145.4330127018922383 ) ) ;
#4488=CARTESIAN_POINT ( 'NONE',  ( 5.999999999999949374, 1.607695154586804565, -113.0966878364870638 ) ) ;
#4489=ORIENTED_EDGE ( 'NONE', *, *, #6252, .T. ) ;
#4491=CARTESIAN_POINT ( 'NONE',  ( -3.175426480542816066, 5.499999999999865885, -58.37500000000004974 ) ) ;
#4492=CARTESIAN_POINT ( 'NONE',  ( 3.464101615137852974, 5.999999999999884537, -62.83632486540521711 ) ) ;
#4495=VECTOR ( 'NONE', #28538, 1000.000000000000000 ) ;
#4498=CARTESIAN_POINT ( 'NONE',  ( 2.775557561562891351E-14, 6.250000000000033751, -106.0669872981078186 ) ) ;
#4500=EDGE_CURVE ( 'NONE', #22104, #21789, #2226, .T. ) ;
#4502=DIRECTION ( 'NONE',  ( 1.000000000000000000, -5.551115123125773458E-17, -1.260129944081490338E-35 ) ) ;
#4504=VECTOR ( 'NONE', #16769, 1000.000000000000000 ) ;
#4505=CARTESIAN_POINT ( 'NONE',  ( -2.775557561562891351E-14, -5.500000000000115463, -138.7500000000000284 ) ) ;
#4507=VECTOR ( 'NONE', #18687, 1000.000000000000000 ) ;
#4510=CARTESIAN_POINT ( 'NONE',  ( 3.175426480543072749, -5.500000000000105693, -62.12500000000000711 ) ) ;
#4513=AXIS2_PLACEMENT_3D ( 'NONE', #26595, #15591, #29195 ) ;
#4516=DIRECTION ( 'NONE',  ( -7.147005652999508048E-36, 5.642372883946980038E-36, 1.000000000000000000 ) ) ;
#4518=CARTESIAN_POINT ( 'NONE',  ( -2.775557561562891351E-14, -5.500000000000115463, -150.7500000000000568 ) ) ;
#4520=CARTESIAN_POINT ( 'NONE',  ( 4.763139720814407951, -2.749999999999988454, -140.0000000000000000 ) ) ;
#4521=CARTESIAN_POINT ( 'NONE',  ( -5.412658773652684552, -3.125000000000099920, -157.4330127018922383 ) ) ;
#4523=EDGE_CURVE ( 'NONE', #407, #10456, #7680, .T. ) ;
#4524=CARTESIAN_POINT ( 'NONE',  ( 3.175426480543072749, -5.500000000000105693, -75.62500000000001421 ) ) ;
#4525=CARTESIAN_POINT ( 'NONE',  ( -5.999999999999963585, 1.780251999655701777E-13, -69.83632486540523132 ) ) ;
#4526=CARTESIAN_POINT ( 'NONE',  ( -3.175426480542816510, -5.500000000000057732, -75.87500000000001421 ) ) ;
#4528=LINE ( 'NONE', #11792, #18165 ) ;
#4531=CARTESIAN_POINT ( 'NONE',  ( 5.196152422706629359, 3.000000000000002665, -134.0386751345948255 ) ) ;
#4533=CARTESIAN_POINT ( 'NONE',  ( -6.000000000000000888, 1.067854986875958443E-15, 7.560779664488942560E-35 ) ) ;
#4535=ADVANCED_FACE ( 'NONE', ( #28763 ), #7731, .T. ) ;
#4538=CARTESIAN_POINT ( 'NONE',  ( 0.000000000000000000, -5.999999999999991118, -109.0386751345948113 ) ) ;
#4540=CARTESIAN_POINT ( 'NONE',  ( -5.196152422706601826, 2.999999999999975131, -179.4613248654052313 ) ) ;
#4541=ORIENTED_EDGE ( 'NONE', *, *, #3918, .T. ) ;
#4542=ORIENTED_EDGE ( 'NONE', *, *, #14882, .T. ) ;
#4544=ORIENTED_EDGE ( 'NONE', *, *, #533, .F. ) ;
#4545=CARTESIAN_POINT ( 'NONE',  ( -3.175426480542816510, -5.500000000000057732, -86.37500000000005684 ) ) ;
#4546=CARTESIAN_POINT ( 'NONE',  ( 5.412658773652739619, 3.124999999999988898, -105.6830127018922383 ) ) ;
#4547=( BOUNDED_CURVE ( )  B_SPLINE_CURVE ( 2, ( #25579, #20992, #30339, #6989, #21737, #14680, #26907, #1114, #3413 ),
 .UNSPECIFIED., .F., .T. ) 
 B_SPLINE_CURVE_WITH_KNOTS ( ( 3, 2, 2, 2, 3 ),
 ( 0.6138888888888888173, 0.6148148148148148140, 0.6166666666666666963, 0.6185185185185184675, 0.6194444444444444642 ),
 .UNSPECIFIED. ) 
 CURVE ( )  GEOMETRIC_REPRESENTATION_ITEM ( )  RATIONAL_B_SPLINE_CURVE ( ( 0.9330127018922194093, 0.9330127018922154125, 1.000000000000000000, 0.8660254037844388186, 1.000000000000000000, 0.8660254037844388186, 1.000000000000000000, 0.9330127018922154125, 0.9330127018922194093 ) ) 
 REPRESENTATION_ITEM ( '' )  );
#4548=ORIENTED_EDGE ( 'NONE', *, *, #5303, .F. ) ;
#4551=CARTESIAN_POINT ( 'NONE',  ( 6.350852961086080661, -9.614813431917819062E-14, -163.8750000000000284 ) ) ;
#4552=CARTESIAN_POINT ( 'NONE',  ( 4.384309399116693484, -10.08956758734763071, -29.10056064752990679 ) ) ;
#4554=CARTESIAN_POINT ( 'NONE',  ( 3.464101615137757051, -5.999999999999979572, -67.83632486540517448 ) ) ;
#4556=CARTESIAN_POINT ( 'NONE',  ( 3.175426480543072749, 5.499999999999865885, -169.6250000000000000 ) ) ;
#4557=LINE ( 'NONE', #11196, #20392 ) ;
#4558=CARTESIAN_POINT ( 'NONE',  ( -3.175426480542816510, -5.500000000000057732, -165.8750000000000568 ) ) ;
#4561=CARTESIAN_POINT ( 'NONE',  ( 3.175426480543072749, -5.500000000000105693, -99.62500000000007105 ) ) ;
#4562=DIRECTION ( 'NONE',  ( -7.147005652999508048E-36, 5.642372883946980038E-36, 1.000000000000000000 ) ) ;
#4563=CARTESIAN_POINT ( 'NONE',  ( -6.350852961085760029, -1.281975124255709124E-13, -97.12500000000004263 ) ) ;
#4576=ORIENTED_EDGE ( 'NONE', *, *, #21687, .F. ) ;
#4577=CARTESIAN_POINT ( 'NONE',  ( 0.000000000000000000, -5.999999999999991118, -141.4613248654052029 ) ) ;
#4579=CARTESIAN_POINT ( 'NONE',  ( 0.000000000000000000, 5.499999999999991118, -117.0000000000000000 ) ) ;
#4581=ORIENTED_EDGE ( 'NONE', *, *, #11046, .T. ) ;
#4582=CARTESIAN_POINT ( 'NONE',  ( 7.216878364870455975, -6.409875621278545621E-14, -131.3080127018922667 ) ) ;
#4585=CARTESIAN_POINT ( 'NONE',  ( 7.216878364870455975, -6.409875621278545621E-14, -169.4419872981078470 ) ) ;
#4591=CARTESIAN_POINT ( 'NONE',  ( 6.000000000000000888, -1.859271017917181981E-14, -68.16367513459481131 ) ) ;
#4593=CARTESIAN_POINT ( 'NONE',  ( 5.412658773652739619, 3.124999999999988898, -174.6830127018922383 ) ) ;
#4597=CARTESIAN_POINT ( 'NONE',  ( -6.350852961085760029, -1.281975124255709124E-13, -121.1250000000000426 ) ) ;
#4598=CARTESIAN_POINT ( 'NONE',  ( -3.464101615137725076, 5.999999999999979572, -166.0863248654052029 ) ) ;
#4600=AXIS2_PLACEMENT_3D ( 'NONE', #15759, #4023, #13442 ) ;
#4605=EDGE_CURVE ( 'NONE', #21925, #6123, #29994, .T. ) ;
#4606=ORIENTED_EDGE ( 'NONE', *, *, #16341, .T. ) ;
#4609=CARTESIAN_POINT ( 'NONE',  ( 5.412658773652739619, 3.124999999999988898, -109.3169872981077901 ) ) ;
#4611=CARTESIAN_POINT ( 'NONE',  ( -5.999999999999964473, 9.063946212346262433E-15, -174.8363248654052313 ) ) ;
#4616=ORIENTED_EDGE ( 'NONE', *, *, #10478, .T. ) ;
#4617=CARTESIAN_POINT ( 'NONE',  ( -5.412658773652739619, 3.124999999999975131, -135.8169872981078186 ) ) ;
#4621=LINE ( 'NONE', #14052, #19136 ) ;
#4622=CARTESIAN_POINT ( 'NONE',  ( 2.775557561562891351E-14, -6.250000000000061284, -62.68301270189225249 ) ) ;
#4625=CARTESIAN_POINT ( 'NONE',  ( -6.000000000000000888, 1.067854986875958443E-15, 7.560779664488942560E-35 ) ) ;
#4629=EDGE_CURVE ( 'NONE', #3499, #2708, #20482, .T. ) ;
#4630=CARTESIAN_POINT ( 'NONE',  ( -5.196152422706573404, -3.000000000000002665, -95.21132486540517448 ) ) ;
#4631=ADVANCED_FACE ( 'NONE', ( #3874 ), #15612, .T. ) ;
#4632=( BOUNDED_CURVE ( )  B_SPLINE_CURVE ( 2, ( #6859, #16285, #13981, #23321, #11671, #17160, #2551, #2695, #28628 ),
 .UNSPECIFIED., .F., .T. ) 
 B_SPLINE_CURVE_WITH_KNOTS ( ( 3, 2, 2, 2, 3 ),
 ( 0.7472222222222222321, 0.7481481481481481177, 0.7500000000000000000, 0.7518518518518518823, 0.7527777777777777679 ),
 .UNSPECIFIED. ) 
 CURVE ( )  GEOMETRIC_REPRESENTATION_ITEM ( )  RATIONAL_B_SPLINE_CURVE ( ( 0.9330127018922194093, 0.9330127018922194093, 1.000000000000000000, 0.8660254037844388186, 1.000000000000000000, 0.8660254037844388186, 1.000000000000000000, 0.9330127018922194093, 0.9330127018922194093 ) ) 
 REPRESENTATION_ITEM ( '' )  );
#4634=CARTESIAN_POINT ( 'NONE',  ( 7.216878364870455975, -6.409875621278545621E-14, -143.3080127018922667 ) ) ;
#4636=VERTEX_POINT ( 'NONE', #22334 ) ;
#4637=CARTESIAN_POINT ( 'NONE',  ( 0.000000000000000000, 5.499999999999991118, -57.00000000000004974 ) ) ;
#4638=CARTESIAN_POINT ( 'NONE',  ( -6.000000000000007105, -1.607695154586655129, -155.2693375672974412 ) ) ;
#4639=CARTESIAN_POINT ( 'NONE',  ( -5.999999999999963585, -1.487416814333745711E-14, -171.8363248654052313 ) ) ;
#4644=CARTESIAN_POINT ( 'NONE',  ( 7.216878364870455975, -6.409875621278545621E-14, -106.4419872981078470 ) ) ;
#4645=AXIS2_PLACEMENT_3D ( 'NONE', #7752, #26483, #21908 ) ;
#4647=LINE ( 'NONE', #25847, #13158 ) ;
#4649=CARTESIAN_POINT ( 'NONE',  ( 0.000000000000000000, 0.000000000000000000, 0.000000000000000000 ) ) ;
#4650=CARTESIAN_POINT ( 'NONE',  ( 3.175426480543072749, 5.499999999999865885, -135.1250000000000000 ) ) ;
#4651=ORIENTED_EDGE ( 'NONE', *, *, #3057, .F. ) ;
#4652=ORIENTED_EDGE ( 'NONE', *, *, #5887, .F. ) ;
#4653=VECTOR ( 'NONE', #6075, 1000.000000000000000 ) ;
#4654=CARTESIAN_POINT ( 'NONE',  ( -4.763139720814407951, 2.749999999999946709, -67.25000000000002842 ) ) ;
#4655=LINE ( 'NONE', #30315, #5762 ) ;
#4659=CYLINDRICAL_SURFACE ( 'NONE', #312, 6.000000000000000888 ) ;
#4660=EDGE_CURVE ( 'NONE', #26117, #7780, #13450, .T. ) ;
#4661=CARTESIAN_POINT ( 'NONE',  ( 0.000000000000000000, 0.000000000000000000, 0.000000000000000000 ) ) ;
#4663=EDGE_CURVE ( 'NONE', #26866, #18250, #15991, .T. ) ;
#4664=CARTESIAN_POINT ( 'NONE',  ( 0.000000000000000000, 5.499999999999991118, -151.5000000000000284 ) ) ;
#4666=CARTESIAN_POINT ( 'NONE',  ( -3.175426480542816510, 5.499999999999865885, -137.8750000000000568 ) ) ;
#4667=CARTESIAN_POINT ( 'NONE',  ( 3.608439182435180470, -6.249999999999997335, -158.5580127018922383 ) ) ;
#4668=CARTESIAN_POINT ( 'NONE',  ( -4.763139720814407951, -2.750000000000016431, -82.00000000000001421 ) ) ;
#4669=CARTESIAN_POINT ( 'NONE',  ( 0.000000000000000000, 5.499999999999991118, -67.50000000000000000 ) ) ;
#4672=CARTESIAN_POINT ( 'NONE',  ( -5.999999999999962697, -1.607695154586733954, -175.3466878364870354 ) ) ;
#4677=( BOUNDED_CURVE ( )  B_SPLINE_CURVE ( 2, ( #7776, #5320, #5172, #19767, #24217, #8071, #17192, #10264, #14729 ),
 .UNSPECIFIED., .F., .F. ) 
 B_SPLINE_CURVE_WITH_KNOTS ( ( 3, 2, 2, 2, 3 ),
 ( 0.5249999999999999112, 0.5259259259259259078, 0.5277777777777777901, 0.5296296296296296724, 0.5305555555555555580 ),
 .UNSPECIFIED. ) 
 CURVE ( )  GEOMETRIC_REPRESENTATION_ITEM ( )  RATIONAL_B_SPLINE_CURVE ( ( 0.9330127018922194093, 0.9330127018922154125, 1.000000000000000000, 0.8660254037844388186, 1.000000000000000000, 0.8660254037844388186, 1.000000000000000000, 0.9330127018922194093, 0.9330127018922194093 ) ) 
 REPRESENTATION_ITEM ( '' )  );
#4678=FACE_OUTER_BOUND ( 'NONE', #13386, .T. ) ;
#4680=DIRECTION ( 'NONE',  ( -7.147005652999508048E-36, 5.642372883946980038E-36, 1.000000000000000000 ) ) ;
#4688=ORIENTED_EDGE ( 'NONE', *, *, #10167, .F. ) ;
#4689=CARTESIAN_POINT ( 'NONE',  ( 4.763139720814407951, -2.749999999999988454, -92.00000000000002842 ) ) ;
#4690=CARTESIAN_POINT ( 'NONE',  ( -3.608439182435052128, -6.250000000000110134, -107.8080127018922667 ) ) ;
#4692=CARTESIAN_POINT ( 'NONE',  ( 0.8083154347086104474, 10.97740844234572677, -30.95886765600325319 ) ) ;
#4694=CARTESIAN_POINT ( 'NONE',  ( -6.350852961085760029, -1.281975124255709124E-13, -166.1249999999999716 ) ) ;
#4695=CARTESIAN_POINT ( 'NONE',  ( 6.000000000000000888, -1.859271017917181981E-14, -105.6636751345948397 ) ) ;
#4697=CARTESIAN_POINT ( 'NONE',  ( -6.000000000000007105, -1.607695154586655129, -68.26933756729739855 ) ) ;
#4698=SHAPE_REPRESENTATION_RELATIONSHIP ( 'NONE' , 'NONE' ,  #13689, #15129 ) ;
#4700=CARTESIAN_POINT ( 'NONE',  ( -3.175426480542816066, -5.500000000000057732, -171.8750000000000284 ) ) ;
#4701=CYLINDRICAL_SURFACE ( 'NONE', #8619, 6.000000000000000888 ) ;
#4702=CARTESIAN_POINT ( 'NONE',  ( 0.000000000000000000, 5.499999999999991118, -157.5000000000000284 ) ) ;
#4704=CARTESIAN_POINT ( 'NONE',  ( 0.000000000000000000, 5.499999999999991118, -102.0000000000000284 ) ) ;
#4705=CARTESIAN_POINT ( 'NONE',  ( 5.196152422706629359, -2.999999999999988898, -159.2113248654052313 ) ) ;
#4707=CARTESIAN_POINT ( 'NONE',  ( 4.763139720814407951, -2.749999999999988454, -89.00000000000002842 ) ) ;
#4711=VERTEX_POINT ( 'NONE', #25073 ) ;
#4719=ORIENTED_EDGE ( 'NONE', *, *, #21426, .T. ) ;
#4722=AXIS2_PLACEMENT_3D ( 'NONE', #9789, #21473, #28795 ) ;
#4723=ORIENTED_EDGE ( 'NONE', *, *, #8408, .F. ) ;
#4726=EDGE_CURVE ( 'NONE', #26400, #15757, #29841, .T. ) ;
#4730=CARTESIAN_POINT ( 'NONE',  ( -3.175426480542816510, -5.500000000000057732, -111.8750000000000568 ) ) ;
#4732=CARTESIAN_POINT ( 'NONE',  ( 5.412658773652712085, -3.125000000000086153, -129.9330127018922383 ) ) ;
#4735=CARTESIAN_POINT ( 'NONE',  ( -3.608439182435052128, -6.250000000000110134, -166.9419872981078470 ) ) ;
#4739=ORIENTED_EDGE ( 'NONE', *, *, #17183, .T. ) ;
#4741=EDGE_CURVE ( 'NONE', #8028, #25601, #6332, .T. ) ;
#4742=CARTESIAN_POINT ( 'NONE',  ( 5.196152422706629359, 3.000000000000002665, -95.96132486540520290 ) ) ;
#4744=CARTESIAN_POINT ( 'NONE',  ( -4.763139720814407951, -2.750000000000016431, -178.0000000000000568 ) ) ;
#4746=CARTESIAN_POINT ( 'NONE',  ( 2.775557561562891351E-14, 6.250000000000033751, -174.4330127018922667 ) ) ;
#4750=CARTESIAN_POINT ( 'NONE',  ( 0.000000000000000000, 5.499999999999991118, -121.5000000000000568 ) ) ;
#4752=ORIENTED_EDGE ( 'NONE', *, *, #12313, .F. ) ;
#4754=LINE ( 'NONE', #16777, #4495 ) ;
#4758=VERTEX_POINT ( 'NONE', #18508 ) ;
#4762=CARTESIAN_POINT ( 'NONE',  ( 6.000000000000000888, 1.743066579297358182E-13, -95.16367513459482552 ) ) ;
#4766=CARTESIAN_POINT ( 'NONE',  ( 3.464101615137852974, 5.999999999999884537, -141.4136751345948255 ) ) ;
#4769=ORIENTED_EDGE ( 'NONE', *, *, #3715, .T. ) ;
#4770=AXIS2_PLACEMENT_3D ( 'NONE', #6350, #22660, #6209 ) ;
#4771=CARTESIAN_POINT ( 'NONE',  ( 2.775557561562891351E-14, -6.250000000000061284, -142.8169872981078186 ) ) ;
#4773=CARTESIAN_POINT ( 'NONE',  ( 0.000000000000000000, 5.999999999999977796, -151.2113248654052313 ) ) ;
#4780=CARTESIAN_POINT ( 'NONE',  ( 0.000000000000000000, 5.999999999999977796, -102.2886751345948255 ) ) ;
#4781=CARTESIAN_POINT ( 'NONE',  ( 0.000000000000000000, 0.000000000000000000, 0.000000000000000000 ) ) ;
#4782=LINE ( 'NONE', #4625, #17835 ) ;
#4784=CARTESIAN_POINT ( 'NONE',  ( -5.196152422706601826, 2.999999999999975131, -113.4613248654052171 ) ) ;
#4787=ORIENTED_EDGE ( 'NONE', *, *, #16682, .T. ) ;
#4788=CARTESIAN_POINT ( 'NONE',  ( 3.175426480543072749, 5.499999999999865885, -54.12500000000003553 ) ) ;
#4790=VERTEX_POINT ( 'NONE', #11460 ) ;
#4793=CARTESIAN_POINT ( 'NONE',  ( 3.608439182435180470, 6.249999999999982236, -100.1919872981078186 ) ) ;
#4794=DIRECTION ( 'NONE',  ( -7.147005652999508048E-36, 5.642372883946980038E-36, 1.000000000000000000 ) ) ;
#4795=AXIS2_PLACEMENT_3D ( 'NONE', #2938, #21705, #12653 ) ;
#4798=ADVANCED_FACE ( 'NONE', ( #21250 ), #16525, .T. ) ;
#4799=CARTESIAN_POINT ( 'NONE',  ( 4.763139720814407951, -2.749999999999988454, -134.0000000000000000 ) ) ;
#4800=ORIENTED_EDGE ( 'NONE', *, *, #18705, .T. ) ;
#4802=EDGE_LOOP ( 'NONE', ( #28213, #7708, #15503, #19545 ) ) ;
#4804=CARTESIAN_POINT ( 'NONE',  ( -3.175426480542816510, -5.500000000000057732, -68.37500000000002842 ) ) ;
#4806=CARTESIAN_POINT ( 'NONE',  ( -5.196152422706601826, 2.999999999999975131, -66.03867513459482552 ) ) ;
#4808=CARTESIAN_POINT ( 'NONE',  ( 5.412658773652712085, -3.125000000000086153, -81.93301270189223828 ) ) ;
#4809=( BOUNDED_CURVE ( )  B_SPLINE_CURVE ( 2, ( #12414, #26480, #14276, #2993, #12267, #28495, #23617, #21306, #7750 ),
 .UNSPECIFIED., .F., .T. ) 
 B_SPLINE_CURVE_WITH_KNOTS ( ( 3, 2, 2, 2, 3 ),
 ( 0.8527777777777778567, 0.8537037037037037424, 0.8555555555555556246, 0.8574074074074073959, 0.8583333333333332815 ),
 .UNSPECIFIED. ) 
 CURVE ( )  GEOMETRIC_REPRESENTATION_ITEM ( )  RATIONAL_B_SPLINE_CURVE ( ( 0.9330127018922194093, 0.9330127018922234061, 1.000000000000000000, 0.8660254037844388186, 1.000000000000000000, 0.8660254037844388186, 1.000000000000000000, 0.9330127018922234061, 0.9330127018922194093 ) ) 
 REPRESENTATION_ITEM ( '' )  );
#4813=CARTESIAN_POINT ( 'NONE',  ( 6.000000000000000888, 1.743066579297358182E-13, -61.58632486540521001 ) ) ;
#4816=CARTESIAN_POINT ( 'NONE',  ( 4.763139720814407951, 2.750000000000002665, -148.7500000000000568 ) ) ;
#4818=CARTESIAN_POINT ( 'NONE',  ( 2.775557561562891351E-14, -6.250000000000061284, -160.1830127018922667 ) ) ;
#4819=( NAMED_UNIT ( * ) PLANE_ANGLE_UNIT ( ) SI_UNIT ( $, .RADIAN. ) );
#4820=DIRECTION ( 'NONE',  ( -7.147005652999508048E-36, 5.642372883946980038E-36, 1.000000000000000000 ) ) ;
#4822=CARTESIAN_POINT ( 'NONE',  ( 4.763139720814407951, -2.749999999999988454, -62.00000000000000000 ) ) ;
#4825=DIRECTION ( 'NONE',  ( -7.147005652999508048E-36, 5.642372883946980038E-36, 1.000000000000000000 ) ) ;
#4836=EDGE_CURVE ( 'NONE', #29837, #14973, #4647, .T. ) ;
#4842=CARTESIAN_POINT ( 'NONE',  ( 6.350852961086080661, -9.614813431917819062E-14, -85.87500000000005684 ) ) ;
#4843=EDGE_LOOP ( 'NONE', ( #16138, #22753, #11096, #1313 ) ) ;
#4847=CARTESIAN_POINT ( 'NONE',  ( -6.350852961085760029, -1.281975124255709124E-13, -175.1250000000000284 ) ) ;
#4848=CARTESIAN_POINT ( 'NONE',  ( -2.000000000000000000, 3.559516622919861969E-16, -200.0000000000000000 ) ) ;
#4849=CARTESIAN_POINT ( 'NONE',  ( -4.763139720814407951, -2.750000000000016431, -151.0000000000000284 ) ) ;
#4853=CARTESIAN_POINT ( 'NONE',  ( -2.775557561562891351E-14, -5.500000000000115463, -102.7500000000000142 ) ) ;
#4855=DIRECTION ( 'NONE',  ( 7.147005652999508048E-36, -5.642372883946980038E-36, -1.000000000000000000 ) ) ;
#4856=CARTESIAN_POINT ( 'NONE',  ( -2.775557561562891351E-14, -5.500000000000115463, -155.2500000000000000 ) ) ;
#4857=CARTESIAN_POINT ( 'NONE',  ( -4.763139720814407951, -2.750000000000016431, -91.00000000000002842 ) ) ;
#4859=VERTEX_POINT ( 'NONE', #2497 ) ;
#4862=CARTESIAN_POINT ( 'NONE',  ( -5.196152422706601826, 2.999999999999975131, -126.0386751345948824 ) ) ;
#4869=CARTESIAN_POINT ( 'NONE',  ( 6.000000000000000888, 1.743066579297358182E-13, -52.58632486540518869 ) ) ;
#4872=ORIENTED_EDGE ( 'NONE', *, *, #570, .T. ) ;
#4873=CARTESIAN_POINT ( 'NONE',  ( -6.350852961085760029, -1.281975124255709124E-13, -115.1250000000000000 ) ) ;
#4875=CARTESIAN_POINT ( 'NONE',  ( -3.608439182435052128, -6.250000000000110134, -130.3080127018922383 ) ) ;
#4876=VERTEX_POINT ( 'NONE', #25694 ) ;
#4877=FACE_OUTER_BOUND ( 'NONE', #1315, .T. ) ;
#4878=CARTESIAN_POINT ( 'NONE',  ( -5.412658773652684552, -3.125000000000099920, -167.0669872981078186 ) ) ;
#4882=LINE ( 'NONE', #25792, #14374 ) ;
#4884=CARTESIAN_POINT ( 'NONE',  ( -2.775557561562891351E-14, -5.500000000000115463, -177.7500000000000284 ) ) ;
#4886=CARTESIAN_POINT ( 'NONE',  ( 6.000000000000000888, 1.743066579297358182E-13, -111.0863248654051887 ) ) ;
#4887=CARTESIAN_POINT ( 'NONE',  ( 7.216878364870455975, -6.409875621278545621E-14, -180.8080127018922099 ) ) ;
#4889=CARTESIAN_POINT ( 'NONE',  ( 6.000000000000000888, 1.743066579297358182E-13, -53.16367513459481131 ) ) ;
#4891=CARTESIAN_POINT ( 'NONE',  ( -4.763139720814407951, 2.749999999999946709, -113.7500000000000142 ) ) ;
#4893=CARTESIAN_POINT ( 'NONE',  ( -5.196152422706601826, 2.999999999999975131, -145.5386751345948539 ) ) ;
#4894=VERTEX_POINT ( 'NONE', #23413 ) ;
#4895=EDGE_CURVE ( 'NONE', #26645, #14008, #4357, .T. ) ;
#4896=DIRECTION ( 'NONE',  ( -7.147005652999508048E-36, 5.642372883946980038E-36, 1.000000000000000000 ) ) ;
#4898=LINE ( 'NONE', #23667, #11160 ) ;
#4904=CARTESIAN_POINT ( 'NONE',  ( 5.196152422706629359, -2.999999999999988898, -176.2886751345948539 ) ) ;
#4905=CARTESIAN_POINT ( 'NONE',  ( 6.000000000000052403, -1.607695154586662678, -95.23066243270257303 ) ) ;
#4907=LINE ( 'NONE', #7229, #7393 ) ;
#4908=EDGE_LOOP ( 'NONE', ( #15687, #13085, #7514, #17307 ) ) ;
#4913=CARTESIAN_POINT ( 'NONE',  ( -5.412658773652684552, -3.125000000000099920, -141.5669872981077901 ) ) ;
#4919=CARTESIAN_POINT ( 'NONE',  ( -3.464101615137725076, 5.999999999999979572, -102.1636751345948255 ) ) ;
#4920=CARTESIAN_POINT ( 'NONE',  ( -5.999999999999962697, 3.323446944526963260E-14, -161.3363248654052597 ) ) ;
#4921=CARTESIAN_POINT ( 'NONE',  ( -5.999999999999919176, 1.607695154586804565, -146.4033121635129930 ) ) ;
#4922=AXIS2_PLACEMENT_3D ( 'NONE', #25645, #6294, #1841 ) ;
#4924=FACE_OUTER_BOUND ( 'NONE', #6201, .T. ) ;
#4926=CARTESIAN_POINT ( 'NONE',  ( 3.464101615137757051, -5.999999999999979572, -142.8363248654052029 ) ) ;
#4929=ORIENTED_EDGE ( 'NONE', *, *, #21716, .T. ) ;
#4930=EDGE_CURVE ( 'NONE', #6568, #15139, #1091, .T. ) ;
#4931=CARTESIAN_POINT ( 'NONE',  ( 0.000000000000000000, -5.999999999999991118, -106.9613248654052171 ) ) ;
#4932=CARTESIAN_POINT ( 'NONE',  ( 0.000000000000000000, 5.999999999999977796, -52.78867513459483973 ) ) ;
#4934=CARTESIAN_POINT ( 'NONE',  ( 0.000000000000000000, -5.999999999999991118, -178.9613248654052313 ) ) ;
#4938=CARTESIAN_POINT ( 'NONE',  ( -3.608439182435115633, 6.249999999999965361, -105.9419872981078470 ) ) ;
#4940=EDGE_CURVE ( 'NONE', #11050, #20611, #28306, .T. ) ;
#4941=VECTOR ( 'NONE', #4855, 1000.000000000000000 ) ;
#4944=CARTESIAN_POINT ( 'NONE',  ( 6.350852961086080661, -9.614813431917819062E-14, -127.8749999999999858 ) ) ;
#4947=CARTESIAN_POINT ( 'NONE',  ( 4.763139720814407951, -2.749999999999988454, -66.50000000000000000 ) ) ;
#4948=CARTESIAN_POINT ( 'NONE',  ( 6.000000000000052403, -1.607695154586662678, -81.15331216351296462 ) ) ;
#4950=CARTESIAN_POINT ( 'NONE',  ( 7.216878364870455975, -6.409875621278545621E-14, -81.80801270189226670 ) ) ;
#4951=CARTESIAN_POINT ( 'NONE',  ( 6.000000000000000888, 7.762456499804234384E-14, -140.1636751345948255 ) ) ;
#4953=CARTESIAN_POINT ( 'NONE',  ( -5.999999999999963585, -2.788906526875773208E-15, -176.3363248654052029 ) ) ;
#4954=COLOUR_RGB ( '', 0.09019608, 0.27058824, 0.51372549) ;
#4955=CARTESIAN_POINT ( 'NONE',  ( -5.999999999999963585, 1.780251999655701777E-13, -94.41367513459482552 ) ) ;
#4957=CARTESIAN_POINT ( 'NONE',  ( -4.763139720814407951, -2.750000000000016431, -137.5000000000000000 ) ) ;
#4959=CIRCLE ( 'NONE', #8913, 11.00000000000001599 ) ;
#4960=CARTESIAN_POINT ( 'NONE',  ( 3.608439182435180470, -6.249999999999997335, -152.5580127018922099 ) ) ;
#4963=ADVANCED_FACE ( 'NONE', ( #7845 ), #5237, .T. ) ;
#4964=CARTESIAN_POINT ( 'NONE',  ( -3.175426480542816066, 5.499999999999865885, -79.37500000000002842 ) ) ;
#4965=CARTESIAN_POINT ( 'NONE',  ( -5.196152422706601826, 2.999999999999975131, -114.0386751345948113 ) ) ;
#4966=CARTESIAN_POINT ( 'NONE',  ( -2.775557561562891351E-14, -5.500000000000115463, -66.75000000000002842 ) ) ;
#4967=CARTESIAN_POINT ( 'NONE',  ( 5.999999999999999112, 2.951592740943527306E-14, -155.1636751345948539 ) ) ;
#4968=CARTESIAN_POINT ( 'NONE',  ( -3.464101615137757051, -5.999999999999979572, -148.1636751345947971 ) ) ;
#4972=CARTESIAN_POINT ( 'NONE',  ( 0.000000000000000000, -5.999999999999991118, -49.96132486540522422 ) ) ;
#4974=EDGE_CURVE ( 'NONE', #22535, #18178, #5514, .T. ) ;
#4984=CARTESIAN_POINT ( 'NONE',  ( 3.608439182435180470, 6.249999999999982236, -152.6919872981078186 ) ) ;
#4986=CARTESIAN_POINT ( 'NONE',  ( -4.763139720814407951, -2.750000000000016431, -88.00000000000002842 ) ) ;
#4991=CARTESIAN_POINT ( 'NONE',  ( 1.960615434941584301, -10.82557180451506085, -19.32589338774632282 ) ) ;
#4993=CARTESIAN_POINT ( 'NONE',  ( 3.175426480543072749, 5.499999999999865885, -166.6250000000000000 ) ) ;
#4994=CARTESIAN_POINT ( 'NONE',  ( -5.999999999999919176, 1.607695154586804565, -57.90331216351300014 ) ) ;
#4995=CARTESIAN_POINT ( 'NONE',  ( -4.763139720814407951, 2.749999999999946709, -152.7500000000000568 ) ) ;
#4998=CARTESIAN_POINT ( 'NONE',  ( 3.175426480543072749, 5.499999999999865885, -103.6250000000000142 ) ) ;
#4999=CARTESIAN_POINT ( 'NONE',  ( 6.000000000000000888, 1.743066579297358182E-13, -60.08632486540520290 ) ) ;
#5000=EDGE_CURVE ( 'NONE', #11352, #25418, #8678, .T. ) ;
#5001=CARTESIAN_POINT ( 'NONE',  ( 6.350852961086080661, -9.614813431917819062E-14, -85.87500000000005684 ) ) ;
#5009=CARTESIAN_POINT ( 'NONE',  ( -5.196152422706601826, 2.999999999999975131, -78.03867513459483973 ) ) ;
#5010=ORIENTED_EDGE ( 'NONE', *, *, #13796, .F. ) ;
#5011=CARTESIAN_POINT ( 'NONE',  ( 0.000000000000000000, 10.49588505988223375, 0.000000000000000000 ) ) ;
#5012=DIRECTION ( 'NONE',  ( -7.147005652999508048E-36, 5.642372883946980038E-36, 1.000000000000000000 ) ) ;
#5015=EDGE_LOOP ( 'NONE', ( #8507, #27747, #5826, #6157 ) ) ;
#5016=CARTESIAN_POINT ( 'NONE',  ( 0.000000000000000000, 5.499999999999991118, -113.9999999999999858 ) ) ;
#5018=CARTESIAN_POINT ( 'NONE',  ( 2.775557561562891351E-14, -6.250000000000061284, -121.1830127018922383 ) ) ;
#5022=CARTESIAN_POINT ( 'NONE',  ( 5.412658773652739619, 3.124999999999988898, -164.8169872981077901 ) ) ;
#5026=CARTESIAN_POINT ( 'NONE',  ( -4.509628467067655855, 10.03401783428613925, -21.03762154299059262 ) ) ;
#5028=CARTESIAN_POINT ( 'NONE',  ( -5.999999999999956479, -1.607695154586745057, -150.7693375672974412 ) ) ;
#5031=CARTESIAN_POINT ( 'NONE',  ( -5.412658773652739619, 3.124999999999975131, -180.1830127018922383 ) ) ;
#5032=CARTESIAN_POINT ( 'NONE',  ( 0.000000000000000000, 5.999999999999977796, -76.21132486540521711 ) ) ;
#5033=CARTESIAN_POINT ( 'NONE',  ( -5.999999999999963585, -1.487416814333745711E-14, -101.9136751345948397 ) ) ;
#5034=CARTESIAN_POINT ( 'NONE',  ( -3.175426480542816066, -5.500000000000057732, -126.8749999999999858 ) ) ;
#5038=CARTESIAN_POINT ( 'NONE',  ( 3.175426480543072749, 5.499999999999865885, -111.1249999999999716 ) ) ;
#5040=CARTESIAN_POINT ( 'NONE',  ( -3.464101615137725076, 5.999999999999979572, -100.6636751345948113 ) ) ;
#5042=DIRECTION ( 'NONE',  ( -7.147005652999508048E-36, 5.642372883946980038E-36, 1.000000000000000000 ) ) ;
#5044=CARTESIAN_POINT ( 'NONE',  ( -5.999999999999962697, 3.323446944526963260E-14, -155.3363248654052313 ) ) ;
#5045=AXIS2_PLACEMENT_3D ( 'NONE', #5602, #17937, #22528 ) ;
#5047=CARTESIAN_POINT ( 'NONE',  ( 5.196152422706629359, -2.999999999999988898, -126.2113248654052029 ) ) ;
#5048=LINE ( 'NONE', #2608, #19976 ) ;
#5054=ORIENTED_EDGE ( 'NONE', *, *, #3778, .T. ) ;
#5057=EDGE_LOOP ( 'NONE', ( #20908, #7809, #11425, #17225 ) ) ;
#5058=CARTESIAN_POINT ( 'NONE',  ( 5.412658773652712085, -3.125000000000086153, -139.5669872981077901 ) ) ;
#5061=EDGE_CURVE ( 'NONE', #20652, #22535, #14798, .T. ) ;
#5062=CYLINDRICAL_SURFACE ( 'NONE', #7389, 6.000000000000000888 ) ;
#5065=FACE_OUTER_BOUND ( 'NONE', #6997, .T. ) ;
#5070=DIRECTION ( 'NONE',  ( -7.147005652999508048E-36, 5.642372883946980038E-36, 1.000000000000000000 ) ) ;
#5072=CARTESIAN_POINT ( 'NONE',  ( 3.464101615137852974, 5.999999999999884537, -60.41367513459482552 ) ) ;
#5073=CARTESIAN_POINT ( 'NONE',  ( -5.999999999999971578, 1.607695154586715303, -113.4033121635130072 ) ) ;
#5075=EDGE_CURVE ( 'NONE', #19519, #28690, #24359, .T. ) ;
#5076=EDGE_LOOP ( 'NONE', ( #27362, #17209, #7964, #7510 ) ) ;
#5077=CARTESIAN_POINT ( 'NONE',  ( 4.763139720814407951, -2.749999999999988454, -48.49999999999998579 ) ) ;
#5079=CARTESIAN_POINT ( 'NONE',  ( 0.000000000000000000, 0.000000000000000000, 0.000000000000000000 ) ) ;
#5080=CARTESIAN_POINT ( 'NONE',  ( -5.999999999999962697, 3.323446944526963260E-14, -152.3363248654052313 ) ) ;
#5081=EDGE_LOOP ( 'NONE', ( #25310, #17800, #17660, #8345 ) ) ;
#5083=CARTESIAN_POINT ( 'NONE',  ( 3.608439182435180470, -6.249999999999997335, -106.6919872981078612 ) ) ;
#5084=CARTESIAN_POINT ( 'NONE',  ( -5.196152422706601826, 2.999999999999975131, -172.5386751345947971 ) ) ;
#5087=CARTESIAN_POINT ( 'NONE',  ( -3.175426480542816510, 5.499999999999865885, -130.3750000000000284 ) ) ;
#5091=CARTESIAN_POINT ( 'NONE',  ( -5.999999999999919176, 1.607695154586804565, -95.98066243270261566 ) ) ;
#5093=CARTESIAN_POINT ( 'NONE',  ( -3.175426480542816510, -5.500000000000057732, -54.87500000000003553 ) ) ;
#5096=CARTESIAN_POINT ( 'NONE',  ( 5.412658773652739619, 3.124999999999988898, -81.68301270189226670 ) ) ;
#5098=LINE ( 'NONE', #14810, #86 ) ;
#5099=CARTESIAN_POINT ( 'NONE',  ( -3.464101615137725076, 5.999999999999979572, -149.5863248654051176 ) ) ;
#5101=CARTESIAN_POINT ( 'NONE',  ( 3.464101615137757051, -5.999999999999979572, -175.8363248654052029 ) ) ;
#5102=CARTESIAN_POINT ( 'NONE',  ( -5.999999999999963585, 1.780251999655701777E-13, -60.83632486540522422 ) ) ;
#5104=EDGE_CURVE ( 'NONE', #124, #18584, #19108, .T. ) ;
#5106=ADVANCED_FACE ( 'NONE', ( #4462 ), #14335, .T. ) ;
#5107=CARTESIAN_POINT ( 'NONE',  ( -3.175426480542816066, 5.499999999999865885, -140.8750000000000568 ) ) ;
#5109=CARTESIAN_POINT ( 'NONE',  ( 3.608439182435180470, 6.249999999999982236, -150.5580127018922667 ) ) ;
#5111=CARTESIAN_POINT ( 'NONE',  ( 6.350852961086080661, -9.614813431917819062E-14, -70.87500000000004263 ) ) ;
#5113=CARTESIAN_POINT ( 'NONE',  ( -3.175426480542816510, -5.500000000000057732, -65.37500000000001421 ) ) ;
#5114=CARTESIAN_POINT ( 'NONE',  ( -5.196152422706601826, 2.999999999999975131, -53.46132486540522422 ) ) ;
#5118=CARTESIAN_POINT ( 'NONE',  ( 6.000000000000000888, 1.743066579297358182E-13, -98.16367513459481131 ) ) ;
#5125=CARTESIAN_POINT ( 'NONE',  ( 7.216878364870455975, -6.409875621278545621E-14, -46.44198729810782567 ) ) ;
#5127=CARTESIAN_POINT ( 'NONE',  ( 7.216878364870455975, -6.409875621278545621E-14, -152.9419872981078186 ) ) ;
#5130=CARTESIAN_POINT ( 'NONE',  ( -4.763139720814407951, 2.749999999999946709, -82.25000000000004263 ) ) ;
#5132=CARTESIAN_POINT ( 'NONE',  ( -3.608439182435115633, 6.249999999999965361, -99.30801270189222407 ) ) ;
#5137=DIRECTION ( 'NONE',  ( 1.000000000000000000, -5.551115123125773458E-17, -1.260129944081490338E-35 ) ) ;
#5140=EDGE_CURVE ( 'NONE', #8549, #7308, #23235, .T. ) ;
#5142=CARTESIAN_POINT ( 'NONE',  ( 3.175426480543072749, -5.500000000000105693, -165.6250000000000000 ) ) ;
#5143=CARTESIAN_POINT ( 'NONE',  ( 6.000000000000052403, -1.607695154586662678, -60.15331216351297883 ) ) ;
#5144=CARTESIAN_POINT ( 'NONE',  ( -3.175426480542816510, 5.499999999999865885, -157.3750000000000000 ) ) ;
#5147=CARTESIAN_POINT ( 'NONE',  ( -2.775557561562891351E-14, -5.500000000000115463, -92.25000000000000000 ) ) ;
#5149=( BOUNDED_CURVE ( )  B_SPLINE_CURVE ( 2, ( #17326, #19905, #26642, #3299, #15007, #24346, #10400, #19752, #15163 ),
 .UNSPECIFIED., .F., .F. ) 
 B_SPLINE_CURVE_WITH_KNOTS ( ( 3, 2, 2, 2, 3 ),
 ( 0.6083333333333333925, 0.6092592592592592782, 0.6111111111111111605, 0.6129629629629629317, 0.6138888888888889284 ),
 .UNSPECIFIED. ) 
 CURVE ( )  GEOMETRIC_REPRESENTATION_ITEM ( )  RATIONAL_B_SPLINE_CURVE ( ( 0.9330127018922194093, 0.9330127018922234061, 1.000000000000000000, 0.8660254037844388186, 1.000000000000000000, 0.8660254037844388186, 1.000000000000000000, 0.9330127018922154125, 0.9330127018922194093 ) ) 
 REPRESENTATION_ITEM ( '' )  );
#5150=CARTESIAN_POINT ( 'NONE',  ( 6.350852961086080661, -9.614813431917819062E-14, -91.87500000000001421 ) ) ;
#5156=CARTESIAN_POINT ( 'NONE',  ( 6.000000000000000888, 1.743066579297358182E-13, -73.58632486540520290 ) ) ;
#5160=AXIS2_PLACEMENT_3D ( 'NONE', #17672, #19800, #5959 ) ;
#5161=DIRECTION ( 'NONE',  ( 1.000000000000000000, -5.551115123125773458E-17, -1.260129944081490338E-35 ) ) ;
#5164=VERTEX_POINT ( 'NONE', #9229 ) ;
#5166=VECTOR ( 'NONE', #3445, 1000.000000000000000 ) ;
#5168=CARTESIAN_POINT ( 'NONE',  ( -4.763139720814407951, -2.750000000000016431, -108.9999999999999858 ) ) ;
#5170=CARTESIAN_POINT ( 'NONE',  ( 2.775557561562891351E-14, -6.250000000000061284, -125.6830127018922525 ) ) ;
#5171=ORIENTED_EDGE ( 'NONE', *, *, #5691, .F. ) ;
#5172=CARTESIAN_POINT ( 'NONE',  ( -5.196152422706573404, -3.000000000000002665, -110.7886751345948397 ) ) ;
#5173=CARTESIAN_POINT ( 'NONE',  ( -3.608439182435115633, 6.249999999999965361, -162.9419872981077901 ) ) ;
#5176=CARTESIAN_POINT ( 'NONE',  ( 3.608439182435180470, -6.249999999999997335, -61.05801270189223828 ) ) ;
#5178=CARTESIAN_POINT ( 'NONE',  ( 5.196152422706629359, 3.000000000000002665, -167.9613248654052029 ) ) ;
#5180=CARTESIAN_POINT ( 'NONE',  ( -0.7970850910874407447, 10.97816267869983875, -19.03975521967168660 ) ) ;
#5182=CARTESIAN_POINT ( 'NONE',  ( -3.175426480542816510, 5.499999999999865885, -175.3750000000000568 ) ) ;
#5185=CARTESIAN_POINT ( 'NONE',  ( -3.464101615137725076, 5.999999999999979572, -100.0863248654052029 ) ) ;
#5186=CARTESIAN_POINT ( 'NONE',  ( 2.775557561562891351E-14, 6.250000000000033751, -180.4330127018922667 ) ) ;
#5189=CARTESIAN_POINT ( 'NONE',  ( 4.763139720814407951, -2.749999999999988454, -126.5000000000000568 ) ) ;
#5191=CARTESIAN_POINT ( 'NONE',  ( 4.763139720814407951, 2.750000000000002665, -109.7500000000000142 ) ) ;
#5195=VERTEX_POINT ( 'NONE', #12473 ) ;
#5198=CARTESIAN_POINT ( 'NONE',  ( -5.999999999999963585, -1.487416814333745711E-14, -137.3363248654052313 ) ) ;
#5200=CARTESIAN_POINT ( 'NONE',  ( -3.464101615137757051, -5.999999999999979572, -126.5863248654051887 ) ) ;
#5201=CARTESIAN_POINT ( 'NONE',  ( 3.175426480543072749, 5.499999999999865885, -177.1250000000000284 ) ) ;
#5202=EDGE_LOOP ( 'NONE', ( #5010, #27511, #10723, #12735 ) ) ;
#5203=DIRECTION ( 'NONE',  ( 1.000000000000000000, -5.551115123125773458E-17, -1.260129944081490338E-35 ) ) ;
#5204=ORIENTED_EDGE ( 'NONE', *, *, #30306, .F. ) ;
#5205=ORIENTED_EDGE ( 'NONE', *, *, #29025, .T. ) ;
#5208=ADVANCED_FACE ( 'NONE', ( #9693 ), #28994, .T. ) ;
#5209=EDGE_CURVE ( 'NONE', #1357, #18127, #10298, .T. ) ;
#5211=CARTESIAN_POINT ( 'NONE',  ( -3.608439182435052128, -6.250000000000110134, -127.9419872981078186 ) ) ;
#5214=CARTESIAN_POINT ( 'NONE',  ( -5.999999999999963585, -1.487416814333745711E-14, -128.9136751345948539 ) ) ;
#5217=DIRECTION ( 'NONE',  ( -7.147005652999508048E-36, 5.642372883946980038E-36, 1.000000000000000000 ) ) ;
#5220=CARTESIAN_POINT ( 'NONE',  ( 6.000000000000000888, 1.743066579297358182E-13, -99.08632486540518869 ) ) ;
#5225=CARTESIAN_POINT ( 'NONE',  ( -3.464101615137757051, -5.999999999999979572, -143.0863248654052029 ) ) ;
#5226=CARTESIAN_POINT ( 'NONE',  ( -3.175426480542816510, 5.499999999999865885, -140.8750000000000568 ) ) ;
#5229=CARTESIAN_POINT ( 'NONE',  ( -3.175426480542816066, 5.499999999999865885, -50.87500000000001421 ) ) ;
#5230=CARTESIAN_POINT ( 'NONE',  ( 0.000000000000000000, -5.999999999999991118, -133.0386751345948824 ) ) ;
#5231=CARTESIAN_POINT ( 'NONE',  ( 3.464101615137757051, -5.999999999999979572, -99.91367513459481131 ) ) ;
#5232=ORIENTED_EDGE ( 'NONE', *, *, #25362, .T. ) ;
#5234=CARTESIAN_POINT ( 'NONE',  ( -6.000000000000000888, 1.067854986875958443E-15, 7.560779664488942560E-35 ) ) ;
#5236=CARTESIAN_POINT ( 'NONE',  ( 2.775557561562891351E-14, 6.250000000000033751, -92.56698729810780435 ) ) ;
#5237=CYLINDRICAL_SURFACE ( 'NONE', #4795, 6.000000000000000888 ) ;
#5242=AXIS2_PLACEMENT_3D ( 'NONE', #20334, #12996, #17747 ) ;
#5244=CARTESIAN_POINT ( 'NONE',  ( -2.775557561562891351E-14, -5.500000000000115463, -128.2500000000000284 ) ) ;
#5249=CARTESIAN_POINT ( 'NONE',  ( -4.763139720814407951, 2.749999999999946709, -59.75000000000002842 ) ) ;
#5250=CYLINDRICAL_SURFACE ( 'NONE', #14128, 6.000000000000000888 ) ;
#5252=CARTESIAN_POINT ( 'NONE',  ( 2.775557561562891351E-14, 10.99999999999998224, -31.00000000000002842 ) ) ;
#5253=CARTESIAN_POINT ( 'NONE',  ( 3.608439182435180470, -6.249999999999997335, -82.05801270189219565 ) ) ;
#5255=LINE ( 'NONE', #14663, #12851 ) ;
#5260=CARTESIAN_POINT ( 'NONE',  ( -6.350852961085760029, -1.281975124255709124E-13, -143.6250000000000000 ) ) ;
#5262=CARTESIAN_POINT ( 'NONE',  ( 0.000000000000000000, -5.999999999999991118, -70.96132486540524553 ) ) ;
#5263=CARTESIAN_POINT ( 'NONE',  ( 6.000000000000000888, -1.859271017917181981E-14, -72.66367513459483973 ) ) ;
#5264=CARTESIAN_POINT ( 'NONE',  ( 4.763139720814407951, -2.749999999999988454, -71.00000000000001421 ) ) ;
#5267=CARTESIAN_POINT ( 'NONE',  ( 6.350852961086080661, -9.614813431917819062E-14, -66.37500000000004263 ) ) ;
#5272=CARTESIAN_POINT ( 'NONE',  ( 0.000000000000000000, -5.999999999999991118, -104.5386751345948113 ) ) ;
#5274=FACE_OUTER_BOUND ( 'NONE', #22874, .T. ) ;
#5275=ORIENTED_EDGE ( 'NONE', *, *, #9213, .T. ) ;
#5277=AXIS2_PLACEMENT_3D ( 'NONE', #28209, #7185, #21030 ) ;
#5278=CARTESIAN_POINT ( 'NONE',  ( -5.196152422706573404, -3.000000000000002665, -102.7113248654052455 ) ) ;
#5280=CARTESIAN_POINT ( 'NONE',  ( 2.775557561562891351E-14, -6.250000000000061284, -46.81698729810779014 ) ) ;
#5283=ORIENTED_EDGE ( 'NONE', *, *, #22117, .T. ) ;
#5284=CARTESIAN_POINT ( 'NONE',  ( 0.000000000000000000, 5.499999999999991118, -84.00000000000001421 ) ) ;
#5286=CARTESIAN_POINT ( 'NONE',  ( 6.000000000000000888, -1.859271017917181981E-14, -54.66367513459481842 ) ) ;
#5287=CYLINDRICAL_SURFACE ( 'NONE', #27320, 6.000000000000000888 ) ;
#5289=CARTESIAN_POINT ( 'NONE',  ( -3.175426480542816066, -5.500000000000057732, -161.3750000000000284 ) ) ;
#5291=CARTESIAN_POINT ( 'NONE',  ( -4.763139720814407951, 2.749999999999946709, -158.7500000000000568 ) ) ;
#5293=CARTESIAN_POINT ( 'NONE',  ( -4.763139720814407951, 2.749999999999946709, -94.25000000000000000 ) ) ;
#5296=CARTESIAN_POINT ( 'NONE',  ( -4.763139720814407951, 2.749999999999946709, -91.25000000000005684 ) ) ;
#5299=CARTESIAN_POINT ( 'NONE',  ( 3.464101615137852974, 5.999999999999884537, -64.91367513459485394 ) ) ;
#5300=CARTESIAN_POINT ( 'NONE',  ( 5.196152422706629359, -2.999999999999988898, -135.7886751345947971 ) ) ;
#5303=EDGE_CURVE ( 'NONE', #13381, #8715, #13292, .T. ) ;
#5304=CARTESIAN_POINT ( 'NONE',  ( 0.000000000000000000, 5.999999999999977796, -126.2886751345948539 ) ) ;
#5306=DIRECTION ( 'NONE',  ( 1.000000000000000000, -5.551115123125773458E-17, -1.260129944081490338E-35 ) ) ;
#5308=CYLINDRICAL_SURFACE ( 'NONE', #16302, 6.000000000000000888 ) ;
#5310=EDGE_LOOP ( 'NONE', ( #3915, #25629, #24549, #13091 ) ) ;
#5311=EDGE_CURVE ( 'NONE', #651, #1699, #27943, .T. ) ;
#5313=VERTEX_POINT ( 'NONE', #20403 ) ;
#5316=CARTESIAN_POINT ( 'NONE',  ( -4.763139720814407951, -2.750000000000016431, -104.5000000000000426 ) ) ;
#5318=CARTESIAN_POINT ( 'NONE',  ( 2.775557561562891351E-14, -6.250000000000061284, -119.6830127018922383 ) ) ;
#5320=CARTESIAN_POINT ( 'NONE',  ( -6.000000000000007105, -1.607695154586655129, -110.8466878364870354 ) ) ;
#5321=CARTESIAN_POINT ( 'NONE',  ( 5.412658773652712085, -3.125000000000086153, -157.5669872981078186 ) ) ;
#5323=CARTESIAN_POINT ( 'NONE',  ( -7.216878364870328078, 0.000000000000000000, -61.55801270189223828 ) ) ;
#5324=VERTEX_POINT ( 'NONE', #24996 ) ;
#5325=( BOUNDED_CURVE ( )  B_SPLINE_CURVE ( 2, ( #7692, #5832, #15247, #636, #24579, #5231, #3528, #12958, #17252 ),
 .UNSPECIFIED., .F., .F. ) 
 B_SPLINE_CURVE_WITH_KNOTS ( ( 3, 2, 2, 2, 3 ),
 ( 0.6027777777777777457, 0.6037037037037037424, 0.6055555555555555136, 0.6074074074074073959, 0.6083333333333333925 ),
 .UNSPECIFIED. ) 
 CURVE ( )  GEOMETRIC_REPRESENTATION_ITEM ( )  RATIONAL_B_SPLINE_CURVE ( ( 0.9330127018922194093, 0.9330127018922154125, 1.000000000000000000, 0.8660254037844388186, 1.000000000000000000, 0.8660254037844388186, 1.000000000000000000, 0.9330127018922154125, 0.9330127018922194093 ) ) 
 REPRESENTATION_ITEM ( '' )  );
#5327=CARTESIAN_POINT ( 'NONE',  ( -3.464101615137725076, 5.999999999999979572, -137.5863248654051745 ) ) ;
#5328=CYLINDRICAL_SURFACE ( 'NONE', #28775, 6.000000000000000888 ) ;
#5331=CARTESIAN_POINT ( 'NONE',  ( 7.216878364870455975, -6.409875621278545621E-14, -168.8080127018922099 ) ) ;
#5334=CARTESIAN_POINT ( 'NONE',  ( 0.000000000000000000, 5.499999999999991118, -117.0000000000000000 ) ) ;
#5336=CARTESIAN_POINT ( 'NONE',  ( -3.175426480542816510, -5.500000000000057732, -116.3750000000000142 ) ) ;
#5339=CARTESIAN_POINT ( 'NONE',  ( 0.000000000000000000, 0.000000000000000000, 0.000000000000000000 ) ) ;
#5340=CARTESIAN_POINT ( 'NONE',  ( 6.000000000000000888, 1.743066579297358182E-13, -112.5863248654052029 ) ) ;
#5341=ORIENTED_EDGE ( 'NONE', *, *, #19889, .F. ) ;
#5345=CARTESIAN_POINT ( 'NONE',  ( -3.464101615137725076, 5.999999999999979572, -109.0863248654051745 ) ) ;
#5346=ORIENTED_EDGE ( 'NONE', *, *, #28734, .F. ) ;
#5348=CARTESIAN_POINT ( 'NONE',  ( 0.000000000000000000, 5.499999999999991118, -178.5000000000000000 ) ) ;
#5351=EDGE_CURVE ( 'NONE', #18174, #11659, #3808, .T. ) ;
#5352=CARTESIAN_POINT ( 'NONE',  ( 0.000000000000000000, 0.000000000000000000, 0.000000000000000000 ) ) ;
#5355=ORIENTED_EDGE ( 'NONE', *, *, #18630, .T. ) ;
#5359=CARTESIAN_POINT ( 'NONE',  ( 3.608439182435180470, -6.249999999999997335, -135.1919872981078470 ) ) ;
#5360=CARTESIAN_POINT ( 'NONE',  ( -5.196152422706601826, 2.999999999999975131, -130.5386751345948255 ) ) ;
#5361=CARTESIAN_POINT ( 'NONE',  ( 3.464101615137757051, -5.999999999999979572, -116.4136751345948255 ) ) ;
#5370=DIRECTION ( 'NONE',  ( 1.000000000000000000, -5.551115123125773458E-17, -1.260129944081490338E-35 ) ) ;
#5371=CARTESIAN_POINT ( 'NONE',  ( 6.000000000000000888, 1.743066579297358182E-13, -69.08632486540523132 ) ) ;
#5374=CARTESIAN_POINT ( 'NONE',  ( 4.763139720814407951, -2.749999999999988454, -137.0000000000000000 ) ) ;
#5376=EDGE_LOOP ( 'NONE', ( #11207, #21820, #19522, #21892 ) ) ;
#5377=( BOUNDED_CURVE ( )  B_SPLINE_CURVE ( 2, ( #27017, #22592, #18146, #8278, #8760, #17538, #20284, #3821, #29632 ),
 .UNSPECIFIED., .F., .F. ) 
 B_SPLINE_CURVE_WITH_KNOTS ( ( 3, 2, 2, 2, 3 ),
 ( 0.07499999999999999722, 0.07592592592592592449, 0.07777777777777777901, 0.07962962962962963354, 0.08055555555555556080 ),
 .UNSPECIFIED. ) 
 CURVE ( )  GEOMETRIC_REPRESENTATION_ITEM ( )  RATIONAL_B_SPLINE_CURVE ( ( 0.9330127018922194093, 0.9330127018922194093, 1.000000000000000000, 0.8660254037844388186, 1.000000000000000000, 0.8660254037844388186, 1.000000000000000000, 0.9330127018922194093, 0.9330127018922194093 ) ) 
 REPRESENTATION_ITEM ( '' )  );
#5379=LINE ( 'NONE', #788, #6729 ) ;
#5380=CARTESIAN_POINT ( 'NONE',  ( 6.000000000000000888, -1.859271017917181981E-14, -88.58632486540523132 ) ) ;
#5381=DIRECTION ( 'NONE',  ( -7.147005652999508048E-36, 5.642372883946980038E-36, 1.000000000000000000 ) ) ;
#5383=CARTESIAN_POINT ( 'NONE',  ( -3.464101615137757051, -5.999999999999979572, -164.0863248654052029 ) ) ;
#5387=CARTESIAN_POINT ( 'NONE',  ( 3.608439182435180470, -6.249999999999997335, -96.19198729810781856 ) ) ;
#5388=( BOUNDED_CURVE ( )  B_SPLINE_CURVE ( 2, ( #30146, #16070, #29989, #4336, #22638, #10830, #11127, #3718, #1883 ),
 .UNSPECIFIED., .F., .T. ) 
 B_SPLINE_CURVE_WITH_KNOTS ( ( 3, 2, 2, 2, 3 ),
 ( 0.1750000000000000444, 0.1759259259259259300, 0.1777777777777778123, 0.1796296296296295836, 0.1805555555555554692 ),
 .UNSPECIFIED. ) 
 CURVE ( )  GEOMETRIC_REPRESENTATION_ITEM ( )  RATIONAL_B_SPLINE_CURVE ( ( 0.9330127018922194093, 0.9330127018922234061, 1.000000000000000000, 0.8660254037844388186, 1.000000000000000000, 0.8660254037844388186, 1.000000000000000000, 0.9330127018922234061, 0.9330127018922194093 ) ) 
 REPRESENTATION_ITEM ( '' )  );
#5394=CARTESIAN_POINT ( 'NONE',  ( 0.000000000000000000, 5.499999999999991118, -130.5000000000000000 ) ) ;
#5398=CARTESIAN_POINT ( 'NONE',  ( 6.350852961086080661, -9.614813431917819062E-14, -55.87500000000003553 ) ) ;
#5399=DIRECTION ( 'NONE',  ( 1.000000000000000000, -5.551115123125774074E-17, 7.147005652999508048E-36 ) ) ;
#5400=CARTESIAN_POINT ( 'NONE',  ( -3.464101615137757051, -5.999999999999979572, -59.66367513459482552 ) ) ;
#5401=CARTESIAN_POINT ( 'NONE',  ( -5.412658773652684552, -3.125000000000099920, -82.43301270189223828 ) ) ;
#5402=CARTESIAN_POINT ( 'NONE',  ( 0.000000000000000000, 5.999999999999977796, -149.7113248654052313 ) ) ;
#5403=CARTESIAN_POINT ( 'NONE',  ( 5.196152422706629359, -2.999999999999988898, -168.2113248654052313 ) ) ;
#5405=CARTESIAN_POINT ( 'NONE',  ( -2.775557561562891351E-14, -5.500000000000115463, -143.2500000000000000 ) ) ;
#5407=CARTESIAN_POINT ( 'NONE',  ( 5.412658773652712085, -3.125000000000086153, -152.4330127018922383 ) ) ;
#5408=CARTESIAN_POINT ( 'NONE',  ( -6.000000000000000888, 1.067854986875958443E-15, 7.560779664488942560E-35 ) ) ;
#5410=CARTESIAN_POINT ( 'NONE',  ( -3.175426480542816066, -5.500000000000057732, -68.37500000000002842 ) ) ;
#5412=CARTESIAN_POINT ( 'NONE',  ( -2.775557561562891351E-14, -5.500000000000115463, -59.25000000000002842 ) ) ;
#5415=ORIENTED_EDGE ( 'NONE', *, *, #15316, .T. ) ;
#5420=CARTESIAN_POINT ( 'NONE',  ( 6.000000000000000888, 1.743066579297358182E-13, -57.66367513459481842 ) ) ;
#5421=CARTESIAN_POINT ( 'NONE',  ( 5.999999999999949374, 1.607695154586804565, -82.51933756729744118 ) ) ;
#5422=( BOUNDED_CURVE ( )  B_SPLINE_CURVE ( 2, ( #20106, #13081, #17829, #1047, #29450, #24399, #26683, #3643, #10596 ),
 .UNSPECIFIED., .F., .T. ) 
 B_SPLINE_CURVE_WITH_KNOTS ( ( 3, 2, 2, 2, 3 ),
 ( 0.1416666666666667185, 0.1425925925925926041, 0.1444444444444444864, 0.1462962962962962576, 0.1472222222222221433 ),
 .UNSPECIFIED. ) 
 CURVE ( )  GEOMETRIC_REPRESENTATION_ITEM ( )  RATIONAL_B_SPLINE_CURVE ( ( 0.9330127018922194093, 0.9330127018922234061, 1.000000000000000000, 0.8660254037844388186, 1.000000000000000000, 0.8660254037844388186, 1.000000000000000000, 0.9330127018922234061, 0.9330127018922194093 ) ) 
 REPRESENTATION_ITEM ( '' )  );
#5425=CARTESIAN_POINT ( 'NONE',  ( -5.999999999999963585, 1.780251999655701777E-13, -102.8363248654052313 ) ) ;
#5426=CARTESIAN_POINT ( 'NONE',  ( 3.175426480543072749, -5.500000000000105693, -176.1250000000000284 ) ) ;
#5429=CARTESIAN_POINT ( 'NONE',  ( -2.775557561562891351E-14, -5.500000000000115463, -80.25000000000004263 ) ) ;
#5430=AXIS2_PLACEMENT_3D ( 'NONE', #17576, #29670, #22932 ) ;
#5432=CARTESIAN_POINT ( 'NONE',  ( 5.196152422706629359, -2.999999999999988898, -127.7113248654052597 ) ) ;
#5433=EDGE_CURVE ( 'NONE', #5997, #18475, #26952, .T. ) ;
#5434=CARTESIAN_POINT ( 'NONE',  ( 6.000000000000000000, 2.951592740943527306E-14, -162.6636751345948824 ) ) ;
#5435=CARTESIAN_POINT ( 'NONE',  ( 5.792970643772029860, -9.351264793308468271, -23.42496030963405218 ) ) ;
#5438=CARTESIAN_POINT ( 'NONE',  ( -4.763139720814407951, 2.749999999999946709, -160.2500000000000000 ) ) ;
#5440=CARTESIAN_POINT ( 'NONE',  ( -6.350852961085760029, -1.281975124255709124E-13, -143.6250000000000000 ) ) ;
#5442=CARTESIAN_POINT ( 'NONE',  ( -3.175426480542816066, -5.500000000000057732, -98.37500000000000000 ) ) ;
#5444=CARTESIAN_POINT ( 'NONE',  ( 4.763139720814407951, 2.750000000000002665, -81.25000000000004263 ) ) ;
#5447=CARTESIAN_POINT ( 'NONE',  ( -5.999999999999982236, -1.607695154586700426, -136.3466878364870070 ) ) ;
#5450=CARTESIAN_POINT ( 'NONE',  ( -5.999999999999944933, 1.607695154586759934, -125.9806624327026157 ) ) ;
#5454=EDGE_LOOP ( 'NONE', ( #20110, #13772 ) ) ;
#5456=FACE_OUTER_BOUND ( 'NONE', #17221, .T. ) ;
#5460=ORIENTED_EDGE ( 'NONE', *, *, #14977, .F. ) ;
#5461=( BOUNDED_CURVE ( )  B_SPLINE_CURVE ( 2, ( #29779, #6743, #1983, #21451, #26185, #11546, #28489, #23043, #382 ),
 .UNSPECIFIED., .F., .F. ) 
 B_SPLINE_CURVE_WITH_KNOTS ( ( 3, 2, 2, 2, 3 ),
 ( 0.2527777777777777679, 0.2537037037037037090, 0.2555555555555555358, 0.2574074074074074181, 0.2583333333333333037 ),
 .UNSPECIFIED. ) 
 CURVE ( )  GEOMETRIC_REPRESENTATION_ITEM ( )  RATIONAL_B_SPLINE_CURVE ( ( 0.9330127018922194093, 0.9330127018922194093, 1.000000000000000000, 0.8660254037844388186, 1.000000000000000000, 0.8660254037844388186, 1.000000000000000000, 0.9330127018922214077, 0.9330127018922194093 ) ) 
 REPRESENTATION_ITEM ( '' )  );
#5462=CARTESIAN_POINT ( 'NONE',  ( 3.175426480543072749, 5.499999999999865885, -103.6250000000000142 ) ) ;
#5464=CARTESIAN_POINT ( 'NONE',  ( 7.216878364870455975, -6.409875621278545621E-14, -125.3080127018922099 ) ) ;
#5465=EDGE_LOOP ( 'NONE', ( #11801, #2141, #25296, #16813 ) ) ;
#5467=CARTESIAN_POINT ( 'NONE',  ( -3.608439182435052128, -6.250000000000110134, -163.9419872981077901 ) ) ;
#5470=CARTESIAN_POINT ( 'NONE',  ( 6.000000000000000888, -1.859271017917181981E-14, -63.66367513459483973 ) ) ;
#5472=VECTOR ( 'NONE', #29121, 1000.000000000000000 ) ;
#5473=CARTESIAN_POINT ( 'NONE',  ( -3.608439182435052128, -6.250000000000110134, -61.30801270189223828 ) ) ;
#5474=ORIENTED_EDGE ( 'NONE', *, *, #5000, .F. ) ;
#5475=CARTESIAN_POINT ( 'NONE',  ( 6.000000000000000888, -1.859271017917181981E-14, -100.5863248654052171 ) ) ;
#5476=CARTESIAN_POINT ( 'NONE',  ( -5.920437777358313447, 9.270953676058804049, -24.00610273346770640 ) ) ;
#5478=CARTESIAN_POINT ( 'NONE',  ( -4.763139720814407951, 2.749999999999946709, -169.2500000000000000 ) ) ;
#5481=CARTESIAN_POINT ( 'NONE',  ( 3.608439182435180470, 6.249999999999982236, -168.5580127018922383 ) ) ;
#5484=CARTESIAN_POINT ( 'NONE',  ( -2.775557561562891351E-14, -5.500000000000115463, -119.2500000000000284 ) ) ;
#5487=CARTESIAN_POINT ( 'NONE',  ( -2.775557561562891351E-14, -5.500000000000115463, -116.2500000000000142 ) ) ;
#5488=CARTESIAN_POINT ( 'NONE',  ( 0.000000000000000000, 5.999999999999977796, -142.7886751345948255 ) ) ;
#5489=CARTESIAN_POINT ( 'NONE',  ( 6.000000000000000888, -1.859271017917181981E-14, -84.08632486540520290 ) ) ;
#5492=CARTESIAN_POINT ( 'NONE',  ( -5.196152422706601826, 2.999999999999975131, -168.0386751345947971 ) ) ;
#5493=ORIENTED_EDGE ( 'NONE', *, *, #22387, .F. ) ;
#5494=CARTESIAN_POINT ( 'NONE',  ( -5.999999999999956479, -1.607695154586745057, -127.3466878364870354 ) ) ;
#5495=CARTESIAN_POINT ( 'NONE',  ( 2.775557561562891351E-14, 6.250000000000033751, -83.56698729810784698 ) ) ;
#5496=VERTEX_POINT ( 'NONE', #7913 ) ;
#5500=( BOUNDED_CURVE ( )  B_SPLINE_CURVE ( 2, ( #29128, #17356, #1173, #3629, #10278, #29436, #8240, #24526, #22245 ),
 .UNSPECIFIED., .F., .T. ) 
 B_SPLINE_CURVE_WITH_KNOTS ( ( 3, 2, 2, 2, 3 ),
 ( 0.9861111111111111605, 0.9870370370370370461, 0.9888888888888889284, 0.9907407407407406996, 0.9916666666666665853 ),
 .UNSPECIFIED. ) 
 CURVE ( )  GEOMETRIC_REPRESENTATION_ITEM ( )  RATIONAL_B_SPLINE_CURVE ( ( 0.9330127018922194093, 0.9330127018922234061, 1.000000000000000000, 0.8660254037844388186, 1.000000000000000000, 0.8660254037844388186, 1.000000000000000000, 0.9330127018922234061, 0.9330127018922194093 ) ) 
 REPRESENTATION_ITEM ( '' )  );
#5504=CARTESIAN_POINT ( 'NONE',  ( -5.412658773652684552, -3.125000000000099920, -131.0669872981078470 ) ) ;
#5505=CARTESIAN_POINT ( 'NONE',  ( 0.000000000000000000, -5.999999999999991118, -135.4613248654051745 ) ) ;
#5509=ORIENTED_EDGE ( 'NONE', *, *, #10809, .T. ) ;
#5511=DIRECTION ( 'NONE',  ( -7.147005652999508048E-36, 5.642372883946980038E-36, 1.000000000000000000 ) ) ;
#5513=FACE_OUTER_BOUND ( 'NONE', #14492, .T. ) ;
#5514=( BOUNDED_CURVE ( )  B_SPLINE_CURVE ( 2, ( #12807, #10486, #26582, #19404, #19836, #26139, #5084, #2789, #17107 ),
 .UNSPECIFIED., .F., .T. ) 
 B_SPLINE_CURVE_WITH_KNOTS ( ( 3, 2, 2, 2, 3 ),
 ( 0.06388888888888888395, 0.06481481481481481122, 0.06666666666666666574, 0.06851851851851852027, 0.06944444444444444753 ),
 .UNSPECIFIED. ) 
 CURVE ( )  GEOMETRIC_REPRESENTATION_ITEM ( )  RATIONAL_B_SPLINE_CURVE ( ( 0.9330127018922194093, 0.9330127018922194093, 1.000000000000000000, 0.8660254037844388186, 1.000000000000000000, 0.8660254037844388186, 1.000000000000000000, 0.9330127018922194093, 0.9330127018922194093 ) ) 
 REPRESENTATION_ITEM ( '' )  );
#5518=FACE_OUTER_BOUND ( 'NONE', #7341, .T. ) ;
#5522=CARTESIAN_POINT ( 'NONE',  ( -3.175426480542816510, -5.500000000000057732, -138.8750000000000568 ) ) ;
#5524=EDGE_CURVE ( 'NONE', #23417, #226, #5966, .T. ) ;
#5528=CARTESIAN_POINT ( 'NONE',  ( 4.763139720814407951, 2.750000000000002665, -46.75000000000001421 ) ) ;
#5530=LINE ( 'NONE', #923, #17862 ) ;
#5535=CARTESIAN_POINT ( 'NONE',  ( 2.775557561562891351E-14, 6.250000000000033751, -95.56698729810780435 ) ) ;
#5536=CARTESIAN_POINT ( 'NONE',  ( -3.464101615137757051, -5.999999999999979572, -50.66367513459485394 ) ) ;
#5539=CARTESIAN_POINT ( 'NONE',  ( 6.000000000000000888, -1.859271017917181981E-14, -146.1636751345948255 ) ) ;
#5542=VECTOR ( 'NONE', #5996, 1000.000000000000000 ) ;
#5545=CARTESIAN_POINT ( 'NONE',  ( 3.175426480543072749, 5.499999999999865885, -58.62499999999998579 ) ) ;
#5548=CARTESIAN_POINT ( 'NONE',  ( 4.520452470708214321, 10.03252783106553103, -21.03609891486515338 ) ) ;
#5549=CARTESIAN_POINT ( 'NONE',  ( 2.775557561562891351E-14, 6.250000000000033751, -72.43301270189222407 ) ) ;
#5552=CARTESIAN_POINT ( 'NONE',  ( 6.000000000000001776, 5.345404176511898156E-15, -174.0863248654052313 ) ) ;
#5556=CARTESIAN_POINT ( 'NONE',  ( 4.763139720814407951, 2.750000000000002665, -142.7500000000000568 ) ) ;
#5557=CARTESIAN_POINT ( 'NONE',  ( -3.464101615137725076, 5.999999999999979572, -68.58632486540524553 ) ) ;
#5558=CARTESIAN_POINT ( 'NONE',  ( -5.412658773652739619, 3.124999999999975131, -151.6830127018922099 ) ) ;
#5559=CARTESIAN_POINT ( 'NONE',  ( 5.999999999999949374, 1.607695154586804565, -102.0193375672974128 ) ) ;
#5560=CARTESIAN_POINT ( 'NONE',  ( -3.464101615137725076, 5.999999999999979572, -51.16367513459485394 ) ) ;
#5561=CARTESIAN_POINT ( 'NONE',  ( 3.175426480543072749, 5.499999999999865885, -73.62500000000007105 ) ) ;
#5562=CARTESIAN_POINT ( 'NONE',  ( -3.175426480542816510, 5.499999999999865885, -53.87500000000003553 ) ) ;
#5564=ORIENTED_EDGE ( 'NONE', *, *, #17253, .F. ) ;
#5567=CARTESIAN_POINT ( 'NONE',  ( -5.196152422706601826, 2.999999999999975131, -133.5386751345948255 ) ) ;
#5573=CARTESIAN_POINT ( 'NONE',  ( 5.412658773652712085, -3.125000000000086153, -46.56698729810781856 ) ) ;
#5575=CARTESIAN_POINT ( 'NONE',  ( -3.608439182435115633, 6.249999999999965361, -149.4419872981077901 ) ) ;
#5576=ORIENTED_EDGE ( 'NONE', *, *, #21518, .F. ) ;
#5577=CARTESIAN_POINT ( 'NONE',  ( -3.175426480542816510, 5.499999999999865885, -77.87500000000001421 ) ) ;
#5581=CARTESIAN_POINT ( 'NONE',  ( 2.775557561562891351E-14, 6.250000000000033751, -93.43301270189225249 ) ) ;
#5584=CARTESIAN_POINT ( 'NONE',  ( 0.7970850910875092454, -10.97816267869983342, -19.03975521967169016 ) ) ;
#5588=CARTESIAN_POINT ( 'NONE',  ( -4.763139720814407951, -2.750000000000016431, -163.0000000000000284 ) ) ;
#5590=CARTESIAN_POINT ( 'NONE',  ( -3.175426480542816510, -5.500000000000057732, -146.3750000000000284 ) ) ;
#5593=CARTESIAN_POINT ( 'NONE',  ( -6.350852961085760029, -1.281975124255709124E-13, -94.12500000000001421 ) ) ;
#5594=CARTESIAN_POINT ( 'NONE',  ( -3.464101615137725076, 5.999999999999979572, -125.5863248654051887 ) ) ;
#5595=CARTESIAN_POINT ( 'NONE',  ( -5.196152422706573404, -3.000000000000002665, -131.2113248654052029 ) ) ;
#5596=CARTESIAN_POINT ( 'NONE',  ( 0.000000000000000000, 5.499999999999991118, -79.50000000000001421 ) ) ;
#5599=CARTESIAN_POINT ( 'NONE',  ( 5.196152422706629359, 3.000000000000002665, -65.03867513459482552 ) ) ;
#5600=CARTESIAN_POINT ( 'NONE',  ( 0.000000000000000000, 0.000000000000000000, -44.99152654425658682 ) ) ;
#5602=CARTESIAN_POINT ( 'NONE',  ( 0.000000000000000000, 0.000000000000000000, 0.000000000000000000 ) ) ;
#5603=CARTESIAN_POINT ( 'NONE',  ( 5.196152422706629359, 3.000000000000002665, -78.53867513459483973 ) ) ;
#5604=ORIENTED_EDGE ( 'NONE', *, *, #5140, .F. ) ;
#5610=ORIENTED_EDGE ( 'NONE', *, *, #14882, .F. ) ;
#5612=CARTESIAN_POINT ( 'NONE',  ( 3.175426480543072749, -5.500000000000105693, -104.1250000000000142 ) ) ;
#5615=CARTESIAN_POINT ( 'NONE',  ( 3.608439182435180470, 6.249999999999982236, -114.5580127018922241 ) ) ;
#5618=CARTESIAN_POINT ( 'NONE',  ( 3.608439182435180470, 6.249999999999982236, -161.6919872981078470 ) ) ;
#5621=CARTESIAN_POINT ( 'NONE',  ( -5.412658773652684552, -3.125000000000099920, -59.93301270189221697 ) ) ;
#5622=EDGE_LOOP ( 'NONE', ( #21711, #25592, #14757, #7921 ) ) ;
#5625=CARTESIAN_POINT ( 'NONE',  ( -5.608370619328715279, 9.463293048187475520, -22.85879529262371079 ) ) ;
#5627=CARTESIAN_POINT ( 'NONE',  ( 0.000000000000000000, 5.499999999999991118, -172.5000000000000000 ) ) ;
#5630=CARTESIAN_POINT ( 'NONE',  ( 2.775557561562891351E-14, 6.250000000000033751, -165.4330127018922667 ) ) ;
#5633=VECTOR ( 'NONE', #11216, 1000.000000000000000 ) ;
#5634=CARTESIAN_POINT ( 'NONE',  ( 3.175426480543072749, -5.500000000000105693, -113.1249999999999858 ) ) ;
#5636=CARTESIAN_POINT ( 'NONE',  ( 3.175426480543072749, 5.499999999999865885, -103.6250000000000142 ) ) ;
#5639=CYLINDRICAL_SURFACE ( 'NONE', #22033, 6.000000000000000888 ) ;
#5644=CARTESIAN_POINT ( 'NONE',  ( 6.000000000000052403, -1.607695154586662678, -71.23066243270258724 ) ) ;
#5648=CARTESIAN_POINT ( 'NONE',  ( 3.608439182435180470, -6.249999999999997335, -85.69198729810781856 ) ) ;
#5649=( BOUNDED_CURVE ( )  B_SPLINE_CURVE ( 2, ( #27160, #17841, #10925, #25007, #11388, #20575, #29925, #13387, #6422 ),
 .UNSPECIFIED., .F., .F. ) 
 B_SPLINE_CURVE_WITH_KNOTS ( ( 3, 2, 2, 2, 3 ),
 ( 0.1527777777777777901, 0.1537037037037037035, 0.1555555555555555580, 0.1574074074074074125, 0.1583333333333333259 ),
 .UNSPECIFIED. ) 
 CURVE ( )  GEOMETRIC_REPRESENTATION_ITEM ( )  RATIONAL_B_SPLINE_CURVE ( ( 0.9330127018922194093, 0.9330127018922204085, 1.000000000000000000, 0.8660254037844388186, 1.000000000000000000, 0.8660254037844388186, 1.000000000000000000, 0.9330127018922205195, 0.9330127018922196314 ) ) 
 REPRESENTATION_ITEM ( '' )  );
#5652=ORIENTED_EDGE ( 'NONE', *, *, #23751, .F. ) ;
#5657=CARTESIAN_POINT ( 'NONE',  ( 7.216878364870455975, -6.409875621278545621E-14, -134.9419872981077901 ) ) ;
#5659=CARTESIAN_POINT ( 'NONE',  ( 6.000000000000000888, 1.607695154586715303, -84.01933756729741276 ) ) ;
#5663=DIRECTION ( 'NONE',  ( 1.000000000000000000, -5.551115123125773458E-17, -1.260129944081490338E-35 ) ) ;
#5667=CARTESIAN_POINT ( 'NONE',  ( -7.216878364870328078, 0.000000000000000000, -66.69198729810779014 ) ) ;
#5668=VECTOR ( 'NONE', #666, 1000.000000000000000 ) ;
#5669=CARTESIAN_POINT ( 'NONE',  ( -3.608439182435052128, -6.250000000000110134, -52.94198729810779014 ) ) ;
#5671=CARTESIAN_POINT ( 'NONE',  ( -5.999999999999963585, -1.487416814333745711E-14, -127.4136751345948113 ) ) ;
#5672=CARTESIAN_POINT ( 'NONE',  ( -2.775557561562891351E-14, -5.500000000000115463, -128.2500000000000284 ) ) ;
#5673=DIRECTION ( 'NONE',  ( 1.000000000000000000, -5.551115123125773458E-17, -1.260129944081490338E-35 ) ) ;
#5676=CARTESIAN_POINT ( 'NONE',  ( -5.999999999999866773, 1.607695154586893826, -119.4033121635130215 ) ) ;
#5679=ORIENTED_EDGE ( 'NONE', *, *, #384, .F. ) ;
#5683=ADVANCED_FACE ( 'NONE', ( #4065 ), #22678, .T. ) ;
#5684=CARTESIAN_POINT ( 'NONE',  ( 7.216878364870455975, -6.409875621278545621E-14, -97.44198729810781856 ) ) ;
#5685=CARTESIAN_POINT ( 'NONE',  ( 0.000000000000000000, -5.999999999999991118, -78.46132486540524553 ) ) ;
#5691=EDGE_CURVE ( 'NONE', #16117, #1801, #22859, .T. ) ;
#5696=CARTESIAN_POINT ( 'NONE',  ( -3.175426480542816510, -5.500000000000057732, -48.87500000000001421 ) ) ;
#5698=VECTOR ( 'NONE', #21580, 1000.000000000000000 ) ;
#5700=DIRECTION ( 'NONE',  ( -7.147005652999508048E-36, 5.642372883946980038E-36, 1.000000000000000000 ) ) ;
#5701=CARTESIAN_POINT ( 'NONE',  ( -3.608439182435052128, -6.250000000000110134, -77.80801270189225249 ) ) ;
#5702=FACE_OUTER_BOUND ( 'NONE', #19699, .T. ) ;
#5704=CARTESIAN_POINT ( 'NONE',  ( 5.999999999999949374, 1.607695154586804565, -169.5193375672974696 ) ) ;
#5705=CARTESIAN_POINT ( 'NONE',  ( -5.999999999999963585, 9.296355089585909904E-15, -168.8363248654052029 ) ) ;
#5706=CYLINDRICAL_SURFACE ( 'NONE', #29489, 6.000000000000000888 ) ;
#5707=CARTESIAN_POINT ( 'NONE',  ( -2.775557561562891351E-14, -5.500000000000115463, -135.7500000000000284 ) ) ;
#5709=CARTESIAN_POINT ( 'NONE',  ( -5.999999999999971578, 1.607695154586715303, -101.4033121635129930 ) ) ;
#5710=CARTESIAN_POINT ( 'NONE',  ( 6.000000000000000888, -1.607695154586752384, -72.73066243270262987 ) ) ;
#5711=CARTESIAN_POINT ( 'NONE',  ( 4.763139720814407951, 2.750000000000002665, -69.25000000000002842 ) ) ;
#5712=CARTESIAN_POINT ( 'NONE',  ( -3.175426480542816510, -5.500000000000057732, -59.37500000000005684 ) ) ;
#5714=VERTEX_POINT ( 'NONE', #6074 ) ;
#5716=CARTESIAN_POINT ( 'NONE',  ( -5.999999999999963585, 1.780251999655701777E-13, -89.91367513459485394 ) ) ;
#5719=CARTESIAN_POINT ( 'NONE',  ( -5.999999999999963585, 1.780251999655701777E-13, -58.41367513459482552 ) ) ;
#5721=ORIENTED_EDGE ( 'NONE', *, *, #29940, .F. ) ;
#5726=CARTESIAN_POINT ( 'NONE',  ( -4.763139720814407951, -2.750000000000016431, -143.5000000000000284 ) ) ;
#5727=CARTESIAN_POINT ( 'NONE',  ( 0.000000000000000000, 5.499999999999991118, -181.5000000000000000 ) ) ;
#5730=CARTESIAN_POINT ( 'NONE',  ( 2.775557561562891351E-14, 6.250000000000033751, -145.0669872981078470 ) ) ;
#5731=CARTESIAN_POINT ( 'NONE',  ( -4.763139720814407951, 2.749999999999946709, -77.74999999999998579 ) ) ;
#5733=CARTESIAN_POINT ( 'NONE',  ( 5.412658773652712085, -3.125000000000086153, -95.43301270189225249 ) ) ;
#5734=ORIENTED_EDGE ( 'NONE', *, *, #7157, .T. ) ;
#5736=DIRECTION ( 'NONE',  ( -7.147005652999508048E-36, 5.642372883946980038E-36, 1.000000000000000000 ) ) ;
#5738=CARTESIAN_POINT ( 'NONE',  ( 6.000000000000052403, -1.607695154586662678, -90.73066243270264408 ) ) ;
#5739=CARTESIAN_POINT ( 'NONE',  ( 3.464101615137757051, -5.999999999999979572, -58.83632486540520290 ) ) ;
#5742=CARTESIAN_POINT ( 'NONE',  ( -6.350852961085760029, -1.281975124255709124E-13, -152.6250000000000284 ) ) ;
#5743=CARTESIAN_POINT ( 'NONE',  ( 3.175426480543072749, 5.499999999999865885, -144.1250000000000000 ) ) ;
#5744=FACE_OUTER_BOUND ( 'NONE', #14861, .T. ) ;
#5746=CARTESIAN_POINT ( 'NONE',  ( -4.763139720814407951, 2.749999999999946709, -79.25000000000004263 ) ) ;
#5749=CARTESIAN_POINT ( 'NONE',  ( -3.464101615137725076, 5.999999999999979572, -131.5863248654052313 ) ) ;
#5751=CARTESIAN_POINT ( 'NONE',  ( -3.464101615137757051, -5.999999999999979572, -165.5863248654052029 ) ) ;
#5753=CARTESIAN_POINT ( 'NONE',  ( 6.000000000000000888, 1.607695154586715303, -72.59668783648704959 ) ) ;
#5754=EDGE_CURVE ( 'NONE', #1086, #11750, #4655, .T. ) ;
#5756=CARTESIAN_POINT ( 'NONE',  ( -5.999999999999968026, -1.607695154586722186, -157.3466878364870070 ) ) ;
#5757=CARTESIAN_POINT ( 'NONE',  ( -5.196152422706573404, -3.000000000000002665, -79.28867513459481131 ) ) ;
#5761=ORIENTED_EDGE ( 'NONE', *, *, #26226, .T. ) ;
#5762=VECTOR ( 'NONE', #27532, 1000.000000000000000 ) ;
#5764=CARTESIAN_POINT ( 'NONE',  ( 3.175426480543072749, -5.500000000000105693, -108.6250000000000284 ) ) ;
#5766=CARTESIAN_POINT ( 'NONE',  ( -5.412658773652739619, 3.124999999999975131, -118.6830127018922383 ) ) ;
#5769=CARTESIAN_POINT ( 'NONE',  ( -5.412658773652739619, 3.124999999999975131, -156.8169872981078470 ) ) ;
#5770=CARTESIAN_POINT ( 'NONE',  ( -6.000000000000000888, 1.067854986875958443E-15, 7.560779664488942560E-35 ) ) ;
#5775=( BOUNDED_CURVE ( )  B_SPLINE_CURVE ( 2, ( #19636, #19193, #26523, #19346, #28665, #16903, #28522, #7492, #7639 ),
 .UNSPECIFIED., .F., .T. ) 
 B_SPLINE_CURVE_WITH_KNOTS ( ( 3, 2, 2, 2, 3 ),
 ( 0.6361111111111110716, 0.6370370370370370683, 0.6388888888888888395, 0.6407407407407407218, 0.6416666666666666075 ),
 .UNSPECIFIED. ) 
 CURVE ( )  GEOMETRIC_REPRESENTATION_ITEM ( )  RATIONAL_B_SPLINE_CURVE ( ( 0.9330127018922194093, 0.9330127018922154125, 1.000000000000000000, 0.8660254037844388186, 1.000000000000000000, 0.8660254037844388186, 1.000000000000000000, 0.9330127018922234061, 0.9330127018922194093 ) ) 
 REPRESENTATION_ITEM ( '' )  );
#5777=CARTESIAN_POINT ( 'NONE',  ( 3.175426480543072749, 5.499999999999865885, -168.1250000000000000 ) ) ;
#5779=CARTESIAN_POINT ( 'NONE',  ( 7.216878364870455975, -6.409875621278545621E-14, -171.8080127018922667 ) ) ;
#5782=CARTESIAN_POINT ( 'NONE',  ( 3.175426480543072749, 5.499999999999865885, -114.1249999999999858 ) ) ;
#5784=CARTESIAN_POINT ( 'NONE',  ( 3.175426480543072749, 5.499999999999865885, -105.1250000000000284 ) ) ;
#5785=CARTESIAN_POINT ( 'NONE',  ( 5.999999999999988454, 1.607695154586737729, -152.0966878364870638 ) ) ;
#5786=CARTESIAN_POINT ( 'NONE',  ( -5.196152422706601826, 2.999999999999975131, -117.9613248654052313 ) ) ;
#5791=EDGE_CURVE ( 'NONE', #25744, #1672, #15626, .T. ) ;
#5792=EDGE_LOOP ( 'NONE', ( #23597, #17827, #10147, #3954 ) ) ;
#5793=CARTESIAN_POINT ( 'NONE',  ( 3.175426480543072749, -5.500000000000105693, -159.6250000000000284 ) ) ;
#5794=CARTESIAN_POINT ( 'NONE',  ( 5.196152422706629359, 3.000000000000002665, -156.5386751345948539 ) ) ;
#5796=CARTESIAN_POINT ( 'NONE',  ( 3.608439182435180470, -6.249999999999997335, -78.19198729810784698 ) ) ;
#5803=CARTESIAN_POINT ( 'NONE',  ( -7.216878364870328078, 0.000000000000000000, -139.5580127018922099 ) ) ;
#5805=AXIS2_PLACEMENT_3D ( 'NONE', #29981, #29829, #27663 ) ;
#5806=CARTESIAN_POINT ( 'NONE',  ( 5.412658773652739619, 3.124999999999988898, -130.3169872981078186 ) ) ;
#5807=CARTESIAN_POINT ( 'NONE',  ( 3.175426480543072749, -5.500000000000105693, -171.6250000000000284 ) ) ;
#5808=CARTESIAN_POINT ( 'NONE',  ( -5.999999999999963585, 8.134310703387671600E-14, -130.4136751345948539 ) ) ;
#5809=EDGE_LOOP ( 'NONE', ( #12518, #15049, #23957, #17991 ) ) ;
#5812=CARTESIAN_POINT ( 'NONE',  ( 5.999999999999988454, 1.607695154586737729, -164.0966878364870070 ) ) ;
#5814=CARTESIAN_POINT ( 'NONE',  ( -5.999999999999963585, 1.780251999655701777E-13, -89.91367513459485394 ) ) ;
#5815=CARTESIAN_POINT ( 'NONE',  ( 3.464101615137757051, -5.999999999999979572, -107.4136751345947971 ) ) ;
#5816=CARTESIAN_POINT ( 'NONE',  ( -5.999999999999963585, 1.780251999655701777E-13, -47.33632486540523132 ) ) ;
#5817=CARTESIAN_POINT ( 'NONE',  ( -5.412658773652684552, -3.125000000000099920, -71.06698729810784698 ) ) ;
#5818=CARTESIAN_POINT ( 'NONE',  ( -5.412658773652684552, -3.125000000000099920, -54.56698729810782567 ) ) ;
#5819=EDGE_CURVE ( 'NONE', #2096, #5313, #11307, .T. ) ;
#5823=CARTESIAN_POINT ( 'NONE',  ( 3.175426480543072749, 5.499999999999865885, -127.6249999999999858 ) ) ;
#5824=CYLINDRICAL_SURFACE ( 'NONE', #23039, 6.000000000000000888 ) ;
#5826=ORIENTED_EDGE ( 'NONE', *, *, #3030, .T. ) ;
#5827=DIRECTION ( 'NONE',  ( -7.147005652999508048E-36, 5.642372883946980038E-36, 1.000000000000000000 ) ) ;
#5828=( BOUNDED_CURVE ( )  B_SPLINE_CURVE ( 2, ( #18485, #11434, #27200, #4161, #30126, #15588, #6316, #24903, #8947 ),
 .UNSPECIFIED., .F., .F. ) 
 B_SPLINE_CURVE_WITH_KNOTS ( ( 3, 2, 2, 2, 3 ),
 ( 0.4527777777777777790, 0.4537037037037037202, 0.4555555555555555469, 0.4574074074074074292, 0.4583333333333333148 ),
 .UNSPECIFIED. ) 
 CURVE ( )  GEOMETRIC_REPRESENTATION_ITEM ( )  RATIONAL_B_SPLINE_CURVE ( ( 0.9330127018922194093, 0.9330127018922194093, 1.000000000000000000, 0.8660254037844388186, 1.000000000000000000, 0.8660254037844388186, 1.000000000000000000, 0.9330127018922214077, 0.9330127018922194093 ) ) 
 REPRESENTATION_ITEM ( '' )  );
#5831=CARTESIAN_POINT ( 'NONE',  ( -5.999999999999971578, 1.607695154586715303, -96.90331216351299304 ) ) ;
#5832=CARTESIAN_POINT ( 'NONE',  ( -6.000000000000007105, -1.607695154586655129, -100.3466878364870496 ) ) ;
#5833=CARTESIAN_POINT ( 'NONE',  ( 3.464101615137757051, -5.999999999999979572, -144.3363248654052029 ) ) ;
#5835=ORIENTED_EDGE ( 'NONE', *, *, #3679, .T. ) ;
#5837=DIRECTION ( 'NONE',  ( -7.147005652999508048E-36, 5.642372883946980038E-36, 1.000000000000000000 ) ) ;
#5839=CARTESIAN_POINT ( 'NONE',  ( 5.412658773652739619, 3.124999999999988898, -94.31698729810783277 ) ) ;
#5840=CARTESIAN_POINT ( 'NONE',  ( 6.000000000000000888, -1.607695154586752384, -54.15331216351300014 ) ) ;
#5843=CYLINDRICAL_SURFACE ( 'NONE', #21353, 6.000000000000000888 ) ;
#5847=VECTOR ( 'NONE', #22516, 1000.000000000000000 ) ;
#5850=CARTESIAN_POINT ( 'NONE',  ( -7.216878364870328078, 0.000000000000000000, -73.55801270189223828 ) ) ;
#5855=PRESENTATION_STYLE_ASSIGNMENT (( #20173 ) ) ;
#5859=CARTESIAN_POINT ( 'NONE',  ( -6.350852961085760029, -1.281975124255709124E-13, -136.1250000000000568 ) ) ;
#5861=CARTESIAN_POINT ( 'NONE',  ( 5.196152422706629359, 3.000000000000002665, -101.9613248654052171 ) ) ;
#5863=CARTESIAN_POINT ( 'NONE',  ( -6.350852961085760029, -1.281975124255709124E-13, -59.62500000000000000 ) ) ;
#5865=CARTESIAN_POINT ( 'NONE',  ( 0.000000000000000000, 5.499999999999991118, -55.49999999999999289 ) ) ;
#5866=( BOUNDED_CURVE ( )  B_SPLINE_CURVE ( 2, ( #20360, #8374, #8207, #13333, #17623, #18084, #6070, #8846, #11164 ),
 .UNSPECIFIED., .F., .T. ) 
 B_SPLINE_CURVE_WITH_KNOTS ( ( 3, 2, 2, 2, 3 ),
 ( 0.7083333333333333703, 0.7092592592592592560, 0.7111111111111111382, 0.7129629629629630205, 0.7138888888888887951 ),
 .UNSPECIFIED. ) 
 CURVE ( )  GEOMETRIC_REPRESENTATION_ITEM ( )  RATIONAL_B_SPLINE_CURVE ( ( 0.9330127018922194093, 0.9330127018922194093, 1.000000000000000000, 0.8660254037844388186, 1.000000000000000000, 0.8660254037844388186, 1.000000000000000000, 0.9330127018922274029, 0.9330127018922194093 ) ) 
 REPRESENTATION_ITEM ( '' )  );
#5868=ORIENTED_EDGE ( 'NONE', *, *, #12748, .F. ) ;
#5871=CARTESIAN_POINT ( 'NONE',  ( 6.000000000000000888, -1.607695154586752384, -88.65331216351300725 ) ) ;
#5875=AXIS2_PLACEMENT_3D ( 'NONE', #13548, #1830, #24561 ) ;
#5879=CARTESIAN_POINT ( 'NONE',  ( -4.763139720814407951, -2.750000000000016431, -149.5000000000000284 ) ) ;
#5881=EDGE_LOOP ( 'NONE', ( #21804, #22423, #18656, #19364 ) ) ;
#5882=CARTESIAN_POINT ( 'NONE',  ( 3.608439182435180470, 6.249999999999982236, -148.1919872981077901 ) ) ;
#5883=CARTESIAN_POINT ( 'NONE',  ( -2.775557561562891351E-14, -5.500000000000115463, -71.25000000000002842 ) ) ;
#5884=CARTESIAN_POINT ( 'NONE',  ( 2.775557561562891351E-14, -6.250000000000061284, -94.18301270189222407 ) ) ;
#5885=ORIENTED_EDGE ( 'NONE', *, *, #24185, .F. ) ;
#5886=CARTESIAN_POINT ( 'NONE',  ( 0.000000000000000000, -5.999999999999991118, -127.9613248654052313 ) ) ;
#5887=EDGE_CURVE ( 'NONE', #16367, #8576, #11469, .T. ) ;
#5888=CARTESIAN_POINT ( 'NONE',  ( 5.196152422706629359, -2.999999999999988898, -96.21132486540523132 ) ) ;
#5889=CARTESIAN_POINT ( 'NONE',  ( -6.000000000000000888, 1.067854986875958443E-15, 7.560779664488942560E-35 ) ) ;
#5892=CARTESIAN_POINT ( 'NONE',  ( 4.763139720814407951, -2.749999999999988454, -158.0000000000000284 ) ) ;
#5893=DIRECTION ( 'NONE',  ( -7.147005652999508048E-36, 5.642372883946980038E-36, 1.000000000000000000 ) ) ;
#5894=CARTESIAN_POINT ( 'NONE',  ( -4.763139720814407951, 2.749999999999946709, -145.2500000000000000 ) ) ;
#5895=CARTESIAN_POINT ( 'NONE',  ( -3.606777763894024602, 4.527305315996938972, -180.0000000000000853 ) ) ;
#5896=CARTESIAN_POINT ( 'NONE',  ( -5.999999999999956479, -1.607695154586745057, -92.84668783648702117 ) ) ;
#5897=CARTESIAN_POINT ( 'NONE',  ( -6.350852961085760029, -1.281975124255709124E-13, -83.62499999999997158 ) ) ;
#5901=CARTESIAN_POINT ( 'NONE',  ( -6.350852961085760029, -1.281975124255709124E-13, -80.62500000000004263 ) ) ;
#5903=FACE_OUTER_BOUND ( 'NONE', #26428, .T. ) ;
#5905=CARTESIAN_POINT ( 'NONE',  ( -5.196152422706601826, 2.999999999999975131, -103.5386751345947971 ) ) ;
#5912=FACE_OUTER_BOUND ( 'NONE', #16925, .T. ) ;
#5914=AXIS2_PLACEMENT_3D ( 'NONE', #7716, #24445, #24156 ) ;
#5915=CARTESIAN_POINT ( 'NONE',  ( 5.196152422706629359, -2.999999999999988898, -115.7113248654052455 ) ) ;
#5921=CARTESIAN_POINT ( 'NONE',  ( 6.350852961086080661, -9.614813431917819062E-14, -94.87500000000004263 ) ) ;
#5923=CARTESIAN_POINT ( 'NONE',  ( -5.412658773652684552, -3.125000000000099920, -112.4330127018922099 ) ) ;
#5924=ORIENTED_EDGE ( 'NONE', *, *, #26577, .T. ) ;
#5925=CARTESIAN_POINT ( 'NONE',  ( -5.999999999999963585, 1.780251999655701777E-13, -91.41367513459486815 ) ) ;
#5926=DIRECTION ( 'NONE',  ( -7.147005652999508048E-36, 5.642372883946980038E-36, 1.000000000000000000 ) ) ;
#5929=CARTESIAN_POINT ( 'NONE',  ( -5.412658773652739619, 3.124999999999975131, -49.68301270189223828 ) ) ;
#5930=EDGE_LOOP ( 'NONE', ( #8625, #11809, #727, #4548 ) ) ;
#5931=CARTESIAN_POINT ( 'NONE',  ( 0.000000000000000000, 5.999999999999977796, -153.2886751345948824 ) ) ;
#5932=ADVANCED_FACE ( 'NONE', ( #21714 ), #5250, .T. ) ;
#5934=CARTESIAN_POINT ( 'NONE',  ( 3.464101615137757051, -5.999999999999979572, -61.83632486540521001 ) ) ;
#5936=CARTESIAN_POINT ( 'NONE',  ( -6.350852961085760029, -1.281975124255709124E-13, -169.1249999999999716 ) ) ;
#5939=CARTESIAN_POINT ( 'NONE',  ( -5.412658773652739619, 3.124999999999975131, -169.6830127018922383 ) ) ;
#5941=AXIS2_PLACEMENT_3D ( 'NONE', #26812, #22392, #29123 ) ;
#5942=CARTESIAN_POINT ( 'NONE',  ( -4.763139720814407951, -2.750000000000016431, -110.5000000000000426 ) ) ;
#5944=CARTESIAN_POINT ( 'NONE',  ( 3.175426480543072749, -5.500000000000105693, -107.1250000000000284 ) ) ;
#5945=CARTESIAN_POINT ( 'NONE',  ( -5.999999999999963585, -1.487416814333745711E-14, -87.83632486540521711 ) ) ;
#5954=AXIS2_PLACEMENT_3D ( 'NONE', #3298, #11719, #11878 ) ;
#5955=CARTESIAN_POINT ( 'NONE',  ( -3.608439182435052128, -6.250000000000110134, -84.44198729810780435 ) ) ;
#5957=CARTESIAN_POINT ( 'NONE',  ( -3.464101615137757051, -5.999999999999979572, -103.1636751345948397 ) ) ;
#5958=VERTEX_POINT ( 'NONE', #3094 ) ;
#5959=DIRECTION ( 'NONE',  ( 1.000000000000000000, -5.551115123125773458E-17, -1.260129944081490338E-35 ) ) ;
#5961=ORIENTED_EDGE ( 'NONE', *, *, #13476, .T. ) ;
#5964=AXIS2_PLACEMENT_3D ( 'NONE', #28616, #9920, #10369 ) ;
#5965=CARTESIAN_POINT ( 'NONE',  ( 0.000000000000000000, 5.499999999999991118, -132.0000000000000000 ) ) ;
#5966=( BOUNDED_CURVE ( )  B_SPLINE_CURVE ( 2, ( #19753, #5753, #28645, #12726, #26643, #15164, #26495, #12134, #21477 ),
 .UNSPECIFIED., .F., .F. ) 
 B_SPLINE_CURVE_WITH_KNOTS ( ( 3, 2, 2, 2, 3 ),
 ( 0.8083333333333333481, 0.8092592592592592338, 0.8111111111111111160, 0.8129629629629629983, 0.8138888888888888840 ),
 .UNSPECIFIED. ) 
 CURVE ( )  GEOMETRIC_REPRESENTATION_ITEM ( )  RATIONAL_B_SPLINE_CURVE ( ( 0.9330127018922194093, 0.9330127018922194093, 1.000000000000000000, 0.8660254037844388186, 1.000000000000000000, 0.8660254037844388186, 1.000000000000000000, 0.9330127018922194093, 0.9330127018922194093 ) ) 
 REPRESENTATION_ITEM ( '' )  );
#5967=CARTESIAN_POINT ( 'NONE',  ( 5.412658773652739619, 3.124999999999988898, -141.6830127018922099 ) ) ;
#5970=CARTESIAN_POINT ( 'NONE',  ( 2.775557561562891351E-14, -6.250000000000061284, -121.8169872981078612 ) ) ;
#5972=CARTESIAN_POINT ( 'NONE',  ( -3.175426480542816510, 5.499999999999865885, -175.3750000000000568 ) ) ;
#5974=CARTESIAN_POINT ( 'NONE',  ( -6.000000000000000888, 1.067854986875958443E-15, 7.560779664488942560E-35 ) ) ;
#5976=EDGE_CURVE ( 'NONE', #2098, #22382, #7333, .T. ) ;
#5977=ORIENTED_EDGE ( 'NONE', *, *, #18630, .F. ) ;
#5980=EDGE_CURVE ( 'NONE', #23459, #22223, #28443, .T. ) ;
#5982=CARTESIAN_POINT ( 'NONE',  ( 5.196152422706629359, -2.999999999999988898, -107.2886751345948397 ) ) ;
#5985=CARTESIAN_POINT ( 'NONE',  ( 7.216878364870455975, -6.409875621278545621E-14, -64.44198729810784698 ) ) ;
#5986=CARTESIAN_POINT ( 'NONE',  ( 5.412658773652712085, -3.125000000000086153, -54.06698729810782567 ) ) ;
#5988=CARTESIAN_POINT ( 'NONE',  ( 6.000000000000026645, -1.607695154586707753, -128.2306624327026157 ) ) ;
#5991=CARTESIAN_POINT ( 'NONE',  ( 3.175426480543072749, 5.499999999999865885, -129.1250000000000284 ) ) ;
#5993=CARTESIAN_POINT ( 'NONE',  ( -3.464101615137725076, 5.999999999999979572, -157.6636751345948255 ) ) ;
#5994=FACE_OUTER_BOUND ( 'NONE', #5376, .T. ) ;
#5996=DIRECTION ( 'NONE',  ( -7.147005652999508048E-36, 5.642372883946980038E-36, 1.000000000000000000 ) ) ;
#5997=VERTEX_POINT ( 'NONE', #7113 ) ;
#5999=DIRECTION ( 'NONE',  ( -7.147005652999508048E-36, 5.642372883946980038E-36, 1.000000000000000000 ) ) ;
#6001=CARTESIAN_POINT ( 'NONE',  ( -3.608439182435115633, 6.249999999999965361, -113.4419872981078328 ) ) ;
#6002=CARTESIAN_POINT ( 'NONE',  ( -5.999999999999962697, -1.607695154586733954, -173.8466878364870354 ) ) ;
#6003=CARTESIAN_POINT ( 'NONE',  ( -5.999999999999963585, 1.780251999655701777E-13, -90.83632486540521711 ) ) ;
#6005=ORIENTED_EDGE ( 'NONE', *, *, #11079, .F. ) ;
#6007=EDGE_CURVE ( 'NONE', #16120, #24823, #8304, .T. ) ;
#6011=CARTESIAN_POINT ( 'NONE',  ( 3.175426480543072749, -5.500000000000105693, -47.12500000000006395 ) ) ;
#6013=CARTESIAN_POINT ( 'NONE',  ( 0.000000000000000000, 0.000000000000000000, 0.000000000000000000 ) ) ;
#6014=CARTESIAN_POINT ( 'NONE',  ( -5.999999999999963585, -1.487416814333745711E-14, -80.33632486540523132 ) ) ;
#6015=CARTESIAN_POINT ( 'NONE',  ( 5.412658773652712085, -3.125000000000086153, -77.43301270189223828 ) ) ;
#6016=EDGE_CURVE ( 'NONE', #21299, #1154, #3997, .T. ) ;
#6020=CARTESIAN_POINT ( 'NONE',  ( 5.999999999999993783, 1.607695154586726627, -177.5966878364870070 ) ) ;
#6021=CARTESIAN_POINT ( 'NONE',  ( -5.999999999999963585, 1.780251999655701777E-13, -99.83632486540521711 ) ) ;
#6022=CARTESIAN_POINT ( 'NONE',  ( 6.000000000000000888, 1.607695154586715303, -105.0193375672974554 ) ) ;
#6023=CARTESIAN_POINT ( 'NONE',  ( 4.763139720814407951, -2.749999999999988454, -131.0000000000000000 ) ) ;
#6025=FACE_OUTER_BOUND ( 'NONE', #13686, .T. ) ;
#6026=CARTESIAN_POINT ( 'NONE',  ( 0.000000000000000000, 5.999999999999977796, -178.2113248654052597 ) ) ;
#6027=EDGE_LOOP ( 'NONE', ( #12549, #12007, #25159, #342 ) ) ;
#6028=CARTESIAN_POINT ( 'NONE',  ( -3.175426480542816066, 5.499999999999865885, -65.87500000000002842 ) ) ;
#6029=CARTESIAN_POINT ( 'NONE',  ( -3.175426480542816510, 5.499999999999865885, -55.37500000000004263 ) ) ;
#6030=CARTESIAN_POINT ( 'NONE',  ( 3.464101615137852974, 5.999999999999884537, -170.8363248654052029 ) ) ;
#6041=ADVANCED_FACE ( 'NONE', ( #7556 ), #13628, .T. ) ;
#6043=ORIENTED_EDGE ( 'NONE', *, *, #22963, .F. ) ;
#6045=CARTESIAN_POINT ( 'NONE',  ( -3.175426480542816510, 5.499999999999865885, -146.8750000000000284 ) ) ;
#6048=ORIENTED_EDGE ( 'NONE', *, *, #5976, .F. ) ;
#6049=CARTESIAN_POINT ( 'NONE',  ( 4.763139720814407951, 2.750000000000002665, -76.74999999999998579 ) ) ;
#6052=CARTESIAN_POINT ( 'NONE',  ( 7.216878364870455975, -6.409875621278545621E-14, -92.30801270189225249 ) ) ;
#6056=DIRECTION ( 'NONE',  ( -7.147005652999508048E-36, 5.642372883946980038E-36, 1.000000000000000000 ) ) ;
#6057=CARTESIAN_POINT ( 'NONE',  ( 0.000000000000000000, -5.999999999999991118, -91.03867513459485394 ) ) ;
#6060=( BOUNDED_CURVE ( )  B_SPLINE_CURVE ( 2, ( #26350, #29094, #5599, #5299, #3296, #14712, #24055, #12421, #17784 ),
 .UNSPECIFIED., .F., .T. ) 
 B_SPLINE_CURVE_WITH_KNOTS ( ( 3, 2, 2, 2, 3 ),
 ( 0.8638888888888889284, 0.8648148148148148140, 0.8666666666666666963, 0.8685185185185184675, 0.8694444444444443532 ),
 .UNSPECIFIED. ) 
 CURVE ( )  GEOMETRIC_REPRESENTATION_ITEM ( )  RATIONAL_B_SPLINE_CURVE ( ( 0.9330127018922194093, 0.9330127018922234061, 1.000000000000000000, 0.8660254037844388186, 1.000000000000000000, 0.8660254037844388186, 1.000000000000000000, 0.9330127018922234061, 0.9330127018922194093 ) ) 
 REPRESENTATION_ITEM ( '' )  );
#6061=CARTESIAN_POINT ( 'NONE',  ( -4.763139720814407951, 2.749999999999946709, -155.7500000000000568 ) ) ;
#6062=CYLINDRICAL_SURFACE ( 'NONE', #766, 6.000000000000000888 ) ;
#6063=AXIS2_PLACEMENT_3D ( 'NONE', #25528, #6649, #16068 ) ;
#6064=DIRECTION ( 'NONE',  ( -7.147005652999508048E-36, 5.642372883946980038E-36, 1.000000000000000000 ) ) ;
#6066=CARTESIAN_POINT ( 'NONE',  ( -2.775557561562891351E-14, -5.500000000000115463, -87.75000000000000000 ) ) ;
#6068=CARTESIAN_POINT ( 'NONE',  ( 3.175426480543072749, -5.500000000000105693, -83.12500000000004263 ) ) ;
#6070=CARTESIAN_POINT ( 'NONE',  ( 5.196152422706629359, 3.000000000000002665, -142.4613248654052029 ) ) ;
#6073=CARTESIAN_POINT ( 'NONE',  ( -5.196152422706601826, 2.999999999999975131, -124.5386751345948255 ) ) ;
#6074=CARTESIAN_POINT ( 'NONE',  ( 6.000000000000000888, 7.762456499804235646E-14, -123.0863248654052313 ) ) ;
#6075=DIRECTION ( 'NONE',  ( -7.147005652999508048E-36, 5.642372883946980038E-36, 1.000000000000000000 ) ) ;
#6076=VERTEX_POINT ( 'NONE', #1404 ) ;
#6082=ORIENTED_EDGE ( 'NONE', *, *, #15662, .T. ) ;
#6083=CARTESIAN_POINT ( 'NONE',  ( -4.763139720814407951, -2.750000000000016431, -100.0000000000000284 ) ) ;
#6087=EDGE_CURVE ( 'NONE', #2251, #5496, #7148, .T. ) ;
#6088=CARTESIAN_POINT ( 'NONE',  ( 5.412658773652739619, 3.124999999999988898, -117.6830127018922383 ) ) ;
#6090=ORIENTED_EDGE ( 'NONE', *, *, #21156, .T. ) ;
#6091=CARTESIAN_POINT ( 'NONE',  ( 3.464101615137852974, 5.999999999999884537, -94.33632486540517448 ) ) ;
#6092=CARTESIAN_POINT ( 'NONE',  ( 6.000000000000000888, -3.330669073875464691E-16, -7.560779664488942560E-35 ) ) ;
#6093=CARTESIAN_POINT ( 'NONE',  ( -5.999999999999963585, 1.780251999655701777E-13, -62.91367513459483973 ) ) ;
#6094=CARTESIAN_POINT ( 'NONE',  ( 2.775557561562891351E-14, 6.250000000000033751, -55.93301270189221697 ) ) ;
#6100=CARTESIAN_POINT ( 'NONE',  ( 3.175426480543072749, -5.500000000000105693, -171.6250000000000284 ) ) ;
#6102=CARTESIAN_POINT ( 'NONE',  ( 3.464101615137852974, 5.999999999999884537, -107.8363248654052313 ) ) ;
#6103=CARTESIAN_POINT ( 'NONE',  ( -7.216878364870328078, 0.000000000000000000, -163.5580127018922099 ) ) ;
#6105=CARTESIAN_POINT ( 'NONE',  ( 3.175426480543072749, 5.499999999999865885, -112.6249999999999858 ) ) ;
#6107=CARTESIAN_POINT ( 'NONE',  ( 0.000000000000000000, 5.499999999999991118, -103.5000000000000426 ) ) ;
#6108=CARTESIAN_POINT ( 'NONE',  ( 5.196152422706629359, -2.999999999999988898, -111.7886751345948397 ) ) ;
#6110=CARTESIAN_POINT ( 'NONE',  ( -5.999999999999971578, 1.607695154586715303, -117.9033121635130072 ) ) ;
#6111=ORIENTED_EDGE ( 'NONE', *, *, #17010, .F. ) ;
#6114=FACE_OUTER_BOUND ( 'NONE', #7553, .T. ) ;
#6115=VERTEX_POINT ( 'NONE', #19702 ) ;
#6116=CARTESIAN_POINT ( 'NONE',  ( 6.350852961086080661, -9.614813431917819062E-14, -157.8750000000000000 ) ) ;
#6117=CARTESIAN_POINT ( 'NONE',  ( -5.412658773652684552, -3.125000000000099920, -80.06698729810779014 ) ) ;
#6120=ORIENTED_EDGE ( 'NONE', *, *, #11215, .T. ) ;
#6121=LINE ( 'NONE', #21962, #27718 ) ;
#6123=VERTEX_POINT ( 'NONE', #2334 ) ;
#6127=CARTESIAN_POINT ( 'NONE',  ( 4.763139720814407951, -2.749999999999988454, -120.5000000000000568 ) ) ;
#6128=EDGE_CURVE ( 'NONE', #91, #1235, #21227, .T. ) ;
#6129=CARTESIAN_POINT ( 'NONE',  ( 2.775557561562891351E-14, 6.250000000000033751, -135.4330127018922383 ) ) ;
#6132=CARTESIAN_POINT ( 'NONE',  ( -5.412658773652739619, 3.124999999999975131, -126.8169872981078612 ) ) ;
#6133=CARTESIAN_POINT ( 'NONE',  ( -5.999999999999963585, 8.134310703387671600E-14, -146.3363248654052313 ) ) ;
#6134=CARTESIAN_POINT ( 'NONE',  ( -3.175426480542816510, -5.500000000000057732, -170.3750000000000568 ) ) ;
#6138=CYLINDRICAL_SURFACE ( 'NONE', #8845, 6.000000000000000888 ) ;
#6141=CARTESIAN_POINT ( 'NONE',  ( 0.000000000000000000, 0.000000000000000000, 0.000000000000000000 ) ) ;
#6144=CARTESIAN_POINT ( 'NONE',  ( 3.608439182435180470, 6.249999999999982236, -65.69198729810780435 ) ) ;
#6145=CARTESIAN_POINT ( 'NONE',  ( -6.000000000000000888, 1.067854986875958443E-15, 7.560779664488942560E-35 ) ) ;
#6146=CARTESIAN_POINT ( 'NONE',  ( 6.000000000000000888, -1.607695154586752384, -63.73066243270262987 ) ) ;
#6149=CARTESIAN_POINT ( 'NONE',  ( 3.175426480543072749, -5.500000000000105693, -129.6250000000000284 ) ) ;
#6152=CARTESIAN_POINT ( 'NONE',  ( -5.196152422706573404, -3.000000000000002665, -119.2113248654052029 ) ) ;
#6157=ORIENTED_EDGE ( 'NONE', *, *, #21884, .F. ) ;
#6159=FACE_OUTER_BOUND ( 'NONE', #29428, .T. ) ;
#6161=CARTESIAN_POINT ( 'NONE',  ( -3.608439182435052128, -6.250000000000110134, -112.9419872981078186 ) ) ;
#6162=ADVANCED_FACE ( 'NONE', ( #28260 ), #7239, .T. ) ;
#6164=EDGE_CURVE ( 'NONE', #16384, #29310, #685, .T. ) ;
#6166=VECTOR ( 'NONE', #20213, 1000.000000000000000 ) ;
#6169=ORIENTED_EDGE ( 'NONE', *, *, #5980, .T. ) ;
#6173=AXIS2_PLACEMENT_3D ( 'NONE', #9912, #225, #9610 ) ;
#6174=CARTESIAN_POINT ( 'NONE',  ( 3.175426480543072749, 5.499999999999865885, -48.12500000000000000 ) ) ;
#6176=DIRECTION ( 'NONE',  ( -7.147005652999508048E-36, 5.642372883946980038E-36, 1.000000000000000000 ) ) ;
#6177=CARTESIAN_POINT ( 'NONE',  ( -7.216878364870328078, 0.000000000000000000, -66.05801270189226670 ) ) ;
#6178=CARTESIAN_POINT ( 'NONE',  ( 6.000000000000000888, 1.743066579297358182E-13, -81.66367513459481131 ) ) ;
#6180=CARTESIAN_POINT ( 'NONE',  ( 5.999999999999949374, 1.607695154586804565, -102.5966878364870780 ) ) ;
#6183=LINE ( 'NONE', #8161, #8396 ) ;
#6184=CARTESIAN_POINT ( 'NONE',  ( -3.175426480542816066, -5.500000000000057732, -134.3750000000000284 ) ) ;
#6186=ORIENTED_EDGE ( 'NONE', *, *, #22000, .F. ) ;
#6188=CARTESIAN_POINT ( 'NONE',  ( -3.175426480542816066, 5.499999999999865885, -62.87500000000001421 ) ) ;
#6189=CARTESIAN_POINT ( 'NONE',  ( -6.000000000000000888, 1.067854986875958443E-15, 7.560779664488942560E-35 ) ) ;
#6195=EDGE_CURVE ( 'NONE', #20877, #25219, #24253, .T. ) ;
#6196=ORIENTED_EDGE ( 'NONE', *, *, #10297, .T. ) ;
#6199=EDGE_LOOP ( 'NONE', ( #20071, #10414, #11424, #25587 ) ) ;
#6200=CARTESIAN_POINT ( 'NONE',  ( -6.350852961085760029, -1.281975124255709124E-13, -142.1250000000000000 ) ) ;
#6201=EDGE_LOOP ( 'NONE', ( #9682, #17910, #13654, #13534 ) ) ;
#6203=ORIENTED_EDGE ( 'NONE', *, *, #9114, .T. ) ;
#6204=CARTESIAN_POINT ( 'NONE',  ( 6.350852961086080661, -9.614813431917819062E-14, -70.87500000000004263 ) ) ;
#6206=CARTESIAN_POINT ( 'NONE',  ( -3.608439182435115633, 6.249999999999965361, -96.30801270189219565 ) ) ;
#6207=CARTESIAN_POINT ( 'NONE',  ( -1.000434615788078574, -10.95616177385589651, -19.08065934301228239 ) ) ;
#6208=CARTESIAN_POINT ( 'NONE',  ( 5.196152422706629359, 3.000000000000002665, -107.0386751345948682 ) ) ;
#6209=DIRECTION ( 'NONE',  ( 1.000000000000000000, -5.551115123125773458E-17, -1.260129944081490338E-35 ) ) ;
#6211=CARTESIAN_POINT ( 'NONE',  ( 3.464101615137757051, -5.999999999999979572, -64.83632486540523132 ) ) ;
#6213=CARTESIAN_POINT ( 'NONE',  ( -6.350852961085760029, -1.281975124255709124E-13, -155.6249999999999716 ) ) ;
#6215=CARTESIAN_POINT ( 'NONE',  ( -4.293779821584444711, 3.976156217467954779, -179.9999999999999147 ) ) ;
#6216=EDGE_CURVE ( 'NONE', #4423, #21660, #9313, .T. ) ;
#6218=CARTESIAN_POINT ( 'NONE',  ( -6.350852961085760029, -1.281975124255709124E-13, -85.12499999999998579 ) ) ;
#6221=CARTESIAN_POINT ( 'NONE',  ( -3.175426480542816510, -5.500000000000057732, -71.37499999999997158 ) ) ;
#6223=CARTESIAN_POINT ( 'NONE',  ( 0.000000000000000000, 0.000000000000000000, 0.000000000000000000 ) ) ;
#6224=CARTESIAN_POINT ( 'NONE',  ( 5.999999999999949374, 1.607695154586804565, -104.0966878364870638 ) ) ;
#6226=FACE_OUTER_BOUND ( 'NONE', #197, .T. ) ;
#6230=CARTESIAN_POINT ( 'NONE',  ( 3.464101615137757051, -5.999999999999979572, -171.9136751345948255 ) ) ;
#6235=CARTESIAN_POINT ( 'NONE',  ( -4.763139720814407951, -2.750000000000016431, -97.00000000000002842 ) ) ;
#6236=LINE ( 'NONE', #4077, #7238 ) ;
#6238=CARTESIAN_POINT ( 'NONE',  ( 3.608439182435180470, -6.249999999999997335, -116.5580127018922525 ) ) ;
#6239=ORIENTED_EDGE ( 'NONE', *, *, #14386, .F. ) ;
#6240=CARTESIAN_POINT ( 'NONE',  ( 5.999999999999949374, 1.607695154586804565, -141.0193375672974128 ) ) ;
#6242=CARTESIAN_POINT ( 'NONE',  ( 6.000000000000000888, 1.743066579297358182E-13, -52.58632486540518869 ) ) ;
#6243=CARTESIAN_POINT ( 'NONE',  ( 5.412658773652739619, 3.124999999999988898, -54.68301270189223828 ) ) ;
#6244=ORIENTED_EDGE ( 'NONE', *, *, #5524, .T. ) ;
#6245=CARTESIAN_POINT ( 'NONE',  ( 5.999999999999999112, 2.951592740943527306E-14, -153.6636751345948539 ) ) ;
#6247=CARTESIAN_POINT ( 'NONE',  ( 0.000000000000000000, 5.999999999999977796, -136.2113248654052029 ) ) ;
#6249=CARTESIAN_POINT ( 'NONE',  ( 3.175426480543072749, -5.500000000000105693, -164.1249999999999716 ) ) ;
#6252=EDGE_CURVE ( 'NONE', #13261, #18063, #17762, .T. ) ;
#6253=CARTESIAN_POINT ( 'NONE',  ( 4.763139720814407951, 2.750000000000002665, -106.7500000000000142 ) ) ;
#6255=CARTESIAN_POINT ( 'NONE',  ( -6.350852961085760029, -1.281975124255709124E-13, -109.1250000000000426 ) ) ;
#6256=CARTESIAN_POINT ( 'NONE',  ( 3.464101615137852974, 5.999999999999884537, -151.9136751345947971 ) ) ;
#6257=CARTESIAN_POINT ( 'NONE',  ( -3.464101615137757051, -5.999999999999979572, -82.16367513459481131 ) ) ;
#6262=EDGE_CURVE ( 'NONE', #17525, #27786, #20710, .T. ) ;
#6263=ADVANCED_FACE ( 'NONE', ( #15224 ), #10152, .T. ) ;
#6266=CARTESIAN_POINT ( 'NONE',  ( 2.775557561562891351E-14, 6.250000000000033751, -88.06698729810780435 ) ) ;
#6269=CARTESIAN_POINT ( 'NONE',  ( -0.4053696738521141985, 10.99999999999998579, -31.00000000000003553 ) ) ;
#6270=CARTESIAN_POINT ( 'NONE',  ( -6.350852961085760029, -1.281975124255709124E-13, -151.1250000000000568 ) ) ;
#6273=CARTESIAN_POINT ( 'NONE',  ( 3.175426480543072749, -5.500000000000105693, -123.6250000000000426 ) ) ;
#6274=CARTESIAN_POINT ( 'NONE',  ( 7.216878364870455975, -6.409875621278545621E-14, -140.3080127018922099 ) ) ;
#6275=ORIENTED_EDGE ( 'NONE', *, *, #25722, .T. ) ;
#6277=CARTESIAN_POINT ( 'NONE',  ( -5.412658773652684552, -3.125000000000099920, -122.0669872981078328 ) ) ;
#6278=CARTESIAN_POINT ( 'NONE',  ( -5.412658773652739619, 3.124999999999975131, -174.8169872981077901 ) ) ;
#6279=CARTESIAN_POINT ( 'NONE',  ( 6.350852961086080661, -9.614813431917819062E-14, -174.3750000000000284 ) ) ;
#6281=ORIENTED_EDGE ( 'NONE', *, *, #10770, .T. ) ;
#6287=CARTESIAN_POINT ( 'NONE',  ( -7.216878364870328078, 0.000000000000000000, -69.69198729810781856 ) ) ;
#6288=CARTESIAN_POINT ( 'NONE',  ( 2.775557561562891351E-14, 6.250000000000033751, -53.56698729810782567 ) ) ;
#6290=CARTESIAN_POINT ( 'NONE',  ( 3.175426480543072749, 5.499999999999865885, -51.12500000000002132 ) ) ;
#6291=CARTESIAN_POINT ( 'NONE',  ( 6.000000000000000888, -1.859271017917181981E-14, -171.0863248654052313 ) ) ;
#6292=( BOUNDED_SURFACE ( )  B_SPLINE_SURFACE ( 1, 2, ( 
 ( #15222, #6892, #20887, #16315, #2144, #8590, #6739, #25009, #25158, #25308, #22882, #25637, #11544, #25467, #6585, #20577, #13242, #9201, #13389, #27608, #27763, #1675, #20276, #4121, #16007, #22585, #1982, #11228, #27452, #13543, #29624, #30238, #4431, #15859, #6424, #16158, #18593, #29775, #20416, #8752, #1825, #8904, #1515, #13857, #23197, #18294, #10927, #17994, #27310, #27915, #6278, #15698, #3962, #29927, #4279, #22732, #18139, #13702, #23041, #11390, #20733, #30084, #9053, #18444, #11700, #19053, #21339, #2296, #11543, #28370, #18750, #25307, #6891, #7048, #25787, #18905, #4278, #23501, #13701, #134, #280, #23355, #9052, #4430, #13856, #30391, #23649, #14308, #18592, #27914, #16610, #16006, #18443, #4585, #30237, #2582, #11854, #11389, #14010, #20886, #9358, #25636, #25931, #9200, #9518, #2445, #30083, #21044, #21192, #28072, #28224, #7198, #4878, #4735, #16460, #23196, #1981, #27762, #25466, #16157, #12005, #2143, #23040, #9663, #20732, #16314, #14164, #6738, #19628, #19189, #5022, #24218, #23938, #574, #421, #21494, #7931, #5467, #14452, #26372, #17041, #12740, #28967, #12590, #17342, #5173, #23787, #14731, #16756, #14876, #10114, #14587, #7350, #26657, #12295, #5618, #28659, #10416, #17193, #26517, #15026, #7488, #19484, #28517, #9962, #3166, #24369, #21931, #19768, #2876, #3314, #12150, #21639, #10265, #26080, #26218, #21786, #9810, #28815, #7777, #2723, #1016, #19340, #22082, #864, #16898, #3023, #7631, #5321, #24074, #12441, #729, #29114, #8072, #5769, #26803, #15178, #17491, #16713, #19145, #14838, #23893, #25886, #7590, #830, #14266, #17149, #21446, #17001, #16859, #14690, #26037, #23604, #11966, #12108, #24035, #28482, #9770, #2979, #7447, #12400, #26180, #7741, #10226, #3127, #5127, #21748, #4984, #21893, #378, #7151, #16565, #14550, #21293, #233, #21596, #528, #23080, #3421, #18333, #25344, #17449, #1127, #22036, #17302, #17757, #29385, #15304, #2022, #11266, #1862, #24629, #19588, #5575, #7889, #20617, #4320, #14981, #28926, #26921, #3578, #6625, #26620, #5882, #4157, #22193, #972, #24321, #3274, #29224, #13006, #12701, #13737, #22345, #15140, #10373, #1280, #19729, #10525, #10691, #8350, #22919, #29076, #27081, #8040, #13579, #26764, #20038, #5730, #24470, #12849, #6469, #27648, #16045, #19879, #8189, #29964, #17604, #15895, #25192, #8942, #9701, #7236, #6776, #6, #6924, #4771, #21076, #12038, #25667, #25967, #18942, #25505, #16495, #16644, #28106, #4913, #2618, #14342, #170, #25822, #18628, #27799, #4470, #20924, #28259, #9391, #16195, #9086, #14198, #11732, #313, #5058, #21226, #7385, #14488, #19084, #23825, #28406, #13895, #23680, #23236, #23385, #23533, #18785, #11430, #16792, #21377, #2474, #7080, #20774, #26113, #11579, #11891, #30122, #30273, #18481, #2333, #9549, #2176, #9235, #27948, #4617, #16348, #14046, #10452, #15063, #5359, #17080, #5657, #22120, #19374, #614, #21677, #14766, #21822, #28698, #26557, #12484, #3349, #26408, #17376, #10300, #16932, #7815, #29003, #19523, #7968, #24407, #12777, #21967, #17231, #10000, #19224, #26260, #12330, #19662, #768, #7521, #457, #5504, #3059, #1063, #26844, #12623, #29151, #5806, #19806, #15221, #8111, #28553, #26693, #14624, #24111, #14912, #10151, #2762, #17530, #12190, #24251, #28857, #21531, #9847, #2910, #3200, #5211, #7670, #23973, #900, #17993, #24553, #13388, #22584, #8436, #6132, #1199, #1824, #6423, #27161, #17842, #27451, #13542, #10774, #22425, #13093, #15545, #20275, #6584, #15858, #25157, #29623, #3506, #10605, #12935, #4120, #8903, #19959, #22271, #1514, #8589, #11227, #27607, #10926, #8751, #24864, #27006, #29311, #8267, #3812, #27309, #17682, #29926, #6277, #20122, #5970, #15697, #15390, #13241, #25008, #3961, #22881, #24714, #1674, #3657, #18138, #18293, #22731, #1364, #29465, #11069, #20415, #20576, #29774, #22613, #1547, #20608, #2012, #13120, #8617, #13270, #18324, #15886, #15419, #27342, #29341, #18171, #22761, #27190, #19989, #1852, #24891, #11256, #10955, #23071, #29803, #8782, #27638, #20153, #1703, #10803, #20305, #27482, #6616, #6460, #8301, #15578, #16038, #24745, #17873, #22911, #17712, #8466, #3994, #22458, #11100, #20446, #27035, #13729, #29650, #29954, #13571, #6001, #15729, #8934, #3685, #6161, #1392, #25185, #29501, #18025, #6305, #25038, #13414, #4151, #25335, #4310, #9382, #18618, #20766, #6914, #7071, #30112, #11495, #23226, #16337, #30263, #25658, #25496, #9077, #18469, #13887, #14039, #11571, #2171, #4609, #20916, #23377, #9228, #11723, #16486, #18776, #27941, #2323, #6767, #28095, #27791, #21066, #11421, #16187, #4460, #483, #14509, #336, #9877, #21105, #5083, #12216, #4644, #18810, #9266, #4498, #4938, #16670, #6952, #23850, #23412, #13921, #9728, #12061, #11760, #28136, #7262, #19106, #18659, #23264, #23707, #2358, #34, #30303, #20952, #7410, #14369, #2206, #25846, #16524, #21556, #28431, #21403, #16816, #14077, #11610, #23557, #9422, #19253, #9574, #16224, #7104, #28284, #2642, #26138, #25537, #2788, #27978, #6800, #16370, #14221, #25693, #4793, #2495, #21249, #11920, #190, #18968, #10178, #29182, #10639, #21704, #17258, #12508, #26877, #24432, #23994, #26581, #24139, #21993, #7843, #8142, #21846, #12806, #5684, #12354, #3227, #3380, #14941, #22147, #19835, #10485, #17407, #12652, #5387, #14648, #643, #7697, #15094, #5535, #2937, #26286, #928, #28881, #17560, #22300, #8001, #24583, #1231, #5839, #28580, #15254, #10025, #3532, #19403, #19549, #10328, #24280, #7549, #12963, #16958, #29036, #26721, #5236, #28726, #17106, #26431, #14795, #3083, #794, #6409, #20562, #10913, #6571, #13531, #18125, #15846, #17979, #27750, #11379, #27439, #25144, #1970, #9040, #20402, #11056, #1662, #4108, #1809, #20267, #30070, #20722, #11214, #29614, #15685, #27293, #18428, #8574, #22718, #6266, #18281, #15995, #24994, #3949, #23024, #29759, #25293, #22871, #29913, #8891, #6728, #16146, #8738, #27594, #4264, #13684, #25452, #4416, #5648, #17219, #13083, #24702, #24400, #1050, #19950, #1350, #893, #26547, #5955, #15052, #12768, #12618, #3192, #20107, #17669, #5495, #8102, #29143, #24853, #10763, #3645, #29452, #17369, #14902, #26832, #28845, #26993, #22261, #26684, #19514, #8425, #3342, #17831, #10442, #22571, #29301, #8256, #27149, #19653, #1190, #10288, #22110, #15376, #6117, #22415, #1502, #19797, #15534, #24243, #17518, #3801, #7802, #7960, #3495, #21959, #10597, #13229, #28993, #5796, #15210, #24544, #12922, #6898, #25315, #13867, #13399, #22894, #22743, #30095, #11083, #1685, #13710, #29935, #23051, #20427, #11239, #4291, #27925, #11398, #18149, #18453, #29787, #6439, #8763, #1990, #25476, #20745, #23207, #8915, #25167, #4131, #16016, #2153, #9060, #27773, #4442, #6750, #20899, #16171, #9211, #27461, #15869, #11555, #18603, #1836, #20587, #18305, #27619, #6594, #17540, #20286, #15710, #29634, #15558, #25020, #5817, #8600, #27324, #19816, #3518, #24416, #19675, #18006, #24875, #3975, #15234, #6287, #21979, #29162, #12946, #3360, #29015, #20133, #1376, #22132, #912, #8125, #7980, #3824, #27172, #26857, #22283, #22439, #13254, #12788, #17387, #8448, #24567, #1211, #15075, #5667, #22595, #29480, #26703, #10619, #19970, #10309, #1527, #6144, #10936, #29323, #1073, #8281, #10463, #17855, #24727, #17694, #27020, #5985, #15403, #3668, #13103, #10786, #9061, #18454, #9212, #25168, #20746, #4132, #8916, #27774, #18604, #6751, #16323, #11240, #30245, #18150, #22895, #13868, #11084, #13552, #1991, #6441, #30096, #16172, #20429, #6899, #20588, #11556, #4443, #25642, #13711, #2154, #1686, #29936, #29788, #23208, #27462, #8764, #20900, #25316, #27926, #15870, #23052, #1837, #18306, #27620, #4292, #6595, #16017, #11400, #29635, #12947, #1377, #29324, #20134, #8126, #17388, #26704, #15235, #17856, #1212, #22284, #29481, #8282, #3825, #17695, #13255, #22744, #8601, #27021, #8450, #1075, #27325, #22133, #1528, #10937, #5818, #18008, #3976, #24568, #5986, #10310, #26858, #10621, #6288, #15404, #7981, #22440, #19676, #5669, #15711, #24728, #27173, #3669, #15560, #13105, #15076, #24417, #20287, #25021, #29017, #3361, #12789, #10464, #19817, #15463, #4317, #22190, #20773, #13167, #27646, #3575, #1124, #13003, #13736, #11428, #20035, #10522, #19876, #8186, #17601, #26918, #22503, #15301, #22342, #1438, #1277, #20199, #27078, #29382, #8347, #29549, #8505, #9921, #21443, #17300, #28924, #28617, #5280, #24180, #5573, #5125, #376, #10224, #19295 ),
 ( #5727, #9768, #12105, #24319, #8037, #19143, #23748, #686, #28769, #10371, #26761, #10071, #7887, #26324, #14548, #28480, #7445, #2977, #7739, #2680, #29073, #17147, #7588, #16856, #26470, #23890, #14687, #14836, #3125, #3271, #2833, #828, #12255, #22034, #24032, #12398, #12699, #21593, #525, #21746, #16998, #970, #19586, #5426, #12547, #21890, #17446, #1366, #15699, #5972, #8591, #10928, #24554, #8438, #20277, #29466, #29625, #6279, #17995, #22586, #27163, #8269, #26846, #3508, #10606, #27312, #10776, #15223, #8113, #17843, #22428, #3963, #29777, #13243, #1676, #8753, #22733, #18140, #13390, #5807, #25010, #12936, #3659, #15546, #20124, #19807, #11070, #20417, #24865, #6134, #17532, #22272, #13094, #1200, #19960, #3815, #27008, #1516, #29312, #17684, #15392, #24716, #12261, #19302, #11973, #24042, #7594, #2987, #12408, #21753, #693, #16720, #10079, #28337, #16571, #240, #19014, #16425, #25748, #20849, #7158, #11191, #13505, #4694, #9479, #20539, #25120, #2104, #30203, #21155, #28184, #18558, #9320, #27726, #27568, #18254, #6548, #13817, #25599, #4084, #18863, #4551, #20696, #22846, #14129, #1784, #23468, #2406, #15968, #25266, #1944, #11350, #30046, #6705, #3944, #24700, #8100, #24542, #3492, #10759, #24398, #19947, #20266, #3340, #29297, #8253, #1188, #3642, #29449, #1046, #10441, #19795, #17828, #29141, #12920, #5793, #17516, #26830, #17668, #15208, #22568, #29611, #22258, #26991, #13080, #22413, #27148, #8572, #1500, #6116, #15531, #7170, #6603, #16025, #25906, #9491, #25324, #23624, #4299, #16585, #11982, #21312, #19029, #23058, #254, #1999, #28347, #13717, #2558, #18873, #4856, #14282, #9637, #11408, #20754, #109, #28196, #12101, #30190, #11653, #18852, #14118, #21441, #27874, #16416, #2539, #11963, #23307, #15310, #26768, #17608, #20042, #29388, #8355, #17763, #16754, #12439, #19482, #11060, #1666, #8580, #17984, #24999, #6270, #15689, #27300, #18901, #130, #23934, #2871, #19763, #9958, #28656, #7627, #17883, #15967, #5879, #15774, #1592, #3573, #15137, #10995, #22652, #22341, #29380, #17912, #29692, #29221, #24467, #3879, #13002, #10688, #10521, #1123, #18064, #15619, #3418, #6045, #27077, #22802, #8664, #20338, #27378, #15300, #12846, #24787, #26759, #24930, #1276, #20034, #19875, #8185, #6340, #13312, #22188, #15460, #3731, #1740, #25081, #4038, #13458, #24625, #17600, #13165, #5726, #11139, #20197, #8346, #17445, #20487, #17754, #29846, #22500, #26916, #27229, #6200, #1435, #10845, #29548, #8503, #11464, #6958, #25852, #27985, #11926, #4342, #7108, #13610, #6663, #11766, #27526, #27681, #23269, #1894, #20958, #9270, #6504, #2499, #13767, #9429, #2365, #21255, #4505, #40, #8826, #16078, #18208, #30309, #15928, #25225, #6806, #23113, #25543, #4194, #25383, #30156, #16529, #13926, #22957, #18664, #11300, #20651, #28142, #2063, #16376, #27836, #25698, #20808, #29997, #8973, #9119, #4650, #18513, #16230, #14082, #2211, #23419, #11616, #21110, #18364, #4799, #18813, #14227, #23563, #17678, #12066, #14801, #3087, #26142, #28886, #24709, #8264, #24145, #3653, #14514, #27002, #5965, #28438, #12220, #2647, #28291, #26292, #19110, #15385, #12515, #16822, #7269, #21853, #5394, #5087, #21559, #648, #798, #21408, #16675, #17112, #21710, #18973, #13089, #28585, #23854, #16964, #194, #7415, #488, #9579, #5244, #25997, #12360, #4944, #14375, #19554, #2795, #10032, #19258, #19408, #9884, #23710, #340, #7552, #7705, #14655, #23999, #28733, #2943, #10183, #26439, #9734, #25459, #11384, #1669, #11222, #13237, #9046, #3807, #6579, #25302, #17988, #20727, #16152, #30078, #16002, #4424, #6273, #18438, #27755, #20273, #3957, #24860, #20118, #18132, #10923, #6733, #4273, #8585, #29460, #13695, #27600, #27304, #13384, #22876, #23033, #22580, #8433, #8898, #15693, #25004, #15541, #6127, #1976, #20572, #17839, #11065, #20410, #22421, #1360, #10769, #27157, #29619, #1510, #29770, #22727, #29920, #25152, #8747, #27447, #6419, #15853, #4115, #13538, #1818, #18289, #2577, #21489, #14005, #25925, #4579, #16455, #12000, #415, #21332, #16893, #9353, #12144, #18587, #11695, #16749, #2137, #2290, #28220, #6885, #4873, #14304, #11538, #7481, #18745, #14447, #7343, #26212, #9512, #5016, #13852, #21039, #23192, #23495, #20879, #9804, #26075, #7193, #21187, #30232, #19182, #23350, #16604, #28364, #30385, #9195, #4730, #23644, #27907, #275, #11849, #28066, #25782, #16310, #28512, #23782, #14158, #7042, #2717, #25631, #2438, #128, #18899, #9657, #19048, #17637, #26798, #17485, #860, #5168, #21635, #23932, #5764, #19918, #568, #14579, #12586, #10260, #22226, #8224, #21928, #19762, #7770, #7625, #9956, #19335, #14869, #19620, #2869, #10559, #28963, #724, #12289, #7926, #28654, #26511, #26652, #15022, #8068, #17034, #12736, #26367, #29109, #29263, #17336, #5316, #24068, #3018, #5612, #12891, #3457, #17187, #5462, #15174, #14725, #12434, #24212, #19478, #1157, #1010, #21781, #3161, #10109, #24363, #3310, #24508, #28810, #22076, #10412, #10729, #1627, #22839, #13347, #1780, #18247, #29882, #15813, #11028, #3772, #13046, #20076, #6083, #13498, #15656, #1317, #24667, #20374, #27264, #15962, #20690, #6380, #22996, #17951, #25260, #4233, #22537, #22379, #20533, #8389, #8545, #8705, #26959, #8863, #1471, #27561, #6235, #30041, #25115, #4076, #13656, #27115, #18097, #17796, #29585, #11183, #1939, #6541, #9011, #10883, #11344, #29419, #24825, #5921, #15349, #15500, #29728, #13204, #27413, #3612, #20238, #24963, #3916, #22690, #11969, #380, #14123, #9618, #18403, #16272, #27720, #9472, #6699, #16118, #16421, #13970, #4689, #21448, #6847, #9315, #26039, #23462, #25422, #89, #4384, #13811, #7309, #11660, #18858, #7001, #28179, #25593, #23158, #2099, #23311, #25888, #18706, #30350, #7153, #28028, #2544, #25742, #21295, #11506, #16715, #2400, #16567, #9160, #4986, #30198, #235, #19009, #2255, #14416, #12111, #23752, #28332, #20845, #21004, #2684, #18553, #4545, #11812, #27879, #21149, #4842, #14268, #23606, #24323, #26329, #7449, #3276, #14982, #14692, #21750, #10229, #22039, #21598, #16861, #26621, #5284, #2981, #2836, #23895, #10374, #7891, #26182, #28773, #19447, #15141, #974, #12703, #19730, #7592, #5130, #17151, #19147, #17304, #12551, #17005, #24183, #12258, #21895, #19590, #14552, #3423, #24037, #29077, #8041, #22194, #5429, #17450, #9772, #12402, #28484, #832, #530, #9924, #7743, #689, #26473, #12850, #28620, #10074, #26765, #14840, #19298, #28928, #3129, #5577, #5731, #24471, #22655, #20202, #10999, #20039, #8190, #17605, #6049, #8670, #22506, #13170, #1596, #10849, #15778, #29552, #4041, #4197, #20492, #8509, #20344, #22346, #18213, #13007, #25084, #13462, #27083, #29850, #25228, #8829, #22805, #13615, #15466, #27529, #6507, #29386, #1441, #3579, #29225, #27233, #8351, #15932, #1745, #17758, #26922, #11144, #6344, #24791, #17917, #29696, #1128, #1281, #5883, #18068, #3736, #6204, #24630, #15306, #10526, #27382, #10692, #15623, #24933, #19880, #3882, #13315, #2503, #20812, #8976, #30314, #1899, #21112, #25701, #30160, #22961, #4804, #27840, #14232, #13931, #26001, #2369, #11770, #199, #23118, #4654, #13774, #25548, #47, #9585, #9432, #4947, #18518, #21259, #27684, #9123, #25856, #11305, #11468, #18818, #6666, #27989, #28144, #9274, #7112, #23568, #11930, #16532, #6961, #6810, #18368, #16082, #2067, #18975, #11619, #25388, #20655, #16380, #23274, #28294, #16678, #7274, #30002, #2215, #4346, #16237, #4510, #20963, #18670, #14086, #23422, #26443, #24002, #26731, #12664, #26589, #7710, #21713, #14379, #10339, #14520, #28737, #28891, #2798, #21411, #5249, #17117, #23714, #3093, #12363, #28588, #26294, #344, #22001, #5545, #16972, #7555, #17268, #3237, #492, #12225, #21562, #14658, #10036, #2649, #14949, #24291, #19412, #12073, #9736, #19112, #938, #29044, #28442, #7419, #655, #5398, #19701, #17417, #14806, #7857, #2948, #16825, #26145, #5093, #24149, #12520, #23859, #8010, #21857, #9888, #19262, #803, #10189, #19557, #27198, #15586, #8629, #24439, #13279, #3389, #20314, #20456, #13127, #29190, #24593, #3542, #20164, #13424, #4008, #8312, #17721, #6314, #18179, #8151, #24757, #19999, #22769, #1560, #1098, #3697, #1241, #29513, #15430, #15737, #29350, #29661, #12816, #29816, #10648, #25048, #18035, #5696, #1403, #27351, #15107, #12974, #22159, #6174, #10494, #19843, #22465, #27047, #10814, #8793, #22309, #6011, #1713, #8475, #17569, #17884, #26886 ) ),
 .UNSPECIFIED., .F., .F., .F. ) 
 B_SPLINE_SURFACE_WITH_KNOTS ( ( 2, 2 ),
 ( 3, 2, 2, 2, 2, 2, 2, 2, 2, 2, 2, 2, 2, 2, 2, 2, 2, 2, 2, 2, 2, 2, 2, 2, 2, 2, 2, 2, 2, 2, 2, 2, 2, 2, 2, 2, 2, 2, 2, 2, 2, 2, 2, 2, 2, 2, 2, 2, 2, 2, 2, 2, 2, 2, 2, 2, 2, 2, 2, 2, 2, 2, 2, 2, 2, 2, 2, 2, 2, 2, 2, 2, 2, 2, 2, 2, 2, 2, 2, 2, 2, 2, 2, 2, 2, 2, 2, 2, 2, 2, 2, 2, 2, 2, 2, 2, 2, 2, 2, 2, 2, 2, 2, 2, 2, 2, 2, 2, 2, 2, 2, 2, 2, 2, 2, 2, 2, 2, 2, 2, 2, 2, 2, 2, 2, 2, 2, 2, 2, 2, 2, 2, 2, 2, 2, 2, 2, 2, 2, 2, 2, 2, 2, 2, 2, 2, 2, 2, 2, 2, 2, 2, 2, 2, 2, 2, 2, 2, 2, 2, 2, 2, 2, 2, 2, 2, 2, 2, 2, 2, 2, 2, 2, 2, 2, 2, 2, 2, 2, 2, 2, 2, 2, 2, 2, 2, 2, 2, 2, 2, 2, 2, 2, 2, 2, 2, 2, 2, 2, 2, 2, 2, 2, 2, 2, 2, 2, 2, 2, 2, 2, 2, 2, 2, 2, 2, 2, 2, 2, 2, 2, 2, 2, 2, 2, 2, 2, 2, 2, 2, 2, 2, 2, 2, 2, 2, 2, 2, 2, 2, 2, 2, 2, 2, 2, 2, 2, 2, 2, 2, 2, 2, 2, 2, 2, 2, 2, 2, 2, 2, 2, 2, 2, 2, 2, 2, 2, 2, 2, 2, 2, 2, 2, 2, 2, 2, 2, 2, 2, 2, 2, 2, 2, 2, 2, 2, 2, 2, 2, 2, 2, 2, 2, 2, 2, 2, 2, 2, 2, 2, 2, 2, 2, 2, 2, 2, 2, 2, 2, 2, 2, 2, 2, 2, 2, 2, 2, 2, 2, 2, 2, 2, 2, 2, 2, 2, 2, 2, 2, 2, 2, 2, 2, 2, 2, 2, 2, 2, 2, 2, 2, 2, 2, 2, 2, 2, 2, 2, 2, 2, 2, 2, 2, 2, 2, 2, 2, 2, 2, 2, 2, 2, 2, 2, 2, 2, 2, 2, 2, 2, 2, 2, 2, 2, 2, 2, 2, 2, 2, 2, 2, 2, 2, 2, 2, 2, 2, 2, 2, 2, 2, 2, 2, 2, 2, 2, 2, 2, 2, 2, 2, 2, 2, 2, 2, 2, 2, 2, 2, 2, 2, 2, 2, 2, 2, 2, 2, 2, 2, 2, 2, 2, 2, 2, 2, 2, 2, 2, 2, 2, 2, 2, 2, 2, 2, 2, 2, 2, 2, 2, 2, 2, 2, 2, 2, 2, 2, 2, 2, 2, 2, 2, 2, 2, 2, 2, 2, 2, 2, 2, 2, 2, 2, 2, 2, 2, 2, 2, 2, 2, 2, 2, 2, 2, 2, 2, 2, 2, 2, 2, 2, 2, 2, 2, 2, 2, 2, 2, 2, 2, 2, 2, 2, 2, 2, 2, 2, 2, 2, 2, 2, 2, 2, 2, 2, 2, 2, 2, 2, 2, 2, 2, 2, 2, 2, 2, 2, 2, 2, 2, 2, 2, 2, 2, 2, 2, 2, 2, 2, 2, 2, 2, 2, 2, 2, 2, 2, 2, 2, 2, 3 ),
 ( 0.000000000000000000, 1.000000000000000000 ),
 ( 0.000000000000000000, 0.001851851851851851923, 0.003703703703703703845, 0.005555555555555555768, 0.007407407407407407690, 0.009259259259259258745, 0.01111111111111111154, 0.01296296296296296259, 0.01481481481481481538, 0.01666666666666666644, 0.01851851851851851749, 0.02037037037037037202, 0.02222222222222222307, 0.02407407407407407413, 0.02592592592592592518, 0.02777777777777777624, 0.02962962962962963076, 0.03148148148148147835, 0.03333333333333333287, 0.03518518518518518740, 0.03703703703703703498, 0.03888888888888888951, 0.04074074074074074403, 0.04259259259259259162, 0.04444444444444444614, 0.04629629629629629373, 0.04814814814814814825, 0.05000000000000000278, 0.05185185185185185036, 0.05370370370370370489, 0.05555555555555555247, 0.05740740740740740700, 0.05925925925925926152, 0.06111111111111110911, 0.06296296296296295669, 0.06481481481481481122, 0.06666666666666666574, 0.06851851851851852027, 0.07037037037037037479, 0.07222222222222221544, 0.07407407407407406996, 0.07592592592592592449, 0.07777777777777777901, 0.07962962962962963354, 0.08148148148148148806, 0.08333333333333332871, 0.08518518518518518323, 0.08703703703703703776, 0.08888888888888889228, 0.09074074074074074681, 0.09259259259259258745, 0.09444444444444444198, 0.09629629629629629650, 0.09814814814814815103, 0.1000000000000000056, 0.1018518518518518462, 0.1037037037037037007, 0.1055555555555555552, 0.1074074074074074098, 0.1092592592592592643, 0.1111111111111111049, 0.1129629629629629595, 0.1148148148148148140, 0.1166666666666666685, 0.1185185185185185230, 0.1203703703703703637, 0.1222222222222222182, 0.1240740740740740727, 0.1259259259259259134, 0.1277777777777777679, 0.1296296296296296224, 0.1314814814814814770, 0.1333333333333333315, 0.1351851851851851860, 0.1370370370370370405, 0.1388888888888888951, 0.1407407407407407496, 0.1425925925925926041, 0.1444444444444444309, 0.1462962962962962854, 0.1481481481481481399, 0.1499999999999999944, 0.1518518518518518490, 0.1537037037037037035, 0.1555555555555555580, 0.1574074074074074125, 0.1592592592592592671, 0.1611111111111111216, 0.1629629629629629761, 0.1648148148148148029, 0.1666666666666666574, 0.1685185185185185119, 0.1703703703703703665, 0.1722222222222222210, 0.1740740740740740755, 0.1759259259259259300, 0.1777777777777777846, 0.1796296296296296391, 0.1814814814814814936, 0.1833333333333333204, 0.1851851851851851749, 0.1870370370370370294, 0.1888888888888888840, 0.1907407407407407385, 0.1925925925925925930, 0.1944444444444444475, 0.1962962962962963021, 0.1981481481481481566, 0.2000000000000000111, 0.2018518518518518656, 0.2037037037037036924, 0.2055555555555555469, 0.2074074074074074014, 0.2092592592592592560, 0.2111111111111111105, 0.2129629629629629650, 0.2148148148148148195, 0.2166666666666666741, 0.2185185185185185286, 0.2203703703703703831, 0.2222222222222222099, 0.2240740740740740644, 0.2259259259259259189, 0.2277777777777777735, 0.2296296296296296280, 0.2314814814814814825, 0.2333333333333333370, 0.2351851851851851916, 0.2370370370370370461, 0.2388888888888889006, 0.2407407407407407274, 0.2425925925925925819, 0.2444444444444444364, 0.2462962962962962910, 0.2481481481481481455, 0.2500000000000000000, 0.2518518518518518268, 0.2537037037037037090, 0.2555555555555555358, 0.2574074074074074181, 0.2592592592592592449, 0.2611111111111111271, 0.2629629629629629539, 0.2648148148148148362, 0.2666666666666666630, 0.2685185185185185452, 0.2703703703703703720, 0.2722222222222221988, 0.2740740740740740811, 0.2759259259259259078, 0.2777777777777777901, 0.2796296296296296169, 0.2814814814814814992, 0.2833333333333333259, 0.2851851851851852082, 0.2870370370370370350, 0.2888888888888888618, 0.2907407407407407440, 0.2925925925925925708, 0.2944444444444444531, 0.2962962962962962798, 0.2981481481481481621, 0.2999999999999999889, 0.3018518518518518712, 0.3037037037037036979, 0.3055555555555555802, 0.3074074074074074070, 0.3092592592592592338, 0.3111111111111111160, 0.3129629629629629428, 0.3148148148148148251, 0.3166666666666666519, 0.3185185185185185341, 0.3203703703703703609, 0.3222222222222222432, 0.3240740740740740700, 0.3259259259259259522, 0.3277777777777777790, 0.3296296296296296058, 0.3314814814814814881, 0.3333333333333333148, 0.3351851851851851971, 0.3370370370370370239, 0.3388888888888889062, 0.3407407407407407329, 0.3425925925925926152, 0.3444444444444444420, 0.3462962962962962687, 0.3481481481481481510, 0.3499999999999999778, 0.3518518518518518601, 0.3537037037037036868, 0.3555555555555555691, 0.3574074074074073959, 0.3592592592592592782, 0.3611111111111111049, 0.3629629629629629872, 0.3648148148148148140, 0.3666666666666666408, 0.3685185185185185230, 0.3703703703703703498, 0.3722222222222222321, 0.3740740740740740589, 0.3759259259259259411, 0.3777777777777777679, 0.3796296296296296502, 0.3814814814814814770, 0.3833333333333333592, 0.3851851851851851860, 0.3870370370370370128, 0.3888888888888888951, 0.3907407407407407218, 0.3925925925925926041, 0.3944444444444444309, 0.3962962962962963132, 0.3981481481481481399, 0.4000000000000000222, 0.4018518518518518490, 0.4037037037037037313, 0.4055555555555555580, 0.4074074074074073848, 0.4092592592592592671, 0.4111111111111110938, 0.4129629629629629761, 0.4148148148148148029, 0.4166666666666666852, 0.4185185185185185119, 0.4203703703703703942, 0.4222222222222222210, 0.4240740740740740478, 0.4259259259259259300, 0.4277777777777777568, 0.4296296296296296391, 0.4314814814814814659, 0.4333333333333333481, 0.4351851851851851749, 0.4370370370370370572, 0.4388888888888888840, 0.4407407407407407662, 0.4425925925925925930, 0.4444444444444444198, 0.4462962962962963021, 0.4481481481481481288, 0.4500000000000000111, 0.4518518518518518379, 0.4537037037037037202, 0.4555555555555555469, 0.4574074074074074292, 0.4592592592592592560, 0.4611111111111111382, 0.4629629629629629650, 0.4648148148148147918, 0.4666666666666666741, 0.4685185185185185008, 0.4703703703703703831, 0.4722222222222222099, 0.4740740740740740922, 0.4759259259259259189, 0.4777777777777778012, 0.4796296296296296280, 0.4814814814814814548, 0.4833333333333333370, 0.4851851851851851638, 0.4870370370370370461, 0.4888888888888888729, 0.4907407407407407551, 0.4925925925925925819, 0.4944444444444444642, 0.4962962962962962910, 0.4981481481481481732, 0.5000000000000000000, 0.5018518518518518823, 0.5037037037037036535, 0.5055555555555555358, 0.5074074074074074181, 0.5092592592592593004, 0.5111111111111110716, 0.5129629629629629539, 0.5148148148148148362, 0.5166666666666667185, 0.5185185185185184897, 0.5203703703703703720, 0.5222222222222222543, 0.5240740740740740256, 0.5259259259259259078, 0.5277777777777777901, 0.5296296296296296724, 0.5314814814814814437, 0.5333333333333333259, 0.5351851851851852082, 0.5370370370370370905, 0.5388888888888888618, 0.5407407407407407440, 0.5425925925925926263, 0.5444444444444443976, 0.5462962962962962798, 0.5481481481481481621, 0.5500000000000000444, 0.5518518518518518157, 0.5537037037037036979, 0.5555555555555555802, 0.5574074074074074625, 0.5592592592592592338, 0.5611111111111111160, 0.5629629629629629983, 0.5648148148148147696, 0.5666666666666666519, 0.5685185185185185341, 0.5703703703703704164, 0.5722222222222221877, 0.5740740740740740700, 0.5759259259259259522, 0.5777777777777777235, 0.5796296296296296058, 0.5814814814814814881, 0.5833333333333333703, 0.5851851851851851416, 0.5870370370370370239, 0.5888888888888889062, 0.5907407407407407884, 0.5925925925925925597, 0.5944444444444444420, 0.5962962962962963243, 0.5981481481481480955, 0.5999999999999999778, 0.6018518518518518601, 0.6037037037037037424, 0.6055555555555555136, 0.6074074074074073959, 0.6092592592592592782, 0.6111111111111111605, 0.6129629629629629317, 0.6148148148148148140, 0.6166666666666666963, 0.6185185185185184675, 0.6203703703703703498, 0.6222222222222222321, 0.6240740740740741144, 0.6259259259259258856, 0.6277777777777777679, 0.6296296296296296502, 0.6314814814814815325, 0.6333333333333333037, 0.6351851851851851860, 0.6370370370370370683, 0.6388888888888888395, 0.6407407407407407218, 0.6425925925925926041, 0.6444444444444444864, 0.6462962962962962576, 0.6481481481481481399, 0.6500000000000000222, 0.6518518518518519045, 0.6537037037037036757, 0.6555555555555555580, 0.6574074074074074403, 0.6592592592592592116, 0.6611111111111110938, 0.6629629629629629761, 0.6648148148148148584, 0.6666666666666666297, 0.6685185185185185119, 0.6703703703703703942, 0.6722222222222222765, 0.6740740740740740478, 0.6759259259259259300, 0.6777777777777778123, 0.6796296296296295836, 0.6814814814814814659, 0.6833333333333333481, 0.6851851851851852304, 0.6870370370370370017, 0.6888888888888888840, 0.6907407407407407662, 0.6925925925925925375, 0.6944444444444444198, 0.6962962962962963021, 0.6981481481481481843, 0.6999999999999999556, 0.7018518518518518379, 0.7037037037037037202, 0.7055555555555556024, 0.7074074074074073737, 0.7092592592592592560, 0.7111111111111111382, 0.7129629629629629095, 0.7148148148148147918, 0.7166666666666666741, 0.7185185185185185563, 0.7203703703703703276, 0.7222222222222222099, 0.7240740740740740922, 0.7259259259259259744, 0.7277777777777777457, 0.7296296296296296280, 0.7314814814814815103, 0.7333333333333332815, 0.7351851851851851638, 0.7370370370370370461, 0.7388888888888889284, 0.7407407407407406996, 0.7425925925925925819, 0.7444444444444444642, 0.7462962962962963465, 0.7481481481481481177, 0.7500000000000000000, 0.7518518518518518823, 0.7537037037037036535, 0.7555555555555555358, 0.7574074074074074181, 0.7592592592592593004, 0.7611111111111110716, 0.7629629629629629539, 0.7648148148148148362, 0.7666666666666667185, 0.7685185185185184897, 0.7703703703703703720, 0.7722222222222222543, 0.7740740740740740256, 0.7759259259259259078, 0.7777777777777777901, 0.7796296296296296724, 0.7814814814814814437, 0.7833333333333333259, 0.7851851851851852082, 0.7870370370370370905, 0.7888888888888888618, 0.7907407407407407440, 0.7925925925925926263, 0.7944444444444443976, 0.7962962962962962798, 0.7981481481481481621, 0.8000000000000000444, 0.8018518518518518157, 0.8037037037037036979, 0.8055555555555555802, 0.8074074074074074625, 0.8092592592592592338, 0.8111111111111111160, 0.8129629629629629983, 0.8148148148148147696, 0.8166666666666666519, 0.8185185185185185341, 0.8203703703703704164, 0.8222222222222221877, 0.8240740740740740700, 0.8259259259259259522, 0.8277777777777777235, 0.8296296296296296058, 0.8314814814814814881, 0.8333333333333333703, 0.8351851851851851416, 0.8370370370370370239, 0.8388888888888889062, 0.8407407407407407884, 0.8425925925925925597, 0.8444444444444444420, 0.8462962962962963243, 0.8481481481481480955, 0.8499999999999999778, 0.8518518518518518601, 0.8537037037037037424, 0.8555555555555555136, 0.8574074074074073959, 0.8592592592592592782, 0.8611111111111111605, 0.8629629629629629317, 0.8648148148148148140, 0.8666666666666666963, 0.8685185185185184675, 0.8703703703703703498, 0.8722222222222222321, 0.8740740740740741144, 0.8759259259259258856, 0.8777777777777777679, 0.8796296296296296502, 0.8814814814814815325, 0.8833333333333333037, 0.8851851851851851860, 0.8870370370370370683, 0.8888888888888888395, 0.8907407407407407218, 0.8925925925925926041, 0.8944444444444444864, 0.8962962962962962576, 0.8981481481481481399, 0.9000000000000000222, 0.9018518518518519045, 0.9037037037037036757, 0.9055555555555555580, 0.9074074074074074403, 0.9092592592592592116, 0.9111111111111110938, 0.9129629629629629761, 0.9148148148148148584, 0.9166666666666666297, 0.9185185185185185119, 0.9203703703703703942, 0.9222222222222222765, 0.9240740740740740478, 0.9259259259259259300, 0.9277777777777778123, 0.9296296296296295836, 0.9314814814814814659, 0.9333333333333333481, 0.9351851851851852304, 0.9370370370370370017, 0.9388888888888888840, 0.9407407407407407662, 0.9425925925925925375, 0.9444444444444444198, 0.9462962962962963021, 0.9481481481481481843, 0.9499999999999999556, 0.9518518518518518379, 0.9537037037037037202, 0.9555555555555556024, 0.9574074074074073737, 0.9592592592592592560, 0.9611111111111111382, 0.9629629629629629095, 0.9648148148148147918, 0.9666666666666666741, 0.9685185185185185563, 0.9703703703703703276, 0.9722222222222222099, 0.9740740740740740922, 0.9759259259259259744, 0.9777777777777777457, 0.9796296296296296280, 0.9814814814814815103, 0.9833333333333332815, 0.9851851851851851638, 0.9870370370370370461, 0.9888888888888889284, 0.9907407407407406996, 0.9925925925925925819, 0.9944444444444444642, 0.9962962962962963465, 0.9981481481481481177, 1.000000000000000000 ),
 .UNSPECIFIED. ) 
 GEOMETRIC_REPRESENTATION_ITEM ( )  RATIONAL_B_SPLINE_SURFACE ( (
 ( 1.000000000000000000, 0.8660254037844387076, 1.000000000000000000, 0.8660254037844387076, 1.000000000000000000, 0.8660254037844387076, 1.000000000000000000, 0.8660254037844387076, 1.000000000000000000, 0.8660254037844387076, 1.000000000000000000, 0.8660254037844387076, 1.000000000000000000, 0.8660254037844387076, 1.000000000000000000, 0.8660254037844387076, 1.000000000000000000, 0.8660254037844387076, 1.000000000000000000, 0.8660254037844387076, 1.000000000000000000, 0.8660254037844387076, 1.000000000000000000, 0.8660254037844387076, 1.000000000000000000, 0.8660254037844387076, 1.000000000000000000, 0.8660254037844387076, 1.000000000000000000, 0.8660254037844387076, 1.000000000000000000, 0.8660254037844387076, 1.000000000000000000, 0.8660254037844387076, 1.000000000000000000, 0.8660254037844387076, 1.000000000000000000, 0.8660254037844387076, 1.000000000000000000, 0.8660254037844387076, 1.000000000000000000, 0.8660254037844387076, 1.000000000000000000, 0.8660254037844387076, 1.000000000000000000, 0.8660254037844387076, 1.000000000000000000, 0.8660254037844387076, 1.000000000000000000, 0.8660254037844387076, 1.000000000000000000, 0.8660254037844387076, 1.000000000000000000, 0.8660254037844387076, 1.000000000000000000, 0.8660254037844387076, 1.000000000000000000, 0.8660254037844387076, 1.000000000000000000, 0.8660254037844387076, 1.000000000000000000, 0.8660254037844387076, 1.000000000000000000, 0.8660254037844387076, 1.000000000000000000, 0.8660254037844387076, 1.000000000000000000, 0.8660254037844387076, 1.000000000000000000, 0.8660254037844387076, 1.000000000000000000, 0.8660254037844387076, 1.000000000000000000, 0.8660254037844387076, 1.000000000000000000, 0.8660254037844387076, 1.000000000000000000, 0.8660254037844387076, 1.000000000000000000, 0.8660254037844387076, 1.000000000000000000, 0.8660254037844387076, 1.000000000000000000, 0.8660254037844387076, 1.000000000000000000, 0.8660254037844387076, 1.000000000000000000, 0.8660254037844387076, 1.000000000000000000, 0.8660254037844387076, 1.000000000000000000, 0.8660254037844387076, 1.000000000000000000, 0.8660254037844387076, 1.000000000000000000, 0.8660254037844387076, 1.000000000000000000, 0.8660254037844387076, 1.000000000000000000, 0.8660254037844387076, 1.000000000000000000, 0.8660254037844387076, 1.000000000000000000, 0.8660254037844387076, 1.000000000000000000, 0.8660254037844387076, 1.000000000000000000, 0.8660254037844387076, 1.000000000000000000, 0.8660254037844387076, 1.000000000000000000, 0.8660254037844387076, 1.000000000000000000, 0.8660254037844387076, 1.000000000000000000, 0.8660254037844387076, 1.000000000000000000, 0.8660254037844387076, 1.000000000000000000, 0.8660254037844387076, 1.000000000000000000, 0.8660254037844387076, 1.000000000000000000, 0.8660254037844387076, 1.000000000000000000, 0.8660254037844387076, 1.000000000000000000, 0.8660254037844387076, 1.000000000000000000, 0.8660254037844387076, 1.000000000000000000, 0.8660254037844387076, 1.000000000000000000, 0.8660254037844387076, 1.000000000000000000, 0.8660254037844387076, 1.000000000000000000, 0.8660254037844387076, 1.000000000000000000, 0.8660254037844387076, 1.000000000000000000, 0.8660254037844387076, 1.000000000000000000, 0.8660254037844387076, 1.000000000000000000, 0.8660254037844387076, 1.000000000000000000, 0.8660254037844387076, 1.000000000000000000, 0.8660254037844387076, 1.000000000000000000, 0.8660254037844387076, 1.000000000000000000, 0.8660254037844387076, 1.000000000000000000, 0.8660254037844387076, 1.000000000000000000, 0.8660254037844387076, 1.000000000000000000, 0.8660254037844387076, 1.000000000000000000, 0.8660254037844387076, 1.000000000000000000, 0.8660254037844387076, 1.000000000000000000, 0.8660254037844387076, 1.000000000000000000, 0.8660254037844387076, 1.000000000000000000, 0.8660254037844387076, 1.000000000000000000, 0.8660254037844387076, 1.000000000000000000, 0.8660254037844387076, 1.000000000000000000, 0.8660254037844387076, 1.000000000000000000, 0.8660254037844387076, 1.000000000000000000, 0.8660254037844387076, 1.000000000000000000, 0.8660254037844387076, 1.000000000000000000, 0.8660254037844387076, 1.000000000000000000, 0.8660254037844387076, 1.000000000000000000, 0.8660254037844387076, 1.000000000000000000, 0.8660254037844387076, 1.000000000000000000, 0.8660254037844387076, 1.000000000000000000, 0.8660254037844387076, 1.000000000000000000, 0.8660254037844387076, 1.000000000000000000, 0.8660254037844387076, 1.000000000000000000, 0.8660254037844387076, 1.000000000000000000, 0.8660254037844387076, 1.000000000000000000, 0.8660254037844387076, 1.000000000000000000, 0.8660254037844387076, 1.000000000000000000, 0.8660254037844387076, 1.000000000000000000, 0.8660254037844387076, 1.000000000000000000, 0.8660254037844387076, 1.000000000000000000, 0.8660254037844387076, 1.000000000000000000, 0.8660254037844387076, 1.000000000000000000, 0.8660254037844387076, 1.000000000000000000, 0.8660254037844387076, 1.000000000000000000, 0.8660254037844387076, 1.000000000000000000, 0.8660254037844387076, 1.000000000000000000, 0.8660254037844387076, 1.000000000000000000, 0.8660254037844387076, 1.000000000000000000, 0.8660254037844387076, 1.000000000000000000, 0.8660254037844387076, 1.000000000000000000, 0.8660254037844387076, 1.000000000000000000, 0.8660254037844387076, 1.000000000000000000, 0.8660254037844387076, 1.000000000000000000, 0.8660254037844387076, 1.000000000000000000, 0.8660254037844387076, 1.000000000000000000, 0.8660254037844387076, 1.000000000000000000, 0.8660254037844387076, 1.000000000000000000, 0.8660254037844387076, 1.000000000000000000, 0.8660254037844387076, 1.000000000000000000, 0.8660254037844387076, 1.000000000000000000, 0.8660254037844387076, 1.000000000000000000, 0.8660254037844387076, 1.000000000000000000, 0.8660254037844387076, 1.000000000000000000, 0.8660254037844387076, 1.000000000000000000, 0.8660254037844387076, 1.000000000000000000, 0.8660254037844387076, 1.000000000000000000, 0.8660254037844387076, 1.000000000000000000, 0.8660254037844387076, 1.000000000000000000, 0.8660254037844387076, 1.000000000000000000, 0.8660254037844387076, 1.000000000000000000, 0.8660254037844387076, 1.000000000000000000, 0.8660254037844387076, 1.000000000000000000, 0.8660254037844387076, 1.000000000000000000, 0.8660254037844387076, 1.000000000000000000, 0.8660254037844387076, 1.000000000000000000, 0.8660254037844387076, 1.000000000000000000, 0.8660254037844387076, 1.000000000000000000, 0.8660254037844387076, 1.000000000000000000, 0.8660254037844387076, 1.000000000000000000, 0.8660254037844387076, 1.000000000000000000, 0.8660254037844387076, 1.000000000000000000, 0.8660254037844387076, 1.000000000000000000, 0.8660254037844387076, 1.000000000000000000, 0.8660254037844387076, 1.000000000000000000, 0.8660254037844387076, 1.000000000000000000, 0.8660254037844387076, 1.000000000000000000, 0.8660254037844387076, 1.000000000000000000, 0.8660254037844387076, 1.000000000000000000, 0.8660254037844387076, 1.000000000000000000, 0.8660254037844387076, 1.000000000000000000, 0.8660254037844387076, 1.000000000000000000, 0.8660254037844387076, 1.000000000000000000, 0.8660254037844387076, 1.000000000000000000, 0.8660254037844387076, 1.000000000000000000, 0.8660254037844387076, 1.000000000000000000, 0.8660254037844387076, 1.000000000000000000, 0.8660254037844387076, 1.000000000000000000, 0.8660254037844387076, 1.000000000000000000, 0.8660254037844387076, 1.000000000000000000, 0.8660254037844387076, 1.000000000000000000, 0.8660254037844387076, 1.000000000000000000, 0.8660254037844387076, 1.000000000000000000, 0.8660254037844387076, 1.000000000000000000, 0.8660254037844387076, 1.000000000000000000, 0.8660254037844387076, 1.000000000000000000, 0.8660254037844387076, 1.000000000000000000, 0.8660254037844387076, 1.000000000000000000, 0.8660254037844387076, 1.000000000000000000, 0.8660254037844387076, 1.000000000000000000, 0.8660254037844387076, 1.000000000000000000, 0.8660254037844387076, 1.000000000000000000, 0.8660254037844387076, 1.000000000000000000, 0.8660254037844387076, 1.000000000000000000, 0.8660254037844387076, 1.000000000000000000, 0.8660254037844387076, 1.000000000000000000, 0.8660254037844387076, 1.000000000000000000, 0.8660254037844387076, 1.000000000000000000, 0.8660254037844387076, 1.000000000000000000, 0.8660254037844387076, 1.000000000000000000, 0.8660254037844387076, 1.000000000000000000, 0.8660254037844387076, 1.000000000000000000, 0.8660254037844387076, 1.000000000000000000, 0.8660254037844387076, 1.000000000000000000, 0.8660254037844387076, 1.000000000000000000, 0.8660254037844387076, 1.000000000000000000, 0.8660254037844387076, 1.000000000000000000, 0.8660254037844387076, 1.000000000000000000, 0.8660254037844387076, 1.000000000000000000, 0.8660254037844387076, 1.000000000000000000, 0.8660254037844387076, 1.000000000000000000, 0.8660254037844387076, 1.000000000000000000, 0.8660254037844387076, 1.000000000000000000, 0.8660254037844387076, 1.000000000000000000, 0.8660254037844387076, 1.000000000000000000, 0.8660254037844387076, 1.000000000000000000, 0.8660254037844387076, 1.000000000000000000, 0.8660254037844387076, 1.000000000000000000, 0.8660254037844387076, 1.000000000000000000, 0.8660254037844387076, 1.000000000000000000, 0.8660254037844387076, 1.000000000000000000, 0.8660254037844387076, 1.000000000000000000, 0.8660254037844387076, 1.000000000000000000, 0.8660254037844387076, 1.000000000000000000, 0.8660254037844387076, 1.000000000000000000, 0.8660254037844387076, 1.000000000000000000, 0.8660254037844387076, 1.000000000000000000, 0.8660254037844387076, 1.000000000000000000, 0.8660254037844387076, 1.000000000000000000, 0.8660254037844387076, 1.000000000000000000, 0.8660254037844387076, 1.000000000000000000, 0.8660254037844387076, 1.000000000000000000, 0.8660254037844387076, 1.000000000000000000, 0.8660254037844387076, 1.000000000000000000, 0.8660254037844387076, 1.000000000000000000, 0.8660254037844387076, 1.000000000000000000, 0.8660254037844387076, 1.000000000000000000, 0.8660254037844387076, 1.000000000000000000, 0.8660254037844387076, 1.000000000000000000, 0.8660254037844387076, 1.000000000000000000, 0.8660254037844387076, 1.000000000000000000, 0.8660254037844387076, 1.000000000000000000, 0.8660254037844387076, 1.000000000000000000, 0.8660254037844387076, 1.000000000000000000, 0.8660254037844387076, 1.000000000000000000, 0.8660254037844387076, 1.000000000000000000, 0.8660254037844387076, 1.000000000000000000, 0.8660254037844387076, 1.000000000000000000, 0.8660254037844387076, 1.000000000000000000, 0.8660254037844387076, 1.000000000000000000, 0.8660254037844387076, 1.000000000000000000, 0.8660254037844387076, 1.000000000000000000, 0.8660254037844387076, 1.000000000000000000, 0.8660254037844387076, 1.000000000000000000, 0.8660254037844387076, 1.000000000000000000, 0.8660254037844387076, 1.000000000000000000, 0.8660254037844387076, 1.000000000000000000, 0.8660254037844387076, 1.000000000000000000, 0.8660254037844387076, 1.000000000000000000, 0.8660254037844387076, 1.000000000000000000, 0.8660254037844387076, 1.000000000000000000, 0.8660254037844387076, 1.000000000000000000, 0.8660254037844387076, 1.000000000000000000, 0.8660254037844387076, 1.000000000000000000, 0.8660254037844387076, 1.000000000000000000, 0.8660254037844387076, 1.000000000000000000, 0.8660254037844387076, 1.000000000000000000, 0.8660254037844387076, 1.000000000000000000, 0.8660254037844387076, 1.000000000000000000, 0.8660254037844387076, 1.000000000000000000, 0.8660254037844387076, 1.000000000000000000, 0.8660254037844387076, 1.000000000000000000, 0.8660254037844387076, 1.000000000000000000, 0.8660254037844387076, 1.000000000000000000, 0.8660254037844387076, 1.000000000000000000, 0.8660254037844387076, 1.000000000000000000, 0.8660254037844387076, 1.000000000000000000, 0.8660254037844387076, 1.000000000000000000, 0.8660254037844387076, 1.000000000000000000, 0.8660254037844387076, 1.000000000000000000, 0.8660254037844387076, 1.000000000000000000, 0.8660254037844387076, 1.000000000000000000, 0.8660254037844387076, 1.000000000000000000, 0.8660254037844387076, 1.000000000000000000, 0.8660254037844387076, 1.000000000000000000, 0.8660254037844387076, 1.000000000000000000, 0.8660254037844387076, 1.000000000000000000, 0.8660254037844387076, 1.000000000000000000, 0.8660254037844387076, 1.000000000000000000, 0.8660254037844387076, 1.000000000000000000, 0.8660254037844387076, 1.000000000000000000, 0.8660254037844387076, 1.000000000000000000, 0.8660254037844387076, 1.000000000000000000, 0.8660254037844387076, 1.000000000000000000, 0.8660254037844387076, 1.000000000000000000, 0.8660254037844387076, 1.000000000000000000, 0.8660254037844387076, 1.000000000000000000, 0.8660254037844387076, 1.000000000000000000, 0.8660254037844387076, 1.000000000000000000, 0.8660254037844387076, 1.000000000000000000, 0.8660254037844387076, 1.000000000000000000, 0.8660254037844387076, 1.000000000000000000, 0.8660254037844387076, 1.000000000000000000, 0.8660254037844387076, 1.000000000000000000, 0.8660254037844387076, 1.000000000000000000, 0.8660254037844387076, 1.000000000000000000, 0.8660254037844387076, 1.000000000000000000, 0.8660254037844387076, 1.000000000000000000, 0.8660254037844387076, 1.000000000000000000, 0.8660254037844387076, 1.000000000000000000, 0.8660254037844387076, 1.000000000000000000, 0.8660254037844387076, 1.000000000000000000, 0.8660254037844387076, 1.000000000000000000, 0.8660254037844387076, 1.000000000000000000, 0.8660254037844387076, 1.000000000000000000, 0.8660254037844387076, 1.000000000000000000, 0.8660254037844387076, 1.000000000000000000, 0.8660254037844387076, 1.000000000000000000, 0.8660254037844387076, 1.000000000000000000, 0.8660254037844387076, 1.000000000000000000, 0.8660254037844387076, 1.000000000000000000, 0.8660254037844387076, 1.000000000000000000, 0.8660254037844387076, 1.000000000000000000, 0.8660254037844387076, 1.000000000000000000, 0.8660254037844387076, 1.000000000000000000, 0.8660254037844387076, 1.000000000000000000, 0.8660254037844387076, 1.000000000000000000, 0.8660254037844387076, 1.000000000000000000, 0.8660254037844387076, 1.000000000000000000, 0.8660254037844387076, 1.000000000000000000, 0.8660254037844387076, 1.000000000000000000, 0.8660254037844387076, 1.000000000000000000, 0.8660254037844387076, 1.000000000000000000, 0.8660254037844387076, 1.000000000000000000, 0.8660254037844387076, 1.000000000000000000, 0.8660254037844387076, 1.000000000000000000, 0.8660254037844387076, 1.000000000000000000, 0.8660254037844387076, 1.000000000000000000, 0.8660254037844387076, 1.000000000000000000, 0.8660254037844387076, 1.000000000000000000, 0.8660254037844387076, 1.000000000000000000, 0.8660254037844387076, 1.000000000000000000, 0.8660254037844387076, 1.000000000000000000, 0.8660254037844387076, 1.000000000000000000, 0.8660254037844387076, 1.000000000000000000, 0.8660254037844387076, 1.000000000000000000, 0.8660254037844387076, 1.000000000000000000, 0.8660254037844387076, 1.000000000000000000, 0.8660254037844387076, 1.000000000000000000, 0.8660254037844387076, 1.000000000000000000, 0.8660254037844387076, 1.000000000000000000, 0.8660254037844387076, 1.000000000000000000, 0.8660254037844387076, 1.000000000000000000, 0.8660254037844387076, 1.000000000000000000, 0.8660254037844387076, 1.000000000000000000, 0.8660254037844387076, 1.000000000000000000, 0.8660254037844387076, 1.000000000000000000, 0.8660254037844387076, 1.000000000000000000, 0.8660254037844387076, 1.000000000000000000, 0.8660254037844387076, 1.000000000000000000, 0.8660254037844387076, 1.000000000000000000, 0.8660254037844387076, 1.000000000000000000, 0.8660254037844387076, 1.000000000000000000, 0.8660254037844387076, 1.000000000000000000, 0.8660254037844387076, 1.000000000000000000, 0.8660254037844387076, 1.000000000000000000, 0.8660254037844387076, 1.000000000000000000, 0.8660254037844387076, 1.000000000000000000, 0.8660254037844387076, 1.000000000000000000, 0.8660254037844387076, 1.000000000000000000, 0.8660254037844387076, 1.000000000000000000, 0.8660254037844387076, 1.000000000000000000, 0.8660254037844387076, 1.000000000000000000, 0.8660254037844387076, 1.000000000000000000, 0.8660254037844387076, 1.000000000000000000, 0.8660254037844387076, 1.000000000000000000, 0.8660254037844387076, 1.000000000000000000, 0.8660254037844387076, 1.000000000000000000, 0.8660254037844387076, 1.000000000000000000, 0.8660254037844387076, 1.000000000000000000, 0.8660254037844387076, 1.000000000000000000, 0.8660254037844387076, 1.000000000000000000, 0.8660254037844387076, 1.000000000000000000, 0.8660254037844387076, 1.000000000000000000, 0.8660254037844387076, 1.000000000000000000, 0.8660254037844387076, 1.000000000000000000, 0.8660254037844387076, 1.000000000000000000, 0.8660254037844387076, 1.000000000000000000, 0.8660254037844387076, 1.000000000000000000, 0.8660254037844387076, 1.000000000000000000, 0.8660254037844387076, 1.000000000000000000, 0.8660254037844387076, 1.000000000000000000, 0.8660254037844387076, 1.000000000000000000, 0.8660254037844387076, 1.000000000000000000, 0.8660254037844387076, 1.000000000000000000, 0.8660254037844387076, 1.000000000000000000, 0.8660254037844387076, 1.000000000000000000, 0.8660254037844387076, 1.000000000000000000, 0.8660254037844387076, 1.000000000000000000, 0.8660254037844387076, 1.000000000000000000, 0.8660254037844387076, 1.000000000000000000, 0.8660254037844387076, 1.000000000000000000, 0.8660254037844387076, 1.000000000000000000, 0.8660254037844387076, 1.000000000000000000, 0.8660254037844387076, 1.000000000000000000, 0.8660254037844387076, 1.000000000000000000, 0.8660254037844387076, 1.000000000000000000, 0.8660254037844387076, 1.000000000000000000, 0.8660254037844387076, 1.000000000000000000, 0.8660254037844387076, 1.000000000000000000, 0.8660254037844387076, 1.000000000000000000, 0.8660254037844387076, 1.000000000000000000, 0.8660254037844387076, 1.000000000000000000, 0.8660254037844387076, 1.000000000000000000, 0.8660254037844387076, 1.000000000000000000, 0.8660254037844387076, 1.000000000000000000, 0.8660254037844387076, 1.000000000000000000, 0.8660254037844387076, 1.000000000000000000, 0.8660254037844387076, 1.000000000000000000, 0.8660254037844387076, 1.000000000000000000, 0.8660254037844387076, 1.000000000000000000, 0.8660254037844387076, 1.000000000000000000, 0.8660254037844387076, 1.000000000000000000, 0.8660254037844387076, 1.000000000000000000, 0.8660254037844387076, 1.000000000000000000, 0.8660254037844387076, 1.000000000000000000, 0.8660254037844387076, 1.000000000000000000, 0.8660254037844387076, 1.000000000000000000, 0.8660254037844387076, 1.000000000000000000, 0.8660254037844387076, 1.000000000000000000, 0.8660254037844387076, 1.000000000000000000, 0.8660254037844387076, 1.000000000000000000, 0.8660254037844387076, 1.000000000000000000, 0.8660254037844387076, 1.000000000000000000, 0.8660254037844387076, 1.000000000000000000, 0.8660254037844387076, 1.000000000000000000, 0.8660254037844387076, 1.000000000000000000, 0.8660254037844387076, 1.000000000000000000, 0.8660254037844387076, 1.000000000000000000, 0.8660254037844387076, 1.000000000000000000, 0.8660254037844387076, 1.000000000000000000, 0.8660254037844387076, 1.000000000000000000, 0.8660254037844387076, 1.000000000000000000, 0.8660254037844387076, 1.000000000000000000, 0.8660254037844387076, 1.000000000000000000, 0.8660254037844387076, 1.000000000000000000, 0.8660254037844387076, 1.000000000000000000, 0.8660254037844387076, 1.000000000000000000, 0.8660254037844387076, 1.000000000000000000, 0.8660254037844387076, 1.000000000000000000, 0.8660254037844387076, 1.000000000000000000, 0.8660254037844387076, 1.000000000000000000, 0.8660254037844387076, 1.000000000000000000, 0.8660254037844387076, 1.000000000000000000, 0.8660254037844387076, 1.000000000000000000, 0.8660254037844387076, 1.000000000000000000, 0.8660254037844387076, 1.000000000000000000, 0.8660254037844387076, 1.000000000000000000, 0.8660254037844387076, 1.000000000000000000, 0.8660254037844387076, 1.000000000000000000, 0.8660254037844387076, 1.000000000000000000, 0.8660254037844387076, 1.000000000000000000, 0.8660254037844387076, 1.000000000000000000, 0.8660254037844387076, 1.000000000000000000, 0.8660254037844387076, 1.000000000000000000, 0.8660254037844387076, 1.000000000000000000, 0.8660254037844387076, 1.000000000000000000, 0.8660254037844387076, 1.000000000000000000, 0.8660254037844387076, 1.000000000000000000, 0.8660254037844387076, 1.000000000000000000, 0.8660254037844387076, 1.000000000000000000, 0.8660254037844387076, 1.000000000000000000, 0.8660254037844387076, 1.000000000000000000, 0.8660254037844387076, 1.000000000000000000, 0.8660254037844387076, 1.000000000000000000, 0.8660254037844387076, 1.000000000000000000, 0.8660254037844387076, 1.000000000000000000, 0.8660254037844387076, 1.000000000000000000, 0.8660254037844387076, 1.000000000000000000, 0.8660254037844387076, 1.000000000000000000, 0.8660254037844387076, 1.000000000000000000, 0.8660254037844387076, 1.000000000000000000, 0.8660254037844387076, 1.000000000000000000, 0.8660254037844387076, 1.000000000000000000, 0.8660254037844387076, 1.000000000000000000, 0.8660254037844387076, 1.000000000000000000, 0.8660254037844387076, 1.000000000000000000, 0.8660254037844387076, 1.000000000000000000, 0.8660254037844387076, 1.000000000000000000, 0.8660254037844387076, 1.000000000000000000, 0.8660254037844387076, 1.000000000000000000, 0.8660254037844387076, 1.000000000000000000, 0.8660254037844387076, 1.000000000000000000, 0.8660254037844387076, 1.000000000000000000, 0.8660254037844387076, 1.000000000000000000, 0.8660254037844387076, 1.000000000000000000, 0.8660254037844387076, 1.000000000000000000, 0.8660254037844387076, 1.000000000000000000, 0.8660254037844387076, 1.000000000000000000, 0.8660254037844387076, 1.000000000000000000, 0.8660254037844387076, 1.000000000000000000, 0.8660254037844387076, 1.000000000000000000, 0.8660254037844387076, 1.000000000000000000, 0.8660254037844387076, 1.000000000000000000, 0.8660254037844387076, 1.000000000000000000, 0.8660254037844387076, 1.000000000000000000, 0.8660254037844387076, 1.000000000000000000, 0.8660254037844387076, 1.000000000000000000, 0.8660254037844387076, 1.000000000000000000, 0.8660254037844387076, 1.000000000000000000, 0.8660254037844387076, 1.000000000000000000, 0.8660254037844387076, 1.000000000000000000, 0.8660254037844387076, 1.000000000000000000, 0.8660254037844387076, 1.000000000000000000, 0.8660254037844387076, 1.000000000000000000, 0.8660254037844387076, 1.000000000000000000, 0.8660254037844387076, 1.000000000000000000, 0.8660254037844387076, 1.000000000000000000, 0.8660254037844387076, 1.000000000000000000, 0.8660254037844387076, 1.000000000000000000, 0.8660254037844387076, 1.000000000000000000, 0.8660254037844387076, 1.000000000000000000, 0.8660254037844387076, 1.000000000000000000, 0.8660254037844387076, 1.000000000000000000, 0.8660254037844387076, 1.000000000000000000, 0.8660254037844387076, 1.000000000000000000, 0.8660254037844387076, 1.000000000000000000, 0.8660254037844387076, 1.000000000000000000, 0.8660254037844387076, 1.000000000000000000, 0.8660254037844387076, 1.000000000000000000, 0.8660254037844387076, 1.000000000000000000, 0.8660254037844387076, 1.000000000000000000, 0.8660254037844387076, 1.000000000000000000, 0.8660254037844387076, 1.000000000000000000, 0.8660254037844387076, 1.000000000000000000, 0.8660254037844387076, 1.000000000000000000, 0.8660254037844387076, 1.000000000000000000, 0.8660254037844387076, 1.000000000000000000, 0.8660254037844387076, 1.000000000000000000, 0.8660254037844387076, 1.000000000000000000, 0.8660254037844387076, 1.000000000000000000, 0.8660254037844387076, 1.000000000000000000, 0.8660254037844387076, 1.000000000000000000, 0.8660254037844387076, 1.000000000000000000, 0.8660254037844387076, 1.000000000000000000, 0.8660254037844387076, 1.000000000000000000, 0.8660254037844387076, 1.000000000000000000, 0.8660254037844387076, 1.000000000000000000, 0.8660254037844387076, 1.000000000000000000, 0.8660254037844387076, 1.000000000000000000, 0.8660254037844387076, 1.000000000000000000, 0.8660254037844387076, 1.000000000000000000, 0.8660254037844387076, 1.000000000000000000, 0.8660254037844387076, 1.000000000000000000, 0.8660254037844387076, 1.000000000000000000),
 ( 1.000000000000000000, 0.8660254037844387076, 1.000000000000000000, 0.8660254037844387076, 1.000000000000000000, 0.8660254037844387076, 1.000000000000000000, 0.8660254037844387076, 1.000000000000000000, 0.8660254037844387076, 1.000000000000000000, 0.8660254037844387076, 1.000000000000000000, 0.8660254037844387076, 1.000000000000000000, 0.8660254037844387076, 1.000000000000000000, 0.8660254037844387076, 1.000000000000000000, 0.8660254037844387076, 1.000000000000000000, 0.8660254037844387076, 1.000000000000000000, 0.8660254037844387076, 1.000000000000000000, 0.8660254037844387076, 1.000000000000000000, 0.8660254037844387076, 1.000000000000000000, 0.8660254037844387076, 1.000000000000000000, 0.8660254037844387076, 1.000000000000000000, 0.8660254037844387076, 1.000000000000000000, 0.8660254037844387076, 1.000000000000000000, 0.8660254037844387076, 1.000000000000000000, 0.8660254037844387076, 1.000000000000000000, 0.8660254037844387076, 1.000000000000000000, 0.8660254037844387076, 1.000000000000000000, 0.8660254037844387076, 1.000000000000000000, 0.8660254037844387076, 1.000000000000000000, 0.8660254037844387076, 1.000000000000000000, 0.8660254037844387076, 1.000000000000000000, 0.8660254037844387076, 1.000000000000000000, 0.8660254037844387076, 1.000000000000000000, 0.8660254037844387076, 1.000000000000000000, 0.8660254037844387076, 1.000000000000000000, 0.8660254037844387076, 1.000000000000000000, 0.8660254037844387076, 1.000000000000000000, 0.8660254037844387076, 1.000000000000000000, 0.8660254037844387076, 1.000000000000000000, 0.8660254037844387076, 1.000000000000000000, 0.8660254037844387076, 1.000000000000000000, 0.8660254037844387076, 1.000000000000000000, 0.8660254037844387076, 1.000000000000000000, 0.8660254037844387076, 1.000000000000000000, 0.8660254037844387076, 1.000000000000000000, 0.8660254037844387076, 1.000000000000000000, 0.8660254037844387076, 1.000000000000000000, 0.8660254037844387076, 1.000000000000000000, 0.8660254037844387076, 1.000000000000000000, 0.8660254037844387076, 1.000000000000000000, 0.8660254037844387076, 1.000000000000000000, 0.8660254037844387076, 1.000000000000000000, 0.8660254037844387076, 1.000000000000000000, 0.8660254037844387076, 1.000000000000000000, 0.8660254037844387076, 1.000000000000000000, 0.8660254037844387076, 1.000000000000000000, 0.8660254037844387076, 1.000000000000000000, 0.8660254037844387076, 1.000000000000000000, 0.8660254037844387076, 1.000000000000000000, 0.8660254037844387076, 1.000000000000000000, 0.8660254037844387076, 1.000000000000000000, 0.8660254037844387076, 1.000000000000000000, 0.8660254037844387076, 1.000000000000000000, 0.8660254037844387076, 1.000000000000000000, 0.8660254037844387076, 1.000000000000000000, 0.8660254037844387076, 1.000000000000000000, 0.8660254037844387076, 1.000000000000000000, 0.8660254037844387076, 1.000000000000000000, 0.8660254037844387076, 1.000000000000000000, 0.8660254037844387076, 1.000000000000000000, 0.8660254037844387076, 1.000000000000000000, 0.8660254037844387076, 1.000000000000000000, 0.8660254037844387076, 1.000000000000000000, 0.8660254037844387076, 1.000000000000000000, 0.8660254037844387076, 1.000000000000000000, 0.8660254037844387076, 1.000000000000000000, 0.8660254037844387076, 1.000000000000000000, 0.8660254037844387076, 1.000000000000000000, 0.8660254037844387076, 1.000000000000000000, 0.8660254037844387076, 1.000000000000000000, 0.8660254037844387076, 1.000000000000000000, 0.8660254037844387076, 1.000000000000000000, 0.8660254037844387076, 1.000000000000000000, 0.8660254037844387076, 1.000000000000000000, 0.8660254037844387076, 1.000000000000000000, 0.8660254037844387076, 1.000000000000000000, 0.8660254037844387076, 1.000000000000000000, 0.8660254037844387076, 1.000000000000000000, 0.8660254037844387076, 1.000000000000000000, 0.8660254037844387076, 1.000000000000000000, 0.8660254037844387076, 1.000000000000000000, 0.8660254037844387076, 1.000000000000000000, 0.8660254037844387076, 1.000000000000000000, 0.8660254037844387076, 1.000000000000000000, 0.8660254037844387076, 1.000000000000000000, 0.8660254037844387076, 1.000000000000000000, 0.8660254037844387076, 1.000000000000000000, 0.8660254037844387076, 1.000000000000000000, 0.8660254037844387076, 1.000000000000000000, 0.8660254037844387076, 1.000000000000000000, 0.8660254037844387076, 1.000000000000000000, 0.8660254037844387076, 1.000000000000000000, 0.8660254037844387076, 1.000000000000000000, 0.8660254037844387076, 1.000000000000000000, 0.8660254037844387076, 1.000000000000000000, 0.8660254037844387076, 1.000000000000000000, 0.8660254037844387076, 1.000000000000000000, 0.8660254037844387076, 1.000000000000000000, 0.8660254037844387076, 1.000000000000000000, 0.8660254037844387076, 1.000000000000000000, 0.8660254037844387076, 1.000000000000000000, 0.8660254037844387076, 1.000000000000000000, 0.8660254037844387076, 1.000000000000000000, 0.8660254037844387076, 1.000000000000000000, 0.8660254037844387076, 1.000000000000000000, 0.8660254037844387076, 1.000000000000000000, 0.8660254037844387076, 1.000000000000000000, 0.8660254037844387076, 1.000000000000000000, 0.8660254037844387076, 1.000000000000000000, 0.8660254037844387076, 1.000000000000000000, 0.8660254037844387076, 1.000000000000000000, 0.8660254037844387076, 1.000000000000000000, 0.8660254037844387076, 1.000000000000000000, 0.8660254037844387076, 1.000000000000000000, 0.8660254037844387076, 1.000000000000000000, 0.8660254037844387076, 1.000000000000000000, 0.8660254037844387076, 1.000000000000000000, 0.8660254037844387076, 1.000000000000000000, 0.8660254037844387076, 1.000000000000000000, 0.8660254037844387076, 1.000000000000000000, 0.8660254037844387076, 1.000000000000000000, 0.8660254037844387076, 1.000000000000000000, 0.8660254037844387076, 1.000000000000000000, 0.8660254037844387076, 1.000000000000000000, 0.8660254037844387076, 1.000000000000000000, 0.8660254037844387076, 1.000000000000000000, 0.8660254037844387076, 1.000000000000000000, 0.8660254037844387076, 1.000000000000000000, 0.8660254037844387076, 1.000000000000000000, 0.8660254037844387076, 1.000000000000000000, 0.8660254037844387076, 1.000000000000000000, 0.8660254037844387076, 1.000000000000000000, 0.8660254037844387076, 1.000000000000000000, 0.8660254037844387076, 1.000000000000000000, 0.8660254037844387076, 1.000000000000000000, 0.8660254037844387076, 1.000000000000000000, 0.8660254037844387076, 1.000000000000000000, 0.8660254037844387076, 1.000000000000000000, 0.8660254037844387076, 1.000000000000000000, 0.8660254037844387076, 1.000000000000000000, 0.8660254037844387076, 1.000000000000000000, 0.8660254037844387076, 1.000000000000000000, 0.8660254037844387076, 1.000000000000000000, 0.8660254037844387076, 1.000000000000000000, 0.8660254037844387076, 1.000000000000000000, 0.8660254037844387076, 1.000000000000000000, 0.8660254037844387076, 1.000000000000000000, 0.8660254037844387076, 1.000000000000000000, 0.8660254037844387076, 1.000000000000000000, 0.8660254037844387076, 1.000000000000000000, 0.8660254037844387076, 1.000000000000000000, 0.8660254037844387076, 1.000000000000000000, 0.8660254037844387076, 1.000000000000000000, 0.8660254037844387076, 1.000000000000000000, 0.8660254037844387076, 1.000000000000000000, 0.8660254037844387076, 1.000000000000000000, 0.8660254037844387076, 1.000000000000000000, 0.8660254037844387076, 1.000000000000000000, 0.8660254037844387076, 1.000000000000000000, 0.8660254037844387076, 1.000000000000000000, 0.8660254037844387076, 1.000000000000000000, 0.8660254037844387076, 1.000000000000000000, 0.8660254037844387076, 1.000000000000000000, 0.8660254037844387076, 1.000000000000000000, 0.8660254037844387076, 1.000000000000000000, 0.8660254037844387076, 1.000000000000000000, 0.8660254037844387076, 1.000000000000000000, 0.8660254037844387076, 1.000000000000000000, 0.8660254037844387076, 1.000000000000000000, 0.8660254037844387076, 1.000000000000000000, 0.8660254037844387076, 1.000000000000000000, 0.8660254037844387076, 1.000000000000000000, 0.8660254037844387076, 1.000000000000000000, 0.8660254037844387076, 1.000000000000000000, 0.8660254037844387076, 1.000000000000000000, 0.8660254037844387076, 1.000000000000000000, 0.8660254037844387076, 1.000000000000000000, 0.8660254037844387076, 1.000000000000000000, 0.8660254037844387076, 1.000000000000000000, 0.8660254037844387076, 1.000000000000000000, 0.8660254037844387076, 1.000000000000000000, 0.8660254037844387076, 1.000000000000000000, 0.8660254037844387076, 1.000000000000000000, 0.8660254037844387076, 1.000000000000000000, 0.8660254037844387076, 1.000000000000000000, 0.8660254037844387076, 1.000000000000000000, 0.8660254037844387076, 1.000000000000000000, 0.8660254037844387076, 1.000000000000000000, 0.8660254037844387076, 1.000000000000000000, 0.8660254037844387076, 1.000000000000000000, 0.8660254037844387076, 1.000000000000000000, 0.8660254037844387076, 1.000000000000000000, 0.8660254037844387076, 1.000000000000000000, 0.8660254037844387076, 1.000000000000000000, 0.8660254037844387076, 1.000000000000000000, 0.8660254037844387076, 1.000000000000000000, 0.8660254037844387076, 1.000000000000000000, 0.8660254037844387076, 1.000000000000000000, 0.8660254037844387076, 1.000000000000000000, 0.8660254037844387076, 1.000000000000000000, 0.8660254037844387076, 1.000000000000000000, 0.8660254037844387076, 1.000000000000000000, 0.8660254037844387076, 1.000000000000000000, 0.8660254037844387076, 1.000000000000000000, 0.8660254037844387076, 1.000000000000000000, 0.8660254037844387076, 1.000000000000000000, 0.8660254037844387076, 1.000000000000000000, 0.8660254037844387076, 1.000000000000000000, 0.8660254037844387076, 1.000000000000000000, 0.8660254037844387076, 1.000000000000000000, 0.8660254037844387076, 1.000000000000000000, 0.8660254037844387076, 1.000000000000000000, 0.8660254037844387076, 1.000000000000000000, 0.8660254037844387076, 1.000000000000000000, 0.8660254037844387076, 1.000000000000000000, 0.8660254037844387076, 1.000000000000000000, 0.8660254037844387076, 1.000000000000000000, 0.8660254037844387076, 1.000000000000000000, 0.8660254037844387076, 1.000000000000000000, 0.8660254037844387076, 1.000000000000000000, 0.8660254037844387076, 1.000000000000000000, 0.8660254037844387076, 1.000000000000000000, 0.8660254037844387076, 1.000000000000000000, 0.8660254037844387076, 1.000000000000000000, 0.8660254037844387076, 1.000000000000000000, 0.8660254037844387076, 1.000000000000000000, 0.8660254037844387076, 1.000000000000000000, 0.8660254037844387076, 1.000000000000000000, 0.8660254037844387076, 1.000000000000000000, 0.8660254037844387076, 1.000000000000000000, 0.8660254037844387076, 1.000000000000000000, 0.8660254037844387076, 1.000000000000000000, 0.8660254037844387076, 1.000000000000000000, 0.8660254037844387076, 1.000000000000000000, 0.8660254037844387076, 1.000000000000000000, 0.8660254037844387076, 1.000000000000000000, 0.8660254037844387076, 1.000000000000000000, 0.8660254037844387076, 1.000000000000000000, 0.8660254037844387076, 1.000000000000000000, 0.8660254037844387076, 1.000000000000000000, 0.8660254037844387076, 1.000000000000000000, 0.8660254037844387076, 1.000000000000000000, 0.8660254037844387076, 1.000000000000000000, 0.8660254037844387076, 1.000000000000000000, 0.8660254037844387076, 1.000000000000000000, 0.8660254037844387076, 1.000000000000000000, 0.8660254037844387076, 1.000000000000000000, 0.8660254037844387076, 1.000000000000000000, 0.8660254037844387076, 1.000000000000000000, 0.8660254037844387076, 1.000000000000000000, 0.8660254037844387076, 1.000000000000000000, 0.8660254037844387076, 1.000000000000000000, 0.8660254037844387076, 1.000000000000000000, 0.8660254037844387076, 1.000000000000000000, 0.8660254037844387076, 1.000000000000000000, 0.8660254037844387076, 1.000000000000000000, 0.8660254037844387076, 1.000000000000000000, 0.8660254037844387076, 1.000000000000000000, 0.8660254037844387076, 1.000000000000000000, 0.8660254037844387076, 1.000000000000000000, 0.8660254037844387076, 1.000000000000000000, 0.8660254037844387076, 1.000000000000000000, 0.8660254037844387076, 1.000000000000000000, 0.8660254037844387076, 1.000000000000000000, 0.8660254037844387076, 1.000000000000000000, 0.8660254037844387076, 1.000000000000000000, 0.8660254037844387076, 1.000000000000000000, 0.8660254037844387076, 1.000000000000000000, 0.8660254037844387076, 1.000000000000000000, 0.8660254037844387076, 1.000000000000000000, 0.8660254037844387076, 1.000000000000000000, 0.8660254037844387076, 1.000000000000000000, 0.8660254037844387076, 1.000000000000000000, 0.8660254037844387076, 1.000000000000000000, 0.8660254037844387076, 1.000000000000000000, 0.8660254037844387076, 1.000000000000000000, 0.8660254037844387076, 1.000000000000000000, 0.8660254037844387076, 1.000000000000000000, 0.8660254037844387076, 1.000000000000000000, 0.8660254037844387076, 1.000000000000000000, 0.8660254037844387076, 1.000000000000000000, 0.8660254037844387076, 1.000000000000000000, 0.8660254037844387076, 1.000000000000000000, 0.8660254037844387076, 1.000000000000000000, 0.8660254037844387076, 1.000000000000000000, 0.8660254037844387076, 1.000000000000000000, 0.8660254037844387076, 1.000000000000000000, 0.8660254037844387076, 1.000000000000000000, 0.8660254037844387076, 1.000000000000000000, 0.8660254037844387076, 1.000000000000000000, 0.8660254037844387076, 1.000000000000000000, 0.8660254037844387076, 1.000000000000000000, 0.8660254037844387076, 1.000000000000000000, 0.8660254037844387076, 1.000000000000000000, 0.8660254037844387076, 1.000000000000000000, 0.8660254037844387076, 1.000000000000000000, 0.8660254037844387076, 1.000000000000000000, 0.8660254037844387076, 1.000000000000000000, 0.8660254037844387076, 1.000000000000000000, 0.8660254037844387076, 1.000000000000000000, 0.8660254037844387076, 1.000000000000000000, 0.8660254037844387076, 1.000000000000000000, 0.8660254037844387076, 1.000000000000000000, 0.8660254037844387076, 1.000000000000000000, 0.8660254037844387076, 1.000000000000000000, 0.8660254037844387076, 1.000000000000000000, 0.8660254037844387076, 1.000000000000000000, 0.8660254037844387076, 1.000000000000000000, 0.8660254037844387076, 1.000000000000000000, 0.8660254037844387076, 1.000000000000000000, 0.8660254037844387076, 1.000000000000000000, 0.8660254037844387076, 1.000000000000000000, 0.8660254037844387076, 1.000000000000000000, 0.8660254037844387076, 1.000000000000000000, 0.8660254037844387076, 1.000000000000000000, 0.8660254037844387076, 1.000000000000000000, 0.8660254037844387076, 1.000000000000000000, 0.8660254037844387076, 1.000000000000000000, 0.8660254037844387076, 1.000000000000000000, 0.8660254037844387076, 1.000000000000000000, 0.8660254037844387076, 1.000000000000000000, 0.8660254037844387076, 1.000000000000000000, 0.8660254037844387076, 1.000000000000000000, 0.8660254037844387076, 1.000000000000000000, 0.8660254037844387076, 1.000000000000000000, 0.8660254037844387076, 1.000000000000000000, 0.8660254037844387076, 1.000000000000000000, 0.8660254037844387076, 1.000000000000000000, 0.8660254037844387076, 1.000000000000000000, 0.8660254037844387076, 1.000000000000000000, 0.8660254037844387076, 1.000000000000000000, 0.8660254037844387076, 1.000000000000000000, 0.8660254037844387076, 1.000000000000000000, 0.8660254037844387076, 1.000000000000000000, 0.8660254037844387076, 1.000000000000000000, 0.8660254037844387076, 1.000000000000000000, 0.8660254037844387076, 1.000000000000000000, 0.8660254037844387076, 1.000000000000000000, 0.8660254037844387076, 1.000000000000000000, 0.8660254037844387076, 1.000000000000000000, 0.8660254037844387076, 1.000000000000000000, 0.8660254037844387076, 1.000000000000000000, 0.8660254037844387076, 1.000000000000000000, 0.8660254037844387076, 1.000000000000000000, 0.8660254037844387076, 1.000000000000000000, 0.8660254037844387076, 1.000000000000000000, 0.8660254037844387076, 1.000000000000000000, 0.8660254037844387076, 1.000000000000000000, 0.8660254037844387076, 1.000000000000000000, 0.8660254037844387076, 1.000000000000000000, 0.8660254037844387076, 1.000000000000000000, 0.8660254037844387076, 1.000000000000000000, 0.8660254037844387076, 1.000000000000000000, 0.8660254037844387076, 1.000000000000000000, 0.8660254037844387076, 1.000000000000000000, 0.8660254037844387076, 1.000000000000000000, 0.8660254037844387076, 1.000000000000000000, 0.8660254037844387076, 1.000000000000000000, 0.8660254037844387076, 1.000000000000000000, 0.8660254037844387076, 1.000000000000000000, 0.8660254037844387076, 1.000000000000000000, 0.8660254037844387076, 1.000000000000000000, 0.8660254037844387076, 1.000000000000000000, 0.8660254037844387076, 1.000000000000000000, 0.8660254037844387076, 1.000000000000000000, 0.8660254037844387076, 1.000000000000000000, 0.8660254037844387076, 1.000000000000000000, 0.8660254037844387076, 1.000000000000000000, 0.8660254037844387076, 1.000000000000000000, 0.8660254037844387076, 1.000000000000000000, 0.8660254037844387076, 1.000000000000000000, 0.8660254037844387076, 1.000000000000000000, 0.8660254037844387076, 1.000000000000000000, 0.8660254037844387076, 1.000000000000000000, 0.8660254037844387076, 1.000000000000000000, 0.8660254037844387076, 1.000000000000000000, 0.8660254037844387076, 1.000000000000000000, 0.8660254037844387076, 1.000000000000000000, 0.8660254037844387076, 1.000000000000000000, 0.8660254037844387076, 1.000000000000000000, 0.8660254037844387076, 1.000000000000000000, 0.8660254037844387076, 1.000000000000000000, 0.8660254037844387076, 1.000000000000000000, 0.8660254037844387076, 1.000000000000000000, 0.8660254037844387076, 1.000000000000000000, 0.8660254037844387076, 1.000000000000000000, 0.8660254037844387076, 1.000000000000000000, 0.8660254037844387076, 1.000000000000000000, 0.8660254037844387076, 1.000000000000000000, 0.8660254037844387076, 1.000000000000000000, 0.8660254037844387076, 1.000000000000000000, 0.8660254037844387076, 1.000000000000000000, 0.8660254037844387076, 1.000000000000000000, 0.8660254037844387076, 1.000000000000000000, 0.8660254037844387076, 1.000000000000000000, 0.8660254037844387076, 1.000000000000000000, 0.8660254037844387076, 1.000000000000000000, 0.8660254037844387076, 1.000000000000000000, 0.8660254037844387076, 1.000000000000000000, 0.8660254037844387076, 1.000000000000000000, 0.8660254037844387076, 1.000000000000000000, 0.8660254037844387076, 1.000000000000000000, 0.8660254037844387076, 1.000000000000000000, 0.8660254037844387076, 1.000000000000000000, 0.8660254037844387076, 1.000000000000000000, 0.8660254037844387076, 1.000000000000000000, 0.8660254037844387076, 1.000000000000000000, 0.8660254037844387076, 1.000000000000000000, 0.8660254037844387076, 1.000000000000000000, 0.8660254037844387076, 1.000000000000000000, 0.8660254037844387076, 1.000000000000000000, 0.8660254037844387076, 1.000000000000000000, 0.8660254037844387076, 1.000000000000000000, 0.8660254037844387076, 1.000000000000000000, 0.8660254037844387076, 1.000000000000000000, 0.8660254037844387076, 1.000000000000000000, 0.8660254037844387076, 1.000000000000000000, 0.8660254037844387076, 1.000000000000000000, 0.8660254037844387076, 1.000000000000000000, 0.8660254037844387076, 1.000000000000000000, 0.8660254037844387076, 1.000000000000000000, 0.8660254037844387076, 1.000000000000000000, 0.8660254037844387076, 1.000000000000000000, 0.8660254037844387076, 1.000000000000000000, 0.8660254037844387076, 1.000000000000000000, 0.8660254037844387076, 1.000000000000000000, 0.8660254037844387076, 1.000000000000000000, 0.8660254037844387076, 1.000000000000000000, 0.8660254037844387076, 1.000000000000000000, 0.8660254037844387076, 1.000000000000000000, 0.8660254037844387076, 1.000000000000000000, 0.8660254037844387076, 1.000000000000000000, 0.8660254037844387076, 1.000000000000000000, 0.8660254037844387076, 1.000000000000000000, 0.8660254037844387076, 1.000000000000000000, 0.8660254037844387076, 1.000000000000000000, 0.8660254037844387076, 1.000000000000000000, 0.8660254037844387076, 1.000000000000000000, 0.8660254037844387076, 1.000000000000000000, 0.8660254037844387076, 1.000000000000000000, 0.8660254037844387076, 1.000000000000000000, 0.8660254037844387076, 1.000000000000000000, 0.8660254037844387076, 1.000000000000000000, 0.8660254037844387076, 1.000000000000000000, 0.8660254037844387076, 1.000000000000000000, 0.8660254037844387076, 1.000000000000000000, 0.8660254037844387076, 1.000000000000000000, 0.8660254037844387076, 1.000000000000000000, 0.8660254037844387076, 1.000000000000000000, 0.8660254037844387076, 1.000000000000000000, 0.8660254037844387076, 1.000000000000000000, 0.8660254037844387076, 1.000000000000000000, 0.8660254037844387076, 1.000000000000000000, 0.8660254037844387076, 1.000000000000000000, 0.8660254037844387076, 1.000000000000000000, 0.8660254037844387076, 1.000000000000000000, 0.8660254037844387076, 1.000000000000000000, 0.8660254037844387076, 1.000000000000000000, 0.8660254037844387076, 1.000000000000000000, 0.8660254037844387076, 1.000000000000000000, 0.8660254037844387076, 1.000000000000000000, 0.8660254037844387076, 1.000000000000000000, 0.8660254037844387076, 1.000000000000000000, 0.8660254037844387076, 1.000000000000000000, 0.8660254037844387076, 1.000000000000000000, 0.8660254037844387076, 1.000000000000000000, 0.8660254037844387076, 1.000000000000000000, 0.8660254037844387076, 1.000000000000000000, 0.8660254037844387076, 1.000000000000000000, 0.8660254037844387076, 1.000000000000000000, 0.8660254037844387076, 1.000000000000000000, 0.8660254037844387076, 1.000000000000000000, 0.8660254037844387076, 1.000000000000000000, 0.8660254037844387076, 1.000000000000000000, 0.8660254037844387076, 1.000000000000000000, 0.8660254037844387076, 1.000000000000000000, 0.8660254037844387076, 1.000000000000000000, 0.8660254037844387076, 1.000000000000000000, 0.8660254037844387076, 1.000000000000000000, 0.8660254037844387076, 1.000000000000000000, 0.8660254037844387076, 1.000000000000000000, 0.8660254037844387076, 1.000000000000000000, 0.8660254037844387076, 1.000000000000000000, 0.8660254037844387076, 1.000000000000000000, 0.8660254037844387076, 1.000000000000000000, 0.8660254037844387076, 1.000000000000000000, 0.8660254037844387076, 1.000000000000000000, 0.8660254037844387076, 1.000000000000000000, 0.8660254037844387076, 1.000000000000000000, 0.8660254037844387076, 1.000000000000000000, 0.8660254037844387076, 1.000000000000000000, 0.8660254037844387076, 1.000000000000000000, 0.8660254037844387076, 1.000000000000000000, 0.8660254037844387076, 1.000000000000000000, 0.8660254037844387076, 1.000000000000000000, 0.8660254037844387076, 1.000000000000000000, 0.8660254037844387076, 1.000000000000000000, 0.8660254037844387076, 1.000000000000000000, 0.8660254037844387076, 1.000000000000000000, 0.8660254037844387076, 1.000000000000000000, 0.8660254037844387076, 1.000000000000000000, 0.8660254037844387076, 1.000000000000000000, 0.8660254037844387076, 1.000000000000000000, 0.8660254037844387076, 1.000000000000000000, 0.8660254037844387076, 1.000000000000000000, 0.8660254037844387076, 1.000000000000000000, 0.8660254037844387076, 1.000000000000000000, 0.8660254037844387076, 1.000000000000000000, 0.8660254037844387076, 1.000000000000000000, 0.8660254037844387076, 1.000000000000000000, 0.8660254037844387076, 1.000000000000000000, 0.8660254037844387076, 1.000000000000000000, 0.8660254037844387076, 1.000000000000000000, 0.8660254037844387076, 1.000000000000000000, 0.8660254037844387076, 1.000000000000000000, 0.8660254037844387076, 1.000000000000000000, 0.8660254037844387076, 1.000000000000000000, 0.8660254037844387076, 1.000000000000000000, 0.8660254037844387076, 1.000000000000000000, 0.8660254037844387076, 1.000000000000000000, 0.8660254037844387076, 1.000000000000000000, 0.8660254037844387076, 1.000000000000000000, 0.8660254037844387076, 1.000000000000000000, 0.8660254037844387076, 1.000000000000000000, 0.8660254037844387076, 1.000000000000000000, 0.8660254037844387076, 1.000000000000000000, 0.8660254037844387076, 1.000000000000000000, 0.8660254037844387076, 1.000000000000000000, 0.8660254037844387076, 1.000000000000000000, 0.8660254037844387076, 1.000000000000000000, 0.8660254037844387076, 1.000000000000000000, 0.8660254037844387076, 1.000000000000000000, 0.8660254037844387076, 1.000000000000000000, 0.8660254037844387076, 1.000000000000000000, 0.8660254037844387076, 1.000000000000000000) ) ) 
 REPRESENTATION_ITEM ( '' )  SURFACE ( )  );
#6293=EDGE_CURVE ( 'NONE', #20611, #26866, #9125, .T. ) ;
#6294=DIRECTION ( 'NONE',  ( 7.147005652999508048E-36, -5.642372883946980038E-36, -1.000000000000000000 ) ) ;
#6295=CARTESIAN_POINT ( 'NONE',  ( -4.763139720814407951, -2.750000000000016431, -131.5000000000000000 ) ) ;
#6298=ORIENTED_EDGE ( 'NONE', *, *, #29132, .F. ) ;
#6300=LINE ( 'NONE', #17866, #18532 ) ;
#6305=CARTESIAN_POINT ( 'NONE',  ( 5.412658773652739619, 3.124999999999988898, -112.3169872981077901 ) ) ;
#6312=EDGE_LOOP ( 'NONE', ( #10524, #29794, #17806, #19040 ) ) ;
#6314=CARTESIAN_POINT ( 'NONE',  ( 6.350852961086080661, -9.614813431917819062E-14, -51.37500000000002132 ) ) ;
#6316=CARTESIAN_POINT ( 'NONE',  ( -5.196152422706601826, 2.999999999999975131, -120.0386751345948255 ) ) ;
#6317=CARTESIAN_POINT ( 'NONE',  ( 3.608439182435180470, 6.249999999999982236, -65.05801270189225249 ) ) ;
#6319=CARTESIAN_POINT ( 'NONE',  ( -5.999999999999963585, -1.487416814333745711E-14, -122.9136751345948255 ) ) ;
#6323=DIRECTION ( 'NONE',  ( -7.147005652999508048E-36, 5.642372883946980038E-36, 1.000000000000000000 ) ) ;
#6325=CARTESIAN_POINT ( 'NONE',  ( -3.175426480542816066, -5.500000000000057732, -129.8750000000000284 ) ) ;
#6326=CARTESIAN_POINT ( 'NONE',  ( 5.412658773652739619, 3.124999999999988898, -147.6830127018922099 ) ) ;
#6327=LINE ( 'NONE', #3863, #27749 ) ;
#6329=CARTESIAN_POINT ( 'NONE',  ( 0.000000000000000000, 5.499999999999991118, -66.00000000000000000 ) ) ;
#6332=( BOUNDED_CURVE ( )  B_SPLINE_CURVE ( 2, ( #7411, #30151, #16817, #36, #2643, #18811, #12062, #11761, #18969 ),
 .UNSPECIFIED., .F., .T. ) 
 B_SPLINE_CURVE_WITH_KNOTS ( ( 3, 2, 2, 2, 3 ),
 ( 0.9638888888888889062, 0.9648148148148147918, 0.9666666666666666741, 0.9685185185185185563, 0.9694444444444444420 ),
 .UNSPECIFIED. ) 
 CURVE ( )  GEOMETRIC_REPRESENTATION_ITEM ( )  RATIONAL_B_SPLINE_CURVE ( ( 0.9330127018922194093, 0.9330127018922194093, 1.000000000000000000, 0.8660254037844388186, 1.000000000000000000, 0.8660254037844388186, 1.000000000000000000, 0.9330127018922194093, 0.9330127018922194093 ) ) 
 REPRESENTATION_ITEM ( '' )  );
#6340=CARTESIAN_POINT ( 'NONE',  ( -4.763139720814407951, -2.750000000000016431, -145.0000000000000284 ) ) ;
#6341=VERTEX_POINT ( 'NONE', #17996 ) ;
#6344=CARTESIAN_POINT ( 'NONE',  ( 0.000000000000000000, 5.499999999999991118, -72.00000000000001421 ) ) ;
#6346=CARTESIAN_POINT ( 'NONE',  ( 3.608439182435180470, -6.249999999999997335, -89.55801270189223828 ) ) ;
#6348=DIRECTION ( 'NONE',  ( -7.147005652999508048E-36, 5.642372883946980038E-36, 1.000000000000000000 ) ) ;
#6350=CARTESIAN_POINT ( 'NONE',  ( 0.000000000000000000, 0.000000000000000000, 0.000000000000000000 ) ) ;
#6355=CARTESIAN_POINT ( 'NONE',  ( 3.175426480543072749, 5.499999999999865885, -159.1250000000000284 ) ) ;
#6357=CARTESIAN_POINT ( 'NONE',  ( 3.464101615137852974, 5.999999999999884537, -49.33632486540521711 ) ) ;
#6359=CARTESIAN_POINT ( 'NONE',  ( -3.175426480542816066, -5.500000000000057732, -86.37500000000005684 ) ) ;
#6361=CARTESIAN_POINT ( 'NONE',  ( -4.763139720814407951, -2.750000000000016431, -70.00000000000000000 ) ) ;
#6362=CARTESIAN_POINT ( 'NONE',  ( -5.196152422706573404, -3.000000000000002665, -120.7113248654052597 ) ) ;
#6364=CARTESIAN_POINT ( 'NONE',  ( 5.196152422706629359, 3.000000000000002665, -106.4613248654052740 ) ) ;
#6365=CARTESIAN_POINT ( 'NONE',  ( 0.000000000000000000, -5.999999999999991118, -175.0386751345948255 ) ) ;
#6371=CARTESIAN_POINT ( 'NONE',  ( 0.000000000000000000, 5.999999999999977796, -75.28867513459481131 ) ) ;
#6372=VERTEX_POINT ( 'NONE', #29778 ) ;
#6374=CARTESIAN_POINT ( 'NONE',  ( 6.000000000000052403, -1.607695154586662678, -108.7306624327026157 ) ) ;
#6376=FACE_OUTER_BOUND ( 'NONE', #6578, .T. ) ;
#6380=CARTESIAN_POINT ( 'NONE',  ( -3.175426480542816510, 5.499999999999865885, -98.87499999999998579 ) ) ;
#6381=CARTESIAN_POINT ( 'NONE',  ( 6.000000000000000888, -1.859271017917181981E-14, -89.16367513459485394 ) ) ;
#6382=CARTESIAN_POINT ( 'NONE',  ( 3.608439182435180470, 6.249999999999982236, -110.0580127018922099 ) ) ;
#6384=CARTESIAN_POINT ( 'NONE',  ( -5.999999999999963585, 1.780251999655701777E-13, -93.83632486540518869 ) ) ;
#6389=CARTESIAN_POINT ( 'NONE',  ( 5.196152422706629359, 3.000000000000002665, -153.5386751345948539 ) ) ;
#6391=EDGE_CURVE ( 'NONE', #11657, #22729, #24983, .T. ) ;
#6392=CARTESIAN_POINT ( 'NONE',  ( 5.196152422706629359, -2.999999999999988898, -61.71132486540520290 ) ) ;
#6393=CARTESIAN_POINT ( 'NONE',  ( -4.763139720814407951, 2.749999999999946709, -166.2500000000000000 ) ) ;
#6395=CARTESIAN_POINT ( 'NONE',  ( -5.196152422706573404, -3.000000000000002665, -158.2113248654052313 ) ) ;
#6396=CARTESIAN_POINT ( 'NONE',  ( -3.175426480542816066, -5.500000000000057732, -107.3750000000000284 ) ) ;
#6398=LINE ( 'NONE', #20548, #22621 ) ;
#6399=CARTESIAN_POINT ( 'NONE',  ( -6.350852961085760029, -1.281975124255709124E-13, -95.62500000000004263 ) ) ;
#6400=CARTESIAN_POINT ( 'NONE',  ( 0.000000000000000000, -5.999999999999991118, -112.0386751345948682 ) ) ;
#6401=CARTESIAN_POINT ( 'NONE',  ( -5.196152422706601826, 2.999999999999975131, -162.0386751345948539 ) ) ;
#6402=CARTESIAN_POINT ( 'NONE',  ( 6.000000000000000888, 1.743066579297358182E-13, -81.66367513459481131 ) ) ;
#6403=VERTEX_POINT ( 'NONE', #19919 ) ;
#6409=CARTESIAN_POINT ( 'NONE',  ( 3.608439182435180470, -6.249999999999997335, -91.69198729810777593 ) ) ;
#6411=VERTEX_POINT ( 'NONE', #17952 ) ;
#6412=CARTESIAN_POINT ( 'NONE',  ( -4.874391507318773797, 9.861790235658084214, -28.50395189876372370 ) ) ;
#6413=( BOUNDED_CURVE ( )  B_SPLINE_CURVE ( 2, ( #10361, #14970, #10060, #24023, #16700, #19719, #26169, #28761, #819 ),
 .UNSPECIFIED., .F., .T. ) 
 B_SPLINE_CURVE_WITH_KNOTS ( ( 3, 2, 2, 2, 3 ),
 ( 0.5972222222222222099, 0.5981481481481480955, 0.5999999999999999778, 0.6018518518518518601, 0.6027777777777777457 ),
 .UNSPECIFIED. ) 
 CURVE ( )  GEOMETRIC_REPRESENTATION_ITEM ( )  RATIONAL_B_SPLINE_CURVE ( ( 0.9330127018922194093, 0.9330127018922194093, 1.000000000000000000, 0.8660254037844388186, 1.000000000000000000, 0.8660254037844388186, 1.000000000000000000, 0.9330127018922194093, 0.9330127018922194093 ) ) 
 REPRESENTATION_ITEM ( '' )  );
#6414=VECTOR ( 'NONE', #20939, 1000.000000000000000 ) ;
#6415=EDGE_LOOP ( 'NONE', ( #22650, #26990, #7636, #10846 ) ) ;
#6416=ORIENTED_EDGE ( 'NONE', *, *, #23, .T. ) ;
#6418=ADVANCED_FACE ( 'NONE', ( #8865 ), #26961, .T. ) ;
#6419=CARTESIAN_POINT ( 'NONE',  ( -4.763139720814407951, 2.749999999999946709, -118.2500000000000284 ) ) ;
#6420=CARTESIAN_POINT ( 'NONE',  ( 2.775557561562891351E-14, 6.250000000000033751, -138.4330127018922383 ) ) ;
#6422=CARTESIAN_POINT ( 'NONE',  ( -5.999999999999962697, 3.323446944526963891E-14, -160.4136751345948255 ) ) ;
#6423=CARTESIAN_POINT ( 'NONE',  ( -3.608439182435052128, -6.250000000000110134, -126.4419872981078186 ) ) ;
#6424=CARTESIAN_POINT ( 'NONE',  ( 5.412658773652739619, 3.124999999999988898, -176.8169872981077901 ) ) ;
#6435=EDGE_CURVE ( 'NONE', #17334, #8787, #6236, .T. ) ;
#6436=AXIS2_PLACEMENT_3D ( 'NONE', #26208, #122, #5161 ) ;
#6439=CARTESIAN_POINT ( 'NONE',  ( 3.608439182435180470, -6.249999999999997335, -75.19198729810783277 ) ) ;
#6440=VECTOR ( 'NONE', #19267, 1000.000000000000000 ) ;
#6441=CARTESIAN_POINT ( 'NONE',  ( 7.216878364870455975, -6.409875621278545621E-14, -61.44198729810783277 ) ) ;
#6442=CARTESIAN_POINT ( 'NONE',  ( -5.999999999999963585, 8.134310703387671600E-14, -121.4136751345948255 ) ) ;
#6443=CARTESIAN_POINT ( 'NONE',  ( 4.763139720814407951, -2.749999999999988454, -53.00000000000004974 ) ) ;
#6446=CARTESIAN_POINT ( 'NONE',  ( -2.775557561562891351E-14, -5.500000000000115463, -119.2500000000000284 ) ) ;
#6447=CARTESIAN_POINT ( 'NONE',  ( -5.999999999999971578, 1.607695154586715303, -137.9806624327025872 ) ) ;
#6448=VECTOR ( 'NONE', #30258, 1000.000000000000000 ) ;
#6449=ORIENTED_EDGE ( 'NONE', *, *, #6535, .T. ) ;
#6450=CARTESIAN_POINT ( 'NONE',  ( 6.000000000000000888, -1.607695154586752384, -118.6533121635130357 ) ) ;
#6455=ORIENTED_EDGE ( 'NONE', *, *, #14788, .T. ) ;
#6460=CARTESIAN_POINT ( 'NONE',  ( 3.608439182435180470, -6.249999999999997335, -115.6919872981078328 ) ) ;
#6463=ORIENTED_EDGE ( 'NONE', *, *, #5351, .T. ) ;
#6467=ADVANCED_FACE ( 'NONE', ( #10730 ), #24509, .T. ) ;
#6468=EDGE_LOOP ( 'NONE', ( #5204, #13832, #12773, #3691 ) ) ;
#6469=CARTESIAN_POINT ( 'NONE',  ( -7.216878364870328078, 0.000000000000000000, -144.6919872981078470 ) ) ;
#6471=AXIS2_PLACEMENT_3D ( 'NONE', #1136, #18077, #8364 ) ;
#6479=CARTESIAN_POINT ( 'NONE',  ( 2.775557561562891351E-14, -6.250000000000061284, -65.68301270189225249 ) ) ;
#6480=EDGE_CURVE ( 'NONE', #15355, #17525, #1781, .T. ) ;
#6483=CARTESIAN_POINT ( 'NONE',  ( -21.99999999999998934, -10.99999999999992362, -14.99152654425661879 ) ) ;
#6484=CARTESIAN_POINT ( 'NONE',  ( 6.000000000000000888, 5.577813053751546416E-15, -165.6636751345948255 ) ) ;
#6486=CARTESIAN_POINT ( 'NONE',  ( 5.196152422706629359, -2.999999999999988898, -66.78867513459485394 ) ) ;
#6487=CARTESIAN_POINT ( 'NONE',  ( 3.175426480543072749, 5.499999999999865885, -121.6250000000000426 ) ) ;
#6488=CARTESIAN_POINT ( 'NONE',  ( 3.608439182435180470, 6.249999999999982236, -146.0580127018922667 ) ) ;
#6491=CARTESIAN_POINT ( 'NONE',  ( 3.175426480543072749, 5.499999999999865885, -55.62500000000004263 ) ) ;
#6492=CARTESIAN_POINT ( 'NONE',  ( -5.196152422706573404, -3.000000000000002665, -154.2886751345948255 ) ) ;
#6493=CARTESIAN_POINT ( 'NONE',  ( -6.000000000000007105, -1.607695154586655129, -77.26933756729744118 ) ) ;
#6495=ORIENTED_EDGE ( 'NONE', *, *, #7345, .T. ) ;
#6502=ORIENTED_EDGE ( 'NONE', *, *, #17253, .T. ) ;
#6504=CARTESIAN_POINT ( 'NONE',  ( 0.000000000000000000, 5.499999999999991118, -139.5000000000000000 ) ) ;
#6507=CARTESIAN_POINT ( 'NONE',  ( 0.000000000000000000, 5.499999999999991118, -73.50000000000001421 ) ) ;
#6509=EDGE_CURVE ( 'NONE', #17900, #9152, #11309, .T. ) ;
#6510=( BOUNDED_CURVE ( )  B_SPLINE_CURVE ( 2, ( #13870, #16021, #11242, #28081, #30247, #7056, #16174, #6901, #25319 ),
 .UNSPECIFIED., .F., .T. ) 
 B_SPLINE_CURVE_WITH_KNOTS ( ( 3, 2, 2, 2, 3 ),
 ( 0.4805555555555555136, 0.4814814814814815103, 0.4833333333333332815, 0.4851851851851851638, 0.4861111111111111605 ),
 .UNSPECIFIED. ) 
 CURVE ( )  GEOMETRIC_REPRESENTATION_ITEM ( )  RATIONAL_B_SPLINE_CURVE ( ( 0.9330127018922194093, 0.9330127018922154125, 1.000000000000000000, 0.8660254037844388186, 1.000000000000000000, 0.8660254037844388186, 1.000000000000000000, 0.9330127018922154125, 0.9330127018922194093 ) ) 
 REPRESENTATION_ITEM ( '' )  );
#6511=CARTESIAN_POINT ( 'NONE',  ( -5.960408494996731754, -9.245657484109301549, -25.79492440527506858 ) ) ;
#6512=CARTESIAN_POINT ( 'NONE',  ( 3.464101615137852974, 5.999999999999884537, -150.4136751345947971 ) ) ;
#6513=FACE_OUTER_BOUND ( 'NONE', #28888, .T. ) ;
#6515=( BOUNDED_CURVE ( )  B_SPLINE_CURVE ( 2, ( #1933, #11807, #4540, #21144, #13965, #15808, #11340, #11655, #6694 ),
 .UNSPECIFIED., .F., .F. ) 
 B_SPLINE_CURVE_WITH_KNOTS ( ( 3, 2, 2, 2, 3 ),
 ( 0.9861111111111111605, 0.9870370370370370461, 0.9888888888888889284, 0.9907407407407406996, 0.9910511276943060333 ),
 .UNSPECIFIED. ) 
 CURVE ( )  GEOMETRIC_REPRESENTATION_ITEM ( )  RATIONAL_B_SPLINE_CURVE ( ( 0.9330127018922194093, 0.9330127018922234061, 1.000000000000000000, 0.8660254037844388186, 1.000000000000000000, 0.8660254037844388186, 1.000000000000000000, 0.9775446579417738091, 0.9626167487132855083 ) ) 
 REPRESENTATION_ITEM ( '' )  );
#6516=CARTESIAN_POINT ( 'NONE',  ( -3.175426480542816066, 5.499999999999865885, -151.3749999999999716 ) ) ;
#6518=DIRECTION ( 'NONE',  ( 3.330669073875465184E-16, -1.000000000000000000, -7.523163845262629360E-36 ) ) ;
#6519=CARTESIAN_POINT ( 'NONE',  ( -3.175426480542816066, -5.500000000000057732, -84.87500000000004263 ) ) ;
#6521=CARTESIAN_POINT ( 'NONE',  ( -6.350852961085760029, -1.281975124255709124E-13, -76.12500000000000000 ) ) ;
#6525=CARTESIAN_POINT ( 'NONE',  ( 5.196152422706629359, -2.999999999999988898, -71.28867513459479710 ) ) ;
#6532=ORIENTED_EDGE ( 'NONE', *, *, #16682, .F. ) ;
#6535=EDGE_CURVE ( 'NONE', #8715, #7154, #12303, .T. ) ;
#6536=CARTESIAN_POINT ( 'NONE',  ( 0.000000000000000000, 0.000000000000000000, 0.000000000000000000 ) ) ;
#6541=CARTESIAN_POINT ( 'NONE',  ( -6.350852961085760029, -1.281975124255709124E-13, -95.62500000000004263 ) ) ;
#6542=CARTESIAN_POINT ( 'NONE',  ( -5.999999999999963585, 1.780251999655701777E-13, -89.91367513459485394 ) ) ;
#6543=CARTESIAN_POINT ( 'NONE',  ( -3.608439182435115633, 6.249999999999965361, -109.8080127018922667 ) ) ;
#6547=CARTESIAN_POINT ( 'NONE',  ( -5.196152422706573404, -3.000000000000002665, -143.7886751345948255 ) ) ;
#6548=CARTESIAN_POINT ( 'NONE',  ( -4.763139720814407951, -2.750000000000016431, -164.5000000000000284 ) ) ;
#6549=CARTESIAN_POINT ( 'NONE',  ( 5.412658773652739619, 3.124999999999988898, -47.18301270189223828 ) ) ;
#6551=CARTESIAN_POINT ( 'NONE',  ( 5.999999999999999112, 2.951592740943527306E-14, -160.5863248654052029 ) ) ;
#6552=CARTESIAN_POINT ( 'NONE',  ( 0.000000000000000000, 0.000000000000000000, 0.000000000000000000 ) ) ;
#6554=CARTESIAN_POINT ( 'NONE',  ( -6.350852961085760029, -1.281975124255709124E-13, -160.1250000000000284 ) ) ;
#6557=( BOUNDED_CURVE ( )  B_SPLINE_CURVE ( 2, ( #9405, #18794, #25978, #11439, #23395, #2033, #11592, #28118, #4920 ),
 .UNSPECIFIED., .F., .F. ) 
 B_SPLINE_CURVE_WITH_KNOTS ( ( 3, 2, 2, 2, 3 ),
 ( 0.8472222222222222099, 0.8481481481481480955, 0.8499999999999999778, 0.8518518518518518601, 0.8527777777777778567 ),
 .UNSPECIFIED. ) 
 CURVE ( )  GEOMETRIC_REPRESENTATION_ITEM ( )  RATIONAL_B_SPLINE_CURVE ( ( 0.9330127018922194093, 0.9330127018922194093, 1.000000000000000000, 0.8660254037844388186, 1.000000000000000000, 0.8660254037844388186, 1.000000000000000000, 0.9330127018922154125, 0.9330127018922194093 ) ) 
 REPRESENTATION_ITEM ( '' )  );
#6558=CARTESIAN_POINT ( 'NONE',  ( -6.350852961085760029, -1.281975124255709124E-13, -112.1249999999999858 ) ) ;
#6559=LINE ( 'NONE', #7018, #26043 ) ;
#6560=CARTESIAN_POINT ( 'NONE',  ( -2.775557561562891351E-14, -5.500000000000115463, -96.75000000000000000 ) ) ;
#6565=FACE_OUTER_BOUND ( 'NONE', #17340, .T. ) ;
#6568=VERTEX_POINT ( 'NONE', #21561 ) ;
#6571=CARTESIAN_POINT ( 'NONE',  ( 5.412658773652739619, 3.124999999999988898, -91.31698729810783277 ) ) ;
#6573=CARTESIAN_POINT ( 'NONE',  ( -3.679869817085036576, 10.37177793260014802, -29.75506555745397108 ) ) ;
#6575=ORIENTED_EDGE ( 'NONE', *, *, #11716, .F. ) ;
#6578=EDGE_LOOP ( 'NONE', ( #9774, #18859, #6998, #723 ) ) ;
#6579=CARTESIAN_POINT ( 'NONE',  ( 3.175426480543072749, 5.499999999999865885, -124.6250000000000426 ) ) ;
#6581=CARTESIAN_POINT ( 'NONE',  ( -5.412658773652684552, -3.125000000000099920, -133.4330127018922383 ) ) ;
#6584=CARTESIAN_POINT ( 'NONE',  ( -7.216878364870328078, 0.000000000000000000, -125.1919872981078186 ) ) ;
#6585=CARTESIAN_POINT ( 'NONE',  ( -5.412658773652739619, 3.124999999999975131, -179.3169872981078470 ) ) ;
#6588=ORIENTED_EDGE ( 'NONE', *, *, #6391, .F. ) ;
#6589=CARTESIAN_POINT ( 'NONE',  ( -5.196152422706601826, 2.999999999999975131, -163.5386751345947971 ) ) ;
#6590=CARTESIAN_POINT ( 'NONE',  ( 3.606777763902872191, 4.527305315990890477, -180.0000000000001990 ) ) ;
#6594=CARTESIAN_POINT ( 'NONE',  ( 7.216878364870455975, -6.409875621278545621E-14, -71.94198729810780435 ) ) ;
#6595=CARTESIAN_POINT ( 'NONE',  ( 3.608439182435180470, 6.249999999999982236, -58.19198729810781856 ) ) ;
#6596=CARTESIAN_POINT ( 'NONE',  ( -2.000000000000003109, 3.559516622919867392E-16, 2.520259888162984417E-35 ) ) ;
#6597=CARTESIAN_POINT ( 'NONE',  ( -5.412658773652739619, 3.124999999999975131, -181.6830127018922383 ) ) ;
#6599=CYLINDRICAL_SURFACE ( 'NONE', #7837, 6.000000000000001776 ) ;
#6601=CARTESIAN_POINT ( 'NONE',  ( 6.000000000000000888, 1.743066579297358182E-13, -69.08632486540523132 ) ) ;
#6602=CARTESIAN_POINT ( 'NONE',  ( 0.000000000000000000, 5.499999999999991118, -123.0000000000000000 ) ) ;
#6603=CARTESIAN_POINT ( 'NONE',  ( 0.000000000000000000, 5.499999999999991118, -157.5000000000000284 ) ) ;
#6604=CARTESIAN_POINT ( 'NONE',  ( -3.464101615137725076, 5.999999999999979572, -50.58632486540523132 ) ) ;
#6605=CARTESIAN_POINT ( 'NONE',  ( -5.999999999999963585, -1.487416814333745711E-14, -153.8363248654052313 ) ) ;
#6606=ORIENTED_EDGE ( 'NONE', *, *, #23319, .F. ) ;
#6614=CARTESIAN_POINT ( 'NONE',  ( -5.999999999999963585, 8.134310703387671600E-14, -129.8363248654052313 ) ) ;
#6616=CARTESIAN_POINT ( 'NONE',  ( 2.775557561562891351E-14, -6.250000000000061284, -115.8169872981078470 ) ) ;
#6617=CARTESIAN_POINT ( 'NONE',  ( -5.999999999999959144, -1.607695154586739283, -176.8466878364870922 ) ) ;
#6620=ORIENTED_EDGE ( 'NONE', *, *, #14087, .F. ) ;
#6621=CARTESIAN_POINT ( 'NONE',  ( 0.000000000000000000, 0.000000000000000000, 0.000000000000000000 ) ) ;
#6625=CARTESIAN_POINT ( 'NONE',  ( 7.216878364870455975, -6.409875621278545621E-14, -148.4419872981078470 ) ) ;
#6630=DIRECTION ( 'NONE',  ( 1.000000000000000000, -5.551115123125773458E-17, -1.260129944081490338E-35 ) ) ;
#6631=CARTESIAN_POINT ( 'NONE',  ( 2.775557561562891351E-14, -6.250000000000061284, -68.68301270189225249 ) ) ;
#6635=DIRECTION ( 'NONE',  ( -7.147005652999508048E-36, 5.642372883946980038E-36, 1.000000000000000000 ) ) ;
#6637=AXIS2_PLACEMENT_3D ( 'NONE', #6223, #15641, #22367 ) ;
#6639=CARTESIAN_POINT ( 'NONE',  ( -5.196152422706601826, 2.999999999999975131, -114.9613248654052171 ) ) ;
#6642=CARTESIAN_POINT ( 'NONE',  ( 4.763139720814407951, -2.749999999999988454, -125.0000000000000000 ) ) ;
#6643=FACE_OUTER_BOUND ( 'NONE', #9263, .T. ) ;
#6644=CARTESIAN_POINT ( 'NONE',  ( -7.216878364870328078, 0.000000000000000000, -144.0580127018922383 ) ) ;
#6646=ORIENTED_EDGE ( 'NONE', *, *, #6252, .F. ) ;
#6647=EDGE_CURVE ( 'NONE', #2399, #16363, #12481, .T. ) ;
#6648=CARTESIAN_POINT ( 'NONE',  ( -4.763139720814407951, -2.750000000000016431, -52.00000000000004263 ) ) ;
#6649=DIRECTION ( 'NONE',  ( -7.147005652999508048E-36, 5.642372883946980038E-36, 1.000000000000000000 ) ) ;
#6650=DIRECTION ( 'NONE',  ( -7.147005652999508048E-36, 5.642372883946980038E-36, 1.000000000000000000 ) ) ;
#6658=EDGE_CURVE ( 'NONE', #750, #14484, #15440, .T. ) ;
#6662=( BOUNDED_CURVE ( )  B_SPLINE_CURVE ( 2, ( #771, #21380, #7388, #2913, #316, #5361, #14769, #9705, #21970 ),
 .UNSPECIFIED., .F., .F. ) 
 B_SPLINE_CURVE_WITH_KNOTS ( ( 3, 2, 2, 2, 3 ),
 ( 0.4805555555555555136, 0.4814814814814814548, 0.4833333333333333370, 0.4851851851851851638, 0.4861111111111111049 ),
 .UNSPECIFIED. ) 
 CURVE ( )  GEOMETRIC_REPRESENTATION_ITEM ( )  RATIONAL_B_SPLINE_CURVE ( ( 0.9330127018922194093, 0.9330127018922174109, 1.000000000000000000, 0.8660254037844388186, 1.000000000000000000, 0.8660254037844388186, 1.000000000000000000, 0.9330127018922194093, 0.9330127018922194093 ) ) 
 REPRESENTATION_ITEM ( '' )  );
#6663=CARTESIAN_POINT ( 'NONE',  ( -4.763139720814407951, -2.750000000000016431, -140.5000000000000000 ) ) ;
#6666=CARTESIAN_POINT ( 'NONE',  ( -3.175426480542816510, -5.500000000000057732, -65.37500000000001421 ) ) ;
#6669=CARTESIAN_POINT ( 'NONE',  ( 0.000000000000000000, 5.999999999999977796, -139.7886751345947971 ) ) ;
#6670=DIRECTION ( 'NONE',  ( -7.147005652999508048E-36, 5.642372883946980038E-36, 1.000000000000000000 ) ) ;
#6672=CARTESIAN_POINT ( 'NONE',  ( -4.763139720814407951, 2.749999999999946709, -151.2500000000000000 ) ) ;
#6674=CARTESIAN_POINT ( 'NONE',  ( 5.412658773652712085, -3.125000000000086153, -159.9330127018922383 ) ) ;
#6678=CARTESIAN_POINT ( 'NONE',  ( 0.000000000000000000, 5.499999999999991118, -76.50000000000001421 ) ) ;
#6680=CARTESIAN_POINT ( 'NONE',  ( -4.763139720814407951, -2.750000000000016431, -74.50000000000001421 ) ) ;
#6681=DIRECTION ( 'NONE',  ( 1.000000000000000000, -5.551115123125773458E-17, -1.260129944081490338E-35 ) ) ;
#6684=CARTESIAN_POINT ( 'NONE',  ( 5.196152422706629359, -2.999999999999988898, -75.78867513459486815 ) ) ;
#6685=CARTESIAN_POINT ( 'NONE',  ( -5.999999999999963585, 8.134310703387671600E-14, -116.9136751345948539 ) ) ;
#6687=CARTESIAN_POINT ( 'NONE',  ( -3.464101615137725076, 5.999999999999979572, -55.08632486540518158 ) ) ;
#6689=EDGE_CURVE ( 'NONE', #24216, #14326, #14458, .T. ) ;
#6694=CARTESIAN_POINT ( 'NONE',  ( 5.630955349231442142, 2.071796769705314123, -180.0000000000000568 ) ) ;
#6695=ORIENTED_EDGE ( 'NONE', *, *, #16059, .T. ) ;
#6696=EDGE_LOOP ( 'NONE', ( #10839, #11917, #24146, #24268 ) ) ;
#6697=( BOUNDED_CURVE ( )  B_SPLINE_CURVE ( 2, ( #2812, #5709, #28754, #29204, #19570, #7723, #5861, #5559, #12237 ),
 .UNSPECIFIED., .F., .T. ) 
 B_SPLINE_CURVE_WITH_KNOTS ( ( 3, 2, 2, 2, 3 ),
 ( 0.4083333333333333259, 0.4092592592592592116, 0.4111111111111110938, 0.4129629629629629761, 0.4138888888888888618 ),
 .UNSPECIFIED. ) 
 CURVE ( )  GEOMETRIC_REPRESENTATION_ITEM ( )  RATIONAL_B_SPLINE_CURVE ( ( 0.9330127018922194093, 0.9330127018922194093, 1.000000000000000000, 0.8660254037844388186, 1.000000000000000000, 0.8660254037844388186, 1.000000000000000000, 0.9330127018922234061, 0.9330127018922194093 ) ) 
 REPRESENTATION_ITEM ( '' )  );
#6698=ORIENTED_EDGE ( 'NONE', *, *, #23133, .T. ) ;
#6699=CARTESIAN_POINT ( 'NONE',  ( -4.763139720814407951, -2.750000000000016431, -92.50000000000002842 ) ) ;
#6700=CARTESIAN_POINT ( 'NONE',  ( 3.608439182435180470, 6.249999999999982236, -108.5580127018921957 ) ) ;
#6705=CARTESIAN_POINT ( 'NONE',  ( 6.350852961086080661, -9.614813431917819062E-14, -162.3750000000000284 ) ) ;
#6706=CARTESIAN_POINT ( 'NONE',  ( 0.000000000000000000, -5.999999999999991118, -106.0386751345948682 ) ) ;
#6707=ORIENTED_EDGE ( 'NONE', *, *, #19452, .T. ) ;
#6708=CARTESIAN_POINT ( 'NONE',  ( 6.000000000000000888, -1.607695154586752384, -67.65331216351302146 ) ) ;
#6710=CARTESIAN_POINT ( 'NONE',  ( 3.175426480543072749, -5.500000000000105693, -173.1250000000000284 ) ) ;
#6711=FACE_OUTER_BOUND ( 'NONE', #5881, .T. ) ;
#6712=CARTESIAN_POINT ( 'NONE',  ( 4.763139720814407951, -2.749999999999988454, -161.0000000000000284 ) ) ;
#6714=EDGE_CURVE ( 'NONE', #18709, #13261, #6964, .T. ) ;
#6715=FACE_OUTER_BOUND ( 'NONE', #5622, .T. ) ;
#6718=CARTESIAN_POINT ( 'NONE',  ( 4.763139720814407951, -2.749999999999988454, -93.50000000000002842 ) ) ;
#6719=PRODUCT_DEFINITION ( 'UNKNOWN', '', #3098, #6790 ) ;
#6722=EDGE_LOOP ( 'NONE', ( #11304, #23303, #78, #27062 ) ) ;
#6726=ORIENTED_EDGE ( 'NONE', *, *, #2712, .F. ) ;
#6728=CARTESIAN_POINT ( 'NONE',  ( 3.608439182435180470, 6.249999999999982236, -86.69198729810781856 ) ) ;
#6729=VECTOR ( 'NONE', #23843, 1000.000000000000000 ) ;
#6733=CARTESIAN_POINT ( 'NONE',  ( -4.763139720814407951, -2.750000000000016431, -122.5000000000000568 ) ) ;
#6735=CARTESIAN_POINT ( 'NONE',  ( -5.412658773652684552, -3.125000000000099920, -134.9330127018922383 ) ) ;
#6736=EDGE_LOOP ( 'NONE', ( #5171, #6804, #18272, #936 ) ) ;
#6738=CARTESIAN_POINT ( 'NONE',  ( 3.608439182435180470, -6.249999999999997335, -165.1919872981078186 ) ) ;
#6739=CARTESIAN_POINT ( 'NONE',  ( 2.775557561562891351E-14, -6.250000000000061284, -180.3169872981078470 ) ) ;
#6741=( BOUNDED_CURVE ( )  B_SPLINE_CURVE ( 2, ( #23541, #25356, #2185, #2341, #6933, #18793, #4326, #7088, #2480 ),
 .UNSPECIFIED., .F., .F. ) 
 B_SPLINE_CURVE_WITH_KNOTS ( ( 3, 2, 2, 2, 3 ),
 ( 0.5805555555555554914, 0.5814814814814814881, 0.5833333333333332593, 0.5851851851851852526, 0.5861111111111111382 ),
 .UNSPECIFIED. ) 
 CURVE ( )  GEOMETRIC_REPRESENTATION_ITEM ( )  RATIONAL_B_SPLINE_CURVE ( ( 0.9330127018922194093, 0.9330127018922154125, 1.000000000000000000, 0.8660254037844388186, 1.000000000000000000, 0.8660254037844388186, 1.000000000000000000, 0.9330127018922194093, 0.9330127018922194093 ) ) 
 REPRESENTATION_ITEM ( '' )  );
#6743=CARTESIAN_POINT ( 'NONE',  ( 6.000000000000000888, 1.607695154586715303, -147.5966878364871206 ) ) ;
#6744=ORIENTED_EDGE ( 'NONE', *, *, #24589, .F. ) ;
#6746=CARTESIAN_POINT ( 'NONE',  ( -3.464101615137725076, 5.999999999999979572, -54.16367513459480421 ) ) ;
#6747=CARTESIAN_POINT ( 'NONE',  ( 3.847734726291792473, 4.353436196503639444, -180.0000000000000000 ) ) ;
#6748=CARTESIAN_POINT ( 'NONE',  ( 3.464101615137852974, 5.999999999999884537, -136.9136751345947971 ) ) ;
#6750=CARTESIAN_POINT ( 'NONE',  ( 7.216878364870455975, -6.409875621278545621E-14, -73.44198729810783277 ) ) ;
#6751=CARTESIAN_POINT ( 'NONE',  ( 3.608439182435180470, 6.249999999999982236, -62.69198729810783277 ) ) ;
#6752=CARTESIAN_POINT ( 'NONE',  ( 4.763139720814407951, 2.750000000000002665, -51.25000000000001421 ) ) ;
#6754=CARTESIAN_POINT ( 'NONE',  ( -3.464101615137725076, 5.999999999999979572, -159.1636751345948255 ) ) ;
#6756=CARTESIAN_POINT ( 'NONE',  ( -3.175426480542816510, -5.500000000000057732, -120.8750000000000284 ) ) ;
#6758=CARTESIAN_POINT ( 'NONE',  ( -1.285375204280330350E-15, -10.49588505988223375, 1.184433945098074864E-34 ) ) ;
#6762=DIRECTION ( 'NONE',  ( 1.000000000000000000, -5.551115123125773458E-17, -1.260129944081490338E-35 ) ) ;
#6767=CARTESIAN_POINT ( 'NONE',  ( 3.608439182435180470, -6.249999999999997335, -108.1919872981077901 ) ) ;
#6771=ORIENTED_EDGE ( 'NONE', *, *, #2557, .T. ) ;
#6772=ORIENTED_EDGE ( 'NONE', *, *, #1788, .F. ) ;
#6776=CARTESIAN_POINT ( 'NONE',  ( -7.216878364870328078, 0.000000000000000000, -143.1919872981078186 ) ) ;
#6781=CARTESIAN_POINT ( 'NONE',  ( 5.412658773652739619, 3.124999999999988898, -71.18301270189225249 ) ) ;
#6784=CARTESIAN_POINT ( 'NONE',  ( -5.999999999999963585, 9.296355089585909904E-15, -164.9136751345948255 ) ) ;
#6787=( BOUNDED_CURVE ( )  B_SPLINE_CURVE ( 2, ( #7431, #28907, #24167, #2520, #12383, #7872, #21273, #12088, #2817 ),
 .UNSPECIFIED., .F., .T. ) 
 B_SPLINE_CURVE_WITH_KNOTS ( ( 3, 2, 2, 2, 3 ),
 ( 0.7083333333333333703, 0.7092592592592592560, 0.7111111111111111382, 0.7129629629629629095, 0.7138888888888887951 ),
 .UNSPECIFIED. ) 
 CURVE ( )  GEOMETRIC_REPRESENTATION_ITEM ( )  RATIONAL_B_SPLINE_CURVE ( ( 0.9330127018922194093, 0.9330127018922234061, 1.000000000000000000, 0.8660254037844388186, 1.000000000000000000, 0.8660254037844388186, 1.000000000000000000, 0.9330127018922234061, 0.9330127018922194093 ) ) 
 REPRESENTATION_ITEM ( '' )  );
#6789=CARTESIAN_POINT ( 'NONE',  ( 3.175426480543072749, 5.499999999999865885, -126.1250000000000426 ) ) ;
#6790=PRODUCT_DEFINITION_CONTEXT ( 'detailed design', #22635, 'design' ) ;
#6793=CARTESIAN_POINT ( 'NONE',  ( -2.775557561562891351E-14, -5.500000000000115463, -51.75000000000002132 ) ) ;
#6794=CARTESIAN_POINT ( 'NONE',  ( -6.000000000000023093, 1.607695154586625819, -123.9033121635129646 ) ) ;
#6795=FACE_OUTER_BOUND ( 'NONE', #18964, .T. ) ;
#6796=ORIENTED_EDGE ( 'NONE', *, *, #16874, .T. ) ;
#6800=CARTESIAN_POINT ( 'NONE',  ( 3.608439182435180470, -6.249999999999997335, -100.6919872981078328 ) ) ;
#6801=CARTESIAN_POINT ( 'NONE',  ( 6.000000000000000888, -3.330669073875464691E-16, -7.560779664488942560E-35 ) ) ;
#6804=ORIENTED_EDGE ( 'NONE', *, *, #10167, .T. ) ;
#6806=CARTESIAN_POINT ( 'NONE',  ( -4.763139720814407951, 2.749999999999946709, -137.7500000000000284 ) ) ;
#6810=CARTESIAN_POINT ( 'NONE',  ( -4.763139720814407951, 2.749999999999946709, -64.25000000000002842 ) ) ;
#6811=CARTESIAN_POINT ( 'NONE',  ( 5.999999999999999112, 2.951592740943527306E-14, -164.1636751345948824 ) ) ;
#6812=VECTOR ( 'NONE', #14470, 1000.000000000000000 ) ;
#6813=CARTESIAN_POINT ( 'NONE',  ( -5.196152422706601826, 2.999999999999975131, -139.5386751345948255 ) ) ;
#6814=CARTESIAN_POINT ( 'NONE',  ( 0.000000000000000000, 0.000000000000000000, 0.000000000000000000 ) ) ;
#6818=CARTESIAN_POINT ( 'NONE',  ( 3.175426480543072749, 5.499999999999865885, -145.6250000000000000 ) ) ;
#6820=CARTESIAN_POINT ( 'NONE',  ( -4.763139720814407951, -2.750000000000016431, -137.5000000000000000 ) ) ;
#6821=CARTESIAN_POINT ( 'NONE',  ( -5.412658773652684552, -3.125000000000099920, -161.9330127018922667 ) ) ;
#6822=CARTESIAN_POINT ( 'NONE',  ( 0.000000000000000000, 0.000000000000000000, 0.000000000000000000 ) ) ;
#6824=CARTESIAN_POINT ( 'NONE',  ( 0.000000000000000000, 5.499999999999991118, -81.00000000000001421 ) ) ;
#6825=CARTESIAN_POINT ( 'NONE',  ( 4.763139720814407951, 2.750000000000002665, -75.25000000000004263 ) ) ;
#6826=CARTESIAN_POINT ( 'NONE',  ( 3.464101615137757051, -5.999999999999979572, -156.3363248654052313 ) ) ;
#6831=CARTESIAN_POINT ( 'NONE',  ( 6.000000000000000888, 7.762456499804234384E-14, -134.1636751345948539 ) ) ;
#6835=CARTESIAN_POINT ( 'NONE',  ( -5.196152422706573404, -3.000000000000002665, -147.7113248654052313 ) ) ;
#6837=CARTESIAN_POINT ( 'NONE',  ( 0.000000000000000000, 5.999999999999977796, -169.7886751345948255 ) ) ;
#6839=VECTOR ( 'NONE', #21511, 1000.000000000000000 ) ;
#6842=CARTESIAN_POINT ( 'NONE',  ( -5.999999999999963585, 1.780251999655701777E-13, -85.41367513459483973 ) ) ;
#6844=VERTEX_POINT ( 'NONE', #8944 ) ;
#6847=CARTESIAN_POINT ( 'NONE',  ( 4.763139720814407951, 2.750000000000002665, -91.75000000000000000 ) ) ;
#6848=CARTESIAN_POINT ( 'NONE',  ( -3.608439182435052128, -6.250000000000110134, -106.3080127018922667 ) ) ;
#6849=ORIENTED_EDGE ( 'NONE', *, *, #2322, .F. ) ;
#6850=CARTESIAN_POINT ( 'NONE',  ( 6.000000000000000888, -1.859271017917181981E-14, -68.16367513459481131 ) ) ;
#6852=CARTESIAN_POINT ( 'NONE',  ( 2.775557561562891351E-14, 6.250000000000033751, -48.43301270189226670 ) ) ;
#6858=CARTESIAN_POINT ( 'NONE',  ( -2.775557561562891351E-14, -5.500000000000115463, -168.7500000000000000 ) ) ;
#6859=CARTESIAN_POINT ( 'NONE',  ( -5.999999999999963585, -1.487416814333745711E-14, -80.91367513459482552 ) ) ;
#6860=CARTESIAN_POINT ( 'NONE',  ( -3.175426480542816510, -5.500000000000057732, -161.3750000000000284 ) ) ;
#6861=AXIS2_PLACEMENT_3D ( 'NONE', #22704, #4093, #13513 ) ;
#6865=CARTESIAN_POINT ( 'NONE',  ( 0.000000000000000000, 5.999999999999977796, -87.28867513459481131 ) ) ;
#6866=CARTESIAN_POINT ( 'NONE',  ( -4.763139720814407951, -2.750000000000016431, -98.50000000000002842 ) ) ;
#6869=CARTESIAN_POINT ( 'NONE',  ( -5.999999999999963585, -1.487416814333745711E-14, -143.3363248654052029 ) ) ;
#6870=ORIENTED_EDGE ( 'NONE', *, *, #9918, .F. ) ;
#6875=CARTESIAN_POINT ( 'NONE',  ( -5.999999999999963585, 1.780251999655701777E-13, -86.33632486540524553 ) ) ;
#6878=EDGE_LOOP ( 'NONE', ( #29106, #24437, #11302, #25001 ) ) ;
#6885=CARTESIAN_POINT ( 'NONE',  ( -4.763139720814407951, 2.749999999999946709, -115.2500000000000142 ) ) ;
#6888=CARTESIAN_POINT ( 'NONE',  ( 2.775557561562891351E-14, 6.250000000000033751, -132.4330127018922383 ) ) ;
#6889=ORIENTED_EDGE ( 'NONE', *, *, #25003, .F. ) ;
#6891=CARTESIAN_POINT ( 'NONE',  ( 2.775557561562891351E-14, 6.250000000000033751, -172.0669872981078186 ) ) ;
#6892=CARTESIAN_POINT ( 'NONE',  ( -3.608439182435115633, 6.249999999999965361, -180.9419872981078186 ) ) ;
#6895=DIRECTION ( 'NONE',  ( -7.147005652999508048E-36, 5.642372883946980038E-36, 1.000000000000000000 ) ) ;
#6898=CARTESIAN_POINT ( 'NONE',  ( 3.608439182435180470, 6.249999999999982236, -77.69198729810784698 ) ) ;
#6899=CARTESIAN_POINT ( 'NONE',  ( -3.608439182435115633, 6.249999999999965361, -60.94198729810783277 ) ) ;
#6900=CARTESIAN_POINT ( 'NONE',  ( 3.608439182435180470, -6.249999999999997335, -181.0580127018922099 ) ) ;
#6901=CARTESIAN_POINT ( 'NONE',  ( -6.000000000000007105, -1.607695154586655129, -111.7693375672974270 ) ) ;
#6902=FACE_OUTER_BOUND ( 'NONE', #28362, .T. ) ;
#6905=CARTESIAN_POINT ( 'NONE',  ( -3.175426480542816510, 5.499999999999865885, -119.8750000000000284 ) ) ;
#6906=CARTESIAN_POINT ( 'NONE',  ( 0.000000000000000000, 5.999999999999977796, -166.2113248654052313 ) ) ;
#6910=CARTESIAN_POINT ( 'NONE',  ( -5.999999999999971578, 1.607695154586715303, -122.4033121635129930 ) ) ;
#6914=CARTESIAN_POINT ( 'NONE',  ( 3.608439182435180470, -6.249999999999997335, -111.1919872981078186 ) ) ;
#6924=CARTESIAN_POINT ( 'NONE',  ( -3.608439182435052128, -6.250000000000110134, -142.9419872981078470 ) ) ;
#6925=VECTOR ( 'NONE', #29911, 1000.000000000000000 ) ;
#6929=DIRECTION ( 'NONE',  ( -7.147005652999508048E-36, 5.642372883946980038E-36, 1.000000000000000000 ) ) ;
#6930=CARTESIAN_POINT ( 'NONE',  ( -5.412658773652684552, -3.125000000000099920, -61.43301270189221697 ) ) ;
#6933=CARTESIAN_POINT ( 'NONE',  ( 0.000000000000000000, -5.999999999999991118, -124.9613248654052313 ) ) ;
#6935=CARTESIAN_POINT ( 'NONE',  ( -5.999999999999919176, 1.607695154586804565, -73.48066243270262987 ) ) ;
#6939=CARTESIAN_POINT ( 'NONE',  ( 3.464101615137757051, -5.999999999999979572, -66.91367513459479710 ) ) ;
#6941=FACE_OUTER_BOUND ( 'NONE', #26754, .T. ) ;
#6946=CARTESIAN_POINT ( 'NONE',  ( 3.175426480543072749, 5.499999999999865885, -51.12500000000001421 ) ) ;
#6947=CARTESIAN_POINT ( 'NONE',  ( -5.196152422706601826, 2.999999999999975131, -78.96132486540518869 ) ) ;
#6952=CARTESIAN_POINT ( 'NONE',  ( -7.216878364870328078, 0.000000000000000000, -105.6919872981078470 ) ) ;
#6955=DIRECTION ( 'NONE',  ( -7.147005652999508048E-36, 5.642372883946980038E-36, 1.000000000000000000 ) ) ;
#6958=CARTESIAN_POINT ( 'NONE',  ( 6.350852961086080661, -9.614813431917819062E-14, -141.3750000000000568 ) ) ;
#6961=CARTESIAN_POINT ( 'NONE',  ( -3.175426480542816510, 5.499999999999865885, -64.37500000000001421 ) ) ;
#6963=CARTESIAN_POINT ( 'NONE',  ( 0.000000000000000000, -5.999999999999991118, -124.0386751345948824 ) ) ;
#6964=( BOUNDED_CURVE ( )  B_SPLINE_CURVE ( 2, ( #19556, #19700, #3092, #26442, #29189, #14805, #12519, #8150, #10187 ),
 .UNSPECIFIED., .F., .T. ) 
 B_SPLINE_CURVE_WITH_KNOTS ( ( 3, 2, 2, 2, 3 ),
 ( 0.2694444444444443754, 0.2703703703703703720, 0.2722222222222222543, 0.2740740740740740256, 0.2750000000000000222 ),
 .UNSPECIFIED. ) 
 CURVE ( )  GEOMETRIC_REPRESENTATION_ITEM ( )  RATIONAL_B_SPLINE_CURVE ( ( 0.9330127018922194093, 0.9330127018922154125, 1.000000000000000000, 0.8660254037844388186, 1.000000000000000000, 0.8660254037844388186, 1.000000000000000000, 0.9330127018922154125, 0.9330127018922194093 ) ) 
 REPRESENTATION_ITEM ( '' )  );
#6965=ORIENTED_EDGE ( 'NONE', *, *, #4426, .T. ) ;
#6968=DIRECTION ( 'NONE',  ( 1.000000000000000000, -5.551115123125773458E-17, 0.000000000000000000 ) ) ;
#6969=FACE_OUTER_BOUND ( 'NONE', #7371, .T. ) ;
#6971=CARTESIAN_POINT ( 'NONE',  ( 4.763139720814407951, -2.749999999999988454, -146.0000000000000284 ) ) ;
#6973=CARTESIAN_POINT ( 'NONE',  ( 6.350852961086080661, -9.614813431917819062E-14, -133.8750000000000284 ) ) ;
#6974=CARTESIAN_POINT ( 'NONE',  ( 2.775557561562891351E-14, -6.250000000000061284, -163.1830127018922383 ) ) ;
#6975=CARTESIAN_POINT ( 'NONE',  ( 6.000000000000052403, -1.607695154586662678, -148.6533121635129930 ) ) ;
#6976=CARTESIAN_POINT ( 'NONE',  ( 6.000000000000000888, 1.743066579297358182E-13, -90.08632486540521711 ) ) ;
#6977=AXIS2_PLACEMENT_3D ( 'NONE', #21735, #7729, #26462 ) ;
#6979=CARTESIAN_POINT ( 'NONE',  ( -2.775557561562891351E-14, -5.500000000000115463, -75.75000000000004263 ) ) ;
#6981=CARTESIAN_POINT ( 'NONE',  ( -4.763139720814407951, -2.750000000000016431, -65.50000000000000000 ) ) ;
#6983=CARTESIAN_POINT ( 'NONE',  ( 5.196152422706629359, -2.999999999999988898, -114.2113248654051887 ) ) ;
#6989=CARTESIAN_POINT ( 'NONE',  ( -3.464101615137757051, -5.999999999999979572, -98.66367513459481131 ) ) ;
#6991=CARTESIAN_POINT ( 'NONE',  ( 3.464101615137757051, -5.999999999999979572, -97.83632486540517448 ) ) ;
#6997=EDGE_LOOP ( 'NONE', ( #22027, #8571, #1181, #20265 ) ) ;
#6998=ORIENTED_EDGE ( 'NONE', *, *, #10508, .F. ) ;
#7000=ORIENTED_EDGE ( 'NONE', *, *, #19257, .F. ) ;
#7001=CARTESIAN_POINT ( 'NONE',  ( 6.350852961086080661, -9.614813431917819062E-14, -90.37500000000000000 ) ) ;
#7002=CARTESIAN_POINT ( 'NONE',  ( 7.216878364870455975, -6.409875621278545621E-14, -108.8080127018922667 ) ) ;
#7003=ORIENTED_EDGE ( 'NONE', *, *, #28612, .F. ) ;
#7004=CARTESIAN_POINT ( 'NONE',  ( 5.687368478358042267, 9.417270245429904207, -26.95189157943837444 ) ) ;
#7006=CARTESIAN_POINT ( 'NONE',  ( 2.775557561562891351E-14, -11.00000000000001066, -31.00000000000002842 ) ) ;
#7008=CARTESIAN_POINT ( 'NONE',  ( 6.000000000000000888, 1.607695154586715303, -93.59668783648702117 ) ) ;
#7009=( NAMED_UNIT ( * ) SI_UNIT ( $, .STERADIAN. ) SOLID_ANGLE_UNIT ( ) );
#7011=CARTESIAN_POINT ( 'NONE',  ( 4.763139720814407951, -2.749999999999988454, -174.5000000000000000 ) ) ;
#7013=CARTESIAN_POINT ( 'NONE',  ( 4.763139720814407951, -2.749999999999988454, -152.0000000000000284 ) ) ;
#7015=( BOUNDED_CURVE ( )  B_SPLINE_CURVE ( 2, ( #1243, #19703, #19559, #10191, #28894, #26733, #22161, #7859, #22468 ),
 .UNSPECIFIED., .F., .F. ) 
 B_SPLINE_CURVE_WITH_KNOTS ( ( 3, 2, 2, 2, 3 ),
 ( 0.3472222222222222099, 0.3481481481481481510, 0.3499999999999999778, 0.3518518518518518601, 0.3527777777777778012 ),
 .UNSPECIFIED. ) 
 CURVE ( )  GEOMETRIC_REPRESENTATION_ITEM ( )  RATIONAL_B_SPLINE_CURVE ( ( 0.9330127018922194093, 0.9330127018922194093, 1.000000000000000000, 0.8660254037844388186, 1.000000000000000000, 0.8660254037844388186, 1.000000000000000000, 0.9330127018922174109, 0.9330127018922194093 ) ) 
 REPRESENTATION_ITEM ( '' )  );
#7016=CARTESIAN_POINT ( 'NONE',  ( -4.763139720814407951, 2.749999999999946709, -101.7500000000000000 ) ) ;
#7017=DIRECTION ( 'NONE',  ( 1.000000000000000000, -5.551115123125773458E-17, -1.260129944081490338E-35 ) ) ;
#7018=CARTESIAN_POINT ( 'NONE',  ( 6.000000000000000888, -3.330669073875464691E-16, -7.560779664488942560E-35 ) ) ;
#7019=CARTESIAN_POINT ( 'NONE',  ( 4.763139720814407951, 2.750000000000002665, -90.25000000000005684 ) ) ;
#7030=CYLINDRICAL_SURFACE ( 'NONE', #5277, 2.000000000000003109 ) ;
#7031=DIRECTION ( 'NONE',  ( 1.000000000000000000, -5.551115123125773458E-17, -1.260129944081490338E-35 ) ) ;
#7035=CARTESIAN_POINT ( 'NONE',  ( 3.464101615137757051, -5.999999999999979572, -141.3363248654052029 ) ) ;
#7036=VECTOR ( 'NONE', #2124, 1000.000000000000000 ) ;
#7037=EDGE_CURVE ( 'NONE', #11685, #4790, #13652, .T. ) ;
#7041=ORIENTED_EDGE ( 'NONE', *, *, #13078, .T. ) ;
#7042=CARTESIAN_POINT ( 'NONE',  ( -4.763139720814407951, -2.750000000000016431, -110.5000000000000426 ) ) ;
#7045=CARTESIAN_POINT ( 'NONE',  ( -5.412658773652739619, 3.124999999999975131, -133.6830127018922667 ) ) ;
#7048=CARTESIAN_POINT ( 'NONE',  ( -3.608439182435115633, 6.249999999999965361, -171.9419872981078470 ) ) ;
#7050=VERTEX_POINT ( 'NONE', #24502 ) ;
#7052=CARTESIAN_POINT ( 'NONE',  ( 5.061300234018967004, 3.091548682352961208, -180.0000000000001421 ) ) ;
#7053=CARTESIAN_POINT ( 'NONE',  ( 0.000000000000000000, 5.499999999999991118, -181.5000000000000000 ) ) ;
#7055=CARTESIAN_POINT ( 'NONE',  ( -7.216878364870328078, 0.000000000000000000, -180.0580127018922667 ) ) ;
#7056=CARTESIAN_POINT ( 'NONE',  ( -3.464101615137757051, -5.999999999999979572, -111.5863248654051887 ) ) ;
#7057=CARTESIAN_POINT ( 'NONE',  ( -5.999999999999971578, 1.607695154586715303, -122.9806624327025872 ) ) ;
#7059=CARTESIAN_POINT ( 'NONE',  ( -3.175426480542816510, -5.500000000000057732, -123.8749999999999716 ) ) ;
#7068=VERTEX_POINT ( 'NONE', #17476 ) ;
#7071=CARTESIAN_POINT ( 'NONE',  ( 5.412658773652712085, -3.125000000000086153, -111.0669872981078186 ) ) ;
#7078=CARTESIAN_POINT ( 'NONE',  ( 6.000000000000000888, -1.607695154586752384, -141.7306624327026157 ) ) ;
#7080=CARTESIAN_POINT ( 'NONE',  ( -3.608439182435115633, 6.249999999999965361, -137.4419872981078186 ) ) ;
#7085=CARTESIAN_POINT ( 'NONE',  ( -3.464101615137757051, -5.999999999999979572, -171.5863248654051745 ) ) ;
#7086=CARTESIAN_POINT ( 'NONE',  ( 5.412658773652712085, -3.125000000000086153, -59.43301270189227381 ) ) ;
#7088=CARTESIAN_POINT ( 'NONE',  ( -5.999999999999956479, -1.607695154586745057, -125.2693375672974128 ) ) ;
#7089=CYLINDRICAL_SURFACE ( 'NONE', #22656, 6.000000000000000888 ) ;
#7090=CARTESIAN_POINT ( 'NONE',  ( 3.464101615137757051, -5.999999999999979572, -146.4136751345947971 ) ) ;
#7095=EDGE_LOOP ( 'NONE', ( #11410, #16379, #22344, #9621 ) ) ;
#7097=CARTESIAN_POINT ( 'NONE',  ( -4.763139720814407951, 2.749999999999946709, -53.75000000000002132 ) ) ;
#7098=CARTESIAN_POINT ( 'NONE',  ( -3.464101615137725076, 5.999999999999979572, -79.08632486540516027 ) ) ;
#7100=CARTESIAN_POINT ( 'NONE',  ( 4.000000000000006217, -2.220446049250313081E-16, -200.0000000000000000 ) ) ;
#7104=CARTESIAN_POINT ( 'NONE',  ( 2.775557561562891351E-14, 6.250000000000033751, -101.5669872981078186 ) ) ;
#7108=CARTESIAN_POINT ( 'NONE',  ( -4.763139720814407951, 2.749999999999946709, -140.7500000000000284 ) ) ;
#7112=CARTESIAN_POINT ( 'NONE',  ( 6.350852961086080661, -9.614813431917819062E-14, -64.87500000000002842 ) ) ;
#7113=CARTESIAN_POINT ( 'NONE',  ( 6.000000000000000888, 1.743066579297358182E-13, -73.58632486540520290 ) ) ;
#7115=CARTESIAN_POINT ( 'NONE',  ( -7.216878364870328078, 0.000000000000000000, -85.55801270189222407 ) ) ;
#7116=CARTESIAN_POINT ( 'NONE',  ( -5.999999999999963585, -1.487416814333745711E-14, -101.3363248654052171 ) ) ;
#7117=CARTESIAN_POINT ( 'NONE',  ( -5.196152422706573404, -3.000000000000002665, -113.7886751345948397 ) ) ;
#7119=DIRECTION ( 'NONE',  ( -7.147005652999508048E-36, 5.642372883946980038E-36, 1.000000000000000000 ) ) ;
#7122=CARTESIAN_POINT ( 'NONE',  ( -4.763139720814407951, 2.749999999999946709, -149.7500000000000568 ) ) ;
#7125=CARTESIAN_POINT ( 'NONE',  ( -5.412658773652739619, 3.124999999999975131, -160.6830127018922383 ) ) ;
#7126=CARTESIAN_POINT ( 'NONE',  ( -3.464101615137757051, -5.999999999999979572, -149.0863248654052313 ) ) ;
#7128=CARTESIAN_POINT ( 'NONE',  ( 4.763139720814407951, 2.750000000000002665, -82.74999999999998579 ) ) ;
#7130=CARTESIAN_POINT ( 'NONE',  ( 3.175426480543072749, -5.500000000000105693, -62.12500000000000711 ) ) ;
#7135=CARTESIAN_POINT ( 'NONE',  ( -5.999999999999963585, 8.134310703387671600E-14, -144.8363248654052029 ) ) ;
#7138=DIRECTION ( 'NONE',  ( 1.000000000000000000, -5.551115123125773458E-17, -1.260129944081490338E-35 ) ) ;
#7140=CARTESIAN_POINT ( 'NONE',  ( 5.196152422706629359, 3.000000000000002665, -170.0386751345947971 ) ) ;
#7141=( BOUNDED_CURVE ( )  B_SPLINE_CURVE ( 2, ( #222, #11796, #21137, #7299, #4972, #74, #14406, #9459, #18844 ),
 .UNSPECIFIED., .F., .F. ) 
 B_SPLINE_CURVE_WITH_KNOTS ( ( 3, 2, 2, 2, 3 ),
 ( 0.02499999999999991118, 0.02592592592592590783, 0.02777777777777779011, 0.02962962962962967239, 0.03055555555555555802 ),
 .UNSPECIFIED. ) 
 CURVE ( )  GEOMETRIC_REPRESENTATION_ITEM ( )  RATIONAL_B_SPLINE_CURVE ( ( 0.9330127018922194093, 0.9330127018922154125, 1.000000000000000000, 0.8660254037844388186, 1.000000000000000000, 0.8660254037844388186, 1.000000000000000000, 0.9330127018922194093, 0.9330127018922194093 ) ) 
 REPRESENTATION_ITEM ( '' )  );
#7148=( BOUNDED_CURVE ( )  B_SPLINE_CURVE ( 2, ( #21858, #12665, #22467, #19558, #26732, #28893, #7858, #17270, #22002 ),
 .UNSPECIFIED., .F., .T. ) 
 B_SPLINE_CURVE_WITH_KNOTS ( ( 3, 2, 2, 2, 3 ),
 ( 0.8305555555555556024, 0.8314814814814814881, 0.8333333333333333703, 0.8351851851851851416, 0.8361111111111110272 ),
 .UNSPECIFIED. ) 
 CURVE ( )  GEOMETRIC_REPRESENTATION_ITEM ( )  RATIONAL_B_SPLINE_CURVE ( ( 0.9330127018922194093, 0.9330127018922234061, 1.000000000000000000, 0.8660254037844388186, 1.000000000000000000, 0.8660254037844388186, 1.000000000000000000, 0.9330127018922234061, 0.9330127018922194093 ) ) 
 REPRESENTATION_ITEM ( '' )  );
#7149=VECTOR ( 'NONE', #20855, 1000.000000000000000 ) ;
#7151=CARTESIAN_POINT ( 'NONE',  ( -5.412658773652739619, 3.124999999999975131, -152.3169872981078186 ) ) ;
#7153=CARTESIAN_POINT ( 'NONE',  ( -2.775557561562891351E-14, -5.500000000000115463, -89.25000000000005684 ) ) ;
#7154=VERTEX_POINT ( 'NONE', #282 ) ;
#7157=EDGE_CURVE ( 'NONE', #18709, #750, #10737, .T. ) ;
#7158=CARTESIAN_POINT ( 'NONE',  ( 0.000000000000000000, 5.499999999999991118, -166.4999999999999716 ) ) ;
#7161=CARTESIAN_POINT ( 'NONE',  ( 0.000000000000000000, 0.000000000000000000, 0.000000000000000000 ) ) ;
#7163=CARTESIAN_POINT ( 'NONE',  ( 3.175426480543072749, -5.500000000000105693, -170.1250000000000000 ) ) ;
#7165=CARTESIAN_POINT ( 'NONE',  ( 4.763139720814407951, -2.749999999999988454, -153.5000000000000284 ) ) ;
#7167=CARTESIAN_POINT ( 'NONE',  ( 6.350852961086080661, -9.614813431917819062E-14, -103.8750000000000142 ) ) ;
#7169=CARTESIAN_POINT ( 'NONE',  ( 6.000000000000000888, -1.859271017917181981E-14, -84.66367513459482552 ) ) ;
#7170=CARTESIAN_POINT ( 'NONE',  ( 3.175426480543072749, 5.499999999999865885, -157.6250000000000000 ) ) ;
#7171=CARTESIAN_POINT ( 'NONE',  ( 6.350852961086080661, -9.614813431917819062E-14, -88.87500000000000000 ) ) ;
#7174=CARTESIAN_POINT ( 'NONE',  ( -5.196152422706573404, -3.000000000000002665, -136.2886751345947971 ) ) ;
#7175=ORIENTED_EDGE ( 'NONE', *, *, #399, .T. ) ;
#7185=DIRECTION ( 'NONE',  ( -7.147005652999508048E-36, 5.642372883946980038E-36, 1.000000000000000000 ) ) ;
#7188=CARTESIAN_POINT ( 'NONE',  ( 6.000000000000052403, -1.607695154586662678, -141.1533121635129646 ) ) ;
#7190=ORIENTED_EDGE ( 'NONE', *, *, #16445, .F. ) ;
#7193=CARTESIAN_POINT ( 'NONE',  ( 4.763139720814407951, -2.749999999999988454, -112.9999999999999858 ) ) ;
#7195=CARTESIAN_POINT ( 'NONE',  ( 3.608439182435180470, -6.249999999999997335, -128.5580127018922383 ) ) ;
#7198=CARTESIAN_POINT ( 'NONE',  ( -7.216878364870328078, 0.000000000000000000, -167.1919872981078186 ) ) ;
#7202=( BOUNDED_CURVE ( )  B_SPLINE_CURVE ( 2, ( #29164, #29484, #1379, #21980, #10623, #20136, #19972, #6146, #7983 ),
 .UNSPECIFIED., .F., .F. ) 
 B_SPLINE_CURVE_WITH_KNOTS ( ( 3, 2, 2, 2, 3 ),
 ( 0.8694444444444443532, 0.8703703703703703498, 0.8722222222222222321, 0.8740740740740741144, 0.8750000000000000000 ),
 .UNSPECIFIED. ) 
 CURVE ( )  GEOMETRIC_REPRESENTATION_ITEM ( )  RATIONAL_B_SPLINE_CURVE ( ( 0.9330127018922194093, 0.9330127018922154125, 1.000000000000000000, 0.8660254037844388186, 1.000000000000000000, 0.8660254037844388186, 1.000000000000000000, 0.9330127018922194093, 0.9330127018922194093 ) ) 
 REPRESENTATION_ITEM ( '' )  );
#7204=FACE_OUTER_BOUND ( 'NONE', #22588, .T. ) ;
#7205=CARTESIAN_POINT ( 'NONE',  ( -3.175426480542816510, 5.499999999999865885, -181.3750000000000000 ) ) ;
#7207=CARTESIAN_POINT ( 'NONE',  ( 2.775557561562891351E-14, -6.250000000000061284, -176.6830127018922383 ) ) ;
#7210=EDGE_CURVE ( 'NONE', #21073, #3256, #25988, .T. ) ;
#7212=CARTESIAN_POINT ( 'NONE',  ( 0.000000000000000000, 5.499999999999991118, -110.9999999999999858 ) ) ;
#7221=VECTOR ( 'NONE', #28539, 1000.000000000000000 ) ;
#7227=DIRECTION ( 'NONE',  ( 1.000000000000000000, -5.551115123125773458E-17, -1.260129944081490338E-35 ) ) ;
#7228=CYLINDRICAL_SURFACE ( 'NONE', #2709, 6.000000000000000888 ) ;
#7229=CARTESIAN_POINT ( 'NONE',  ( 6.000000000000000888, -3.330669073875464691E-16, -7.560779664488942560E-35 ) ) ;
#7231=ORIENTED_EDGE ( 'NONE', *, *, #23751, .T. ) ;
#7232=ORIENTED_EDGE ( 'NONE', *, *, #23, .F. ) ;
#7235=ORIENTED_EDGE ( 'NONE', *, *, #14496, .T. ) ;
#7236=CARTESIAN_POINT ( 'NONE',  ( -5.412658773652739619, 3.124999999999975131, -143.3169872981078186 ) ) ;
#7238=VECTOR ( 'NONE', #1158, 1000.000000000000000 ) ;
#7239=CYLINDRICAL_SURFACE ( 'NONE', #30275, 6.000000000000000888 ) ;
#7241=EDGE_CURVE ( 'NONE', #28373, #22535, #8230, .T. ) ;
#7243=DIRECTION ( 'NONE',  ( -1.000000000000000000, 5.551115123125774690E-17, 0.000000000000000000 ) ) ;
#7244=( BOUNDED_CURVE ( )  B_SPLINE_CURVE ( 2, ( #27016, #24723, #3970, #3663, #22435, #15706, #24871, #20129, #27168 ),
 .UNSPECIFIED., .F., .T. ) 
 B_SPLINE_CURVE_WITH_KNOTS ( ( 3, 2, 2, 2, 3 ),
 ( 0.5249999999999999112, 0.5259259259259259078, 0.5277777777777777901, 0.5296296296296296724, 0.5305555555555555580 ),
 .UNSPECIFIED. ) 
 CURVE ( )  GEOMETRIC_REPRESENTATION_ITEM ( )  RATIONAL_B_SPLINE_CURVE ( ( 0.9330127018922194093, 0.9330127018922114157, 1.000000000000000000, 0.8660254037844388186, 1.000000000000000000, 0.8660254037844388186, 1.000000000000000000, 0.9330127018922194093, 0.9330127018922194093 ) ) 
 REPRESENTATION_ITEM ( '' )  );
#7246=DIRECTION ( 'NONE',  ( 1.000000000000000000, -5.551115123125773458E-17, -1.260129944081490338E-35 ) ) ;
#7247=CARTESIAN_POINT ( 'NONE',  ( -6.000000000000007105, -1.607695154586655129, -70.34668783648702117 ) ) ;
#7253=ORIENTED_EDGE ( 'NONE', *, *, #12748, .T. ) ;
#7254=CARTESIAN_POINT ( 'NONE',  ( 5.196152422706629359, -2.999999999999988898, -106.7113248654052455 ) ) ;
#7255=CARTESIAN_POINT ( 'NONE',  ( 5.196152422706629359, -2.999999999999988898, -132.7886751345947971 ) ) ;
#7257=CARTESIAN_POINT ( 'NONE',  ( 3.464101615137757051, -5.999999999999979572, -163.8363248654052597 ) ) ;
#7260=VECTOR ( 'NONE', #20841, 1000.000000000000000 ) ;
#7262=CARTESIAN_POINT ( 'NONE',  ( 3.608439182435180470, 6.249999999999982236, -104.6919872981078328 ) ) ;
#7269=CARTESIAN_POINT ( 'NONE',  ( 4.763139720814407951, 2.750000000000002665, -130.7500000000000284 ) ) ;
#7270=ORIENTED_EDGE ( 'NONE', *, *, #9650, .T. ) ;
#7274=CARTESIAN_POINT ( 'NONE',  ( -4.763139720814407951, 2.749999999999946709, -62.75000000000002842 ) ) ;
#7277=CARTESIAN_POINT ( 'NONE',  ( -6.000000000000000888, 1.067854986875958443E-15, 7.560779664488942560E-35 ) ) ;
#7279=CARTESIAN_POINT ( 'NONE',  ( -7.216878364870328078, 0.000000000000000000, -87.05801270189222407 ) ) ;
#7280=CARTESIAN_POINT ( 'NONE',  ( 6.000000000000000888, 1.743066579297358182E-13, -65.16367513459479710 ) ) ;
#7282=CARTESIAN_POINT ( 'NONE',  ( -5.196152422706573404, -3.000000000000002665, -176.2113248654052597 ) ) ;
#7283=CYLINDRICAL_SURFACE ( 'NONE', #20170, 6.000000000000000888 ) ;
#7285=CARTESIAN_POINT ( 'NONE',  ( -6.350852961085760029, -1.281975124255709124E-13, -142.1250000000000000 ) ) ;
#7287=CARTESIAN_POINT ( 'NONE',  ( -3.608439182435052128, -6.250000000000110134, -155.8080127018922383 ) ) ;
#7288=FILL_AREA_STYLE_COLOUR ( '', #10195 ) ;
#7289=CARTESIAN_POINT ( 'NONE',  ( -6.000000000000007105, -1.607695154586655129, -73.34668783648702117 ) ) ;
#7290=CARTESIAN_POINT ( 'NONE',  ( 3.175426480543072749, 5.499999999999865885, -78.12500000000001421 ) ) ;
#7292=CARTESIAN_POINT ( 'NONE',  ( 3.175426480543072749, 5.499999999999865885, -63.12500000000001421 ) ) ;
#7299=CARTESIAN_POINT ( 'NONE',  ( 3.464101615137757051, -5.999999999999979572, -49.83632486540522422 ) ) ;
#7301=CARTESIAN_POINT ( 'NONE',  ( 0.000000000000000000, 0.000000000000000000, 0.000000000000000000 ) ) ;
#7308=VERTEX_POINT ( 'NONE', #11033 ) ;
#7309=CARTESIAN_POINT ( 'NONE',  ( -2.775557561562891351E-14, -5.500000000000115463, -90.75000000000000000 ) ) ;
#7312=ORIENTED_EDGE ( 'NONE', *, *, #28854, .F. ) ;
#7315=CARTESIAN_POINT ( 'NONE',  ( 6.000000000000000888, 1.607695154586715303, -59.09668783648705670 ) ) ;
#7316=CARTESIAN_POINT ( 'NONE',  ( 3.175426480543072749, 5.499999999999865885, -175.6250000000000284 ) ) ;
#7318=CARTESIAN_POINT ( 'NONE',  ( -4.763139720814407951, 2.749999999999946709, -155.7500000000000568 ) ) ;
#7320=CARTESIAN_POINT ( 'NONE',  ( 6.000000000000000888, 1.743066579297358182E-13, -51.66367513459483263 ) ) ;
#7322=CARTESIAN_POINT ( 'NONE',  ( 5.196152422706629359, 3.000000000000002665, -59.96132486540523132 ) ) ;
#7324=CARTESIAN_POINT ( 'NONE',  ( 4.763139720814407951, -2.749999999999988454, -86.00000000000001421 ) ) ;
#7333=( BOUNDED_CURVE ( )  B_SPLINE_CURVE ( 2, ( #23860, #16680, #9889, #9435, #14659, #494, #16533, #19114, #26002 ),
 .UNSPECIFIED., .F., .T. ) 
 B_SPLINE_CURVE_WITH_KNOTS ( ( 3, 2, 2, 2, 3 ),
 ( 0.01388888888888888465, 0.01481481481481481538, 0.01666666666666666644, 0.01851851851851851749, 0.01944444444444445169 ),
 .UNSPECIFIED. ) 
 CURVE ( )  GEOMETRIC_REPRESENTATION_ITEM ( )  RATIONAL_B_SPLINE_CURVE ( ( 0.9330127018922194093, 0.9330127018922190762, 1.000000000000000000, 0.8660254037844388186, 1.000000000000000000, 0.8660254037844388186, 1.000000000000000000, 0.9330127018922189652, 0.9330127018922194093 ) ) 
 REPRESENTATION_ITEM ( '' )  );
#7334=ORIENTED_EDGE ( 'NONE', *, *, #25239, .T. ) ;
#7335=CARTESIAN_POINT ( 'NONE',  ( -5.999999999999965361, 1.607695154586723518, -178.4806624327025872 ) ) ;
#7340=ORIENTED_EDGE ( 'NONE', *, *, #26796, .T. ) ;
#7341=EDGE_LOOP ( 'NONE', ( #16774, #11058, #22995, #17067 ) ) ;
#7343=CARTESIAN_POINT ( 'NONE',  ( 6.350852961086080661, -9.614813431917819062E-14, -114.3750000000000000 ) ) ;
#7345=EDGE_CURVE ( 'NONE', #14802, #21664, #11503, .T. ) ;
#7346=CARTESIAN_POINT ( 'NONE',  ( -3.608439182435115633, 6.249999999999965361, -120.3080127018922667 ) ) ;
#7347=ORIENTED_EDGE ( 'NONE', *, *, #16469, .F. ) ;
#7349=AXIS2_PLACEMENT_3D ( 'NONE', #25726, #29353, #6630 ) ;
#7350=CARTESIAN_POINT ( 'NONE',  ( 5.412658773652712085, -3.125000000000086153, -162.0669872981078186 ) ) ;
#7357=CARTESIAN_POINT ( 'NONE',  ( 3.175426480543072749, 5.499999999999865885, -177.1250000000000284 ) ) ;
#7359=CARTESIAN_POINT ( 'NONE',  ( 3.608439182435180470, 6.249999999999982236, -173.0580127018922667 ) ) ;
#7361=CARTESIAN_POINT ( 'NONE',  ( 6.000000000000000888, -1.607695154586752384, -101.2306624327026157 ) ) ;
#7362=CARTESIAN_POINT ( 'NONE',  ( 0.000000000000000000, 5.499999999999991118, -126.0000000000000000 ) ) ;
#7363=CARTESIAN_POINT ( 'NONE',  ( 3.464101615137757051, -5.999999999999979572, -53.41367513459480421 ) ) ;
#7364=CARTESIAN_POINT ( 'NONE',  ( 6.350852961086080661, -9.614813431917819062E-14, -117.3750000000000142 ) ) ;
#7368=CARTESIAN_POINT ( 'NONE',  ( -6.000000000000000888, 1.067854986875958443E-15, 7.560779664488942560E-35 ) ) ;
#7369=CARTESIAN_POINT ( 'NONE',  ( 3.464101615137852974, 5.999999999999884537, -168.4136751345948255 ) ) ;
#7370=FACE_OUTER_BOUND ( 'NONE', #30006, .T. ) ;
#7371=EDGE_LOOP ( 'NONE', ( #26911, #8889, #6239, #14577 ) ) ;
#7374=CARTESIAN_POINT ( 'NONE',  ( 6.350852961086080661, -9.614813431917819062E-14, -177.3750000000000284 ) ) ;
#7375=EDGE_CURVE ( 'NONE', #15286, #12915, #25264, .T. ) ;
#7377=CARTESIAN_POINT ( 'NONE',  ( -5.999999999999982236, -1.607695154586700426, -125.8466878364870638 ) ) ;
#7381=CARTESIAN_POINT ( 'NONE',  ( -5.999999999999963585, 8.134310703387671600E-14, -140.9136751345947971 ) ) ;
#7384=ORIENTED_EDGE ( 'NONE', *, *, #5104, .F. ) ;
#7385=CARTESIAN_POINT ( 'NONE',  ( 5.412658773652739619, 3.124999999999988898, -139.3169872981078186 ) ) ;
#7388=CARTESIAN_POINT ( 'NONE',  ( -5.196152422706573404, -3.000000000000002665, -116.7886751345948397 ) ) ;
#7389=AXIS2_PLACEMENT_3D ( 'NONE', #16648, #12487, #24114 ) ;
#7392=CARTESIAN_POINT ( 'NONE',  ( 6.000000000000000888, 1.743066579297358182E-13, -91.58632486540523132 ) ) ;
#7393=VECTOR ( 'NONE', #25816, 1000.000000000000000 ) ;
#7396=CARTESIAN_POINT ( 'NONE',  ( -5.999999999999963585, -1.487416814333745711E-14, -92.33632486540518869 ) ) ;
#7397=CARTESIAN_POINT ( 'NONE',  ( -5.999999999999963585, 8.134310703387671600E-14, -146.3363248654052313 ) ) ;
#7403=CARTESIAN_POINT ( 'NONE',  ( 4.763139720814407951, -2.749999999999988454, -50.00000000000004263 ) ) ;
#7404=CARTESIAN_POINT ( 'NONE',  ( -5.196152422706601826, 2.999999999999975131, -52.53867513459481131 ) ) ;
#7405=CARTESIAN_POINT ( 'NONE',  ( 6.000000000000000888, -1.859271017917181981E-14, -79.58632486540520290 ) ) ;
#7410=CARTESIAN_POINT ( 'NONE',  ( 5.412658773652712085, -3.125000000000086153, -103.5669872981078186 ) ) ;
#7411=CARTESIAN_POINT ( 'NONE',  ( -5.999999999999963585, -2.788906526875773208E-15, -176.3363248654052029 ) ) ;
#7415=CARTESIAN_POINT ( 'NONE',  ( -6.350852961085760029, -1.281975124255709124E-13, -128.6250000000000000 ) ) ;
#7416=( BOUNDED_CURVE ( )  B_SPLINE_CURVE ( 2, ( #16779, #26104, #5047, #14478, #7511, #5200, #2901, #12322, #21665 ),
 .UNSPECIFIED., .F., .T. ) 
 B_SPLINE_CURVE_WITH_KNOTS ( ( 3, 2, 2, 2, 3 ),
 ( 0.5916666666666666741, 0.5925925925925925597, 0.5944444444444444420, 0.5962962962962963243, 0.5972222222222222099 ),
 .UNSPECIFIED. ) 
 CURVE ( )  GEOMETRIC_REPRESENTATION_ITEM ( )  RATIONAL_B_SPLINE_CURVE ( ( 0.9330127018922194093, 0.9330127018922194093, 1.000000000000000000, 0.8660254037844388186, 1.000000000000000000, 0.8660254037844388186, 1.000000000000000000, 0.9330127018922194093, 0.9330127018922194093 ) ) 
 REPRESENTATION_ITEM ( '' )  );
#7417=EDGE_CURVE ( 'NONE', #24851, #17475, #23047, .T. ) ;
#7419=CARTESIAN_POINT ( 'NONE',  ( 3.175426480543072749, -5.500000000000105693, -56.12500000000004263 ) ) ;
#7421=CARTESIAN_POINT ( 'NONE',  ( 3.608439182435180470, 6.249999999999982236, -84.55801270189220986 ) ) ;
#7425=CARTESIAN_POINT ( 'NONE',  ( 3.175426480543072749, 5.499999999999865885, -138.1250000000000568 ) ) ;
#7428=CARTESIAN_POINT ( 'NONE',  ( -5.412658773652739619, 3.124999999999975131, -153.1830127018922667 ) ) ;
#7429=CARTESIAN_POINT ( 'NONE',  ( -5.999999999999971578, 1.607695154586715303, -116.4033121635130072 ) ) ;
#7430=CARTESIAN_POINT ( 'NONE',  ( -4.763139720814407951, -2.750000000000016431, -74.50000000000001421 ) ) ;
#7431=CARTESIAN_POINT ( 'NONE',  ( 6.000000000000000888, 1.743066579297358182E-13, -86.16367513459481131 ) ) ;
#7432=CARTESIAN_POINT ( 'NONE',  ( -6.350852961085760029, -1.281975124255709124E-13, -68.62500000000004263 ) ) ;
#7437=CARTESIAN_POINT ( 'NONE',  ( 5.196152422706629359, 3.000000000000002665, -82.46132486540524553 ) ) ;
#7438=ORIENTED_EDGE ( 'NONE', *, *, #14704, .T. ) ;
#7445=CARTESIAN_POINT ( 'NONE',  ( -4.763139720814407951, -2.750000000000016431, -179.5000000000000000 ) ) ;
#7447=CARTESIAN_POINT ( 'NONE',  ( -7.216878364870328078, 0.000000000000000000, -153.6919872981078186 ) ) ;
#7449=CARTESIAN_POINT ( 'NONE',  ( -4.763139720814407951, 2.749999999999946709, -85.25000000000004263 ) ) ;
#7450=CARTESIAN_POINT ( 'NONE',  ( 3.608439182435180470, -6.249999999999997335, -100.0580127018922383 ) ) ;
#7451=ORIENTED_EDGE ( 'NONE', *, *, #10027, .T. ) ;
#7459=CARTESIAN_POINT ( 'NONE',  ( -6.350852961085760029, -1.281975124255709124E-13, -166.1249999999999716 ) ) ;
#7461=CARTESIAN_POINT ( 'NONE',  ( 4.763139720814407951, -2.749999999999988454, -158.0000000000000284 ) ) ;
#7463=CARTESIAN_POINT ( 'NONE',  ( 4.763139720814407951, 2.750000000000002665, -91.75000000000000000 ) ) ;
#7466=CARTESIAN_POINT ( 'NONE',  ( 0.000000000000000000, 5.499999999999991118, -85.50000000000001421 ) ) ;
#7473=DIRECTION ( 'NONE',  ( -7.147005652999508048E-36, 5.642372883946980038E-36, 1.000000000000000000 ) ) ;
#7474=EDGE_CURVE ( 'NONE', #13496, #6372, #13464, .T. ) ;
#7477=CARTESIAN_POINT ( 'NONE',  ( 6.000000000000000888, -3.330669073875464691E-16, -7.560779664488942560E-35 ) ) ;
#7481=CARTESIAN_POINT ( 'NONE',  ( -2.775557561562891351E-14, -5.500000000000115463, -114.7500000000000142 ) ) ;
#7483=CARTESIAN_POINT ( 'NONE',  ( 2.775557561562891351E-14, 6.250000000000033751, -126.4330127018922241 ) ) ;
#7487=CARTESIAN_POINT ( 'NONE',  ( 5.196152422706629359, -2.999999999999988898, -68.28867513459479710 ) ) ;
#7488=CARTESIAN_POINT ( 'NONE',  ( -3.608439182435052128, -6.250000000000110134, -160.9419872981077901 ) ) ;
#7490=ORIENTED_EDGE ( 'NONE', *, *, #9039, .T. ) ;
#7491=( BOUNDED_CURVE ( )  B_SPLINE_CURVE ( 2, ( #16402, #4672, #14107, #27400, #6365, #8847, #15797, #25104, #22823 ),
 .UNSPECIFIED., .F., .T. ) 
 B_SPLINE_CURVE_WITH_KNOTS ( ( 3, 2, 2, 2, 3 ),
 ( 0.04722222222222221405, 0.04814814814814814825, 0.05000000000000000278, 0.05185185185185185036, 0.05277777777777778456 ),
 .UNSPECIFIED. ) 
 CURVE ( )  GEOMETRIC_REPRESENTATION_ITEM ( )  RATIONAL_B_SPLINE_CURVE ( ( 0.9330127018922194093, 0.9330127018922189652, 1.000000000000000000, 0.8660254037844388186, 1.000000000000000000, 0.8660254037844388186, 1.000000000000000000, 0.9330127018922189652, 0.9330127018922194093 ) ) 
 REPRESENTATION_ITEM ( '' )  );
#7492=CARTESIAN_POINT ( 'NONE',  ( -5.999999999999904965, -1.607695154586834541, -132.7693375672974696 ) ) ;
#7495=CARTESIAN_POINT ( 'NONE',  ( 2.775557561562891351E-14, 6.250000000000033751, -178.9330127018922099 ) ) ;
#7498=CARTESIAN_POINT ( 'NONE',  ( 6.350852961086080661, -9.614813431917819062E-14, -126.3749999999999858 ) ) ;
#7500=CARTESIAN_POINT ( 'NONE',  ( 4.763139720814407951, -2.749999999999988454, -109.9999999999999858 ) ) ;
#7501=( BOUNDED_CURVE ( )  B_SPLINE_CURVE ( 2, ( #20759, #11877, #23809, #2898, #21213, #28683, #16920, #14754, #7657 ),
 .UNSPECIFIED., .F., .T. ) 
 B_SPLINE_CURVE_WITH_KNOTS ( ( 3, 2, 2, 2, 3 ),
 ( 0.06944444444444441977, 0.07037037037037041642, 0.07222222222222218768, 0.07407407407407406996, 0.07500000000000006661 ),
 .UNSPECIFIED. ) 
 CURVE ( )  GEOMETRIC_REPRESENTATION_ITEM ( )  RATIONAL_B_SPLINE_CURVE ( ( 0.9330127018922194093, 0.9330127018922154125, 1.000000000000000000, 0.8660254037844388186, 1.000000000000000000, 0.8660254037844388186, 1.000000000000000000, 0.9330127018922154125, 0.9330127018922194093 ) ) 
 REPRESENTATION_ITEM ( '' )  );
#7503=ORIENTED_EDGE ( 'NONE', *, *, #21545, .F. ) ;
#7506=CARTESIAN_POINT ( 'NONE',  ( 5.999999999999949374, -1.607695154586841868, -136.6533121635129930 ) ) ;
#7507=CARTESIAN_POINT ( 'NONE',  ( 0.000000000000000000, 0.000000000000000000, 0.000000000000000000 ) ) ;
#7508=EDGE_CURVE ( 'NONE', #20807, #18212, #21700, .T. ) ;
#7510=ORIENTED_EDGE ( 'NONE', *, *, #20517, .F. ) ;
#7511=CARTESIAN_POINT ( 'NONE',  ( 0.000000000000000000, -5.999999999999991118, -126.4613248654052313 ) ) ;
#7512=CARTESIAN_POINT ( 'NONE',  ( -2.775557561562891351E-14, -5.500000000000115463, -176.2500000000000284 ) ) ;
#7514=ORIENTED_EDGE ( 'NONE', *, *, #21167, .T. ) ;
#7517=VERTEX_POINT ( 'NONE', #19786 ) ;
#7520=ORIENTED_EDGE ( 'NONE', *, *, #16411, .T. ) ;
#7521=CARTESIAN_POINT ( 'NONE',  ( -5.412658773652739619, 3.124999999999975131, -131.3169872981078186 ) ) ;
#7525=ORIENTED_EDGE ( 'NONE', *, *, #7844, .F. ) ;
#7527=DIRECTION ( 'NONE',  ( 1.000000000000000000, -5.551115123125773458E-17, -1.260129944081490338E-35 ) ) ;
#7528=CARTESIAN_POINT ( 'NONE',  ( 6.000000000000000888, -3.330669073875464691E-16, -7.560779664488942560E-35 ) ) ;
#7532=EDGE_CURVE ( 'NONE', #18704, #16190, #24815, .T. ) ;
#7535=CARTESIAN_POINT ( 'NONE',  ( 0.000000000000000000, -5.999999999999991118, -142.9613248654052597 ) ) ;
#7536=CARTESIAN_POINT ( 'NONE',  ( 6.350852961086080661, -9.614813431917819062E-14, -135.3750000000000284 ) ) ;
#7538=( BOUNDED_CURVE ( )  B_SPLINE_CURVE ( 2, ( #7587, #23747, #12397, #19726, #28479, #7738, #16854, #2679, #14686 ),
 .UNSPECIFIED., .F., .F. ) 
 B_SPLINE_CURVE_WITH_KNOTS ( ( 3, 2, 2, 2, 3 ),
 ( 0.1305555555555556468, 0.1314814814814815325, 0.1333333333333333037, 0.1351851851851851860, 0.1361111111111110716 ),
 .UNSPECIFIED. ) 
 CURVE ( )  GEOMETRIC_REPRESENTATION_ITEM ( )  RATIONAL_B_SPLINE_CURVE ( ( 0.9330127018922194093, 0.9330127018922234061, 1.000000000000000000, 0.8660254037844388186, 1.000000000000000000, 0.8660254037844388186, 1.000000000000000000, 0.9330127018922234061, 0.9330127018922194093 ) ) 
 REPRESENTATION_ITEM ( '' )  );
#7541=CARTESIAN_POINT ( 'NONE',  ( -5.999999999999963585, 1.780251999655701777E-13, -107.3363248654052455 ) ) ;
#7542=CARTESIAN_POINT ( 'NONE',  ( 0.000000000000000000, 5.999999999999977796, -88.21132486540523132 ) ) ;
#7549=CARTESIAN_POINT ( 'NONE',  ( 3.608439182435180470, -6.249999999999997335, -93.19198729810779014 ) ) ;
#7552=CARTESIAN_POINT ( 'NONE',  ( 3.175426480543072749, -5.500000000000105693, -126.6250000000000000 ) ) ;
#7553=EDGE_LOOP ( 'NONE', ( #6646, #1152, #1593, #23403 ) ) ;
#7555=CARTESIAN_POINT ( 'NONE',  ( -3.175426480542816510, 5.499999999999865885, -58.37500000000004974 ) ) ;
#7556=FACE_OUTER_BOUND ( 'NONE', #22946, .T. ) ;
#7557=CARTESIAN_POINT ( 'NONE',  ( -3.608439182435115633, 6.249999999999965361, -85.80801270189222407 ) ) ;
#7560=LINE ( 'NONE', #808, #2511 ) ;
#7561=EDGE_CURVE ( 'NONE', #26173, #4711, #26155, .T. ) ;
#7564=CARTESIAN_POINT ( 'NONE',  ( 0.000000000000000000, 5.499999999999991118, -139.5000000000000000 ) ) ;
#7566=CARTESIAN_POINT ( 'NONE',  ( -7.216878364870328078, 0.000000000000000000, -154.5580127018922383 ) ) ;
#7567=CARTESIAN_POINT ( 'NONE',  ( 3.464101615137852974, 5.999999999999884537, -158.8363248654052313 ) ) ;
#7568=CARTESIAN_POINT ( 'NONE',  ( -5.999999999999963585, -1.487416814333745711E-14, -50.91367513459483973 ) ) ;
#7570=VECTOR ( 'NONE', #11785, 1000.000000000000000 ) ;
#7571=CARTESIAN_POINT ( 'NONE',  ( -6.350852961085760029, -1.281975124255709124E-13, -70.12500000000004263 ) ) ;
#7573=CARTESIAN_POINT ( 'NONE',  ( 3.175426480543072749, 5.499999999999865885, -66.12500000000002842 ) ) ;
#7579=CARTESIAN_POINT ( 'NONE',  ( -6.000000000000007105, -1.607695154586655129, -89.26933756729744118 ) ) ;
#7581=CARTESIAN_POINT ( 'NONE',  ( -5.999999999999963585, 8.134310703387671600E-14, -145.4136751345948539 ) ) ;
#7587=CARTESIAN_POINT ( 'NONE',  ( -5.999999999999963585, 1.780251999655701777E-13, -63.83632486540523132 ) ) ;
#7588=CARTESIAN_POINT ( 'NONE',  ( 4.763139720814407951, 2.750000000000002665, -178.7500000000000284 ) ) ;
#7590=CARTESIAN_POINT ( 'NONE',  ( 3.608439182435180470, 6.249999999999982236, -155.6919872981078186 ) ) ;
#7592=CARTESIAN_POINT ( 'NONE',  ( -3.175426480542816510, 5.499999999999865885, -82.37500000000002842 ) ) ;
#7594=CARTESIAN_POINT ( 'NONE',  ( 4.763139720814407951, 2.750000000000002665, -168.2500000000000000 ) ) ;
#7597=DIRECTION ( 'NONE',  ( 1.000000000000000000, -5.551115123125773458E-17, -1.260129944081490338E-35 ) ) ;
#7599=CARTESIAN_POINT ( 'NONE',  ( 3.175426480543072749, 5.499999999999865885, -162.1250000000000284 ) ) ;
#7600=CARTESIAN_POINT ( 'NONE',  ( 4.763139720814407951, 2.750000000000002665, -154.7500000000000568 ) ) ;
#7602=CARTESIAN_POINT ( 'NONE',  ( -5.196152422706573404, -3.000000000000002665, -104.2113248654051887 ) ) ;
#7604=CARTESIAN_POINT ( 'NONE',  ( -2.775557561562891351E-14, -5.500000000000115463, -98.25000000000000000 ) ) ;
#7605=CARTESIAN_POINT ( 'NONE',  ( 5.196152422706629359, 3.000000000000002665, -125.9613248654052313 ) ) ;
#7608=CARTESIAN_POINT ( 'NONE',  ( -6.350852961085760029, -1.281975124255709124E-13, -89.62500000000000000 ) ) ;
#7609=CYLINDRICAL_SURFACE ( 'NONE', #22165, 6.000000000000000888 ) ;
#7611=CARTESIAN_POINT ( 'NONE',  ( -3.464101615137757051, -5.999999999999979572, -72.58632486540520290 ) ) ;
#7615=DIRECTION ( 'NONE',  ( 1.000000000000000000, -5.551115123125773458E-17, -1.260129944081490338E-35 ) ) ;
#7617=CYLINDRICAL_SURFACE ( 'NONE', #1222, 6.000000000000000888 ) ;
#7625=CARTESIAN_POINT ( 'NONE',  ( -2.775557561562891351E-14, -5.500000000000115463, -107.2500000000000142 ) ) ;
#7627=CARTESIAN_POINT ( 'NONE',  ( -3.175426480542816510, 5.499999999999865885, -149.8750000000000568 ) ) ;
#7628=CARTESIAN_POINT ( 'NONE',  ( 3.608439182435180470, 6.249999999999982236, -123.5580127018922099 ) ) ;
#7629=EDGE_LOOP ( 'NONE', ( #10256, #8663, #9468, #2202 ) ) ;
#7630=CARTESIAN_POINT ( 'NONE',  ( -6.000000000000007105, -1.607695154586655129, -61.34668783648706381 ) ) ;
#7631=CARTESIAN_POINT ( 'NONE',  ( 3.608439182435180470, -6.249999999999997335, -157.6919872981078470 ) ) ;
#7635=CARTESIAN_POINT ( 'NONE',  ( 5.412658773652712085, -3.125000000000086153, -62.43301270189222407 ) ) ;
#7636=ORIENTED_EDGE ( 'NONE', *, *, #27252, .T. ) ;
#7639=CARTESIAN_POINT ( 'NONE',  ( -5.999999999999963585, -1.487416814333745711E-14, -132.8363248654052597 ) ) ;
#7641=DIRECTION ( 'NONE',  ( -7.147005652999508048E-36, 5.642372883946980038E-36, 1.000000000000000000 ) ) ;
#7644=CARTESIAN_POINT ( 'NONE',  ( 3.464101615137757051, -5.999999999999979572, -168.9136751345948255 ) ) ;
#7645=CARTESIAN_POINT ( 'NONE',  ( -7.216878364870328078, 0.000000000000000000, -171.0580127018922383 ) ) ;
#7646=CARTESIAN_POINT ( 'NONE',  ( 2.000000000000003109, -1.110223024625156540E-16, -185.0000000000000000 ) ) ;
#7648=CARTESIAN_POINT ( 'NONE',  ( 4.763139720814407951, -2.749999999999988454, -119.0000000000000000 ) ) ;
#7650=CARTESIAN_POINT ( 'NONE',  ( 3.175426480543072749, 5.499999999999865885, -112.6249999999999858 ) ) ;
#7656=DIRECTION ( 'NONE',  ( -7.147005652999508048E-36, 5.642372883946980038E-36, 1.000000000000000000 ) ) ;
#7657=CARTESIAN_POINT ( 'NONE',  ( -5.999999999999963585, 1.780251999655701777E-13, -56.33632486540525264 ) ) ;
#7662=CARTESIAN_POINT ( 'NONE',  ( -6.000000000000007105, -1.607695154586655129, -95.84668783648702117 ) ) ;
#7665=AXIS2_PLACEMENT_3D ( 'NONE', #29018, #26568, #5370 ) ;
#7669=ORIENTED_EDGE ( 'NONE', *, *, #27746, .T. ) ;
#7670=CARTESIAN_POINT ( 'NONE',  ( 2.775557561562891351E-14, -6.250000000000061284, -127.8169872981078043 ) ) ;
#7677=CARTESIAN_POINT ( 'NONE',  ( -3.464101615137757051, -5.999999999999979572, -92.08632486540523132 ) ) ;
#7678=EDGE_CURVE ( 'NONE', #29837, #26645, #24013, .T. ) ;
#7679=CARTESIAN_POINT ( 'NONE',  ( 6.000000000000000888, -3.330669073875464691E-16, -7.560779664488942560E-35 ) ) ;
#7680=( BOUNDED_CURVE ( )  B_SPLINE_CURVE ( 2, ( #26463, #3566, #10217, #26315, #5272, #24025, #10062, #19439, #26613 ),
 .UNSPECIFIED., .F., .T. ) 
 B_SPLINE_CURVE_WITH_KNOTS ( ( 3, 2, 2, 2, 3 ),
 ( 0.5694444444444444198, 0.5703703703703704164, 0.5722222222222221877, 0.5740740740740740700, 0.5750000000000000666 ),
 .UNSPECIFIED. ) 
 CURVE ( )  GEOMETRIC_REPRESENTATION_ITEM ( )  RATIONAL_B_SPLINE_CURVE ( ( 0.9330127018922194093, 0.9330127018922154125, 1.000000000000000000, 0.8660254037844388186, 1.000000000000000000, 0.8660254037844388186, 1.000000000000000000, 0.9330127018922154125, 0.9330127018922194093 ) ) 
 REPRESENTATION_ITEM ( '' )  );
#7682=CARTESIAN_POINT ( 'NONE',  ( -5.999999999999963585, 1.780251999655701777E-13, -99.83632486540521711 ) ) ;
#7683=CARTESIAN_POINT ( 'NONE',  ( 3.464101615137757051, -5.999999999999979572, -139.8363248654052597 ) ) ;
#7684=CARTESIAN_POINT ( 'NONE',  ( -3.464101615137757051, -5.999999999999979572, -69.58632486540518869 ) ) ;
#7687=CARTESIAN_POINT ( 'NONE',  ( -3.175426480542816510, -5.500000000000057732, -134.3750000000000284 ) ) ;
#7689=ORIENTED_EDGE ( 'NONE', *, *, #4930, .F. ) ;
#7690=CARTESIAN_POINT ( 'NONE',  ( -6.350852961085760029, -1.281975124255709124E-13, -47.62500000000000000 ) ) ;
#7691=CARTESIAN_POINT ( 'NONE',  ( -5.999999999999963585, 1.780251999655701777E-13, -93.83632486540518869 ) ) ;
#7692=CARTESIAN_POINT ( 'NONE',  ( -5.999999999999963585, 1.780251999655701777E-13, -100.4136751345948255 ) ) ;
#7694=VECTOR ( 'NONE', #6955, 1000.000000000000000 ) ;
#7697=CARTESIAN_POINT ( 'NONE',  ( 5.412658773652739619, 3.124999999999988898, -95.81698729810783277 ) ) ;
#7701=ORIENTED_EDGE ( 'NONE', *, *, #933, .F. ) ;
#7702=AXIS2_PLACEMENT_3D ( 'NONE', #3613, #11029, #13205 ) ;
#7704=ADVANCED_FACE ( 'NONE', ( #1095 ), #5843, .T. ) ;
#7705=CARTESIAN_POINT ( 'NONE',  ( 4.763139720814407951, -2.749999999999988454, -126.5000000000000568 ) ) ;
#7708=ORIENTED_EDGE ( 'NONE', *, *, #22539, .F. ) ;
#7709=CARTESIAN_POINT ( 'NONE',  ( 5.196152422706629359, -2.999999999999988898, -138.2113248654052029 ) ) ;
#7710=CARTESIAN_POINT ( 'NONE',  ( -3.175426480542816510, -5.500000000000057732, -60.87500000000000000 ) ) ;
#7712=CARTESIAN_POINT ( 'NONE',  ( 4.520081486476311028, 10.03271082534597269, -28.96438617129775395 ) ) ;
#7713=CARTESIAN_POINT ( 'NONE',  ( 2.775557561562891351E-14, -6.250000000000061284, -80.68301270189226670 ) ) ;
#7715=CARTESIAN_POINT ( 'NONE',  ( -3.464101615137757051, -5.999999999999979572, -101.0863248654051887 ) ) ;
#7716=CARTESIAN_POINT ( 'NONE',  ( 0.000000000000000000, 0.000000000000000000, 0.000000000000000000 ) ) ;
#7717=CARTESIAN_POINT ( 'NONE',  ( 0.000000000000000000, -5.999999999999991118, -152.5386751345948539 ) ) ;
#7720=CARTESIAN_POINT ( 'NONE',  ( 6.350852961086080661, -9.614813431917819062E-14, -136.8750000000000568 ) ) ;
#7722=CARTESIAN_POINT ( 'NONE',  ( -7.216878364870328078, 0.000000000000000000, -150.0580127018922667 ) ) ;
#7723=CARTESIAN_POINT ( 'NONE',  ( 3.464101615137852974, 5.999999999999884537, -101.8363248654052029 ) ) ;
#7724=CARTESIAN_POINT ( 'NONE',  ( 3.464101615137852974, 5.999999999999884537, -67.33632486540523132 ) ) ;
#7725=CARTESIAN_POINT ( 'NONE',  ( -3.175426480542816066, 5.499999999999865885, -68.87500000000002842 ) ) ;
#7726=CARTESIAN_POINT ( 'NONE',  ( 0.000000000000000000, 5.499999999999991118, -54.00000000000004974 ) ) ;
#7729=DIRECTION ( 'NONE',  ( 7.147005652999508048E-36, -5.642372883946980038E-36, -1.000000000000000000 ) ) ;
#7731=CYLINDRICAL_SURFACE ( 'NONE', #9686, 6.000000000000000888 ) ;
#7733=CARTESIAN_POINT ( 'NONE',  ( -5.999999999999963585, 1.780251999655701777E-13, -81.83632486540521711 ) ) ;
#7734=ORIENTED_EDGE ( 'NONE', *, *, #30129, .F. ) ;
#7738=CARTESIAN_POINT ( 'NONE',  ( 3.464101615137852974, 5.999999999999884537, -64.33632486540521711 ) ) ;
#7739=CARTESIAN_POINT ( 'NONE',  ( -2.775557561562891351E-14, -5.500000000000115463, -179.2500000000000284 ) ) ;
#7741=CARTESIAN_POINT ( 'NONE',  ( 2.775557561562891351E-14, -6.250000000000061284, -153.3169872981078186 ) ) ;
#7743=CARTESIAN_POINT ( 'NONE',  ( -4.763139720814407951, 2.749999999999946709, -79.25000000000004263 ) ) ;
#7744=ADVANCED_FACE ( 'NONE', ( #12811 ), #21708, .T. ) ;
#7745=CARTESIAN_POINT ( 'NONE',  ( -3.608439182435052128, -6.250000000000110134, -98.80801270189222407 ) ) ;
#7746=DIRECTION ( 'NONE',  ( 1.000000000000000000, -5.551115123125773458E-17, -1.260129944081490338E-35 ) ) ;
#7747=CARTESIAN_POINT ( 'NONE',  ( 5.380303083296117173, -9.596003543682449788, -22.31547897336681174 ) ) ;
#7749=CARTESIAN_POINT ( 'NONE',  ( -3.175426480542816066, 5.499999999999865885, -161.8750000000000000 ) ) ;
#7750=CARTESIAN_POINT ( 'NONE',  ( 5.999999999999999112, 2.951592740943527306E-14, -162.0863248654052029 ) ) ;
#7751=CARTESIAN_POINT ( 'NONE',  ( 3.175426480543072749, -5.500000000000105693, -150.6250000000000284 ) ) ;
#7752=CARTESIAN_POINT ( 'NONE',  ( 0.000000000000000000, 0.000000000000000000, 0.000000000000000000 ) ) ;
#7753=CARTESIAN_POINT ( 'NONE',  ( -4.763139720814407951, -2.750000000000016431, -97.00000000000002842 ) ) ;
#7755=CARTESIAN_POINT ( 'NONE',  ( 3.175426480543072749, 5.499999999999865885, -79.62500000000002842 ) ) ;
#7757=FACE_OUTER_BOUND ( 'NONE', #23337, .T. ) ;
#7760=CARTESIAN_POINT ( 'NONE',  ( 6.000000000000052403, -1.607695154586662678, -66.15331216351299304 ) ) ;
#7761=CARTESIAN_POINT ( 'NONE',  ( 6.000000000000000888, -3.330669073875464691E-16, -7.560779664488942560E-35 ) ) ;
#7762=ORIENTED_EDGE ( 'NONE', *, *, #19625, .T. ) ;
#7763=CARTESIAN_POINT ( 'NONE',  ( 0.000000000000000000, 5.999999999999977796, -91.21132486540523132 ) ) ;
#7764=CARTESIAN_POINT ( 'NONE',  ( -5.999999999999963585, 3.021315404115420679E-15, -178.4136751345947971 ) ) ;
#7769=ORIENTED_EDGE ( 'NONE', *, *, #22745, .T. ) ;
#7770=CARTESIAN_POINT ( 'NONE',  ( -3.175426480542816510, -5.500000000000057732, -107.3750000000000284 ) ) ;
#7773=CARTESIAN_POINT ( 'NONE',  ( 3.608439182435180470, 6.249999999999982236, -122.0580127018922667 ) ) ;
#7774=EDGE_CURVE ( 'NONE', #26402, #25744, #29959, .T. ) ;
#7775=ORIENTED_EDGE ( 'NONE', *, *, #8154, .T. ) ;
#7776=CARTESIAN_POINT ( 'NONE',  ( -5.999999999999963585, 1.780251999655701777E-13, -110.9136751345948255 ) ) ;
#7777=CARTESIAN_POINT ( 'NONE',  ( 3.608439182435180470, 6.249999999999982236, -158.6919872981078470 ) ) ;
#7779=CARTESIAN_POINT ( 'NONE',  ( -5.412658773652739619, 3.124999999999975131, -60.18301270189224539 ) ) ;
#7780=VERTEX_POINT ( 'NONE', #17716 ) ;
#7785=CARTESIAN_POINT ( 'NONE',  ( 0.000000000000000000, 5.499999999999991118, -171.0000000000000284 ) ) ;
#7787=CARTESIAN_POINT ( 'NONE',  ( 3.464101615137757051, -5.999999999999979572, -112.8363248654051887 ) ) ;
#7788=CARTESIAN_POINT ( 'NONE',  ( -5.412658773652684552, -3.125000000000099920, -166.4330127018922667 ) ) ;
#7791=CARTESIAN_POINT ( 'NONE',  ( -3.175426480542816066, -5.500000000000057732, -116.3749999999999858 ) ) ;
#7792=CARTESIAN_POINT ( 'NONE',  ( 3.175426480543072749, 5.499999999999865885, -114.1249999999999858 ) ) ;
#7796=EDGE_LOOP ( 'NONE', ( #14786, #13575, #4800, #25046 ) ) ;
#7798=CARTESIAN_POINT ( 'NONE',  ( 0.000000000000000000, 5.999999999999977796, -168.2886751345948255 ) ) ;
#7799=CARTESIAN_POINT ( 'NONE',  ( 5.196152422706629359, -2.999999999999988898, -145.7113248654052313 ) ) ;
#7801=CARTESIAN_POINT ( 'NONE',  ( 6.350852961086080661, -9.614813431917819062E-14, -178.8750000000000284 ) ) ;
#7802=CARTESIAN_POINT ( 'NONE',  ( 2.775557561562891351E-14, 6.250000000000033751, -79.06698729810779014 ) ) ;
#7804=CARTESIAN_POINT ( 'NONE',  ( -3.464101615137725076, 5.999999999999979572, -109.6636751345947971 ) ) ;
#7806=CARTESIAN_POINT ( 'NONE',  ( -5.999999999999971578, 1.607695154586715303, -143.9806624327026441 ) ) ;
#7807=ADVANCED_FACE ( 'NONE', ( #3692 ), #2018, .T. ) ;
#7809=ORIENTED_EDGE ( 'NONE', *, *, #27468, .F. ) ;
#7810=EDGE_LOOP ( 'NONE', ( #7232, #12925, #272, #16419 ) ) ;
#7814=ORIENTED_EDGE ( 'NONE', *, *, #4940, .T. ) ;
#7815=CARTESIAN_POINT ( 'NONE',  ( 2.775557561562891351E-14, 6.250000000000033751, -133.0669872981078470 ) ) ;
#7818=DIRECTION ( 'NONE',  ( -7.147005652999508048E-36, 5.642372883946980038E-36, 1.000000000000000000 ) ) ;
#7821=CARTESIAN_POINT ( 'NONE',  ( 3.464101615137852974, 5.999999999999884537, -135.4136751345947971 ) ) ;
#7822=CARTESIAN_POINT ( 'NONE',  ( -3.464101615137757051, -5.999999999999979572, -139.1636751345948824 ) ) ;
#7826=CARTESIAN_POINT ( 'NONE',  ( 0.000000000000000000, -5.999999999999991118, -162.4613248654052029 ) ) ;
#7827=CARTESIAN_POINT ( 'NONE',  ( -5.196152422706573404, -3.000000000000002665, -128.7886751345947971 ) ) ;
#7829=CARTESIAN_POINT ( 'NONE',  ( 6.000000000000000888, 1.743066579297358182E-13, -64.58632486540520290 ) ) ;
#7830=AXIS2_PLACEMENT_3D ( 'NONE', #28039, #19016, #12118 ) ;
#7831=CARTESIAN_POINT ( 'NONE',  ( -2.775557561562891351E-14, -5.500000000000115463, -137.2499999999999716 ) ) ;
#7837=AXIS2_PLACEMENT_3D ( 'NONE', #25025, #8768, #30099 ) ;
#7838=CARTESIAN_POINT ( 'NONE',  ( -3.175426480542816066, 5.499999999999865885, -49.37500000000000711 ) ) ;
#7839=CARTESIAN_POINT ( 'NONE',  ( 5.999999999999949374, 1.607695154586804565, -97.51933756729746960 ) ) ;
#7841=ORIENTED_EDGE ( 'NONE', *, *, #26025, .F. ) ;
#7843=CARTESIAN_POINT ( 'NONE',  ( -3.608439182435052128, -6.250000000000110134, -97.94198729810780435 ) ) ;
#7844=EDGE_CURVE ( 'NONE', #17914, #18017, #27194, .T. ) ;
#7845=FACE_OUTER_BOUND ( 'NONE', #22499, .T. ) ;
#7851=ORIENTED_EDGE ( 'NONE', *, *, #21840, .F. ) ;
#7852=DIRECTION ( 'NONE',  ( -7.147005652999508048E-36, 5.642372883946980038E-36, 1.000000000000000000 ) ) ;
#7853=AXIS2_PLACEMENT_3D ( 'NONE', #4081, #11508, #27120 ) ;
#7854=( BOUNDED_CURVE ( )  B_SPLINE_CURVE ( 2, ( #5102, #11939, #21867, #19272, #19566, #26452, #16978, #2807, #4813 ),
 .UNSPECIFIED., .F., .T. ) 
 B_SPLINE_CURVE_WITH_KNOTS ( ( 3, 2, 2, 2, 3 ),
 ( 0.1083333333333333925, 0.1092592592592592782, 0.1111111111111111605, 0.1129629629629629317, 0.1138888888888888173 ),
 .UNSPECIFIED. ) 
 CURVE ( )  GEOMETRIC_REPRESENTATION_ITEM ( )  RATIONAL_B_SPLINE_CURVE ( ( 0.9330127018922194093, 0.9330127018922234061, 1.000000000000000000, 0.8660254037844388186, 1.000000000000000000, 0.8660254037844388186, 1.000000000000000000, 0.9330127018922234061, 0.9330127018922194093 ) ) 
 REPRESENTATION_ITEM ( '' )  );
#7855=VERTEX_POINT ( 'NONE', #13577 ) ;
#7857=CARTESIAN_POINT ( 'NONE',  ( -3.175426480542816510, 5.499999999999865885, -55.37500000000004263 ) ) ;
#7858=CARTESIAN_POINT ( 'NONE',  ( -5.196152422706601826, 2.999999999999975131, -69.03867513459482552 ) ) ;
#7859=CARTESIAN_POINT ( 'NONE',  ( 6.000000000000026645, -1.607695154586707753, -134.2306624327025872 ) ) ;
#7860=CARTESIAN_POINT ( 'NONE',  ( 1.965048709171757446, 10.82948053518397025, -19.31713205297535652 ) ) ;
#7861=CARTESIAN_POINT ( 'NONE',  ( 7.216878364870455975, -6.409875621278545621E-14, -72.80801270189222407 ) ) ;
#7863=CARTESIAN_POINT ( 'NONE',  ( 3.464101615137852974, 5.999999999999884537, -169.3363248654052029 ) ) ;
#7866=CARTESIAN_POINT ( 'NONE',  ( 4.763139720814407951, -2.749999999999988454, -138.5000000000000000 ) ) ;
#7867=CARTESIAN_POINT ( 'NONE',  ( -5.196152422706573404, -3.000000000000002665, -177.7113248654052029 ) ) ;
#7868=CARTESIAN_POINT ( 'NONE',  ( 5.412658773652739619, 3.124999999999988898, -152.1830127018922667 ) ) ;
#7869=CARTESIAN_POINT ( 'NONE',  ( 6.000000000000000888, 1.743066579297358182E-13, -70.58632486540523132 ) ) ;
#7871=CARTESIAN_POINT ( 'NONE',  ( -3.175426480542816066, -5.500000000000057732, -72.87500000000000000 ) ) ;
#7872=CARTESIAN_POINT ( 'NONE',  ( -3.464101615137725076, 5.999999999999979572, -85.66367513459481131 ) ) ;
#7873=CARTESIAN_POINT ( 'NONE',  ( -4.763139720814407951, -2.750000000000016431, -56.49999999999999289 ) ) ;
#7875=ORIENTED_EDGE ( 'NONE', *, *, #127, .T. ) ;
#7878=CARTESIAN_POINT ( 'NONE',  ( -3.464101615137725076, 5.999999999999979572, -97.66367513459481131 ) ) ;
#7883=ORIENTED_EDGE ( 'NONE', *, *, #14386, .T. ) ;
#7885=CARTESIAN_POINT ( 'NONE',  ( -5.196152422706573404, -3.000000000000002665, -122.2113248654052029 ) ) ;
#7886=CARTESIAN_POINT ( 'NONE',  ( 0.000000000000000000, -5.999999999999991118, -102.4613248654052171 ) ) ;
#7887=CARTESIAN_POINT ( 'NONE',  ( 0.000000000000000000, 5.499999999999991118, -180.0000000000000568 ) ) ;
#7889=CARTESIAN_POINT ( 'NONE',  ( -5.412658773652739619, 3.124999999999975131, -149.3169872981078186 ) ) ;
#7891=CARTESIAN_POINT ( 'NONE',  ( -3.175426480542816510, -5.500000000000057732, -83.37500000000004263 ) ) ;
#7892=MECHANICAL_DESIGN_GEOMETRIC_PRESENTATION_REPRESENTATION('',(#9878),#9390);
#7893=CARTESIAN_POINT ( 'NONE',  ( -3.608439182435052128, -6.250000000000110134, -94.30801270189219565 ) ) ;
#7895=CARTESIAN_POINT ( 'NONE',  ( 3.464101615137757051, -5.999999999999979572, -127.8363248654051887 ) ) ;
#7897=CARTESIAN_POINT ( 'NONE',  ( 3.973952007372695494, -10.26128916632342047, -20.48836482813348070 ) ) ;
#7898=CARTESIAN_POINT ( 'NONE',  ( 5.196152422706629359, -2.999999999999988898, -58.71132486540520290 ) ) ;
#7900=CARTESIAN_POINT ( 'NONE',  ( -4.763139720814407951, 2.749999999999946709, -167.7500000000000000 ) ) ;
#7902=CARTESIAN_POINT ( 'NONE',  ( -4.763139720814407951, -2.750000000000016431, -145.0000000000000284 ) ) ;
#7903=CARTESIAN_POINT ( 'NONE',  ( 0.000000000000000000, -5.999999999999991118, -52.03867513459481131 ) ) ;
#7904=ADVANCED_FACE ( 'NONE', ( #22462 ), #1398, .T. ) ;
#7905=CARTESIAN_POINT ( 'NONE',  ( 6.350852961086080661, -9.614813431917819062E-14, -96.37499999999997158 ) ) ;
#7907=CARTESIAN_POINT ( 'NONE',  ( -3.175426480542816510, -5.500000000000057732, -80.37500000000002842 ) ) ;
#7910=CARTESIAN_POINT ( 'NONE',  ( 6.000000000000000888, 1.743066579297358182E-13, -108.0863248654051745 ) ) ;
#7911=CARTESIAN_POINT ( 'NONE',  ( 5.196152422706629359, -2.999999999999988898, -165.2113248654052313 ) ) ;
#7913=CARTESIAN_POINT ( 'NONE',  ( -5.999999999999963585, 1.780251999655701777E-13, -68.91367513459482552 ) ) ;
#7914=LINE ( 'NONE', #17175, #733 ) ;
#7918=PRESENTATION_STYLE_ASSIGNMENT (( #2863 ) ) ;
#7920=ORIENTED_EDGE ( 'NONE', *, *, #1965, .F. ) ;
#7921=ORIENTED_EDGE ( 'NONE', *, *, #4341, .F. ) ;
#7924=ORIENTED_EDGE ( 'NONE', *, *, #4741, .T. ) ;
#7926=CARTESIAN_POINT ( 'NONE',  ( -4.763139720814407951, -2.750000000000016431, -106.0000000000000426 ) ) ;
#7928=CARTESIAN_POINT ( 'NONE',  ( 3.608439182435180470, -6.249999999999997335, -121.0580127018922667 ) ) ;
#7930=CARTESIAN_POINT ( 'NONE',  ( -5.999999999999963585, 1.780251999655701777E-13, -68.91367513459482552 ) ) ;
#7931=CARTESIAN_POINT ( 'NONE',  ( -5.412658773652684552, -3.125000000000099920, -164.0669872981078186 ) ) ;
#7934=AXIS2_PLACEMENT_3D ( 'NONE', #4478, #20933, #18 ) ;
#7935=CARTESIAN_POINT ( 'NONE',  ( 2.775557561562891351E-14, 6.250000000000033751, -61.93301270189222407 ) ) ;
#7937=CARTESIAN_POINT ( 'NONE',  ( 3.464101615137852974, 5.999999999999884537, -117.4136751345948255 ) ) ;
#7940=CARTESIAN_POINT ( 'NONE',  ( -5.682342569962861134, 9.420267146893170462, -26.96534570410892684 ) ) ;
#7942=CARTESIAN_POINT ( 'NONE',  ( 6.350852961086080661, -9.614813431917819062E-14, -171.3750000000000000 ) ) ;
#7945=CARTESIAN_POINT ( 'NONE',  ( 3.608439182435180470, -6.249999999999997335, -170.5580127018922383 ) ) ;
#7946=CARTESIAN_POINT ( 'NONE',  ( 0.000000000000000000, 0.000000000000000000, 0.000000000000000000 ) ) ;
#7947=EDGE_CURVE ( 'NONE', #448, #10456, #15732, .T. ) ;
#7949=CARTESIAN_POINT ( 'NONE',  ( -4.763139720814407951, -2.750000000000016431, -113.5000000000000426 ) ) ;
#7950=CARTESIAN_POINT ( 'NONE',  ( -3.175426480542816510, 5.499999999999865885, -107.8750000000000284 ) ) ;
#7952=LINE ( 'NONE', #14749, #19451 ) ;
#7953=ORIENTED_EDGE ( 'NONE', *, *, #29948, .T. ) ;
#7960=CARTESIAN_POINT ( 'NONE',  ( -3.608439182435115633, 6.249999999999965361, -78.94198729810779014 ) ) ;
#7961=CARTESIAN_POINT ( 'NONE',  ( -5.196152422706601826, 2.999999999999975131, -109.5386751345948113 ) ) ;
#7962=ORIENTED_EDGE ( 'NONE', *, *, #6535, .F. ) ;
#7963=FACE_OUTER_BOUND ( 'NONE', #11124, .T. ) ;
#7964=ORIENTED_EDGE ( 'NONE', *, *, #21438, .T. ) ;
#7968=CARTESIAN_POINT ( 'NONE',  ( -7.216878364870328078, 0.000000000000000000, -132.6919872981078470 ) ) ;
#7969=CARTESIAN_POINT ( 'NONE',  ( -3.464101615137757051, -5.999999999999979572, -135.5863248654051745 ) ) ;
#7970=CARTESIAN_POINT ( 'NONE',  ( -5.999999999999963585, -1.487416814333745711E-14, -167.9136751345948255 ) ) ;
#7971=DIRECTION ( 'NONE',  ( -7.147005652999508048E-36, 5.642372883946980038E-36, 1.000000000000000000 ) ) ;
#7976=DIRECTION ( 'NONE',  ( -7.147005652999508048E-36, 5.642372883946980038E-36, 1.000000000000000000 ) ) ;
#7978=DIRECTION ( 'NONE',  ( 1.000000000000000000, -5.551115123125773458E-17, -1.260129944081490338E-35 ) ) ;
#7980=CARTESIAN_POINT ( 'NONE',  ( -5.412658773652739619, 3.124999999999975131, -68.31698729810781856 ) ) ;
#7981=CARTESIAN_POINT ( 'NONE',  ( -5.412658773652739619, 3.124999999999975131, -53.31698729810785409 ) ) ;
#7983=CARTESIAN_POINT ( 'NONE',  ( 6.000000000000000888, -1.859271017917181981E-14, -63.66367513459483973 ) ) ;
#7985=EDGE_CURVE ( 'NONE', #9162, #25957, #29100, .T. ) ;
#7986=CARTESIAN_POINT ( 'NONE',  ( 5.196152422706629359, 3.000000000000002665, -74.96132486540524553 ) ) ;
#7987=CARTESIAN_POINT ( 'NONE',  ( 6.350852961086080661, -9.614813431917819062E-14, -126.3749999999999858 ) ) ;
#7989=ORIENTED_EDGE ( 'NONE', *, *, #27252, .F. ) ;
#7992=CARTESIAN_POINT ( 'NONE',  ( -5.999999999999963585, 8.134310703387671600E-14, -119.3363248654052455 ) ) ;
#7994=EDGE_CURVE ( 'NONE', #25957, #22536, #30297, .T. ) ;
#7995=DIRECTION ( 'NONE',  ( -7.147005652999508048E-36, 5.642372883946980038E-36, 1.000000000000000000 ) ) ;
#8001=CARTESIAN_POINT ( 'NONE',  ( 3.608439182435180470, -6.249999999999997335, -94.69198729810779014 ) ) ;
#8010=CARTESIAN_POINT ( 'NONE',  ( 6.350852961086080661, -9.614813431917819062E-14, -54.37500000000002842 ) ) ;
#8012=CARTESIAN_POINT ( 'NONE',  ( 6.000000000000000888, 1.743066579297358182E-13, -51.08632486540523132 ) ) ;
#8013=CARTESIAN_POINT ( 'NONE',  ( 3.608439182435180470, 6.249999999999982236, -78.55801270189225249 ) ) ;
#8016=FACE_OUTER_BOUND ( 'NONE', #18400, .T. ) ;
#8017=CARTESIAN_POINT ( 'NONE',  ( -5.196152422706573404, -3.000000000000002665, -152.7886751345948255 ) ) ;
#8020=CARTESIAN_POINT ( 'NONE',  ( 6.000000000000000888, -1.607695154586752384, -93.73066243270260145 ) ) ;
#8022=CARTESIAN_POINT ( 'NONE',  ( 4.763139720814407951, -2.749999999999988454, -129.5000000000000000 ) ) ;
#8023=CYLINDRICAL_SURFACE ( 'NONE', #26751, 6.000000000000000888 ) ;
#8024=CARTESIAN_POINT ( 'NONE',  ( -5.999999999999971578, 1.607695154586715303, -50.98066243270261566 ) ) ;
#8025=CARTESIAN_POINT ( 'NONE',  ( 4.763139720814407951, 2.750000000000002665, -73.75000000000004263 ) ) ;
#8026=CARTESIAN_POINT ( 'NONE',  ( 3.175426480543072749, 5.499999999999865885, -55.62500000000003553 ) ) ;
#8027=( BOUNDED_CURVE ( )  B_SPLINE_CURVE ( 2, ( #20861, #29748, #8879, #11520, #25278, #30056, #9027, #1647, #27892 ),
 .UNSPECIFIED., .F., .T. ) 
 B_SPLINE_CURVE_WITH_KNOTS ( ( 3, 2, 2, 2, 3 ),
 ( 0.4361111111111111160, 0.4370370370370370572, 0.4388888888888888840, 0.4407407407407407662, 0.4416666666666667074 ),
 .UNSPECIFIED. ) 
 CURVE ( )  GEOMETRIC_REPRESENTATION_ITEM ( )  RATIONAL_B_SPLINE_CURVE ( ( 0.9330127018922194093, 0.9330127018922194093, 1.000000000000000000, 0.8660254037844388186, 1.000000000000000000, 0.8660254037844388186, 1.000000000000000000, 0.9330127018922174109, 0.9330127018922194093 ) ) 
 REPRESENTATION_ITEM ( '' )  );
#8028=VERTEX_POINT ( 'NONE', #23819 ) ;
#8034=ORIENTED_EDGE ( 'NONE', *, *, #23620, .T. ) ;
#8037=CARTESIAN_POINT ( 'NONE',  ( -4.763139720814407951, -2.750000000000016431, -181.0000000000000568 ) ) ;
#8040=CARTESIAN_POINT ( 'NONE',  ( 5.412658773652712085, -3.125000000000086153, -145.5669872981077901 ) ) ;
#8041=CARTESIAN_POINT ( 'NONE',  ( -4.763139720814407951, -2.750000000000016431, -80.50000000000001421 ) ) ;
#8043=CARTESIAN_POINT ( 'NONE',  ( 5.412658773652712085, -3.125000000000086153, -98.43301270189225249 ) ) ;
#8047=CARTESIAN_POINT ( 'NONE',  ( -2.775557561562891351E-14, -5.500000000000115463, -161.2500000000000000 ) ) ;
#8048=CARTESIAN_POINT ( 'NONE',  ( 4.763139720814407951, -2.749999999999988454, -147.5000000000000284 ) ) ;
#8049=CARTESIAN_POINT ( 'NONE',  ( -6.000000000000000888, 1.067854986875958443E-15, 7.560779664488942560E-35 ) ) ;
#8050=CARTESIAN_POINT ( 'NONE',  ( -4.763139720814407951, -2.750000000000016431, -92.50000000000002842 ) ) ;
#8052=CARTESIAN_POINT ( 'NONE',  ( -6.350852961085760029, -1.281975124255709124E-13, -85.12499999999998579 ) ) ;
#8057=CARTESIAN_POINT ( 'NONE',  ( 6.000000000000052403, -1.607695154586662678, -165.1533121635129646 ) ) ;
#8059=CYLINDRICAL_SURFACE ( 'NONE', #20364, 6.000000000000000888 ) ;
#8062=DIRECTION ( 'NONE',  ( 1.000000000000000000, -5.551115123125773458E-17, -1.260129944081490338E-35 ) ) ;
#8067=EDGE_CURVE ( 'NONE', #18315, #19006, #2472, .T. ) ;
#8068=CARTESIAN_POINT ( 'NONE',  ( 6.350852961086080661, -9.614813431917819062E-14, -105.3750000000000142 ) ) ;
#8069=CARTESIAN_POINT ( 'NONE',  ( 5.412658773652739619, 3.124999999999988898, -119.1830127018922383 ) ) ;
#8070=EDGE_LOOP ( 'NONE', ( #9565, #26364, #7000, #18800 ) ) ;
#8071=CARTESIAN_POINT ( 'NONE',  ( 3.464101615137757051, -5.999999999999979572, -110.4136751345947971 ) ) ;
#8072=CARTESIAN_POINT ( 'NONE',  ( -3.608439182435115633, 6.249999999999965361, -156.9419872981077617 ) ) ;
#8073=LINE ( 'NONE', #3315, #9347 ) ;
#8076=AXIS2_PLACEMENT_3D ( 'NONE', #8735, #24991, #3490 ) ;
#8077=CARTESIAN_POINT ( 'NONE',  ( 3.608439182435180470, 6.249999999999982236, -51.55801270189225249 ) ) ;
#8080=CARTESIAN_POINT ( 'NONE',  ( -3.464101615137757051, -5.999999999999979572, -56.66367513459481131 ) ) ;
#8082=CARTESIAN_POINT ( 'NONE',  ( 3.464101615137852974, 5.999999999999884537, -136.3363248654052313 ) ) ;
#8084=CARTESIAN_POINT ( 'NONE',  ( -3.175426480542816510, -5.500000000000057732, -173.3750000000000284 ) ) ;
#8087=CARTESIAN_POINT ( 'NONE',  ( -7.216878364870328078, 0.000000000000000000, -165.0580127018922099 ) ) ;
#8090=CARTESIAN_POINT ( 'NONE',  ( 6.350852961086080661, -9.614813431917819062E-14, -115.8750000000000000 ) ) ;
#8092=CARTESIAN_POINT ( 'NONE',  ( 4.763139720814407951, -2.749999999999988454, -102.5000000000000284 ) ) ;
#8094=CARTESIAN_POINT ( 'NONE',  ( 3.464101615137852974, 5.999999999999884537, -118.3363248654052171 ) ) ;
#8097=DIRECTION ( 'NONE',  ( 1.000000000000000000, -5.551115123125773458E-17, -1.260129944081490338E-35 ) ) ;
#8098=CARTESIAN_POINT ( 'NONE',  ( 6.000000000000103917, -1.607695154586573416, -133.6533121635129362 ) ) ;
#8100=CARTESIAN_POINT ( 'NONE',  ( 0.000000000000000000, 5.499999999999991118, -162.0000000000000284 ) ) ;
#8102=CARTESIAN_POINT ( 'NONE',  ( -3.608439182435115633, 6.249999999999965361, -83.44198729810781856 ) ) ;
#8103=CARTESIAN_POINT ( 'NONE',  ( 0.000000000000000000, -5.999999999999991118, -97.03867513459485394 ) ) ;
#8108=( BOUNDED_CURVE ( )  B_SPLINE_CURVE ( 2, ( #14003, #7188, #21036, #7035, #4577, #2574, #14155, #11996, #16599 ),
 .UNSPECIFIED., .F., .T. ) 
 B_SPLINE_CURVE_WITH_KNOTS ( ( 3, 2, 2, 2, 3 ),
 ( 0.7027777777777777235, 0.7037037037037037202, 0.7055555555555554914, 0.7074074074074074847, 0.7083333333333333703 ),
 .UNSPECIFIED. ) 
 CURVE ( )  GEOMETRIC_REPRESENTATION_ITEM ( )  RATIONAL_B_SPLINE_CURVE ( ( 0.9330127018922194093, 0.9330127018922154125, 1.000000000000000000, 0.8660254037844388186, 1.000000000000000000, 0.8660254037844388186, 1.000000000000000000, 0.9330127018922194093, 0.9330127018922194093 ) ) 
 REPRESENTATION_ITEM ( '' )  );
#8109=CARTESIAN_POINT ( 'NONE',  ( -3.608439182435052128, -6.250000000000110134, -137.8080127018922667 ) ) ;
#8110=ORIENTED_EDGE ( 'NONE', *, *, #24910, .T. ) ;
#8111=CARTESIAN_POINT ( 'NONE',  ( -3.608439182435115633, 6.249999999999965361, -129.9419872981078470 ) ) ;
#8113=CARTESIAN_POINT ( 'NONE',  ( 4.763139720814407951, -2.749999999999988454, -173.0000000000000568 ) ) ;
#8115=CARTESIAN_POINT ( 'NONE',  ( -5.999999999999963585, 1.780251999655701777E-13, -83.33632486540520290 ) ) ;
#8116=CARTESIAN_POINT ( 'NONE',  ( 6.000000000000000888, -3.330669073875464691E-16, -7.560779664488942560E-35 ) ) ;
#8117=EDGE_LOOP ( 'NONE', ( #12057, #21223, #16111, #22849 ) ) ;
#8119=FACE_OUTER_BOUND ( 'NONE', #4153, .T. ) ;
#8120=EDGE_CURVE ( 'NONE', #20406, #13461, #2434, .T. ) ;
#8122=LINE ( 'NONE', #17237, #4400 ) ;
#8123=CARTESIAN_POINT ( 'NONE',  ( -5.196152422706573404, -3.000000000000002665, -107.7886751345948397 ) ) ;
#8125=CARTESIAN_POINT ( 'NONE',  ( -3.608439182435115633, 6.249999999999965361, -68.44198729810779014 ) ) ;
#8126=CARTESIAN_POINT ( 'NONE',  ( 3.608439182435180470, -6.249999999999997335, -57.19198729810781145 ) ) ;
#8131=CARTESIAN_POINT ( 'NONE',  ( -4.763139720814407951, 2.749999999999946709, -127.2500000000000284 ) ) ;
#8135=LINE ( 'NONE', #12955, #29305 ) ;
#8141=CARTESIAN_POINT ( 'NONE',  ( 6.000000000000000888, -3.330669073875464691E-16, -7.560779664488942560E-35 ) ) ;
#8142=CARTESIAN_POINT ( 'NONE',  ( 2.775557561562891351E-14, -6.250000000000061284, -97.81698729810783277 ) ) ;
#8143=CARTESIAN_POINT ( 'NONE',  ( 6.000000000000000888, 1.743066579297358182E-13, -78.08632486540520290 ) ) ;
#8147=EDGE_CURVE ( 'NONE', #17914, #28360, #8108, .T. ) ;
#8150=CARTESIAN_POINT ( 'NONE',  ( -6.000000000000007105, -1.607695154586655129, -83.26933756729741276 ) ) ;
#8151=CARTESIAN_POINT ( 'NONE',  ( 3.175426480543072749, 5.499999999999865885, -51.12500000000002132 ) ) ;
#8153=CARTESIAN_POINT ( 'NONE',  ( -5.999999999999963585, -1.487416814333745711E-14, -59.91367513459483263 ) ) ;
#8154=EDGE_CURVE ( 'NONE', #21664, #14180, #4454, .T. ) ;
#8155=CARTESIAN_POINT ( 'NONE',  ( 3.608439182435180470, -6.249999999999997335, -76.05801270189223828 ) ) ;
#8158=CARTESIAN_POINT ( 'NONE',  ( -5.999999999999963585, -2.788906526875773208E-15, -176.9136751345948539 ) ) ;
#8159=CARTESIAN_POINT ( 'NONE',  ( -20.99177011976446394, -10.49588505988223197, -3.158490520261530689E-35 ) ) ;
#8161=CARTESIAN_POINT ( 'NONE',  ( -6.000000000000000888, 1.067854986875958443E-15, 7.560779664488942560E-35 ) ) ;
#8162=( BOUNDED_CURVE ( )  B_SPLINE_CURVE ( 2, ( #22781, #18043, #18494, #30135, #20468, #6939, #6486, #27358, #13907 ),
 .UNSPECIFIED., .F., .F. ) 
 B_SPLINE_CURVE_WITH_KNOTS ( ( 3, 2, 2, 2, 3 ),
 ( 0.8472222222222222099, 0.8481481481481480955, 0.8499999999999999778, 0.8518518518518518601, 0.8527777777777778567 ),
 .UNSPECIFIED. ) 
 CURVE ( )  GEOMETRIC_REPRESENTATION_ITEM ( )  RATIONAL_B_SPLINE_CURVE ( ( 0.9330127018922194093, 0.9330127018922194093, 1.000000000000000000, 0.8660254037844388186, 1.000000000000000000, 0.8660254037844388186, 1.000000000000000000, 0.9330127018922154125, 0.9330127018922194093 ) ) 
 REPRESENTATION_ITEM ( '' )  );
#8164=CARTESIAN_POINT ( 'NONE',  ( -4.763139720814407951, -2.750000000000016431, -130.0000000000000000 ) ) ;
#8166=CARTESIAN_POINT ( 'NONE',  ( -3.464101615137725076, 5.999999999999979572, -158.5863248654052313 ) ) ;
#8167=CARTESIAN_POINT ( 'NONE',  ( -6.000000000000023093, 1.607695154586625819, -177.9033121635129930 ) ) ;
#8168=CARTESIAN_POINT ( 'NONE',  ( 3.175426480543072749, -5.500000000000105693, -62.12500000000000711 ) ) ;
#8169=CARTESIAN_POINT ( 'NONE',  ( 4.763139720814407951, 2.750000000000002665, -58.75000000000002132 ) ) ;
#8170=CARTESIAN_POINT ( 'NONE',  ( -5.999999999999968026, -1.607695154586722186, -163.3466878364870070 ) ) ;
#8171=ORIENTED_EDGE ( 'NONE', *, *, #12886, .T. ) ;
#8175=CARTESIAN_POINT ( 'NONE',  ( 5.196152422706629359, -2.999999999999988898, -88.71132486540523132 ) ) ;
#8183=EDGE_CURVE ( 'NONE', #7068, #16950, #2229, .T. ) ;
#8185=CARTESIAN_POINT ( 'NONE',  ( -6.350852961085760029, -1.281975124255709124E-13, -145.1250000000000284 ) ) ;
#8186=CARTESIAN_POINT ( 'NONE',  ( 3.608439182435180470, 6.249999999999982236, -49.19198729810784698 ) ) ;
#8189=CARTESIAN_POINT ( 'NONE',  ( 3.608439182435180470, -6.249999999999997335, -144.1919872981078470 ) ) ;
#8190=CARTESIAN_POINT ( 'NONE',  ( 4.763139720814407951, -2.749999999999988454, -77.00000000000001421 ) ) ;
#8191=CARTESIAN_POINT ( 'NONE',  ( -3.608439182435052128, -6.250000000000110134, -91.30801270189225249 ) ) ;
#8192=CYLINDRICAL_SURFACE ( 'NONE', #29986, 6.000000000000000888 ) ;
#8194=CARTESIAN_POINT ( 'NONE',  ( 6.000000000000000888, 1.743066579297358182E-13, -90.66367513459483973 ) ) ;
#8197=( BOUNDED_CURVE ( )  B_SPLINE_CURVE ( 2, ( #2084, #28009, #9143, #2238, #20986, #25246, #21133, #30333, #9455 ),
 .UNSPECIFIED., .F., .F. ) 
 B_SPLINE_CURVE_WITH_KNOTS ( ( 3, 2, 2, 2, 3 ),
 ( 0.6916666666666666519, 0.6925925925925925375, 0.6944444444444444198, 0.6962962962962963021, 0.6972222222222222987 ),
 .UNSPECIFIED. ) 
 CURVE ( )  GEOMETRIC_REPRESENTATION_ITEM ( )  RATIONAL_B_SPLINE_CURVE ( ( 0.9330127018922194093, 0.9330127018922194093, 1.000000000000000000, 0.8660254037844388186, 1.000000000000000000, 0.8660254037844388186, 1.000000000000000000, 0.9330127018922154125, 0.9330127018922194093 ) ) 
 REPRESENTATION_ITEM ( '' )  );
#8198=CARTESIAN_POINT ( 'NONE',  ( -2.775557561562891351E-14, -5.500000000000115463, -156.7500000000000568 ) ) ;
#8199=CARTESIAN_POINT ( 'NONE',  ( 6.000000000000000888, -1.859271017917181981E-14, -126.6636751345948397 ) ) ;
#8200=CARTESIAN_POINT ( 'NONE',  ( 0.000000000000000000, 5.499999999999991118, -148.5000000000000284 ) ) ;
#8202=CARTESIAN_POINT ( 'NONE',  ( -4.763139720814407951, 2.749999999999946709, -85.25000000000004263 ) ) ;
#8203=LINE ( 'NONE', #17619, #8579 ) ;
#8204=CARTESIAN_POINT ( 'NONE',  ( -2.775557561562891351E-14, -5.500000000000115463, -81.74999999999998579 ) ) ;
#8207=CARTESIAN_POINT ( 'NONE',  ( -5.196152422706601826, 2.999999999999975131, -141.9613248654052597 ) ) ;
#8212=FACE_OUTER_BOUND ( 'NONE', #22682, .T. ) ;
#8214=DIRECTION ( 'NONE',  ( 1.000000000000000000, -5.551115123125773458E-17, -1.260129944081490338E-35 ) ) ;
#8215=ORIENTED_EDGE ( 'NONE', *, *, #13622, .F. ) ;
#8217=CARTESIAN_POINT ( 'NONE',  ( -5.999999999999963585, 1.780251999655701777E-13, -72.83632486540523132 ) ) ;
#8218=CARTESIAN_POINT ( 'NONE',  ( 5.999999999999949374, 1.607695154586804565, -81.01933756729741276 ) ) ;
#8222=EDGE_CURVE ( 'NONE', #7154, #24608, #2653, .T. ) ;
#8223=ORIENTED_EDGE ( 'NONE', *, *, #10770, .F. ) ;
#8224=CARTESIAN_POINT ( 'NONE',  ( -4.763139720814407951, 2.749999999999946709, -107.7500000000000142 ) ) ;
#8226=CARTESIAN_POINT ( 'NONE',  ( -3.608439182435115633, 6.249999999999965361, -114.3080127018922525 ) ) ;
#8228=DIRECTION ( 'NONE',  ( -7.147005652999508048E-36, 5.642372883946980038E-36, 1.000000000000000000 ) ) ;
#8229=CARTESIAN_POINT ( 'NONE',  ( 6.000000000000000888, 1.743066579297358182E-13, -78.66367513459483973 ) ) ;
#8230=LINE ( 'NONE', #22544, #24820 ) ;
#8231=CARTESIAN_POINT ( 'NONE',  ( -5.412658773652684552, -3.125000000000099920, -50.93301270189220986 ) ) ;
#8234=LINE ( 'NONE', #15185, #5472 ) ;
#8237=CARTESIAN_POINT ( 'NONE',  ( -3.175426480542816510, 5.499999999999865885, -170.8750000000000853 ) ) ;
#8239=CARTESIAN_POINT ( 'NONE',  ( 5.412658773652739619, 3.124999999999988898, -167.1830127018922383 ) ) ;
#8240=CARTESIAN_POINT ( 'NONE',  ( -5.196152422706601826, 2.999999999999975131, -48.03867513459481131 ) ) ;
#8241=CARTESIAN_POINT ( 'NONE',  ( 3.175426480543072749, -5.500000000000105693, -116.1250000000000000 ) ) ;
#8243=CARTESIAN_POINT ( 'NONE',  ( -3.175426480542816510, 5.499999999999865885, -101.8750000000000000 ) ) ;
#8244=CARTESIAN_POINT ( 'NONE',  ( 3.464101615137757051, -5.999999999999979572, -87.33632486540521711 ) ) ;
#8245=CARTESIAN_POINT ( 'NONE',  ( -5.999999999999957367, 1.607695154586737507, -161.9806624327025872 ) ) ;
#8249=CYLINDRICAL_SURFACE ( 'NONE', #16320, 6.000000000000000888 ) ;
#8253=CARTESIAN_POINT ( 'NONE',  ( 6.350852961086080661, -9.614813431917819062E-14, -160.8750000000000284 ) ) ;
#8254=CARTESIAN_POINT ( 'NONE',  ( 5.999999999999988454, 1.607695154586737729, -156.5966878364870638 ) ) ;
#8256=CARTESIAN_POINT ( 'NONE',  ( 7.216878364870455975, -6.409875621278545621E-14, -80.94198729810780435 ) ) ;
#8257=CARTESIAN_POINT ( 'NONE',  ( -5.196152422706573404, -3.000000000000002665, -103.2886751345948255 ) ) ;
#8258=ORIENTED_EDGE ( 'NONE', *, *, #21949, .F. ) ;
#8262=ORIENTED_EDGE ( 'NONE', *, *, #9151, .F. ) ;
#8264=CARTESIAN_POINT ( 'NONE',  ( 3.175426480543072749, -5.500000000000105693, -132.6250000000000000 ) ) ;
#8265=CARTESIAN_POINT ( 'NONE',  ( 3.608439182435180470, -6.249999999999997335, -142.0580127018922383 ) ) ;
#8267=CARTESIAN_POINT ( 'NONE',  ( 3.608439182435180470, 6.249999999999982236, -122.6919872981078043 ) ) ;
#8269=CARTESIAN_POINT ( 'NONE',  ( -3.175426480542816510, 5.499999999999865885, -173.8750000000000000 ) ) ;
#8270=CARTESIAN_POINT ( 'NONE',  ( 5.196152422706629359, 3.000000000000002665, -175.4613248654052313 ) ) ;
#8275=CARTESIAN_POINT ( 'NONE',  ( -3.464101615137725076, 5.999999999999979572, -163.6636751345947971 ) ) ;
#8276=CARTESIAN_POINT ( 'NONE',  ( 5.196152422706629359, 3.000000000000002665, -56.96132486540522422 ) ) ;
#8278=CARTESIAN_POINT ( 'NONE',  ( 3.464101615137852974, 5.999999999999884537, -171.4136751345948255 ) ) ;
#8279=CARTESIAN_POINT ( 'NONE',  ( 6.000000000000000888, 1.607695154586715303, -46.51933756729744118 ) ) ;
#8281=CARTESIAN_POINT ( 'NONE',  ( -7.216878364870328078, 0.000000000000000000, -65.19198729810777593 ) ) ;
#8282=CARTESIAN_POINT ( 'NONE',  ( -7.216878364870328078, 0.000000000000000000, -56.19198729810781145 ) ) ;
#8283=CARTESIAN_POINT ( 'NONE',  ( 3.464101615137757051, -5.999999999999979572, -170.4136751345948255 ) ) ;
#8284=DIRECTION ( 'NONE',  ( -7.147005652999508048E-36, 5.642372883946980038E-36, 1.000000000000000000 ) ) ;
#8287=CARTESIAN_POINT ( 'NONE',  ( 3.175426480543072749, -5.500000000000105693, -131.1250000000000000 ) ) ;
#8288=EDGE_CURVE ( 'NONE', #13246, #8435, #16079, .T. ) ;
#8289=ORIENTED_EDGE ( 'NONE', *, *, #11444, .T. ) ;
#8291=ADVANCED_FACE ( 'NONE', ( #26252 ), #7228, .T. ) ;
#8292=AXIS2_PLACEMENT_3D ( 'NONE', #133, #9199, #27761 ) ;
#8295=CARTESIAN_POINT ( 'NONE',  ( 0.000000000000000000, -5.999999999999991118, -161.5386751345948539 ) ) ;
#8296=( BOUNDED_CURVE ( )  B_SPLINE_CURVE ( 2, ( #21243, #9568, #478, #23844, #19101, #4492, #23407, #2200, #16665 ),
 .UNSPECIFIED., .F., .F. ) 
 B_SPLINE_CURVE_WITH_KNOTS ( ( 3, 2, 2, 2, 3 ),
 ( 0.1194444444444444642, 0.1203703703703703498, 0.1222222222222222321, 0.1240740740740741144, 0.1250000000000000000 ),
 .UNSPECIFIED. ) 
 CURVE ( )  GEOMETRIC_REPRESENTATION_ITEM ( )  RATIONAL_B_SPLINE_CURVE ( ( 0.9330127018922194093, 0.9330127018922234061, 1.000000000000000000, 0.8660254037844388186, 1.000000000000000000, 0.8660254037844388186, 1.000000000000000000, 0.9330127018922194093, 0.9330127018922194093 ) ) 
 REPRESENTATION_ITEM ( '' )  );
#8301=CARTESIAN_POINT ( 'NONE',  ( 5.412658773652712085, -3.125000000000086153, -115.5669872981078328 ) ) ;
#8304=( BOUNDED_CURVE ( )  B_SPLINE_CURVE ( 2, ( #26146, #4948, #21113, #2799, #48, #21412, #21564, #18819, #16973 ),
 .UNSPECIFIED., .F., .T. ) 
 B_SPLINE_CURVE_WITH_KNOTS ( ( 3, 2, 2, 2, 3 ),
 ( 0.2583333333333333037, 0.2592592592592593004, 0.2611111111111110716, 0.2629629629629629539, 0.2638888888888889506 ),
 .UNSPECIFIED. ) 
 CURVE ( )  GEOMETRIC_REPRESENTATION_ITEM ( )  RATIONAL_B_SPLINE_CURVE ( ( 0.9330127018922194093, 0.9330127018922154125, 1.000000000000000000, 0.8660254037844388186, 1.000000000000000000, 0.8660254037844388186, 1.000000000000000000, 0.9330127018922154125, 0.9330127018922194093 ) ) 
 REPRESENTATION_ITEM ( '' )  );
#8312=CARTESIAN_POINT ( 'NONE',  ( 3.175426480543072749, -5.500000000000105693, -51.62500000000001421 ) ) ;
#8313=VECTOR ( 'NONE', #774, 1000.000000000000000 ) ;
#8316=CARTESIAN_POINT ( 'NONE',  ( 5.412658773652712085, -3.125000000000086153, -72.93301270189222407 ) ) ;
#8319=CYLINDRICAL_SURFACE ( 'NONE', #8432, 6.000000000000000888 ) ;
#8320=CARTESIAN_POINT ( 'NONE',  ( 6.000000000000000888, 7.762456499804235646E-14, -118.5863248654052313 ) ) ;
#8324=CARTESIAN_POINT ( 'NONE',  ( -4.763139720814407951, -2.750000000000016431, -136.0000000000000000 ) ) ;
#8325=CARTESIAN_POINT ( 'NONE',  ( -5.999999999999963585, 1.780251999655701777E-13, -74.91367513459485394 ) ) ;
#8328=EDGE_CURVE ( 'NONE', #7517, #4859, #1670, .T. ) ;
#8329=CARTESIAN_POINT ( 'NONE',  ( -4.763139720814407951, -2.750000000000016431, -59.50000000000000000 ) ) ;
#8330=CARTESIAN_POINT ( 'NONE',  ( -4.763139720814407951, 2.749999999999946709, -55.25000000000002132 ) ) ;
#8332=ORIENTED_EDGE ( 'NONE', *, *, #4836, .T. ) ;
#8335=DIRECTION ( 'NONE',  ( -7.147005652999508048E-36, 5.642372883946980038E-36, 1.000000000000000000 ) ) ;
#8345=ORIENTED_EDGE ( 'NONE', *, *, #13078, .F. ) ;
#8346=CARTESIAN_POINT ( 'NONE',  ( 3.175426480543072749, -5.500000000000105693, -143.1250000000000000 ) ) ;
#8347=CARTESIAN_POINT ( 'NONE',  ( 5.412658773652739619, 3.124999999999988898, -47.81698729810779014 ) ) ;
#8350=CARTESIAN_POINT ( 'NONE',  ( -5.412658773652684552, -3.125000000000099920, -146.0669872981078470 ) ) ;
#8351=CARTESIAN_POINT ( 'NONE',  ( -2.775557561562891351E-14, -5.500000000000115463, -72.75000000000004263 ) ) ;
#8353=CARTESIAN_POINT ( 'NONE',  ( 2.775557561562891351E-14, 6.250000000000033751, -97.93301270189225249 ) ) ;
#8355=CARTESIAN_POINT ( 'NONE',  ( -3.175426480542816510, -5.500000000000057732, -152.3750000000000000 ) ) ;
#8356=CARTESIAN_POINT ( 'NONE',  ( -4.763867271839550277, -9.917884865257443394, -21.33175192690178079 ) ) ;
#8357=LINE ( 'NONE', #24188, #9325 ) ;
#8360=CARTESIAN_POINT ( 'NONE',  ( 3.464101615137757051, -5.999999999999979572, -90.91367513459485394 ) ) ;
#8361=DIRECTION ( 'NONE',  ( -7.147005652999508048E-36, 5.642372883946980038E-36, 1.000000000000000000 ) ) ;
#8363=CARTESIAN_POINT ( 'NONE',  ( 3.175426480543072749, -5.500000000000105693, -155.1249999999999716 ) ) ;
#8364=DIRECTION ( 'NONE',  ( 1.000000000000000000, -5.551115123125774074E-17, 0.000000000000000000 ) ) ;
#8365=CARTESIAN_POINT ( 'NONE',  ( -4.763139720814407951, -2.750000000000016431, -149.5000000000000284 ) ) ;
#8368=CARTESIAN_POINT ( 'NONE',  ( 3.175426480543072749, -5.500000000000105693, -87.62500000000000000 ) ) ;
#8369=CYLINDRICAL_SURFACE ( 'NONE', #28605, 6.000000000000000888 ) ;
#8370=CARTESIAN_POINT ( 'NONE',  ( 5.196152422706629359, -2.999999999999988898, -130.7113248654052597 ) ) ;
#8371=CARTESIAN_POINT ( 'NONE',  ( -4.763139720814407951, -2.750000000000016431, -80.50000000000001421 ) ) ;
#8372=CARTESIAN_POINT ( 'NONE',  ( 6.000000000000000888, -1.859271017917181981E-14, -120.0863248654052313 ) ) ;
#8374=CARTESIAN_POINT ( 'NONE',  ( -5.999999999999971578, 1.607695154586715303, -141.9033121635129930 ) ) ;
#8377=CARTESIAN_POINT ( 'NONE',  ( 6.000000000000000888, 1.607695154586715303, -125.0966878364870354 ) ) ;
#8379=ADVANCED_FACE ( 'NONE', ( #7963 ), #26835, .T. ) ;
#8381=ORIENTED_EDGE ( 'NONE', *, *, #12516, .T. ) ;
#8383=CARTESIAN_POINT ( 'NONE',  ( 6.000000000000000888, 1.743066579297358182E-13, -70.58632486540521711 ) ) ;
#8389=CARTESIAN_POINT ( 'NONE',  ( 6.350852961086080661, -9.614813431917819062E-14, -97.87499999999998579 ) ) ;
#8390=CARTESIAN_POINT ( 'NONE',  ( 5.999999999999949374, 1.607695154586804565, -71.09668783648703538 ) ) ;
#8391=( BOUNDED_CURVE ( )  B_SPLINE_CURVE ( 2, ( #17701, #26864, #17547, #21985, #19539, #10471, #1218, #15242, #29331 ),
 .UNSPECIFIED., .F., .F. ) 
 B_SPLINE_CURVE_WITH_KNOTS ( ( 3, 2, 2, 2, 3 ),
 ( 0.1083333333333333370, 0.1092592592592592643, 0.1111111111111111049, 0.1129629629629629595, 0.1138888888888888867 ),
 .UNSPECIFIED. ) 
 CURVE ( )  GEOMETRIC_REPRESENTATION_ITEM ( )  RATIONAL_B_SPLINE_CURVE ( ( 0.9330127018922194093, 0.9330127018922194093, 1.000000000000000000, 0.8660254037844388186, 1.000000000000000000, 0.8660254037844388186, 1.000000000000000000, 0.9330127018922194093, 0.9330127018922194093 ) ) 
 REPRESENTATION_ITEM ( '' )  );
#8392=CARTESIAN_POINT ( 'NONE',  ( 7.216878364870455975, -6.409875621278545621E-14, -114.8080127018922383 ) ) ;
#8393=ORIENTED_EDGE ( 'NONE', *, *, #7210, .F. ) ;
#8394=CARTESIAN_POINT ( 'NONE',  ( -5.196152422706601826, 2.999999999999975131, -93.96132486540520290 ) ) ;
#8396=VECTOR ( 'NONE', #22477, 1000.000000000000000 ) ;
#8397=CARTESIAN_POINT ( 'NONE',  ( 6.000000000000000888, 1.607695154586715303, -63.59668783648704959 ) ) ;
#8398=CARTESIAN_POINT ( 'NONE',  ( 3.608439182435180470, 6.249999999999982236, -54.55801270189220276 ) ) ;
#8401=CARTESIAN_POINT ( 'NONE',  ( -6.000000000000007105, -1.607695154586655129, -167.2693375672974128 ) ) ;
#8403=CARTESIAN_POINT ( 'NONE',  ( -3.175426480542816510, 5.499999999999865885, -172.3750000000000000 ) ) ;
#8405=CARTESIAN_POINT ( 'NONE',  ( -6.000000000000007105, -1.607695154586655129, -158.2693375672974128 ) ) ;
#8406=CARTESIAN_POINT ( 'NONE',  ( 2.775557561562891351E-14, -6.250000000000061284, -158.6830127018922099 ) ) ;
#8407=CARTESIAN_POINT ( 'NONE',  ( 6.000000000000000888, 1.743066579297358182E-13, -82.58632486540520290 ) ) ;
#8408=EDGE_CURVE ( 'NONE', #18931, #6372, #1354, .T. ) ;
#8409=CARTESIAN_POINT ( 'NONE',  ( -4.763139720814407951, -2.750000000000016431, -107.5000000000000426 ) ) ;
#8411=EDGE_CURVE ( 'NONE', #16120, #20574, #6121, .T. ) ;
#8412=CARTESIAN_POINT ( 'NONE',  ( -4.763139720814407951, 2.749999999999946709, -104.7500000000000142 ) ) ;
#8416=VECTOR ( 'NONE', #7656, 1000.000000000000000 ) ;
#8419=CARTESIAN_POINT ( 'NONE',  ( -6.000000000000007105, -1.607695154586655129, -90.76933756729744118 ) ) ;
#8421=CARTESIAN_POINT ( 'NONE',  ( 5.196152422706629359, -2.999999999999988898, -133.7113248654052029 ) ) ;
#8425=CARTESIAN_POINT ( 'NONE',  ( -7.216878364870328078, 0.000000000000000000, -81.69198729810780435 ) ) ;
#8426=CARTESIAN_POINT ( 'NONE',  ( 5.196152422706629359, -2.999999999999988898, -96.78867513459482552 ) ) ;
#8428=CARTESIAN_POINT ( 'NONE',  ( 6.000000000000000888, 7.762456499804234384E-14, -144.6636751345948255 ) ) ;
#8430=EDGE_LOOP ( 'NONE', ( #28534, #11001, #4269, #26823 ) ) ;
#8432=AXIS2_PLACEMENT_3D ( 'NONE', #3856, #17890, #15593 ) ;
#8433=CARTESIAN_POINT ( 'NONE',  ( -6.350852961085760029, -1.281975124255709124E-13, -121.1250000000000426 ) ) ;
#8434=CARTESIAN_POINT ( 'NONE',  ( 3.608439182435180470, 6.249999999999982236, -135.5580127018922667 ) ) ;
#8435=VERTEX_POINT ( 'NONE', #29455 ) ;
#8436=CARTESIAN_POINT ( 'NONE',  ( -3.608439182435115633, 6.249999999999965361, -126.9419872981078328 ) ) ;
#8438=CARTESIAN_POINT ( 'NONE',  ( -3.175426480542816510, -5.500000000000057732, -174.8750000000000284 ) ) ;
#8441=VERTEX_POINT ( 'NONE', #24402 ) ;
#8444=CARTESIAN_POINT ( 'NONE',  ( 6.000000000000000888, 7.762456499804234384E-14, -138.6636751345948255 ) ) ;
#8448=CARTESIAN_POINT ( 'NONE',  ( 3.608439182435180470, 6.249999999999982236, -67.19198729810780435 ) ) ;
#8450=CARTESIAN_POINT ( 'NONE',  ( 5.412658773652739619, 3.124999999999988898, -55.31698729810785409 ) ) ;
#8452=CARTESIAN_POINT ( 'NONE',  ( -3.464101615137757051, -5.999999999999979572, -128.6636751345948255 ) ) ;
#8454=CARTESIAN_POINT ( 'NONE',  ( 6.000000000000000888, 1.743066579297358182E-13, -75.08632486540521711 ) ) ;
#8455=EDGE_CURVE ( 'NONE', #15757, #24851, #9941, .T. ) ;
#8456=CARTESIAN_POINT ( 'NONE',  ( -6.350852961085760029, -1.281975124255709124E-13, -128.6250000000000000 ) ) ;
#8458=CARTESIAN_POINT ( 'NONE',  ( 0.000000000000000000, 5.999999999999977796, -157.7886751345948255 ) ) ;
#8459=CYLINDRICAL_SURFACE ( 'NONE', #11948, 6.000000000000000888 ) ;
#8462=EDGE_LOOP ( 'NONE', ( #18030, #19191, #23892, #1263 ) ) ;
#8464=CARTESIAN_POINT ( 'NONE',  ( 6.000000000000000888, -1.859271017917181981E-14, -72.08632486540521711 ) ) ;
#8466=CARTESIAN_POINT ( 'NONE',  ( -7.216878364870328078, 0.000000000000000000, -114.6919872981078328 ) ) ;
#8469=VERTEX_POINT ( 'NONE', #14905 ) ;
#8470=DIRECTION ( 'NONE',  ( -7.147005652999508048E-36, 5.642372883946980038E-36, 1.000000000000000000 ) ) ;
#8475=CARTESIAN_POINT ( 'NONE',  ( 6.350852961086080661, -9.614813431917819062E-14, -46.87500000000000000 ) ) ;
#8477=CARTESIAN_POINT ( 'NONE',  ( 7.216878364870455975, -6.409875621278545621E-14, -74.30801270189223828 ) ) ;
#8480=CARTESIAN_POINT ( 'NONE',  ( 6.000000000000000888, 1.743066579297358182E-13, -102.6636751345948397 ) ) ;
#8482=DIRECTION ( 'NONE',  ( -7.147005652999508048E-36, 5.642372883946980038E-36, 1.000000000000000000 ) ) ;
#8483=( BOUNDED_CURVE ( )  B_SPLINE_CURVE ( 2, ( #1525, #8598, #22593, #21978, #20285, #911, #29478, #26702, #5816 ),
 .UNSPECIFIED., .F., .F. ) 
 B_SPLINE_CURVE_WITH_KNOTS ( ( 3, 2, 2, 2, 3 ),
 ( 0.002777777777777767909, 0.003703703703703653538, 0.005555555555555535818, 0.007407407407407418098, 0.008333333333333414750 ),
 .UNSPECIFIED. ) 
 CURVE ( )  GEOMETRIC_REPRESENTATION_ITEM ( )  RATIONAL_B_SPLINE_CURVE ( ( 0.9330127018922194093, 0.9330127018922194093, 1.000000000000000000, 0.8660254037844388186, 1.000000000000000000, 0.8660254037844388186, 1.000000000000000000, 0.9330127018922154125, 0.9330127018922194093 ) ) 
 REPRESENTATION_ITEM ( '' )  );
#8484=ADVANCED_FACE ( 'NONE', ( #22264 ), #17371, .T. ) ;
#8485=CARTESIAN_POINT ( 'NONE',  ( -2.775557561562891351E-14, -5.500000000000115463, -131.2500000000000284 ) ) ;
#8487=FACE_OUTER_BOUND ( 'NONE', #16560, .T. ) ;
#8489=VERTEX_POINT ( 'NONE', #22113 ) ;
#8490=CARTESIAN_POINT ( 'NONE',  ( 3.175426480543072749, -5.500000000000105693, -59.12499999999999289 ) ) ;
#8491=CARTESIAN_POINT ( 'NONE',  ( -3.464101615137757051, -5.999999999999979572, -77.08632486540521711 ) ) ;
#8493=CARTESIAN_POINT ( 'NONE',  ( 6.000000000000052403, -1.607695154586662678, -174.1533121635130215 ) ) ;
#8494=EDGE_LOOP ( 'NONE', ( #4101, #30394, #13208, #17097 ) ) ;
#8497=CARTESIAN_POINT ( 'NONE',  ( -5.196152422706573404, -3.000000000000002665, -118.2886751345948397 ) ) ;
#8498=CARTESIAN_POINT ( 'NONE',  ( 5.196152422706629359, -2.999999999999988898, -48.78867513459483973 ) ) ;
#8503=CARTESIAN_POINT ( 'NONE',  ( 3.175426480543072749, -5.500000000000105693, -141.6250000000000000 ) ) ;
#8505=CARTESIAN_POINT ( 'NONE',  ( 2.775557561562891351E-14, 6.250000000000033751, -47.56698729810781856 ) ) ;
#8507=ORIENTED_EDGE ( 'NONE', *, *, #26909, .F. ) ;
#8509=CARTESIAN_POINT ( 'NONE',  ( 6.350852961086080661, -9.614813431917819062E-14, -75.37500000000000000 ) ) ;
#8518=CARTESIAN_POINT ( 'NONE',  ( 3.175426480543072749, -5.500000000000105693, -158.1250000000000284 ) ) ;
#8520=AXIS2_PLACEMENT_3D ( 'NONE', #17099, #21698, #10946 ) ;
#8521=FACE_OUTER_BOUND ( 'NONE', #19619, .T. ) ;
#8522=CARTESIAN_POINT ( 'NONE',  ( 0.000000000000000000, 5.499999999999991118, -90.00000000000002842 ) ) ;
#8523=CARTESIAN_POINT ( 'NONE',  ( -5.196152422706573404, -3.000000000000002665, -140.7886751345947971 ) ) ;
#8525=CARTESIAN_POINT ( 'NONE',  ( 0.000000000000000000, 5.499999999999991118, -73.50000000000001421 ) ) ;
#8526=DIRECTION ( 'NONE',  ( 1.000000000000000000, -5.551115123125773458E-17, -1.260129944081490338E-35 ) ) ;
#8529=CARTESIAN_POINT ( 'NONE',  ( 0.000000000000000000, -5.999999999999991118, -108.4613248654052171 ) ) ;
#8531=( BOUNDED_CURVE ( )  B_SPLINE_CURVE ( 2, ( #27169, #8597, #25017, #20426, #3358, #29320, #29476, #1374, #17691 ),
 .UNSPECIFIED., .F., .F. ) 
 B_SPLINE_CURVE_WITH_KNOTS ( ( 3, 2, 2, 2, 3 ),
 ( 0.9361111111111111160, 0.9370370370370370017, 0.9388888888888888840, 0.9407407407407407662, 0.9416666666666666519 ),
 .UNSPECIFIED. ) 
 CURVE ( )  GEOMETRIC_REPRESENTATION_ITEM ( )  RATIONAL_B_SPLINE_CURVE ( ( 0.9330127018922194093, 0.9330127018922194093, 1.000000000000000000, 0.8660254037844388186, 1.000000000000000000, 0.8660254037844388186, 1.000000000000000000, 0.9330127018922194093, 0.9330127018922194093 ) ) 
 REPRESENTATION_ITEM ( '' )  );
#8534=DIRECTION ( 'NONE',  ( -7.147005652999508048E-36, 5.642372883946980038E-36, 1.000000000000000000 ) ) ;
#8538=CARTESIAN_POINT ( 'NONE',  ( -5.999999999999963585, -1.487416814333745711E-14, -172.4136751345948255 ) ) ;
#8540=( BOUNDED_SURFACE ( )  B_SPLINE_SURFACE ( 1, 2, ( 
 ( #7053, #7205, #2728, #16616, #18756, #26088, #143, #21793, #14314, #19348, #12306, #28078, #14461, #9970, #16465, #18911, #28231, #21502, #21202, #17051, #14595, #2451, #23947, #25794, #28667, #3033, #28377, #429, #4744, #23794, #4884, #11862, #23508, #9818, #9524, #7357, #28523, #23655, #2591, #12010, #21345, #26230, #9670, #286, #19060, #16762, #12157, #19194, #16905, #5182, #2884, #21647, #583, #26525, #15033, #17649, #1026, #22091, #10577, #19776, #24683, #29124, #13060, #13216, #29432, #8084, #29277, #876, #27131, #21940, #3625, #22393, #5627, #8403, #3784, #17811, #1332, #22553, #24380, #6100, #15512, #7942, #10424, #12597, #7785, #8237, #19931, #10274, #24834, #26667, #17201, #10744, #15360, #3323, #17498, #26971, #20089, #19638, #5478, #5936, #12751, #26814, #3176, #24226, #10123, #19494, #14884, #5777, #15189, #28824, #28975, #17352, #24523, #3471, #12905, #22241, #1169, #30053, #4244, #8719, #1486, #13824, #6393, #23168, #22852, #4558, #11357, #20704, #9170, #18263, #27889, #20856, #11040, #9023, #18565, #18413, #13982, #27427, #30209, #6249, #29743, #4398, #20249, #20386, #15974, #18107, #10895, #8875, #13356, #25606, #15826, #2112, #25435, #29598, #27574, #11516, #8558, #1641, #25126, #13667, #3929, #6860, #27733, #15668, #6712, #17963, #16286, #27275, #11197, #23009, #24977, #6554, #22702, #4091, #13511, #25272, #16129, #1790, #1953, #20544, #29894, #18719, #5291, #247, #28343, #9935, #26343, #9630, #7461, #25900, #25754, #393, #4702, #5144, #23618, #23322, #28629, #19023, #18868, #2265, #26052, #11672, #14277, #23765, #21013, #19161, #7318, #14562, #28496, #544, #9783, #14428, #23475, #16430, #7600, #2848, #23906, #12268, #17014, #2552, #19309, #14136, #16728, #11979, #7165, #21613, #16872, #28043, #21307, #28189, #4995, #2696, #30360, #16580, #26193, #9327, #7013, #12121, #2412, #21462, #11824, #21163, #102, #9485, #4849, #21907, #702, #7751, #24194, #1137, #3287, #19459, #12415, #19740, #14994, #3589, #8365, #24484, #10706, #17775, #22356, #27095, #13020, #10086, #8200, #26481, #26632, #26777, #24333, #14700, #1292, #26933, #8048, #22052, #24047, #20050, #14850, #29087, #29236, #3139, #21759, #5590, #17461, #2994, #3434, #12713, #28940, #987, #28787, #29395, #5894, #17316, #7902, #17615, #17161, #841, #12561, #10241, #10388, #5743, #19600, #10538, #15152, #5440, #12866, #22204, #19892, #15321, #24644, #25237, #20822, #9134, #13785, #18526, #25399, #1911, #8987, #11318, #27693, #4360, #23129, #13183, #26572, #10168, #21693, #5226, #10315, #24265, #28003, #12343, #12499, #16391, #4520, #19241, #630, #27851, #17095, #26275, #11782, #9868, #13942, #5522, #19537, #61, #21123, #785, #17246, #14099, #25713, #4666, #28567, #23983, #6820, #28871, #7831, #10013, #5374, #14930, #14639, #12638, #21984, #23288, #16245, #2927, #19391, #916, #25559, #28716, #21837, #7536, #30324, #14783, #9285, #2230, #16947, #11631, #20976, #7687, #23435, #18680, #26423, #6973, #24128, #3075, #2378, #15564, #3674, #1533, #24881, #27330, #27179, #10790, #19823, #12795, #25027, #29640, #10943, #20292, #3981, #29329, #6295, #1079, #13110, #8287, #3522, #18013, #3830, #15081, #17700, #15241, #22446, #27027, #8605, #12952, #13259, #6149, #3366, #24732, #22600, #5991, #15718, #13404, #22750, #8456, #1382, #26863, #5672, #22137, #10469, #17394, #1692, #5823, #22289, #29168, #8131, #19680, #17861, #26708, #15408, #20140, #29022, #7987, #24422, #17546, #24573, #1216, #29487, #10627, #19978, #13873, #18312, #11089, #23366, #16024, #2310, #1998, #14177, #20906, #30250, #18763, #27780, #7059, #30403, #20592, #9219, #28084, #18610, #23514, #6602, #9371, #15875, #8922, #14026, #29793, #29942, #25481, #27624, #20434, #18459, #22899, #4750, #25323, #11711, #4597, #8769, #6756, #21055, #18156, #11244, #4298, #23214, #13559, #16472, #6905, #25173, #16327, #27469, #25801, #6446, #20752, #2160, #4138, #16176, #13716, #1843, #23057, #11562, #11407, #30101, #27931, #9066, #4448, #25647, #7364, #9978, #23803, #14469, #2893, #12164, #17059, #21510, #5336, #5487, #21801, #437, #21656, #23662, #19501, #14322, #26389, #14747, #28384, #748, #26535, #10134, #24091, #14891, #16771, #28833, #7792, #291, #2737, #4891, #149, #592, #12314, #2597, #17207, #19068, #9529, #3041, #7650, #26096, #9825, #19355, #12458, #2455, #11870, #12016, #28676, #21208, #18917, #28238, #5038, #7212, #16624, #9678, #25944, #21352, #19202, #16913, #28531, #7500, #26238, #5191, #14603, #23955, #24841, #17818, #6255, #19937, #15517, #24233, #24388, #3333, #26980, #26676, #13221, #20095, #7950, #29439, #21950, #3791, #22559, #3479, #5944, #20257, #10586, #12758, #17360, #1490, #15366, #10901, #12911, #3632, #22100, #884, #10282, #29133, #1339, #15199, #5784, #24690, #22248, #8412, #1177, #27138, #27281, #29603, #29284, #13069, #15042, #8563, #5636, #6107, #17968, #19784, #3183, #12607, #19645, #28984, #1034, #8092, #10434, #17507, #26820, #24531, #8243, #17655, #22402, #10751, #15833, #2271, #1797, #13363, #9175, #20862, #20549, #27579, #16134, #27894, #27432, #22708, #2117, #11203, #8880, #8725, #29749, #16290, #13829, #1649, #4250, #25280, #21017, #6866, #30212, #25610, #13520, #11047, #23014, #24982, #23175, #18417, #22858, #15674, #4563, #29901, #13987, #6560, #18723, #25440, #4404, #23327, #1959, #18268, #15979, #18114, #6399, #11676, #11521, #20391, #13672, #11364, #30366, #9333, #18572, #28048, #20709, #25132, #30057, #3933, #4097, #27738, #9028, #6718, #19316, #11983, #28637, #28348, #10094, #16878, #26198, #14708, #23767, #2999, #26348, #16586, #5150, #24052, #14565, #19464, #2559, #5296, #11832, #4857, #9940, #25760, #25907, #21470, #14283, #7019, #14434, #18874, #706, #21313, #7608, #551, #16436, #2701, #17020, #4707, #7171, #23625, #9788, #9492, #12419, #2855, #21168, #12274, #14141, #21763, #23480, #16732, #19166, #2417, #12127, #255, #110, #28197, #28500, #9638, #26056, #23912, #19030, #7324, #5001, #398, #21618, #7466, #10394, #29242, #8052, #13025, #17467, #1297, #1456, #17781, #26781, #17620, #19605, #15480, #10248, #22362, #10711, #24339, #27100, #22524, #6068, #20055, #10865, #12720, #24807, #3755, #26637, #19745, #847, #26488, #26940, #8204, #28944, #13188, #14999, #5444, #29401, #3596, #3293, #29091, #5901, #8371, #7907, #14854, #15328, #28793, #17320, #12870, #7755, #5596, #24198, #5746, #22210, #17167, #24649, #15158, #22058, #24490, #3144, #12568, #21913, #992, #3437, #1144, #10543, #19900, #18082, #8686, #22819, #15944, #2235, #11485, #2080, #4214, #27698, #30176, #6521, #20827, #4526, #15637, #20220, #27545, #25242, #6825, #23293, #13633, #4366, #1761, #22669, #6680, #1611, #9141, #20509, #29567, #25567, #22978, #15794, #8525, #1917, #17931, #11162, #20669, #27248, #16100, #11325, #18533, #25404, #27856, #13791, #30023, #20358, #13330, #13948, #16251, #6221, #24947, #3900, #29864, #11014, #29712, #8993, #8843, #4056, #27394, #23136, #6361, #18228, #25100, #18382, #13479, #12240, #25873, #26162, #19129, #25721, #16695, #7432, #28316, #16841, #2818, #14533, #361, #26017, #18834, #28008, #4669, #21129, #28462, #215, #16398, #9292, #4966, #11950, #511, #5267, #21430, #7573, #14674, #19281, #24018, #9905, #6981, #5113, #23441, #23584, #23734, #21275, #11637, #28603, #23873, #14399, #18991, #20983, #16553, #21579, #2522, #30331, #9752, #16988, #26311, #7292, #18686, #14104, #67, #2382, #11789, #9453, #28161, #7130, #4822, #14247, #9601, #2666, #12090, #21876, #17432, #815, #2964, #10355, #14824, #27065, #28908, #3561, #26902, #15448, #29060, #24610, #12384, #3110, #12534, #5712, #5412, #22327, #29208, #17133, #8169, #670, #12991, #1261, #12686, #15123, #29366, #19716, #10209, #26459, #10671, #24454, #20018, #22019, #12831, #19573, #10056, #19431, #7873, #10507, #24305, #14965, #3408, #954, #17585, #8026, #5865, #6029, #8330, #26746, #22175, #24168, #17741, #17286, #15283, #21731, #26608, #28757, #7726, #5562, #3254, #1109, #19862, #23209, #30246, #22747, #6443, #27327, #22597, #23053, #4293, #25023, #11557, #11086, #1530, #18455, #30097, #29790, #15872, #25318, #6752, #6290, #10940, #11401, #20431, #18152, #18010, #8603, #25477, #1993, #20288, #13554, #4135, #9214, #16173, #9062, #4444, #1688, #29637, #1839, #3827, #20747, #27622, #8766, #24877, #13869, #27464, #2155, #15713, #25170, #27776, #13257, #13401, #8918, #22897, #3978, #11241, #20589, #18605 ),
 ( #29938, #18308, #6597, #20902, #16020, #13712, #27927, #6900, #432, #4887, #19197, #19351, #5186, #25939, #5031, #7055, #2887, #28080, #9821, #28526, #11864, #14598, #9973, #23950, #7495, #28670, #145, #12308, #21651, #14172, #28233, #18759, #14020, #14464, #26091, #16467, #586, #2453, #23362, #16908, #21505, #21204, #7207, #16764, #26233, #25796, #2306, #2731, #9526, #18913, #9366, #30399, #16324, #23797, #11706, #14316, #23657, #25643, #4593, #21051, #4746, #23510, #16618, #2593, #12012, #12160, #19062, #21347, #288, #9672, #28379, #7359, #28978, #10747, #17501, #26816, #15362, #24383, #3628, #26974, #17204, #5779, #24686, #15193, #20091, #10428, #14887, #7645, #19934, #12601, #29280, #7945, #17054, #24525, #3474, #13064, #3326, #22396, #5939, #26528, #12907, #1335, #22244, #26384, #3179, #5331, #12453, #5481, #10580, #14741, #24228, #22094, #21943, #24085, #15036, #19497, #3036, #879, #8239, #1172, #21795, #12754, #17652, #743, #7788, #10277, #19779, #10127, #28827, #19640, #17355, #26670, #5630, #1029, #29127, #8087, #2231, #25869, #16246, #18377, #13626, #21124, #11632, #62, #18527, #9286, #27694, #6103, #15514, #4361, #6974, #20823, #11481, #30325, #9135, #14100, #27852, #2379, #2516, #18829, #6821, #18681, #20666, #16547, #11319, #23436, #11783, #25400, #28155, #23579, #7125, #9447, #11946, #13786, #4818, #14244, #6674, #30171, #1912, #27134, #28005, #16392, #30017, #29435, #16093, #24837, #8406, #4667, #23131, #25561, #25714, #17814, #8988, #4209, #22974, #2077, #4521, #13943, #23289, #20977, #19426, #28309, #9902, #506, #26604, #3105, #26456, #812, #19125, #7287, #28598, #210, #28753, #24163, #9597, #9749, #14669, #28456, #21269, #7566, #2661, #14961, #16836, #21872, #10203, #3249, #16984, #19569, #16690, #21424, #7428, #24016, #23728, #28903, #17130, #4960, #5407, #26012, #7868, #17282, #19277, #2961, #5558, #26307, #26157, #14392, #24302, #12379, #12084, #21726, #10048, #5109, #14530, #23869, #2811, #7722, #12236, #21576, #22482, #22322, #15599, #20012, #24913, #15754, #1572, #24769, #1418, #3405, #8642, #10504, #3862, #10980, #26898, #18047, #6326, #27360, #12679, #19712, #12987, #19858, #3711, #20177, #29529, #17894, #22784, #27820, #25524, #6488, #27967, #22939, #29830, #13910, #4487, #11284, #8959, #30140, #2194, #15914, #8806, #23256, #29982, #27664, #25210, #6644, #20941, #9253, #16064, #25366, #23097, #4634, #14065, #4019, #2042, #11449, #20793, #9102, #10450, #29620, #3809, #8265, #1060, #13385, #5967, #22728, #22422, #4117, #17990, #27306, #8748, #17840, #27448, #20412, #10603, #6274, #18134, #15694, #13539, #27003, #29772, #5803, #17679, #3654, #3503, #25005, #12933, #1671, #1361, #19804, #6420, #27159, #15388, #29149, #13238, #8109, #10771, #1511, #17528, #11066, #15542, #15855, #25154, #26841, #15220, #22582, #19957, #24551, #22269, #24711, #13090, #20119, #29462, #8434, #6129, #24861, #16312, #11540, #6735, #21189, #18748, #18290, #20883, #18440, #25634, #2140, #23498, #16154, #7045, #30387, #6581, #27910, #28069, #9197, #16457, #14161, #25784, #11697, #6888, #30080, #8900, #16004, #1978, #9355, #30234, #27604, #20573, #4582, #23194, #11851, #16607, #2293, #18902, #25928, #131, #4875, #9515, #25304, #4732, #4275, #4427, #14007, #18589, #22878, #28222, #2441, #23352, #21041, #1821, #7195, #23037, #11224, #29923, #11386, #13698, #13854, #20729, #9049, #27758, #25463, #28514, #26214, #21336, #21929, #26513, #16895, #7483, #17190, #3163, #417, #12146, #2720, #5170, #9959, #26654, #5464, #14872, #28657, #21783, #24215, #571, #12587, #28965, #9660, #14306, #21636, #19337, #862, #17338, #7628, #28812, #24070, #21491, #277, #19050, #19185, #726, #14583, #23935, #14727, #2872, #7773, #12292, #10262, #23646, #19623, #17038, #3020, #5018, #7928, #26077, #2579, #12002, #9806, #28366, #7346, #16751, #14449, #23784, #26370, #5318, #12437, #10111, #19480, #8069, #3311, #3774, #15502, #5766, #22692, #22228, #12738, #29588, #10885, #10563, #17639, #6088, #17954, #17487, #22078, #22540, #1159, #29266, #29111, #19764, #6238, #13206, #1012, #24670, #15351, #11030, #27266, #20240, #15658, #3459, #10413, #13049, #15023, #1474, #8392, #19920, #5615, #24965, #8226, #3919, #26962, #8709, #24827, #8548, #13348, #22381, #1630, #20376, #15175, #29731, #18099, #24366, #26801, #5923, #24510, #3614, #1320, #10732, #20078, #29421, #17799, #27117, #27415, #4386, #8866, #21150, #22998, #28031, #21005, #9474, #23159, #18708, #6382, #27564, #6543, #30200, #29884, #16422, #23313, #11187, #2257, #25116, #7002, #25743, #6700, #9161, #23465, #13813, #15964, #20535, #4690, #18555, #14125, #16119, #2401, #2100, #25262, #18249, #11813, #27880, #90, #25423, #6848, #4234, #4079, #13501, #1941, #4546, #18405, #9013, #16275, #11507, #11661, #20847, #30351, #15816, #22841, #25594, #13971, #13657, #1782, #11345, #9316, #20691, #30042, #27721, #21898, #14841, #21751, #16568, #21449, #17153, #3130, #16716, #9773, #21298, #14269, #17006, #28621, #19010, #23609, #14417, #2545, #690, #24038, #23754, #19150, #19299, #10075, #236, #9620, #2983, #7450, #26183, #28334, #26041, #28774, #26331, #5132, #14554, #23896, #2837, #7745, #534, #9925, #8043, #26623, #17607, #19592, #8353, #13010, #17453, #10231, #22509, #15143, #1443, #1129, #13317, #20041, #29387, #17919, #26923, #6206, #29554, #19731, #17761, #27235, #27085, #22658, #5733, #15625, #14985, #26767, #13172, #28929, #29079, #24633, #24474, #7893, #5884, #22040, #3885, #3424, #10851, #3738, #5581, #15309, #20204, #24325, #10376, #12854, #22348, #12704, #24935, #6052, #3278, #15467, #976, #10528, #19882, #29229, #1282, #8191, #24792, #3581, #10695, #1901, #14090, #25704, #18371, #11308, #1598, #4349, #29698, #20657, #11470, #6346, #25550, #25390, #13934, #11623, #27993, #20966, #30162, #1747, #4043, #15781, #30317, #13463, #22807, #11146, #30005, #20494, #29852, #13776, #12076, #7279, #21718, #19265, #18821, #21414, #28297, #16828, #2652, #24007, #16683, #7557, #496, #7115, #28446, #28591, #9738, #16974, #14662, #26298, #12228, #7421, #201, #9437, #16535, #2506, #9892, #347, #28147, #21115, #26149, #23718, #12369, #17121, #2801, #19417, #26447, #658, #5401, #10040, #25862, #5253, #4808, #4950, #5096, #19117, #23426, #28741, #2952, #14523, #23862, #2371, #7713, #23571, #21566, #11773, #11934, #50, #14382, #14236, #21261, #9588, #26004, #29048, #26735, #21862, #22470, #27050, #17421, #8013, #17725, #3701, #942, #12668, #22005, #5701, #10496, #27202, #6015, #15434, #29194, #22312, #24761, #19846, #13132, #29516, #10193, #14809, #22162, #8155, #1408, #17886, #17571, #29354, #15110, #12978, #10817, #3546, #24155, #10342, #20167, #19561, #19704, #8477, #3097, #24441, #26888, #3393, #12524, #5850, #26593, #806, #12819, #28896, #8316, #7861, #15268, #17273, #5549, #14954, #24294, #24596, #1245, #10654, #20003, #20317, #2029, #3854, #6781, #4475, #15901, #8948, #2183, #22927, #25053, #29665, #27806, #18339, #16201, #25200, #16053, #4012, #13285, #22628, #11113, #13741, #27501, #18183, #6631, #4163, #20781, #13588, #9091, #9240, #25511, #1869, #25354, #27354, #23241, #18038, #30128, #18487, #1717, #13901, #30282, #11586, #20930, #18634, #20461, #6177, #15590, #13428, #6479, #8634, #1564, #4323, #23087, #6317, #24905, #22773, #10969, #15743, #11435, #29820, #11271, #8797, #20624, #29970, #27655, #14879, #14591, #21642, #15, #11738, #28970, #26520, #4622, #17044, #7635, #3317, #10267, #3170, #7935, #26223, #23391, #5323, #6930, #5473, #735, #5176, #27955, #19632, #2879, #17346, #19343, #1019, #7779, #17196, #5621, #14734, #24373, #26660, #7086, #28113, #18791, #12744, #15028, #22084, #10418, #16353, #26376, #25672, #16501, #21788, #24078, #12300, #2338, #24221, #23942, #3027, #579, #10117, #12444, #9965, #28663, #12593, #21934, #19489, #28819, #870, #6094, #24970, #11035, #22697, #8552, #3780, #26966, #15181, #12899, #29271, #6243, #8398, #24517, #26806, #24830, #20083, #8714, #13506, #29594, #15821, #1785, #27421, #19770, #18103, #3464, #13354, #1164, #1324, #1480, #29427, #29118, #25121, #1635, #13210, #27122, #8077, #4085, #19924, #22545, #3925, #8231, #22234, #10738, #10890, #10571, #17960, #17805, #3618, #15507, #17643, #5929, #20380, #22388, #13055, #29738, #15354, #24677, #20244, #27271, #15665, #6852, #23614, #2407, #23469, #25600, #18712, #21157, #27884, #11818, #25895, #6549, #11192, #18559 ) ),
 .UNSPECIFIED., .F., .F., .F. ) 
 B_SPLINE_SURFACE_WITH_KNOTS ( ( 2, 2 ),
 ( 3, 2, 2, 2, 2, 2, 2, 2, 2, 2, 2, 2, 2, 2, 2, 2, 2, 2, 2, 2, 2, 2, 2, 2, 2, 2, 2, 2, 2, 2, 2, 2, 2, 2, 2, 2, 2, 2, 2, 2, 2, 2, 2, 2, 2, 2, 2, 2, 2, 2, 2, 2, 2, 2, 2, 2, 2, 2, 2, 2, 2, 2, 2, 2, 2, 2, 2, 2, 2, 2, 2, 2, 2, 2, 2, 2, 2, 2, 2, 2, 2, 2, 2, 2, 2, 2, 2, 2, 2, 2, 2, 2, 2, 2, 2, 2, 2, 2, 2, 2, 2, 2, 2, 2, 2, 2, 2, 2, 2, 2, 2, 2, 2, 2, 2, 2, 2, 2, 2, 2, 2, 2, 2, 2, 2, 2, 2, 2, 2, 2, 2, 2, 2, 2, 2, 2, 2, 2, 2, 2, 2, 2, 2, 2, 2, 2, 2, 2, 2, 2, 2, 2, 2, 2, 2, 2, 2, 2, 2, 2, 2, 2, 2, 2, 2, 2, 2, 2, 2, 2, 2, 2, 2, 2, 2, 2, 2, 2, 2, 2, 2, 2, 2, 2, 2, 2, 2, 2, 2, 2, 2, 2, 2, 2, 2, 2, 2, 2, 2, 2, 2, 2, 2, 2, 2, 2, 2, 2, 2, 2, 2, 2, 2, 2, 2, 2, 2, 2, 2, 2, 2, 2, 2, 2, 2, 2, 2, 2, 2, 2, 2, 2, 2, 2, 2, 2, 2, 2, 2, 2, 2, 2, 2, 2, 2, 2, 2, 2, 2, 2, 2, 2, 2, 2, 2, 2, 2, 2, 2, 2, 2, 2, 2, 2, 2, 2, 2, 2, 2, 2, 2, 2, 2, 2, 2, 2, 2, 2, 2, 2, 2, 2, 2, 2, 2, 2, 2, 2, 2, 2, 2, 2, 2, 2, 2, 2, 2, 2, 2, 2, 2, 2, 2, 2, 2, 2, 2, 2, 2, 2, 2, 2, 2, 2, 2, 2, 2, 2, 2, 2, 2, 2, 2, 2, 2, 2, 2, 2, 2, 2, 2, 2, 2, 2, 2, 2, 2, 2, 2, 2, 2, 2, 2, 2, 2, 2, 2, 2, 2, 2, 2, 2, 2, 2, 2, 2, 2, 2, 2, 2, 2, 2, 2, 2, 2, 2, 2, 2, 2, 2, 2, 2, 2, 2, 2, 2, 2, 2, 2, 2, 2, 2, 2, 2, 2, 2, 2, 2, 2, 2, 2, 2, 2, 2, 2, 2, 2, 2, 2, 2, 2, 2, 2, 2, 2, 2, 2, 2, 2, 2, 2, 2, 2, 2, 2, 2, 2, 2, 2, 2, 2, 2, 2, 2, 2, 2, 2, 2, 2, 2, 2, 2, 2, 2, 2, 2, 2, 2, 2, 2, 2, 2, 2, 2, 2, 2, 2, 2, 2, 2, 2, 2, 2, 2, 2, 2, 2, 2, 2, 2, 2, 2, 2, 2, 2, 2, 2, 2, 2, 2, 2, 2, 2, 2, 2, 2, 2, 2, 2, 2, 2, 2, 2, 2, 2, 2, 2, 2, 2, 2, 2, 2, 2, 2, 2, 2, 2, 2, 2, 2, 2, 2, 2, 2, 2, 2, 2, 2, 2, 2, 2, 2, 2, 2, 2, 2, 2, 2, 2, 2, 2, 2, 2, 2, 2, 2, 2, 2, 2, 2, 2, 2, 2, 2, 2, 2, 2, 2, 2, 2, 3 ),
 ( 0.000000000000000000, 1.000000000000000000 ),
 ( 0.000000000000000000, 0.001851851851851851923, 0.003703703703703703845, 0.005555555555555555768, 0.007407407407407407690, 0.009259259259259258745, 0.01111111111111111154, 0.01296296296296296259, 0.01481481481481481538, 0.01666666666666666644, 0.01851851851851851749, 0.02037037037037037202, 0.02222222222222222307, 0.02407407407407407413, 0.02592592592592592518, 0.02777777777777777624, 0.02962962962962963076, 0.03148148148148147835, 0.03333333333333333287, 0.03518518518518518740, 0.03703703703703703498, 0.03888888888888888951, 0.04074074074074074403, 0.04259259259259259162, 0.04444444444444444614, 0.04629629629629629373, 0.04814814814814814825, 0.05000000000000000278, 0.05185185185185185036, 0.05370370370370370489, 0.05555555555555555247, 0.05740740740740740700, 0.05925925925925926152, 0.06111111111111110911, 0.06296296296296295669, 0.06481481481481481122, 0.06666666666666666574, 0.06851851851851852027, 0.07037037037037037479, 0.07222222222222221544, 0.07407407407407406996, 0.07592592592592592449, 0.07777777777777777901, 0.07962962962962963354, 0.08148148148148148806, 0.08333333333333332871, 0.08518518518518518323, 0.08703703703703703776, 0.08888888888888889228, 0.09074074074074074681, 0.09259259259259258745, 0.09444444444444444198, 0.09629629629629629650, 0.09814814814814815103, 0.1000000000000000056, 0.1018518518518518462, 0.1037037037037037007, 0.1055555555555555552, 0.1074074074074074098, 0.1092592592592592643, 0.1111111111111111049, 0.1129629629629629595, 0.1148148148148148140, 0.1166666666666666685, 0.1185185185185185230, 0.1203703703703703637, 0.1222222222222222182, 0.1240740740740740727, 0.1259259259259259134, 0.1277777777777777679, 0.1296296296296296224, 0.1314814814814814770, 0.1333333333333333315, 0.1351851851851851860, 0.1370370370370370405, 0.1388888888888888951, 0.1407407407407407496, 0.1425925925925926041, 0.1444444444444444309, 0.1462962962962962854, 0.1481481481481481399, 0.1499999999999999944, 0.1518518518518518490, 0.1537037037037037035, 0.1555555555555555580, 0.1574074074074074125, 0.1592592592592592671, 0.1611111111111111216, 0.1629629629629629761, 0.1648148148148148029, 0.1666666666666666574, 0.1685185185185185119, 0.1703703703703703665, 0.1722222222222222210, 0.1740740740740740755, 0.1759259259259259300, 0.1777777777777777846, 0.1796296296296296391, 0.1814814814814814936, 0.1833333333333333204, 0.1851851851851851749, 0.1870370370370370294, 0.1888888888888888840, 0.1907407407407407385, 0.1925925925925925930, 0.1944444444444444475, 0.1962962962962963021, 0.1981481481481481566, 0.2000000000000000111, 0.2018518518518518656, 0.2037037037037036924, 0.2055555555555555469, 0.2074074074074074014, 0.2092592592592592560, 0.2111111111111111105, 0.2129629629629629650, 0.2148148148148148195, 0.2166666666666666741, 0.2185185185185185286, 0.2203703703703703831, 0.2222222222222222099, 0.2240740740740740644, 0.2259259259259259189, 0.2277777777777777735, 0.2296296296296296280, 0.2314814814814814825, 0.2333333333333333370, 0.2351851851851851916, 0.2370370370370370461, 0.2388888888888889006, 0.2407407407407407274, 0.2425925925925925819, 0.2444444444444444364, 0.2462962962962962910, 0.2481481481481481455, 0.2500000000000000000, 0.2518518518518518268, 0.2537037037037037090, 0.2555555555555555358, 0.2574074074074074181, 0.2592592592592592449, 0.2611111111111111271, 0.2629629629629629539, 0.2648148148148148362, 0.2666666666666666630, 0.2685185185185185452, 0.2703703703703703720, 0.2722222222222221988, 0.2740740740740740811, 0.2759259259259259078, 0.2777777777777777901, 0.2796296296296296169, 0.2814814814814814992, 0.2833333333333333259, 0.2851851851851852082, 0.2870370370370370350, 0.2888888888888888618, 0.2907407407407407440, 0.2925925925925925708, 0.2944444444444444531, 0.2962962962962962798, 0.2981481481481481621, 0.2999999999999999889, 0.3018518518518518712, 0.3037037037037036979, 0.3055555555555555802, 0.3074074074074074070, 0.3092592592592592338, 0.3111111111111111160, 0.3129629629629629428, 0.3148148148148148251, 0.3166666666666666519, 0.3185185185185185341, 0.3203703703703703609, 0.3222222222222222432, 0.3240740740740740700, 0.3259259259259259522, 0.3277777777777777790, 0.3296296296296296058, 0.3314814814814814881, 0.3333333333333333148, 0.3351851851851851971, 0.3370370370370370239, 0.3388888888888889062, 0.3407407407407407329, 0.3425925925925926152, 0.3444444444444444420, 0.3462962962962962687, 0.3481481481481481510, 0.3499999999999999778, 0.3518518518518518601, 0.3537037037037036868, 0.3555555555555555691, 0.3574074074074073959, 0.3592592592592592782, 0.3611111111111111049, 0.3629629629629629872, 0.3648148148148148140, 0.3666666666666666408, 0.3685185185185185230, 0.3703703703703703498, 0.3722222222222222321, 0.3740740740740740589, 0.3759259259259259411, 0.3777777777777777679, 0.3796296296296296502, 0.3814814814814814770, 0.3833333333333333592, 0.3851851851851851860, 0.3870370370370370128, 0.3888888888888888951, 0.3907407407407407218, 0.3925925925925926041, 0.3944444444444444309, 0.3962962962962963132, 0.3981481481481481399, 0.4000000000000000222, 0.4018518518518518490, 0.4037037037037037313, 0.4055555555555555580, 0.4074074074074073848, 0.4092592592592592671, 0.4111111111111110938, 0.4129629629629629761, 0.4148148148148148029, 0.4166666666666666852, 0.4185185185185185119, 0.4203703703703703942, 0.4222222222222222210, 0.4240740740740740478, 0.4259259259259259300, 0.4277777777777777568, 0.4296296296296296391, 0.4314814814814814659, 0.4333333333333333481, 0.4351851851851851749, 0.4370370370370370572, 0.4388888888888888840, 0.4407407407407407662, 0.4425925925925925930, 0.4444444444444444198, 0.4462962962962963021, 0.4481481481481481288, 0.4500000000000000111, 0.4518518518518518379, 0.4537037037037037202, 0.4555555555555555469, 0.4574074074074074292, 0.4592592592592592560, 0.4611111111111111382, 0.4629629629629629650, 0.4648148148148147918, 0.4666666666666666741, 0.4685185185185185008, 0.4703703703703703831, 0.4722222222222222099, 0.4740740740740740922, 0.4759259259259259189, 0.4777777777777778012, 0.4796296296296296280, 0.4814814814814814548, 0.4833333333333333370, 0.4851851851851851638, 0.4870370370370370461, 0.4888888888888888729, 0.4907407407407407551, 0.4925925925925925819, 0.4944444444444444642, 0.4962962962962962910, 0.4981481481481481732, 0.5000000000000000000, 0.5018518518518518823, 0.5037037037037036535, 0.5055555555555555358, 0.5074074074074074181, 0.5092592592592593004, 0.5111111111111110716, 0.5129629629629629539, 0.5148148148148148362, 0.5166666666666667185, 0.5185185185185184897, 0.5203703703703703720, 0.5222222222222222543, 0.5240740740740740256, 0.5259259259259259078, 0.5277777777777777901, 0.5296296296296296724, 0.5314814814814814437, 0.5333333333333333259, 0.5351851851851852082, 0.5370370370370370905, 0.5388888888888888618, 0.5407407407407407440, 0.5425925925925926263, 0.5444444444444443976, 0.5462962962962962798, 0.5481481481481481621, 0.5500000000000000444, 0.5518518518518518157, 0.5537037037037036979, 0.5555555555555555802, 0.5574074074074074625, 0.5592592592592592338, 0.5611111111111111160, 0.5629629629629629983, 0.5648148148148147696, 0.5666666666666666519, 0.5685185185185185341, 0.5703703703703704164, 0.5722222222222221877, 0.5740740740740740700, 0.5759259259259259522, 0.5777777777777777235, 0.5796296296296296058, 0.5814814814814814881, 0.5833333333333333703, 0.5851851851851851416, 0.5870370370370370239, 0.5888888888888889062, 0.5907407407407407884, 0.5925925925925925597, 0.5944444444444444420, 0.5962962962962963243, 0.5981481481481480955, 0.5999999999999999778, 0.6018518518518518601, 0.6037037037037037424, 0.6055555555555555136, 0.6074074074074073959, 0.6092592592592592782, 0.6111111111111111605, 0.6129629629629629317, 0.6148148148148148140, 0.6166666666666666963, 0.6185185185185184675, 0.6203703703703703498, 0.6222222222222222321, 0.6240740740740741144, 0.6259259259259258856, 0.6277777777777777679, 0.6296296296296296502, 0.6314814814814815325, 0.6333333333333333037, 0.6351851851851851860, 0.6370370370370370683, 0.6388888888888888395, 0.6407407407407407218, 0.6425925925925926041, 0.6444444444444444864, 0.6462962962962962576, 0.6481481481481481399, 0.6500000000000000222, 0.6518518518518519045, 0.6537037037037036757, 0.6555555555555555580, 0.6574074074074074403, 0.6592592592592592116, 0.6611111111111110938, 0.6629629629629629761, 0.6648148148148148584, 0.6666666666666666297, 0.6685185185185185119, 0.6703703703703703942, 0.6722222222222222765, 0.6740740740740740478, 0.6759259259259259300, 0.6777777777777778123, 0.6796296296296295836, 0.6814814814814814659, 0.6833333333333333481, 0.6851851851851852304, 0.6870370370370370017, 0.6888888888888888840, 0.6907407407407407662, 0.6925925925925925375, 0.6944444444444444198, 0.6962962962962963021, 0.6981481481481481843, 0.6999999999999999556, 0.7018518518518518379, 0.7037037037037037202, 0.7055555555555556024, 0.7074074074074073737, 0.7092592592592592560, 0.7111111111111111382, 0.7129629629629629095, 0.7148148148148147918, 0.7166666666666666741, 0.7185185185185185563, 0.7203703703703703276, 0.7222222222222222099, 0.7240740740740740922, 0.7259259259259259744, 0.7277777777777777457, 0.7296296296296296280, 0.7314814814814815103, 0.7333333333333332815, 0.7351851851851851638, 0.7370370370370370461, 0.7388888888888889284, 0.7407407407407406996, 0.7425925925925925819, 0.7444444444444444642, 0.7462962962962963465, 0.7481481481481481177, 0.7500000000000000000, 0.7518518518518518823, 0.7537037037037036535, 0.7555555555555555358, 0.7574074074074074181, 0.7592592592592593004, 0.7611111111111110716, 0.7629629629629629539, 0.7648148148148148362, 0.7666666666666667185, 0.7685185185185184897, 0.7703703703703703720, 0.7722222222222222543, 0.7740740740740740256, 0.7759259259259259078, 0.7777777777777777901, 0.7796296296296296724, 0.7814814814814814437, 0.7833333333333333259, 0.7851851851851852082, 0.7870370370370370905, 0.7888888888888888618, 0.7907407407407407440, 0.7925925925925926263, 0.7944444444444443976, 0.7962962962962962798, 0.7981481481481481621, 0.8000000000000000444, 0.8018518518518518157, 0.8037037037037036979, 0.8055555555555555802, 0.8074074074074074625, 0.8092592592592592338, 0.8111111111111111160, 0.8129629629629629983, 0.8148148148148147696, 0.8166666666666666519, 0.8185185185185185341, 0.8203703703703704164, 0.8222222222222221877, 0.8240740740740740700, 0.8259259259259259522, 0.8277777777777777235, 0.8296296296296296058, 0.8314814814814814881, 0.8333333333333333703, 0.8351851851851851416, 0.8370370370370370239, 0.8388888888888889062, 0.8407407407407407884, 0.8425925925925925597, 0.8444444444444444420, 0.8462962962962963243, 0.8481481481481480955, 0.8499999999999999778, 0.8518518518518518601, 0.8537037037037037424, 0.8555555555555555136, 0.8574074074074073959, 0.8592592592592592782, 0.8611111111111111605, 0.8629629629629629317, 0.8648148148148148140, 0.8666666666666666963, 0.8685185185185184675, 0.8703703703703703498, 0.8722222222222222321, 0.8740740740740741144, 0.8759259259259258856, 0.8777777777777777679, 0.8796296296296296502, 0.8814814814814815325, 0.8833333333333333037, 0.8851851851851851860, 0.8870370370370370683, 0.8888888888888888395, 0.8907407407407407218, 0.8925925925925926041, 0.8944444444444444864, 0.8962962962962962576, 0.8981481481481481399, 0.9000000000000000222, 0.9018518518518519045, 0.9037037037037036757, 0.9055555555555555580, 0.9074074074074074403, 0.9092592592592592116, 0.9111111111111110938, 0.9129629629629629761, 0.9148148148148148584, 0.9166666666666666297, 0.9185185185185185119, 0.9203703703703703942, 0.9222222222222222765, 0.9240740740740740478, 0.9259259259259259300, 0.9277777777777778123, 0.9296296296296295836, 0.9314814814814814659, 0.9333333333333333481, 0.9351851851851852304, 0.9370370370370370017, 0.9388888888888888840, 0.9407407407407407662, 0.9425925925925925375, 0.9444444444444444198, 0.9462962962962963021, 0.9481481481481481843, 0.9499999999999999556, 0.9518518518518518379, 0.9537037037037037202, 0.9555555555555556024, 0.9574074074074073737, 0.9592592592592592560, 0.9611111111111111382, 0.9629629629629629095, 0.9648148148148147918, 0.9666666666666666741, 0.9685185185185185563, 0.9703703703703703276, 0.9722222222222222099, 0.9740740740740740922, 0.9759259259259259744, 0.9777777777777777457, 0.9796296296296296280, 0.9814814814814815103, 0.9833333333333332815, 0.9851851851851851638, 0.9870370370370370461, 0.9888888888888889284, 0.9907407407407406996, 0.9925925925925925819, 0.9944444444444444642, 0.9962962962962963465, 0.9981481481481481177, 1.000000000000000000 ),
 .UNSPECIFIED. ) 
 GEOMETRIC_REPRESENTATION_ITEM ( )  RATIONAL_B_SPLINE_SURFACE ( (
 ( 1.000000000000000000, 0.8660254037844387076, 1.000000000000000000, 0.8660254037844387076, 1.000000000000000000, 0.8660254037844387076, 1.000000000000000000, 0.8660254037844387076, 1.000000000000000000, 0.8660254037844387076, 1.000000000000000000, 0.8660254037844387076, 1.000000000000000000, 0.8660254037844387076, 1.000000000000000000, 0.8660254037844387076, 1.000000000000000000, 0.8660254037844387076, 1.000000000000000000, 0.8660254037844387076, 1.000000000000000000, 0.8660254037844387076, 1.000000000000000000, 0.8660254037844387076, 1.000000000000000000, 0.8660254037844387076, 1.000000000000000000, 0.8660254037844387076, 1.000000000000000000, 0.8660254037844387076, 1.000000000000000000, 0.8660254037844387076, 1.000000000000000000, 0.8660254037844387076, 1.000000000000000000, 0.8660254037844387076, 1.000000000000000000, 0.8660254037844387076, 1.000000000000000000, 0.8660254037844387076, 1.000000000000000000, 0.8660254037844387076, 1.000000000000000000, 0.8660254037844387076, 1.000000000000000000, 0.8660254037844387076, 1.000000000000000000, 0.8660254037844387076, 1.000000000000000000, 0.8660254037844387076, 1.000000000000000000, 0.8660254037844387076, 1.000000000000000000, 0.8660254037844387076, 1.000000000000000000, 0.8660254037844387076, 1.000000000000000000, 0.8660254037844387076, 1.000000000000000000, 0.8660254037844387076, 1.000000000000000000, 0.8660254037844387076, 1.000000000000000000, 0.8660254037844387076, 1.000000000000000000, 0.8660254037844387076, 1.000000000000000000, 0.8660254037844387076, 1.000000000000000000, 0.8660254037844387076, 1.000000000000000000, 0.8660254037844387076, 1.000000000000000000, 0.8660254037844387076, 1.000000000000000000, 0.8660254037844387076, 1.000000000000000000, 0.8660254037844387076, 1.000000000000000000, 0.8660254037844387076, 1.000000000000000000, 0.8660254037844387076, 1.000000000000000000, 0.8660254037844387076, 1.000000000000000000, 0.8660254037844387076, 1.000000000000000000, 0.8660254037844387076, 1.000000000000000000, 0.8660254037844387076, 1.000000000000000000, 0.8660254037844387076, 1.000000000000000000, 0.8660254037844387076, 1.000000000000000000, 0.8660254037844387076, 1.000000000000000000, 0.8660254037844387076, 1.000000000000000000, 0.8660254037844387076, 1.000000000000000000, 0.8660254037844387076, 1.000000000000000000, 0.8660254037844387076, 1.000000000000000000, 0.8660254037844387076, 1.000000000000000000, 0.8660254037844387076, 1.000000000000000000, 0.8660254037844387076, 1.000000000000000000, 0.8660254037844387076, 1.000000000000000000, 0.8660254037844387076, 1.000000000000000000, 0.8660254037844387076, 1.000000000000000000, 0.8660254037844387076, 1.000000000000000000, 0.8660254037844387076, 1.000000000000000000, 0.8660254037844387076, 1.000000000000000000, 0.8660254037844387076, 1.000000000000000000, 0.8660254037844387076, 1.000000000000000000, 0.8660254037844387076, 1.000000000000000000, 0.8660254037844387076, 1.000000000000000000, 0.8660254037844387076, 1.000000000000000000, 0.8660254037844387076, 1.000000000000000000, 0.8660254037844387076, 1.000000000000000000, 0.8660254037844387076, 1.000000000000000000, 0.8660254037844387076, 1.000000000000000000, 0.8660254037844387076, 1.000000000000000000, 0.8660254037844387076, 1.000000000000000000, 0.8660254037844387076, 1.000000000000000000, 0.8660254037844387076, 1.000000000000000000, 0.8660254037844387076, 1.000000000000000000, 0.8660254037844387076, 1.000000000000000000, 0.8660254037844387076, 1.000000000000000000, 0.8660254037844387076, 1.000000000000000000, 0.8660254037844387076, 1.000000000000000000, 0.8660254037844387076, 1.000000000000000000, 0.8660254037844387076, 1.000000000000000000, 0.8660254037844387076, 1.000000000000000000, 0.8660254037844387076, 1.000000000000000000, 0.8660254037844387076, 1.000000000000000000, 0.8660254037844387076, 1.000000000000000000, 0.8660254037844387076, 1.000000000000000000, 0.8660254037844387076, 1.000000000000000000, 0.8660254037844387076, 1.000000000000000000, 0.8660254037844387076, 1.000000000000000000, 0.8660254037844387076, 1.000000000000000000, 0.8660254037844387076, 1.000000000000000000, 0.8660254037844387076, 1.000000000000000000, 0.8660254037844387076, 1.000000000000000000, 0.8660254037844387076, 1.000000000000000000, 0.8660254037844387076, 1.000000000000000000, 0.8660254037844387076, 1.000000000000000000, 0.8660254037844387076, 1.000000000000000000, 0.8660254037844387076, 1.000000000000000000, 0.8660254037844387076, 1.000000000000000000, 0.8660254037844387076, 1.000000000000000000, 0.8660254037844387076, 1.000000000000000000, 0.8660254037844387076, 1.000000000000000000, 0.8660254037844387076, 1.000000000000000000, 0.8660254037844387076, 1.000000000000000000, 0.8660254037844387076, 1.000000000000000000, 0.8660254037844387076, 1.000000000000000000, 0.8660254037844387076, 1.000000000000000000, 0.8660254037844387076, 1.000000000000000000, 0.8660254037844387076, 1.000000000000000000, 0.8660254037844387076, 1.000000000000000000, 0.8660254037844387076, 1.000000000000000000, 0.8660254037844387076, 1.000000000000000000, 0.8660254037844387076, 1.000000000000000000, 0.8660254037844387076, 1.000000000000000000, 0.8660254037844387076, 1.000000000000000000, 0.8660254037844387076, 1.000000000000000000, 0.8660254037844387076, 1.000000000000000000, 0.8660254037844387076, 1.000000000000000000, 0.8660254037844387076, 1.000000000000000000, 0.8660254037844387076, 1.000000000000000000, 0.8660254037844387076, 1.000000000000000000, 0.8660254037844387076, 1.000000000000000000, 0.8660254037844387076, 1.000000000000000000, 0.8660254037844387076, 1.000000000000000000, 0.8660254037844387076, 1.000000000000000000, 0.8660254037844387076, 1.000000000000000000, 0.8660254037844387076, 1.000000000000000000, 0.8660254037844387076, 1.000000000000000000, 0.8660254037844387076, 1.000000000000000000, 0.8660254037844387076, 1.000000000000000000, 0.8660254037844387076, 1.000000000000000000, 0.8660254037844387076, 1.000000000000000000, 0.8660254037844387076, 1.000000000000000000, 0.8660254037844387076, 1.000000000000000000, 0.8660254037844387076, 1.000000000000000000, 0.8660254037844387076, 1.000000000000000000, 0.8660254037844387076, 1.000000000000000000, 0.8660254037844387076, 1.000000000000000000, 0.8660254037844387076, 1.000000000000000000, 0.8660254037844387076, 1.000000000000000000, 0.8660254037844387076, 1.000000000000000000, 0.8660254037844387076, 1.000000000000000000, 0.8660254037844387076, 1.000000000000000000, 0.8660254037844387076, 1.000000000000000000, 0.8660254037844387076, 1.000000000000000000, 0.8660254037844387076, 1.000000000000000000, 0.8660254037844387076, 1.000000000000000000, 0.8660254037844387076, 1.000000000000000000, 0.8660254037844387076, 1.000000000000000000, 0.8660254037844387076, 1.000000000000000000, 0.8660254037844387076, 1.000000000000000000, 0.8660254037844387076, 1.000000000000000000, 0.8660254037844387076, 1.000000000000000000, 0.8660254037844387076, 1.000000000000000000, 0.8660254037844387076, 1.000000000000000000, 0.8660254037844387076, 1.000000000000000000, 0.8660254037844387076, 1.000000000000000000, 0.8660254037844387076, 1.000000000000000000, 0.8660254037844387076, 1.000000000000000000, 0.8660254037844387076, 1.000000000000000000, 0.8660254037844387076, 1.000000000000000000, 0.8660254037844387076, 1.000000000000000000, 0.8660254037844387076, 1.000000000000000000, 0.8660254037844387076, 1.000000000000000000, 0.8660254037844387076, 1.000000000000000000, 0.8660254037844387076, 1.000000000000000000, 0.8660254037844387076, 1.000000000000000000, 0.8660254037844387076, 1.000000000000000000, 0.8660254037844387076, 1.000000000000000000, 0.8660254037844387076, 1.000000000000000000, 0.8660254037844387076, 1.000000000000000000, 0.8660254037844387076, 1.000000000000000000, 0.8660254037844387076, 1.000000000000000000, 0.8660254037844387076, 1.000000000000000000, 0.8660254037844387076, 1.000000000000000000, 0.8660254037844387076, 1.000000000000000000, 0.8660254037844387076, 1.000000000000000000, 0.8660254037844387076, 1.000000000000000000, 0.8660254037844387076, 1.000000000000000000, 0.8660254037844387076, 1.000000000000000000, 0.8660254037844387076, 1.000000000000000000, 0.8660254037844387076, 1.000000000000000000, 0.8660254037844387076, 1.000000000000000000, 0.8660254037844387076, 1.000000000000000000, 0.8660254037844387076, 1.000000000000000000, 0.8660254037844387076, 1.000000000000000000, 0.8660254037844387076, 1.000000000000000000, 0.8660254037844387076, 1.000000000000000000, 0.8660254037844387076, 1.000000000000000000, 0.8660254037844387076, 1.000000000000000000, 0.8660254037844387076, 1.000000000000000000, 0.8660254037844387076, 1.000000000000000000, 0.8660254037844387076, 1.000000000000000000, 0.8660254037844387076, 1.000000000000000000, 0.8660254037844387076, 1.000000000000000000, 0.8660254037844387076, 1.000000000000000000, 0.8660254037844387076, 1.000000000000000000, 0.8660254037844387076, 1.000000000000000000, 0.8660254037844387076, 1.000000000000000000, 0.8660254037844387076, 1.000000000000000000, 0.8660254037844387076, 1.000000000000000000, 0.8660254037844387076, 1.000000000000000000, 0.8660254037844387076, 1.000000000000000000, 0.8660254037844387076, 1.000000000000000000, 0.8660254037844387076, 1.000000000000000000, 0.8660254037844387076, 1.000000000000000000, 0.8660254037844387076, 1.000000000000000000, 0.8660254037844387076, 1.000000000000000000, 0.8660254037844387076, 1.000000000000000000, 0.8660254037844387076, 1.000000000000000000, 0.8660254037844387076, 1.000000000000000000, 0.8660254037844387076, 1.000000000000000000, 0.8660254037844387076, 1.000000000000000000, 0.8660254037844387076, 1.000000000000000000, 0.8660254037844387076, 1.000000000000000000, 0.8660254037844387076, 1.000000000000000000, 0.8660254037844387076, 1.000000000000000000, 0.8660254037844387076, 1.000000000000000000, 0.8660254037844387076, 1.000000000000000000, 0.8660254037844387076, 1.000000000000000000, 0.8660254037844387076, 1.000000000000000000, 0.8660254037844387076, 1.000000000000000000, 0.8660254037844387076, 1.000000000000000000, 0.8660254037844387076, 1.000000000000000000, 0.8660254037844387076, 1.000000000000000000, 0.8660254037844387076, 1.000000000000000000, 0.8660254037844387076, 1.000000000000000000, 0.8660254037844387076, 1.000000000000000000, 0.8660254037844387076, 1.000000000000000000, 0.8660254037844387076, 1.000000000000000000, 0.8660254037844387076, 1.000000000000000000, 0.8660254037844387076, 1.000000000000000000, 0.8660254037844387076, 1.000000000000000000, 0.8660254037844387076, 1.000000000000000000, 0.8660254037844387076, 1.000000000000000000, 0.8660254037844387076, 1.000000000000000000, 0.8660254037844387076, 1.000000000000000000, 0.8660254037844387076, 1.000000000000000000, 0.8660254037844387076, 1.000000000000000000, 0.8660254037844387076, 1.000000000000000000, 0.8660254037844387076, 1.000000000000000000, 0.8660254037844387076, 1.000000000000000000, 0.8660254037844387076, 1.000000000000000000, 0.8660254037844387076, 1.000000000000000000, 0.8660254037844387076, 1.000000000000000000, 0.8660254037844387076, 1.000000000000000000, 0.8660254037844387076, 1.000000000000000000, 0.8660254037844387076, 1.000000000000000000, 0.8660254037844387076, 1.000000000000000000, 0.8660254037844387076, 1.000000000000000000, 0.8660254037844387076, 1.000000000000000000, 0.8660254037844387076, 1.000000000000000000, 0.8660254037844387076, 1.000000000000000000, 0.8660254037844387076, 1.000000000000000000, 0.8660254037844387076, 1.000000000000000000, 0.8660254037844387076, 1.000000000000000000, 0.8660254037844387076, 1.000000000000000000, 0.8660254037844387076, 1.000000000000000000, 0.8660254037844387076, 1.000000000000000000, 0.8660254037844387076, 1.000000000000000000, 0.8660254037844387076, 1.000000000000000000, 0.8660254037844387076, 1.000000000000000000, 0.8660254037844387076, 1.000000000000000000, 0.8660254037844387076, 1.000000000000000000, 0.8660254037844387076, 1.000000000000000000, 0.8660254037844387076, 1.000000000000000000, 0.8660254037844387076, 1.000000000000000000, 0.8660254037844387076, 1.000000000000000000, 0.8660254037844387076, 1.000000000000000000, 0.8660254037844387076, 1.000000000000000000, 0.8660254037844387076, 1.000000000000000000, 0.8660254037844387076, 1.000000000000000000, 0.8660254037844387076, 1.000000000000000000, 0.8660254037844387076, 1.000000000000000000, 0.8660254037844387076, 1.000000000000000000, 0.8660254037844387076, 1.000000000000000000, 0.8660254037844387076, 1.000000000000000000, 0.8660254037844387076, 1.000000000000000000, 0.8660254037844387076, 1.000000000000000000, 0.8660254037844387076, 1.000000000000000000, 0.8660254037844387076, 1.000000000000000000, 0.8660254037844387076, 1.000000000000000000, 0.8660254037844387076, 1.000000000000000000, 0.8660254037844387076, 1.000000000000000000, 0.8660254037844387076, 1.000000000000000000, 0.8660254037844387076, 1.000000000000000000, 0.8660254037844387076, 1.000000000000000000, 0.8660254037844387076, 1.000000000000000000, 0.8660254037844387076, 1.000000000000000000, 0.8660254037844387076, 1.000000000000000000, 0.8660254037844387076, 1.000000000000000000, 0.8660254037844387076, 1.000000000000000000, 0.8660254037844387076, 1.000000000000000000, 0.8660254037844387076, 1.000000000000000000, 0.8660254037844387076, 1.000000000000000000, 0.8660254037844387076, 1.000000000000000000, 0.8660254037844387076, 1.000000000000000000, 0.8660254037844387076, 1.000000000000000000, 0.8660254037844387076, 1.000000000000000000, 0.8660254037844387076, 1.000000000000000000, 0.8660254037844387076, 1.000000000000000000, 0.8660254037844387076, 1.000000000000000000, 0.8660254037844387076, 1.000000000000000000, 0.8660254037844387076, 1.000000000000000000, 0.8660254037844387076, 1.000000000000000000, 0.8660254037844387076, 1.000000000000000000, 0.8660254037844387076, 1.000000000000000000, 0.8660254037844387076, 1.000000000000000000, 0.8660254037844387076, 1.000000000000000000, 0.8660254037844387076, 1.000000000000000000, 0.8660254037844387076, 1.000000000000000000, 0.8660254037844387076, 1.000000000000000000, 0.8660254037844387076, 1.000000000000000000, 0.8660254037844387076, 1.000000000000000000, 0.8660254037844387076, 1.000000000000000000, 0.8660254037844387076, 1.000000000000000000, 0.8660254037844387076, 1.000000000000000000, 0.8660254037844387076, 1.000000000000000000, 0.8660254037844387076, 1.000000000000000000, 0.8660254037844387076, 1.000000000000000000, 0.8660254037844387076, 1.000000000000000000, 0.8660254037844387076, 1.000000000000000000, 0.8660254037844387076, 1.000000000000000000, 0.8660254037844387076, 1.000000000000000000, 0.8660254037844387076, 1.000000000000000000, 0.8660254037844387076, 1.000000000000000000, 0.8660254037844387076, 1.000000000000000000, 0.8660254037844387076, 1.000000000000000000, 0.8660254037844387076, 1.000000000000000000, 0.8660254037844387076, 1.000000000000000000, 0.8660254037844387076, 1.000000000000000000, 0.8660254037844387076, 1.000000000000000000, 0.8660254037844387076, 1.000000000000000000, 0.8660254037844387076, 1.000000000000000000, 0.8660254037844387076, 1.000000000000000000, 0.8660254037844387076, 1.000000000000000000, 0.8660254037844387076, 1.000000000000000000, 0.8660254037844387076, 1.000000000000000000, 0.8660254037844387076, 1.000000000000000000, 0.8660254037844387076, 1.000000000000000000, 0.8660254037844387076, 1.000000000000000000, 0.8660254037844387076, 1.000000000000000000, 0.8660254037844387076, 1.000000000000000000, 0.8660254037844387076, 1.000000000000000000, 0.8660254037844387076, 1.000000000000000000, 0.8660254037844387076, 1.000000000000000000, 0.8660254037844387076, 1.000000000000000000, 0.8660254037844387076, 1.000000000000000000, 0.8660254037844387076, 1.000000000000000000, 0.8660254037844387076, 1.000000000000000000, 0.8660254037844387076, 1.000000000000000000, 0.8660254037844387076, 1.000000000000000000, 0.8660254037844387076, 1.000000000000000000, 0.8660254037844387076, 1.000000000000000000, 0.8660254037844387076, 1.000000000000000000, 0.8660254037844387076, 1.000000000000000000, 0.8660254037844387076, 1.000000000000000000, 0.8660254037844387076, 1.000000000000000000, 0.8660254037844387076, 1.000000000000000000, 0.8660254037844387076, 1.000000000000000000, 0.8660254037844387076, 1.000000000000000000, 0.8660254037844387076, 1.000000000000000000, 0.8660254037844387076, 1.000000000000000000, 0.8660254037844387076, 1.000000000000000000, 0.8660254037844387076, 1.000000000000000000, 0.8660254037844387076, 1.000000000000000000, 0.8660254037844387076, 1.000000000000000000, 0.8660254037844387076, 1.000000000000000000, 0.8660254037844387076, 1.000000000000000000, 0.8660254037844387076, 1.000000000000000000, 0.8660254037844387076, 1.000000000000000000, 0.8660254037844387076, 1.000000000000000000, 0.8660254037844387076, 1.000000000000000000, 0.8660254037844387076, 1.000000000000000000, 0.8660254037844387076, 1.000000000000000000, 0.8660254037844387076, 1.000000000000000000, 0.8660254037844387076, 1.000000000000000000, 0.8660254037844387076, 1.000000000000000000, 0.8660254037844387076, 1.000000000000000000, 0.8660254037844387076, 1.000000000000000000, 0.8660254037844387076, 1.000000000000000000, 0.8660254037844387076, 1.000000000000000000, 0.8660254037844387076, 1.000000000000000000, 0.8660254037844387076, 1.000000000000000000, 0.8660254037844387076, 1.000000000000000000, 0.8660254037844387076, 1.000000000000000000, 0.8660254037844387076, 1.000000000000000000, 0.8660254037844387076, 1.000000000000000000, 0.8660254037844387076, 1.000000000000000000, 0.8660254037844387076, 1.000000000000000000, 0.8660254037844387076, 1.000000000000000000, 0.8660254037844387076, 1.000000000000000000, 0.8660254037844387076, 1.000000000000000000, 0.8660254037844387076, 1.000000000000000000, 0.8660254037844387076, 1.000000000000000000, 0.8660254037844387076, 1.000000000000000000, 0.8660254037844387076, 1.000000000000000000, 0.8660254037844387076, 1.000000000000000000, 0.8660254037844387076, 1.000000000000000000, 0.8660254037844387076, 1.000000000000000000, 0.8660254037844387076, 1.000000000000000000, 0.8660254037844387076, 1.000000000000000000, 0.8660254037844387076, 1.000000000000000000, 0.8660254037844387076, 1.000000000000000000, 0.8660254037844387076, 1.000000000000000000, 0.8660254037844387076, 1.000000000000000000, 0.8660254037844387076, 1.000000000000000000, 0.8660254037844387076, 1.000000000000000000, 0.8660254037844387076, 1.000000000000000000, 0.8660254037844387076, 1.000000000000000000, 0.8660254037844387076, 1.000000000000000000, 0.8660254037844387076, 1.000000000000000000, 0.8660254037844387076, 1.000000000000000000, 0.8660254037844387076, 1.000000000000000000, 0.8660254037844387076, 1.000000000000000000, 0.8660254037844387076, 1.000000000000000000, 0.8660254037844387076, 1.000000000000000000, 0.8660254037844387076, 1.000000000000000000, 0.8660254037844387076, 1.000000000000000000, 0.8660254037844387076, 1.000000000000000000, 0.8660254037844387076, 1.000000000000000000, 0.8660254037844387076, 1.000000000000000000, 0.8660254037844387076, 1.000000000000000000, 0.8660254037844387076, 1.000000000000000000, 0.8660254037844387076, 1.000000000000000000, 0.8660254037844387076, 1.000000000000000000, 0.8660254037844387076, 1.000000000000000000, 0.8660254037844387076, 1.000000000000000000, 0.8660254037844387076, 1.000000000000000000, 0.8660254037844387076, 1.000000000000000000, 0.8660254037844387076, 1.000000000000000000, 0.8660254037844387076, 1.000000000000000000, 0.8660254037844387076, 1.000000000000000000, 0.8660254037844387076, 1.000000000000000000, 0.8660254037844387076, 1.000000000000000000, 0.8660254037844387076, 1.000000000000000000, 0.8660254037844387076, 1.000000000000000000, 0.8660254037844387076, 1.000000000000000000, 0.8660254037844387076, 1.000000000000000000, 0.8660254037844387076, 1.000000000000000000, 0.8660254037844387076, 1.000000000000000000, 0.8660254037844387076, 1.000000000000000000, 0.8660254037844387076, 1.000000000000000000, 0.8660254037844387076, 1.000000000000000000, 0.8660254037844387076, 1.000000000000000000, 0.8660254037844387076, 1.000000000000000000, 0.8660254037844387076, 1.000000000000000000, 0.8660254037844387076, 1.000000000000000000, 0.8660254037844387076, 1.000000000000000000, 0.8660254037844387076, 1.000000000000000000, 0.8660254037844387076, 1.000000000000000000, 0.8660254037844387076, 1.000000000000000000, 0.8660254037844387076, 1.000000000000000000, 0.8660254037844387076, 1.000000000000000000, 0.8660254037844387076, 1.000000000000000000, 0.8660254037844387076, 1.000000000000000000, 0.8660254037844387076, 1.000000000000000000, 0.8660254037844387076, 1.000000000000000000, 0.8660254037844387076, 1.000000000000000000, 0.8660254037844387076, 1.000000000000000000, 0.8660254037844387076, 1.000000000000000000, 0.8660254037844387076, 1.000000000000000000, 0.8660254037844387076, 1.000000000000000000, 0.8660254037844387076, 1.000000000000000000, 0.8660254037844387076, 1.000000000000000000, 0.8660254037844387076, 1.000000000000000000, 0.8660254037844387076, 1.000000000000000000, 0.8660254037844387076, 1.000000000000000000, 0.8660254037844387076, 1.000000000000000000, 0.8660254037844387076, 1.000000000000000000, 0.8660254037844387076, 1.000000000000000000, 0.8660254037844387076, 1.000000000000000000, 0.8660254037844387076, 1.000000000000000000, 0.8660254037844387076, 1.000000000000000000, 0.8660254037844387076, 1.000000000000000000, 0.8660254037844387076, 1.000000000000000000, 0.8660254037844387076, 1.000000000000000000, 0.8660254037844387076, 1.000000000000000000, 0.8660254037844387076, 1.000000000000000000, 0.8660254037844387076, 1.000000000000000000, 0.8660254037844387076, 1.000000000000000000, 0.8660254037844387076, 1.000000000000000000, 0.8660254037844387076, 1.000000000000000000, 0.8660254037844387076, 1.000000000000000000, 0.8660254037844387076, 1.000000000000000000, 0.8660254037844387076, 1.000000000000000000, 0.8660254037844387076, 1.000000000000000000, 0.8660254037844387076, 1.000000000000000000, 0.8660254037844387076, 1.000000000000000000, 0.8660254037844387076, 1.000000000000000000, 0.8660254037844387076, 1.000000000000000000, 0.8660254037844387076, 1.000000000000000000, 0.8660254037844387076, 1.000000000000000000, 0.8660254037844387076, 1.000000000000000000, 0.8660254037844387076, 1.000000000000000000, 0.8660254037844387076, 1.000000000000000000, 0.8660254037844387076, 1.000000000000000000, 0.8660254037844387076, 1.000000000000000000, 0.8660254037844387076, 1.000000000000000000, 0.8660254037844387076, 1.000000000000000000, 0.8660254037844387076, 1.000000000000000000, 0.8660254037844387076, 1.000000000000000000, 0.8660254037844387076, 1.000000000000000000, 0.8660254037844387076, 1.000000000000000000, 0.8660254037844387076, 1.000000000000000000, 0.8660254037844387076, 1.000000000000000000, 0.8660254037844387076, 1.000000000000000000, 0.8660254037844387076, 1.000000000000000000, 0.8660254037844387076, 1.000000000000000000, 0.8660254037844387076, 1.000000000000000000, 0.8660254037844387076, 1.000000000000000000, 0.8660254037844387076, 1.000000000000000000, 0.8660254037844387076, 1.000000000000000000, 0.8660254037844387076, 1.000000000000000000, 0.8660254037844387076, 1.000000000000000000, 0.8660254037844387076, 1.000000000000000000, 0.8660254037844387076, 1.000000000000000000, 0.8660254037844387076, 1.000000000000000000, 0.8660254037844387076, 1.000000000000000000, 0.8660254037844387076, 1.000000000000000000, 0.8660254037844387076, 1.000000000000000000, 0.8660254037844387076, 1.000000000000000000, 0.8660254037844387076, 1.000000000000000000, 0.8660254037844387076, 1.000000000000000000, 0.8660254037844387076, 1.000000000000000000, 0.8660254037844387076, 1.000000000000000000, 0.8660254037844387076, 1.000000000000000000, 0.8660254037844387076, 1.000000000000000000, 0.8660254037844387076, 1.000000000000000000, 0.8660254037844387076, 1.000000000000000000, 0.8660254037844387076, 1.000000000000000000, 0.8660254037844387076, 1.000000000000000000, 0.8660254037844387076, 1.000000000000000000, 0.8660254037844387076, 1.000000000000000000, 0.8660254037844387076, 1.000000000000000000, 0.8660254037844387076, 1.000000000000000000, 0.8660254037844387076, 1.000000000000000000, 0.8660254037844387076, 1.000000000000000000, 0.8660254037844387076, 1.000000000000000000, 0.8660254037844387076, 1.000000000000000000),
 ( 1.000000000000000000, 0.8660254037844387076, 1.000000000000000000, 0.8660254037844387076, 1.000000000000000000, 0.8660254037844387076, 1.000000000000000000, 0.8660254037844387076, 1.000000000000000000, 0.8660254037844387076, 1.000000000000000000, 0.8660254037844387076, 1.000000000000000000, 0.8660254037844387076, 1.000000000000000000, 0.8660254037844387076, 1.000000000000000000, 0.8660254037844387076, 1.000000000000000000, 0.8660254037844387076, 1.000000000000000000, 0.8660254037844387076, 1.000000000000000000, 0.8660254037844387076, 1.000000000000000000, 0.8660254037844387076, 1.000000000000000000, 0.8660254037844387076, 1.000000000000000000, 0.8660254037844387076, 1.000000000000000000, 0.8660254037844387076, 1.000000000000000000, 0.8660254037844387076, 1.000000000000000000, 0.8660254037844387076, 1.000000000000000000, 0.8660254037844387076, 1.000000000000000000, 0.8660254037844387076, 1.000000000000000000, 0.8660254037844387076, 1.000000000000000000, 0.8660254037844387076, 1.000000000000000000, 0.8660254037844387076, 1.000000000000000000, 0.8660254037844387076, 1.000000000000000000, 0.8660254037844387076, 1.000000000000000000, 0.8660254037844387076, 1.000000000000000000, 0.8660254037844387076, 1.000000000000000000, 0.8660254037844387076, 1.000000000000000000, 0.8660254037844387076, 1.000000000000000000, 0.8660254037844387076, 1.000000000000000000, 0.8660254037844387076, 1.000000000000000000, 0.8660254037844387076, 1.000000000000000000, 0.8660254037844387076, 1.000000000000000000, 0.8660254037844387076, 1.000000000000000000, 0.8660254037844387076, 1.000000000000000000, 0.8660254037844387076, 1.000000000000000000, 0.8660254037844387076, 1.000000000000000000, 0.8660254037844387076, 1.000000000000000000, 0.8660254037844387076, 1.000000000000000000, 0.8660254037844387076, 1.000000000000000000, 0.8660254037844387076, 1.000000000000000000, 0.8660254037844387076, 1.000000000000000000, 0.8660254037844387076, 1.000000000000000000, 0.8660254037844387076, 1.000000000000000000, 0.8660254037844387076, 1.000000000000000000, 0.8660254037844387076, 1.000000000000000000, 0.8660254037844387076, 1.000000000000000000, 0.8660254037844387076, 1.000000000000000000, 0.8660254037844387076, 1.000000000000000000, 0.8660254037844387076, 1.000000000000000000, 0.8660254037844387076, 1.000000000000000000, 0.8660254037844387076, 1.000000000000000000, 0.8660254037844387076, 1.000000000000000000, 0.8660254037844387076, 1.000000000000000000, 0.8660254037844387076, 1.000000000000000000, 0.8660254037844387076, 1.000000000000000000, 0.8660254037844387076, 1.000000000000000000, 0.8660254037844387076, 1.000000000000000000, 0.8660254037844387076, 1.000000000000000000, 0.8660254037844387076, 1.000000000000000000, 0.8660254037844387076, 1.000000000000000000, 0.8660254037844387076, 1.000000000000000000, 0.8660254037844387076, 1.000000000000000000, 0.8660254037844387076, 1.000000000000000000, 0.8660254037844387076, 1.000000000000000000, 0.8660254037844387076, 1.000000000000000000, 0.8660254037844387076, 1.000000000000000000, 0.8660254037844387076, 1.000000000000000000, 0.8660254037844387076, 1.000000000000000000, 0.8660254037844387076, 1.000000000000000000, 0.8660254037844387076, 1.000000000000000000, 0.8660254037844387076, 1.000000000000000000, 0.8660254037844387076, 1.000000000000000000, 0.8660254037844387076, 1.000000000000000000, 0.8660254037844387076, 1.000000000000000000, 0.8660254037844387076, 1.000000000000000000, 0.8660254037844387076, 1.000000000000000000, 0.8660254037844387076, 1.000000000000000000, 0.8660254037844387076, 1.000000000000000000, 0.8660254037844387076, 1.000000000000000000, 0.8660254037844387076, 1.000000000000000000, 0.8660254037844387076, 1.000000000000000000, 0.8660254037844387076, 1.000000000000000000, 0.8660254037844387076, 1.000000000000000000, 0.8660254037844387076, 1.000000000000000000, 0.8660254037844387076, 1.000000000000000000, 0.8660254037844387076, 1.000000000000000000, 0.8660254037844387076, 1.000000000000000000, 0.8660254037844387076, 1.000000000000000000, 0.8660254037844387076, 1.000000000000000000, 0.8660254037844387076, 1.000000000000000000, 0.8660254037844387076, 1.000000000000000000, 0.8660254037844387076, 1.000000000000000000, 0.8660254037844387076, 1.000000000000000000, 0.8660254037844387076, 1.000000000000000000, 0.8660254037844387076, 1.000000000000000000, 0.8660254037844387076, 1.000000000000000000, 0.8660254037844387076, 1.000000000000000000, 0.8660254037844387076, 1.000000000000000000, 0.8660254037844387076, 1.000000000000000000, 0.8660254037844387076, 1.000000000000000000, 0.8660254037844387076, 1.000000000000000000, 0.8660254037844387076, 1.000000000000000000, 0.8660254037844387076, 1.000000000000000000, 0.8660254037844387076, 1.000000000000000000, 0.8660254037844387076, 1.000000000000000000, 0.8660254037844387076, 1.000000000000000000, 0.8660254037844387076, 1.000000000000000000, 0.8660254037844387076, 1.000000000000000000, 0.8660254037844387076, 1.000000000000000000, 0.8660254037844387076, 1.000000000000000000, 0.8660254037844387076, 1.000000000000000000, 0.8660254037844387076, 1.000000000000000000, 0.8660254037844387076, 1.000000000000000000, 0.8660254037844387076, 1.000000000000000000, 0.8660254037844387076, 1.000000000000000000, 0.8660254037844387076, 1.000000000000000000, 0.8660254037844387076, 1.000000000000000000, 0.8660254037844387076, 1.000000000000000000, 0.8660254037844387076, 1.000000000000000000, 0.8660254037844387076, 1.000000000000000000, 0.8660254037844387076, 1.000000000000000000, 0.8660254037844387076, 1.000000000000000000, 0.8660254037844387076, 1.000000000000000000, 0.8660254037844387076, 1.000000000000000000, 0.8660254037844387076, 1.000000000000000000, 0.8660254037844387076, 1.000000000000000000, 0.8660254037844387076, 1.000000000000000000, 0.8660254037844387076, 1.000000000000000000, 0.8660254037844387076, 1.000000000000000000, 0.8660254037844387076, 1.000000000000000000, 0.8660254037844387076, 1.000000000000000000, 0.8660254037844387076, 1.000000000000000000, 0.8660254037844387076, 1.000000000000000000, 0.8660254037844387076, 1.000000000000000000, 0.8660254037844387076, 1.000000000000000000, 0.8660254037844387076, 1.000000000000000000, 0.8660254037844387076, 1.000000000000000000, 0.8660254037844387076, 1.000000000000000000, 0.8660254037844387076, 1.000000000000000000, 0.8660254037844387076, 1.000000000000000000, 0.8660254037844387076, 1.000000000000000000, 0.8660254037844387076, 1.000000000000000000, 0.8660254037844387076, 1.000000000000000000, 0.8660254037844387076, 1.000000000000000000, 0.8660254037844387076, 1.000000000000000000, 0.8660254037844387076, 1.000000000000000000, 0.8660254037844387076, 1.000000000000000000, 0.8660254037844387076, 1.000000000000000000, 0.8660254037844387076, 1.000000000000000000, 0.8660254037844387076, 1.000000000000000000, 0.8660254037844387076, 1.000000000000000000, 0.8660254037844387076, 1.000000000000000000, 0.8660254037844387076, 1.000000000000000000, 0.8660254037844387076, 1.000000000000000000, 0.8660254037844387076, 1.000000000000000000, 0.8660254037844387076, 1.000000000000000000, 0.8660254037844387076, 1.000000000000000000, 0.8660254037844387076, 1.000000000000000000, 0.8660254037844387076, 1.000000000000000000, 0.8660254037844387076, 1.000000000000000000, 0.8660254037844387076, 1.000000000000000000, 0.8660254037844387076, 1.000000000000000000, 0.8660254037844387076, 1.000000000000000000, 0.8660254037844387076, 1.000000000000000000, 0.8660254037844387076, 1.000000000000000000, 0.8660254037844387076, 1.000000000000000000, 0.8660254037844387076, 1.000000000000000000, 0.8660254037844387076, 1.000000000000000000, 0.8660254037844387076, 1.000000000000000000, 0.8660254037844387076, 1.000000000000000000, 0.8660254037844387076, 1.000000000000000000, 0.8660254037844387076, 1.000000000000000000, 0.8660254037844387076, 1.000000000000000000, 0.8660254037844387076, 1.000000000000000000, 0.8660254037844387076, 1.000000000000000000, 0.8660254037844387076, 1.000000000000000000, 0.8660254037844387076, 1.000000000000000000, 0.8660254037844387076, 1.000000000000000000, 0.8660254037844387076, 1.000000000000000000, 0.8660254037844387076, 1.000000000000000000, 0.8660254037844387076, 1.000000000000000000, 0.8660254037844387076, 1.000000000000000000, 0.8660254037844387076, 1.000000000000000000, 0.8660254037844387076, 1.000000000000000000, 0.8660254037844387076, 1.000000000000000000, 0.8660254037844387076, 1.000000000000000000, 0.8660254037844387076, 1.000000000000000000, 0.8660254037844387076, 1.000000000000000000, 0.8660254037844387076, 1.000000000000000000, 0.8660254037844387076, 1.000000000000000000, 0.8660254037844387076, 1.000000000000000000, 0.8660254037844387076, 1.000000000000000000, 0.8660254037844387076, 1.000000000000000000, 0.8660254037844387076, 1.000000000000000000, 0.8660254037844387076, 1.000000000000000000, 0.8660254037844387076, 1.000000000000000000, 0.8660254037844387076, 1.000000000000000000, 0.8660254037844387076, 1.000000000000000000, 0.8660254037844387076, 1.000000000000000000, 0.8660254037844387076, 1.000000000000000000, 0.8660254037844387076, 1.000000000000000000, 0.8660254037844387076, 1.000000000000000000, 0.8660254037844387076, 1.000000000000000000, 0.8660254037844387076, 1.000000000000000000, 0.8660254037844387076, 1.000000000000000000, 0.8660254037844387076, 1.000000000000000000, 0.8660254037844387076, 1.000000000000000000, 0.8660254037844387076, 1.000000000000000000, 0.8660254037844387076, 1.000000000000000000, 0.8660254037844387076, 1.000000000000000000, 0.8660254037844387076, 1.000000000000000000, 0.8660254037844387076, 1.000000000000000000, 0.8660254037844387076, 1.000000000000000000, 0.8660254037844387076, 1.000000000000000000, 0.8660254037844387076, 1.000000000000000000, 0.8660254037844387076, 1.000000000000000000, 0.8660254037844387076, 1.000000000000000000, 0.8660254037844387076, 1.000000000000000000, 0.8660254037844387076, 1.000000000000000000, 0.8660254037844387076, 1.000000000000000000, 0.8660254037844387076, 1.000000000000000000, 0.8660254037844387076, 1.000000000000000000, 0.8660254037844387076, 1.000000000000000000, 0.8660254037844387076, 1.000000000000000000, 0.8660254037844387076, 1.000000000000000000, 0.8660254037844387076, 1.000000000000000000, 0.8660254037844387076, 1.000000000000000000, 0.8660254037844387076, 1.000000000000000000, 0.8660254037844387076, 1.000000000000000000, 0.8660254037844387076, 1.000000000000000000, 0.8660254037844387076, 1.000000000000000000, 0.8660254037844387076, 1.000000000000000000, 0.8660254037844387076, 1.000000000000000000, 0.8660254037844387076, 1.000000000000000000, 0.8660254037844387076, 1.000000000000000000, 0.8660254037844387076, 1.000000000000000000, 0.8660254037844387076, 1.000000000000000000, 0.8660254037844387076, 1.000000000000000000, 0.8660254037844387076, 1.000000000000000000, 0.8660254037844387076, 1.000000000000000000, 0.8660254037844387076, 1.000000000000000000, 0.8660254037844387076, 1.000000000000000000, 0.8660254037844387076, 1.000000000000000000, 0.8660254037844387076, 1.000000000000000000, 0.8660254037844387076, 1.000000000000000000, 0.8660254037844387076, 1.000000000000000000, 0.8660254037844387076, 1.000000000000000000, 0.8660254037844387076, 1.000000000000000000, 0.8660254037844387076, 1.000000000000000000, 0.8660254037844387076, 1.000000000000000000, 0.8660254037844387076, 1.000000000000000000, 0.8660254037844387076, 1.000000000000000000, 0.8660254037844387076, 1.000000000000000000, 0.8660254037844387076, 1.000000000000000000, 0.8660254037844387076, 1.000000000000000000, 0.8660254037844387076, 1.000000000000000000, 0.8660254037844387076, 1.000000000000000000, 0.8660254037844387076, 1.000000000000000000, 0.8660254037844387076, 1.000000000000000000, 0.8660254037844387076, 1.000000000000000000, 0.8660254037844387076, 1.000000000000000000, 0.8660254037844387076, 1.000000000000000000, 0.8660254037844387076, 1.000000000000000000, 0.8660254037844387076, 1.000000000000000000, 0.8660254037844387076, 1.000000000000000000, 0.8660254037844387076, 1.000000000000000000, 0.8660254037844387076, 1.000000000000000000, 0.8660254037844387076, 1.000000000000000000, 0.8660254037844387076, 1.000000000000000000, 0.8660254037844387076, 1.000000000000000000, 0.8660254037844387076, 1.000000000000000000, 0.8660254037844387076, 1.000000000000000000, 0.8660254037844387076, 1.000000000000000000, 0.8660254037844387076, 1.000000000000000000, 0.8660254037844387076, 1.000000000000000000, 0.8660254037844387076, 1.000000000000000000, 0.8660254037844387076, 1.000000000000000000, 0.8660254037844387076, 1.000000000000000000, 0.8660254037844387076, 1.000000000000000000, 0.8660254037844387076, 1.000000000000000000, 0.8660254037844387076, 1.000000000000000000, 0.8660254037844387076, 1.000000000000000000, 0.8660254037844387076, 1.000000000000000000, 0.8660254037844387076, 1.000000000000000000, 0.8660254037844387076, 1.000000000000000000, 0.8660254037844387076, 1.000000000000000000, 0.8660254037844387076, 1.000000000000000000, 0.8660254037844387076, 1.000000000000000000, 0.8660254037844387076, 1.000000000000000000, 0.8660254037844387076, 1.000000000000000000, 0.8660254037844387076, 1.000000000000000000, 0.8660254037844387076, 1.000000000000000000, 0.8660254037844387076, 1.000000000000000000, 0.8660254037844387076, 1.000000000000000000, 0.8660254037844387076, 1.000000000000000000, 0.8660254037844387076, 1.000000000000000000, 0.8660254037844387076, 1.000000000000000000, 0.8660254037844387076, 1.000000000000000000, 0.8660254037844387076, 1.000000000000000000, 0.8660254037844387076, 1.000000000000000000, 0.8660254037844387076, 1.000000000000000000, 0.8660254037844387076, 1.000000000000000000, 0.8660254037844387076, 1.000000000000000000, 0.8660254037844387076, 1.000000000000000000, 0.8660254037844387076, 1.000000000000000000, 0.8660254037844387076, 1.000000000000000000, 0.8660254037844387076, 1.000000000000000000, 0.8660254037844387076, 1.000000000000000000, 0.8660254037844387076, 1.000000000000000000, 0.8660254037844387076, 1.000000000000000000, 0.8660254037844387076, 1.000000000000000000, 0.8660254037844387076, 1.000000000000000000, 0.8660254037844387076, 1.000000000000000000, 0.8660254037844387076, 1.000000000000000000, 0.8660254037844387076, 1.000000000000000000, 0.8660254037844387076, 1.000000000000000000, 0.8660254037844387076, 1.000000000000000000, 0.8660254037844387076, 1.000000000000000000, 0.8660254037844387076, 1.000000000000000000, 0.8660254037844387076, 1.000000000000000000, 0.8660254037844387076, 1.000000000000000000, 0.8660254037844387076, 1.000000000000000000, 0.8660254037844387076, 1.000000000000000000, 0.8660254037844387076, 1.000000000000000000, 0.8660254037844387076, 1.000000000000000000, 0.8660254037844387076, 1.000000000000000000, 0.8660254037844387076, 1.000000000000000000, 0.8660254037844387076, 1.000000000000000000, 0.8660254037844387076, 1.000000000000000000, 0.8660254037844387076, 1.000000000000000000, 0.8660254037844387076, 1.000000000000000000, 0.8660254037844387076, 1.000000000000000000, 0.8660254037844387076, 1.000000000000000000, 0.8660254037844387076, 1.000000000000000000, 0.8660254037844387076, 1.000000000000000000, 0.8660254037844387076, 1.000000000000000000, 0.8660254037844387076, 1.000000000000000000, 0.8660254037844387076, 1.000000000000000000, 0.8660254037844387076, 1.000000000000000000, 0.8660254037844387076, 1.000000000000000000, 0.8660254037844387076, 1.000000000000000000, 0.8660254037844387076, 1.000000000000000000, 0.8660254037844387076, 1.000000000000000000, 0.8660254037844387076, 1.000000000000000000, 0.8660254037844387076, 1.000000000000000000, 0.8660254037844387076, 1.000000000000000000, 0.8660254037844387076, 1.000000000000000000, 0.8660254037844387076, 1.000000000000000000, 0.8660254037844387076, 1.000000000000000000, 0.8660254037844387076, 1.000000000000000000, 0.8660254037844387076, 1.000000000000000000, 0.8660254037844387076, 1.000000000000000000, 0.8660254037844387076, 1.000000000000000000, 0.8660254037844387076, 1.000000000000000000, 0.8660254037844387076, 1.000000000000000000, 0.8660254037844387076, 1.000000000000000000, 0.8660254037844387076, 1.000000000000000000, 0.8660254037844387076, 1.000000000000000000, 0.8660254037844387076, 1.000000000000000000, 0.8660254037844387076, 1.000000000000000000, 0.8660254037844387076, 1.000000000000000000, 0.8660254037844387076, 1.000000000000000000, 0.8660254037844387076, 1.000000000000000000, 0.8660254037844387076, 1.000000000000000000, 0.8660254037844387076, 1.000000000000000000, 0.8660254037844387076, 1.000000000000000000, 0.8660254037844387076, 1.000000000000000000, 0.8660254037844387076, 1.000000000000000000, 0.8660254037844387076, 1.000000000000000000, 0.8660254037844387076, 1.000000000000000000, 0.8660254037844387076, 1.000000000000000000, 0.8660254037844387076, 1.000000000000000000, 0.8660254037844387076, 1.000000000000000000, 0.8660254037844387076, 1.000000000000000000, 0.8660254037844387076, 1.000000000000000000, 0.8660254037844387076, 1.000000000000000000, 0.8660254037844387076, 1.000000000000000000, 0.8660254037844387076, 1.000000000000000000, 0.8660254037844387076, 1.000000000000000000, 0.8660254037844387076, 1.000000000000000000, 0.8660254037844387076, 1.000000000000000000, 0.8660254037844387076, 1.000000000000000000, 0.8660254037844387076, 1.000000000000000000, 0.8660254037844387076, 1.000000000000000000, 0.8660254037844387076, 1.000000000000000000, 0.8660254037844387076, 1.000000000000000000, 0.8660254037844387076, 1.000000000000000000, 0.8660254037844387076, 1.000000000000000000, 0.8660254037844387076, 1.000000000000000000, 0.8660254037844387076, 1.000000000000000000, 0.8660254037844387076, 1.000000000000000000, 0.8660254037844387076, 1.000000000000000000, 0.8660254037844387076, 1.000000000000000000, 0.8660254037844387076, 1.000000000000000000, 0.8660254037844387076, 1.000000000000000000, 0.8660254037844387076, 1.000000000000000000, 0.8660254037844387076, 1.000000000000000000, 0.8660254037844387076, 1.000000000000000000, 0.8660254037844387076, 1.000000000000000000, 0.8660254037844387076, 1.000000000000000000, 0.8660254037844387076, 1.000000000000000000, 0.8660254037844387076, 1.000000000000000000, 0.8660254037844387076, 1.000000000000000000, 0.8660254037844387076, 1.000000000000000000, 0.8660254037844387076, 1.000000000000000000, 0.8660254037844387076, 1.000000000000000000, 0.8660254037844387076, 1.000000000000000000, 0.8660254037844387076, 1.000000000000000000, 0.8660254037844387076, 1.000000000000000000, 0.8660254037844387076, 1.000000000000000000, 0.8660254037844387076, 1.000000000000000000, 0.8660254037844387076, 1.000000000000000000, 0.8660254037844387076, 1.000000000000000000, 0.8660254037844387076, 1.000000000000000000, 0.8660254037844387076, 1.000000000000000000, 0.8660254037844387076, 1.000000000000000000, 0.8660254037844387076, 1.000000000000000000, 0.8660254037844387076, 1.000000000000000000, 0.8660254037844387076, 1.000000000000000000, 0.8660254037844387076, 1.000000000000000000, 0.8660254037844387076, 1.000000000000000000, 0.8660254037844387076, 1.000000000000000000, 0.8660254037844387076, 1.000000000000000000, 0.8660254037844387076, 1.000000000000000000, 0.8660254037844387076, 1.000000000000000000, 0.8660254037844387076, 1.000000000000000000, 0.8660254037844387076, 1.000000000000000000, 0.8660254037844387076, 1.000000000000000000, 0.8660254037844387076, 1.000000000000000000, 0.8660254037844387076, 1.000000000000000000, 0.8660254037844387076, 1.000000000000000000, 0.8660254037844387076, 1.000000000000000000, 0.8660254037844387076, 1.000000000000000000, 0.8660254037844387076, 1.000000000000000000, 0.8660254037844387076, 1.000000000000000000, 0.8660254037844387076, 1.000000000000000000, 0.8660254037844387076, 1.000000000000000000, 0.8660254037844387076, 1.000000000000000000, 0.8660254037844387076, 1.000000000000000000, 0.8660254037844387076, 1.000000000000000000, 0.8660254037844387076, 1.000000000000000000, 0.8660254037844387076, 1.000000000000000000, 0.8660254037844387076, 1.000000000000000000, 0.8660254037844387076, 1.000000000000000000, 0.8660254037844387076, 1.000000000000000000, 0.8660254037844387076, 1.000000000000000000, 0.8660254037844387076, 1.000000000000000000, 0.8660254037844387076, 1.000000000000000000, 0.8660254037844387076, 1.000000000000000000, 0.8660254037844387076, 1.000000000000000000, 0.8660254037844387076, 1.000000000000000000, 0.8660254037844387076, 1.000000000000000000, 0.8660254037844387076, 1.000000000000000000, 0.8660254037844387076, 1.000000000000000000, 0.8660254037844387076, 1.000000000000000000, 0.8660254037844387076, 1.000000000000000000, 0.8660254037844387076, 1.000000000000000000, 0.8660254037844387076, 1.000000000000000000, 0.8660254037844387076, 1.000000000000000000, 0.8660254037844387076, 1.000000000000000000, 0.8660254037844387076, 1.000000000000000000, 0.8660254037844387076, 1.000000000000000000, 0.8660254037844387076, 1.000000000000000000, 0.8660254037844387076, 1.000000000000000000, 0.8660254037844387076, 1.000000000000000000, 0.8660254037844387076, 1.000000000000000000, 0.8660254037844387076, 1.000000000000000000, 0.8660254037844387076, 1.000000000000000000, 0.8660254037844387076, 1.000000000000000000, 0.8660254037844387076, 1.000000000000000000, 0.8660254037844387076, 1.000000000000000000, 0.8660254037844387076, 1.000000000000000000, 0.8660254037844387076, 1.000000000000000000, 0.8660254037844387076, 1.000000000000000000, 0.8660254037844387076, 1.000000000000000000, 0.8660254037844387076, 1.000000000000000000, 0.8660254037844387076, 1.000000000000000000, 0.8660254037844387076, 1.000000000000000000, 0.8660254037844387076, 1.000000000000000000, 0.8660254037844387076, 1.000000000000000000, 0.8660254037844387076, 1.000000000000000000, 0.8660254037844387076, 1.000000000000000000, 0.8660254037844387076, 1.000000000000000000, 0.8660254037844387076, 1.000000000000000000, 0.8660254037844387076, 1.000000000000000000, 0.8660254037844387076, 1.000000000000000000, 0.8660254037844387076, 1.000000000000000000, 0.8660254037844387076, 1.000000000000000000, 0.8660254037844387076, 1.000000000000000000, 0.8660254037844387076, 1.000000000000000000, 0.8660254037844387076, 1.000000000000000000, 0.8660254037844387076, 1.000000000000000000, 0.8660254037844387076, 1.000000000000000000, 0.8660254037844387076, 1.000000000000000000, 0.8660254037844387076, 1.000000000000000000, 0.8660254037844387076, 1.000000000000000000, 0.8660254037844387076, 1.000000000000000000, 0.8660254037844387076, 1.000000000000000000, 0.8660254037844387076, 1.000000000000000000, 0.8660254037844387076, 1.000000000000000000, 0.8660254037844387076, 1.000000000000000000, 0.8660254037844387076, 1.000000000000000000, 0.8660254037844387076, 1.000000000000000000, 0.8660254037844387076, 1.000000000000000000, 0.8660254037844387076, 1.000000000000000000, 0.8660254037844387076, 1.000000000000000000, 0.8660254037844387076, 1.000000000000000000, 0.8660254037844387076, 1.000000000000000000, 0.8660254037844387076, 1.000000000000000000, 0.8660254037844387076, 1.000000000000000000, 0.8660254037844387076, 1.000000000000000000, 0.8660254037844387076, 1.000000000000000000, 0.8660254037844387076, 1.000000000000000000, 0.8660254037844387076, 1.000000000000000000, 0.8660254037844387076, 1.000000000000000000, 0.8660254037844387076, 1.000000000000000000, 0.8660254037844387076, 1.000000000000000000, 0.8660254037844387076, 1.000000000000000000, 0.8660254037844387076, 1.000000000000000000, 0.8660254037844387076, 1.000000000000000000, 0.8660254037844387076, 1.000000000000000000, 0.8660254037844387076, 1.000000000000000000, 0.8660254037844387076, 1.000000000000000000, 0.8660254037844387076, 1.000000000000000000, 0.8660254037844387076, 1.000000000000000000, 0.8660254037844387076, 1.000000000000000000, 0.8660254037844387076, 1.000000000000000000, 0.8660254037844387076, 1.000000000000000000, 0.8660254037844387076, 1.000000000000000000, 0.8660254037844387076, 1.000000000000000000, 0.8660254037844387076, 1.000000000000000000, 0.8660254037844387076, 1.000000000000000000, 0.8660254037844387076, 1.000000000000000000, 0.8660254037844387076, 1.000000000000000000, 0.8660254037844387076, 1.000000000000000000, 0.8660254037844387076, 1.000000000000000000, 0.8660254037844387076, 1.000000000000000000, 0.8660254037844387076, 1.000000000000000000, 0.8660254037844387076, 1.000000000000000000) ) ) 
 REPRESENTATION_ITEM ( '' )  SURFACE ( )  );
#8541=DIRECTION ( 'NONE',  ( -7.147005652999508048E-36, 5.642372883946980038E-36, 1.000000000000000000 ) ) ;
#8544=EDGE_CURVE ( 'NONE', #17032, #28335, #27572, .T. ) ;
#8545=CARTESIAN_POINT ( 'NONE',  ( 4.763139720814407951, 2.750000000000002665, -97.75000000000000000 ) ) ;
#8547=CARTESIAN_POINT ( 'NONE',  ( 6.000000000000000888, -1.607695154586752384, -89.23066243270261566 ) ) ;
#8548=CARTESIAN_POINT ( 'NONE',  ( 2.775557561562891351E-14, -6.250000000000061284, -113.6830127018922383 ) ) ;
#8549=VERTEX_POINT ( 'NONE', #20724 ) ;
#8550=CARTESIAN_POINT ( 'NONE',  ( 3.464101615137757051, -5.999999999999979572, -123.9136751345947971 ) ) ;
#8552=CARTESIAN_POINT ( 'NONE',  ( -5.412658773652684552, -3.125000000000099920, -55.43301270189226670 ) ) ;
#8556=CARTESIAN_POINT ( 'NONE',  ( 6.000000000000000888, 5.577813053751546416E-15, -177.6636751345948255 ) ) ;
#8558=CARTESIAN_POINT ( 'NONE',  ( 0.000000000000000000, 5.499999999999991118, -162.0000000000000284 ) ) ;
#8560=CYLINDRICAL_SURFACE ( 'NONE', #6861, 6.000000000000000888 ) ;
#8561=CARTESIAN_POINT ( 'NONE',  ( -6.350852961085760029, -1.281975124255709124E-13, -107.6250000000000426 ) ) ;
#8563=CARTESIAN_POINT ( 'NONE',  ( 4.763139720814407951, 2.750000000000002665, -103.7500000000000142 ) ) ;
#8565=CARTESIAN_POINT ( 'NONE',  ( -5.999999999999962697, 3.323446944526963891E-14, -161.9136751345948539 ) ) ;
#8566=CARTESIAN_POINT ( 'NONE',  ( -5.196152422706601826, 2.999999999999975131, -144.9613248654052597 ) ) ;
#8571=ORIENTED_EDGE ( 'NONE', *, *, #2958, .F. ) ;
#8572=CARTESIAN_POINT ( 'NONE',  ( 3.175426480543072749, -5.500000000000105693, -158.1250000000000284 ) ) ;
#8573=CARTESIAN_POINT ( 'NONE',  ( 6.000000000000000888, 1.743066579297358182E-13, -106.5863248654052313 ) ) ;
#8574=CARTESIAN_POINT ( 'NONE',  ( 5.412658773652739619, 3.124999999999988898, -88.31698729810783277 ) ) ;
#8576=VERTEX_POINT ( 'NONE', #30227 ) ;
#8577=CARTESIAN_POINT ( 'NONE',  ( 3.464101615137757051, -5.999999999999979572, -75.33632486540520290 ) ) ;
#8579=VECTOR ( 'NONE', #22361, 1000.000000000000000 ) ;
#8580=CARTESIAN_POINT ( 'NONE',  ( 0.000000000000000000, 5.499999999999991118, -151.5000000000000284 ) ) ;
#8585=CARTESIAN_POINT ( 'NONE',  ( -2.775557561562891351E-14, -5.500000000000115463, -122.2500000000000284 ) ) ;
#8586=EDGE_CURVE ( 'NONE', #14303, #15775, #22681, .T. ) ;
#8588=CARTESIAN_POINT ( 'NONE',  ( 0.000000000000000000, -5.999999999999991118, -57.46132486540523132 ) ) ;
#8589=CARTESIAN_POINT ( 'NONE',  ( -7.216878364870328078, 0.000000000000000000, -123.6919872981078043 ) ) ;
#8590=CARTESIAN_POINT ( 'NONE',  ( -3.608439182435052128, -6.250000000000110134, -180.4419872981078470 ) ) ;
#8591=CARTESIAN_POINT ( 'NONE',  ( -4.763139720814407951, 2.749999999999946709, -175.2500000000000284 ) ) ;
#8594=ORIENTED_EDGE ( 'NONE', *, *, #25054, .F. ) ;
#8597=CARTESIAN_POINT ( 'NONE',  ( -5.999999999999956479, -1.607695154586745057, -55.34668783648704249 ) ) ;
#8598=CARTESIAN_POINT ( 'NONE',  ( 6.000000000000000888, -1.607695154586752384, -46.65331216351298593 ) ) ;
#8600=CARTESIAN_POINT ( 'NONE',  ( -3.608439182435052128, -6.250000000000110134, -70.94198729810781856 ) ) ;
#8601=CARTESIAN_POINT ( 'NONE',  ( 5.412658773652712085, -3.125000000000086153, -55.56698729810782567 ) ) ;
#8602=CARTESIAN_POINT ( 'NONE',  ( 6.000000000000000888, -1.607695154586752384, -170.2306624327026441 ) ) ;
#8603=CARTESIAN_POINT ( 'NONE',  ( -3.175426480542816510, -5.500000000000057732, -50.37500000000001421 ) ) ;
#8604=CARTESIAN_POINT ( 'NONE',  ( 6.000000000000000888, 1.743066579297358182E-13, -48.66367513459482552 ) ) ;
#8605=CARTESIAN_POINT ( 'NONE',  ( -4.763139720814407951, -2.750000000000016431, -130.0000000000000000 ) ) ;
#8610=AXIS2_PLACEMENT_3D ( 'NONE', #4183, #13296, #20182 ) ;
#8616=LINE ( 'NONE', #9344, #1355 ) ;
#8617=CARTESIAN_POINT ( 'NONE',  ( 2.775557561562891351E-14, -6.250000000000061284, -118.8169872981078612 ) ) ;
#8619=AXIS2_PLACEMENT_3D ( 'NONE', #1789, #18564, #14135 ) ;
#8624=ADVANCED_FACE ( 'NONE', ( #1505 ), #10917, .T. ) ;
#8625=ORIENTED_EDGE ( 'NONE', *, *, #19530, .F. ) ;
#8626=VERTEX_POINT ( 'NONE', #17983 ) ;
#8629=CARTESIAN_POINT ( 'NONE',  ( -2.775557561562891351E-14, -5.500000000000115463, -53.25000000000002132 ) ) ;
#8630=( BOUNDED_CURVE ( )  B_SPLINE_CURVE ( 2, ( #21602, #28930, #24187, #12857, #17609, #3279, #19884, #14843, #22197 ),
 .UNSPECIFIED., .F., .F. ) 
 B_SPLINE_CURVE_WITH_KNOTS ( ( 3, 2, 2, 2, 3 ),
 ( 0.04166666666666667129, 0.04259259259259259162, 0.04444444444444444614, 0.04629629629629629373, 0.04722222222222221405 ),
 .UNSPECIFIED. ) 
 CURVE ( )  GEOMETRIC_REPRESENTATION_ITEM ( )  RATIONAL_B_SPLINE_CURVE ( ( 0.9330127018922194093, 0.9330127018922196314, 1.000000000000000000, 0.8660254037844388186, 1.000000000000000000, 0.8660254037844388186, 1.000000000000000000, 0.9330127018922199644, 0.9330127018922194093 ) ) 
 REPRESENTATION_ITEM ( '' )  );
#8633=CARTESIAN_POINT ( 'NONE',  ( 0.000000000000000000, -5.999999999999991118, -79.96132486540518869 ) ) ;
#8634=CARTESIAN_POINT ( 'NONE',  ( 3.608439182435180470, -6.249999999999997335, -65.55801270189225249 ) ) ;
#8637=CARTESIAN_POINT ( 'NONE',  ( 0.000000000000000000, -5.999999999999991118, -178.0386751345948255 ) ) ;
#8641=CARTESIAN_POINT ( 'NONE',  ( 4.763139720814407951, -2.749999999999988454, -134.0000000000000000 ) ) ;
#8642=CARTESIAN_POINT ( 'NONE',  ( -5.412658773652684552, -3.125000000000099920, -148.4330127018922383 ) ) ;
#8646=CARTESIAN_POINT ( 'NONE',  ( 6.350852961086080661, -9.614813431917819062E-14, -60.37500000000000000 ) ) ;
#8650=CIRCLE ( 'NONE', #12606, 6.000000000000009770 ) ;
#8658=EDGE_CURVE ( 'NONE', #567, #8702, #17138, .T. ) ;
#8662=VECTOR ( 'NONE', #23249, 1000.000000000000000 ) ;
#8663=ORIENTED_EDGE ( 'NONE', *, *, #28060, .F. ) ;
#8664=CARTESIAN_POINT ( 'NONE',  ( -4.763139720814407951, -2.750000000000016431, -146.5000000000000284 ) ) ;
#8670=CARTESIAN_POINT ( 'NONE',  ( 3.175426480543072749, 5.499999999999865885, -76.62500000000001421 ) ) ;
#8674=CARTESIAN_POINT ( 'NONE',  ( 6.000000000000000888, 1.743066579297358182E-13, -69.08632486540523132 ) ) ;
#8678=( BOUNDED_CURVE ( )  B_SPLINE_CURVE ( 2, ( #13572, #3841, #22913, #29805, #10956, #22614, #29955, #1853, #17713 ),
 .UNSPECIFIED., .F., .T. ) 
 B_SPLINE_CURVE_WITH_KNOTS ( ( 3, 2, 2, 2, 3 ),
 ( 0.4694444444444444420, 0.4703703703703703276, 0.4722222222222222099, 0.4740740740740740922, 0.4750000000000000888 ),
 .UNSPECIFIED. ) 
 CURVE ( )  GEOMETRIC_REPRESENTATION_ITEM ( )  RATIONAL_B_SPLINE_CURVE ( ( 0.9330127018922194093, 0.9330127018922194093, 1.000000000000000000, 0.8660254037844388186, 1.000000000000000000, 0.8660254037844388186, 1.000000000000000000, 0.9330127018922154125, 0.9330127018922194093 ) ) 
 REPRESENTATION_ITEM ( '' )  );
#8679=CARTESIAN_POINT ( 'NONE',  ( -6.350852961085760029, -1.281975124255709124E-13, -160.1250000000000284 ) ) ;
#8681=CARTESIAN_POINT ( 'NONE',  ( -5.061300234009625143, 3.091548682366505485, -180.0000000000000568 ) ) ;
#8683=CARTESIAN_POINT ( 'NONE',  ( 4.763139720814407951, -2.749999999999988454, -90.50000000000002842 ) ) ;
#8686=CARTESIAN_POINT ( 'NONE',  ( -2.775557561562891351E-14, -5.500000000000115463, -77.25000000000004263 ) ) ;
#8687=DIRECTION ( 'NONE',  ( -7.147005652999508048E-36, 5.642372883946980038E-36, 1.000000000000000000 ) ) ;
#8689=CARTESIAN_POINT ( 'NONE',  ( 0.000000000000000000, 5.999999999999977796, -106.2113248654051887 ) ) ;
#8696=DIRECTION ( 'NONE',  ( 1.000000000000000000, -5.551115123125773458E-17, -1.260129944081490338E-35 ) ) ;
#8702=VERTEX_POINT ( 'NONE', #14883 ) ;
#8703=ADVANCED_FACE ( 'NONE', ( #16760 ), #24224, .T. ) ;
#8704=ORIENTED_EDGE ( 'NONE', *, *, #28675, .T. ) ;
#8705=CARTESIAN_POINT ( 'NONE',  ( 3.175426480543072749, 5.499999999999865885, -97.62500000000004263 ) ) ;
#8709=CARTESIAN_POINT ( 'NONE',  ( -5.412658773652684552, -3.125000000000099920, -113.9330127018922667 ) ) ;
#8711=CARTESIAN_POINT ( 'NONE',  ( -5.999999999999963585, 8.134310703387671600E-14, -140.3363248654052313 ) ) ;
#8713=CARTESIAN_POINT ( 'NONE',  ( 5.999999999999949374, 1.607695154586804565, -52.51933756729741987 ) ) ;
#8714=CARTESIAN_POINT ( 'NONE',  ( -5.412658773652684552, -3.125000000000099920, -53.93301270189220986 ) ) ;
#8715=VERTEX_POINT ( 'NONE', #23792 ) ;
#8718=STYLED_ITEM ( 'NONE', ( #30172 ), #18784 ) ;
#8719=CARTESIAN_POINT ( 'NONE',  ( 3.175426480543072749, 5.499999999999865885, -166.6249999999999716 ) ) ;
#8721=CARTESIAN_POINT ( 'NONE',  ( 0.000000000000000000, -5.999999999999991118, -157.9613248654052597 ) ) ;
#8722=CARTESIAN_POINT ( 'NONE',  ( -4.763139720814407951, 2.749999999999946709, -110.7500000000000142 ) ) ;
#8725=CARTESIAN_POINT ( 'NONE',  ( 4.763139720814407951, -2.749999999999988454, -99.50000000000002842 ) ) ;
#8726=CARTESIAN_POINT ( 'NONE',  ( 3.464101615137757051, -5.999999999999979572, -111.9136751345948113 ) ) ;
#8727=DIRECTION ( 'NONE',  ( -7.147005652999508048E-36, 5.642372883946980038E-36, 1.000000000000000000 ) ) ;
#8728=CARTESIAN_POINT ( 'NONE',  ( 3.464101615137757051, -5.999999999999979572, -81.91367513459479710 ) ) ;
#8729=ORIENTED_EDGE ( 'NONE', *, *, #11968, .F. ) ;
#8735=CARTESIAN_POINT ( 'NONE',  ( 0.000000000000000000, 4.000000000000017764, -180.0000000000000568 ) ) ;
#8736=ORIENTED_EDGE ( 'NONE', *, *, #10027, .F. ) ;
#8738=CARTESIAN_POINT ( 'NONE',  ( -3.608439182435115633, 6.249999999999965361, -86.44198729810783277 ) ) ;
#8739=CARTESIAN_POINT ( 'NONE',  ( -6.000000000000007105, -1.607695154586655129, -103.3466878364870212 ) ) ;
#8741=EDGE_CURVE ( 'NONE', #15355, #4337, #5775, .T. ) ;
#8747=CARTESIAN_POINT ( 'NONE',  ( 0.000000000000000000, 5.499999999999991118, -118.5000000000000568 ) ) ;
#8748=CARTESIAN_POINT ( 'NONE',  ( -5.412658773652684552, -3.125000000000099920, -140.9330127018922383 ) ) ;
#8751=CARTESIAN_POINT ( 'NONE',  ( 3.608439182435180470, -6.249999999999997335, -123.1919872981078043 ) ) ;
#8752=CARTESIAN_POINT ( 'NONE',  ( -7.216878364870328078, 0.000000000000000000, -176.1919872981077901 ) ) ;
#8753=CARTESIAN_POINT ( 'NONE',  ( -6.350852961085760029, -1.281975124255709124E-13, -172.1250000000000284 ) ) ;
#8755=CYLINDRICAL_SURFACE ( 'NONE', #15260, 2.000000000000003109 ) ;
#8756=ORIENTED_EDGE ( 'NONE', *, *, #21609, .F. ) ;
#8758=CARTESIAN_POINT ( 'NONE',  ( 5.196152422706629359, 3.000000000000002665, -148.4613248654052029 ) ) ;
#8760=CARTESIAN_POINT ( 'NONE',  ( 0.000000000000000000, 5.999999999999977796, -171.2886751345948255 ) ) ;
#8763=CARTESIAN_POINT ( 'NONE',  ( 5.412658773652712085, -3.125000000000086153, -75.06698729810784698 ) ) ;
#8764=CARTESIAN_POINT ( 'NONE',  ( -3.608439182435115633, 6.249999999999965361, -59.44198729810781856 ) ) ;
#8766=CARTESIAN_POINT ( 'NONE',  ( 6.350852961086080661, -9.614813431917819062E-14, -48.37500000000000711 ) ) ;
#8767=CARTESIAN_POINT ( 'NONE',  ( -5.999999999999919176, 1.607695154586804565, -102.9033121635129788 ) ) ;
#8768=DIRECTION ( 'NONE',  ( -5.551115123125774074E-17, -1.000000000000000000, -6.394689268473234689E-36 ) ) ;
#8769=CARTESIAN_POINT ( 'NONE',  ( -4.763139720814407951, -2.750000000000016431, -121.0000000000000000 ) ) ;
#8770=CARTESIAN_POINT ( 'NONE',  ( 5.999999999999949374, 1.607695154586804565, -51.01933756729744118 ) ) ;
#8772=CARTESIAN_POINT ( 'NONE',  ( 5.196152422706629359, 3.000000000000002665, -158.0386751345948539 ) ) ;
#8773=EDGE_CURVE ( 'NONE', #15213, #5324, #15057, .T. ) ;
#8774=CARTESIAN_POINT ( 'NONE',  ( 6.000000000000000888, 1.743066579297358182E-13, -69.66367513459482552 ) ) ;
#8775=DIRECTION ( 'NONE',  ( -7.147005652999508048E-36, 5.642372883946980038E-36, 1.000000000000000000 ) ) ;
#8777=LINE ( 'NONE', #1388, #10069 ) ;
#8778=( BOUNDED_CURVE ( )  B_SPLINE_CURVE ( 2, ( #5044, #12724, #14475, #22062, #19075, #24344, #14330, #14184, #19750 ),
 .UNSPECIFIED., .F., .F. ) 
 B_SPLINE_CURVE_WITH_KNOTS ( ( 3, 2, 2, 2, 3 ),
 ( 0.8083333333333333481, 0.8092592592592592338, 0.8111111111111111160, 0.8129629629629629983, 0.8138888888888888840 ),
 .UNSPECIFIED. ) 
 CURVE ( )  GEOMETRIC_REPRESENTATION_ITEM ( )  RATIONAL_B_SPLINE_CURVE ( ( 0.9330127018922194093, 0.9330127018922234061, 1.000000000000000000, 0.8660254037844388186, 1.000000000000000000, 0.8660254037844388186, 1.000000000000000000, 0.9330127018922234061, 0.9330127018922194093 ) ) 
 REPRESENTATION_ITEM ( '' )  );
#8781=DIRECTION ( 'NONE',  ( 1.000000000000000000, -5.551115123125774074E-17, 7.147005652999508048E-36 ) ) ;
#8782=CARTESIAN_POINT ( 'NONE',  ( 3.608439182435180470, 6.249999999999982236, -116.6919872981078328 ) ) ;
#8787=VERTEX_POINT ( 'NONE', #8556 ) ;
#8790=ORIENTED_EDGE ( 'NONE', *, *, #4185, .T. ) ;
#8791=EDGE_LOOP ( 'NONE', ( #18974, #26963, #23991, #7347 ) ) ;
#8793=CARTESIAN_POINT ( 'NONE',  ( -3.175426480542816510, -5.500000000000057732, -47.37500000000000000 ) ) ;
#8796=FACE_OUTER_BOUND ( 'NONE', #19659, .T. ) ;
#8797=CARTESIAN_POINT ( 'NONE',  ( 3.608439182435180470, -6.249999999999997335, -64.05801270189225249 ) ) ;
#8804=CARTESIAN_POINT ( 'NONE',  ( -3.175426480542816066, 5.499999999999865885, -127.3749999999999858 ) ) ;
#8805=CARTESIAN_POINT ( 'NONE',  ( 0.000000000000000000, -5.999999999999991118, -92.53867513459479710 ) ) ;
#8806=CARTESIAN_POINT ( 'NONE',  ( 5.412658773652739619, 3.124999999999988898, -144.6830127018922099 ) ) ;
#8807=CARTESIAN_POINT ( 'NONE',  ( -5.999999999999963585, -1.487416814333745711E-14, -113.9136751345948255 ) ) ;
#8810=CARTESIAN_POINT ( 'NONE',  ( -2.775557561562891351E-14, -5.500000000000115463, -60.75000000000002842 ) ) ;
#8811=CARTESIAN_POINT ( 'NONE',  ( 6.000000000000000888, -1.859271017917181981E-14, -124.5863248654052171 ) ) ;
#8813=EDGE_CURVE ( 'NONE', #25259, #15491, #21525, .T. ) ;
#8814=CARTESIAN_POINT ( 'NONE',  ( 0.000000000000000000, 5.999999999999977796, -170.7113248654052029 ) ) ;
#8815=ORIENTED_EDGE ( 'NONE', *, *, #11716, .T. ) ;
#8820=DIRECTION ( 'NONE',  ( -7.147005652999508048E-36, 5.642372883946980038E-36, 1.000000000000000000 ) ) ;
#8824=( BOUNDED_CURVE ( )  B_SPLINE_CURVE ( 2, ( #23389, #14201, #2337, #13, #9398, #7085, #2477, #23538, #24560 ),
 .UNSPECIFIED., .F., .F. ) 
 B_SPLINE_CURVE_WITH_KNOTS ( ( 3, 2, 2, 2, 3 ),
 ( 0.9250000000000000444, 0.9259259259259259300, 0.9277777777777778123, 0.9296296296296295836, 0.9305555555555555802 ),
 .UNSPECIFIED. ) 
 CURVE ( )  GEOMETRIC_REPRESENTATION_ITEM ( )  RATIONAL_B_SPLINE_CURVE ( ( 0.9330127018922194093, 0.9330127018922234061, 1.000000000000000000, 0.8660254037844388186, 1.000000000000000000, 0.8660254037844388186, 1.000000000000000000, 0.9330127018922154125, 0.9330127018922194093 ) ) 
 REPRESENTATION_ITEM ( '' )  );
#8826=CARTESIAN_POINT ( 'NONE',  ( 4.763139720814407951, -2.749999999999988454, -138.5000000000000000 ) ) ;
#8829=CARTESIAN_POINT ( 'NONE',  ( 3.175426480543072749, -5.500000000000105693, -74.12500000000007105 ) ) ;
#8831=CARTESIAN_POINT ( 'NONE',  ( -0.1999138633143323907, -11.00000000000000711, -19.00000000000000711 ) ) ;
#8832=CARTESIAN_POINT ( 'NONE',  ( -5.999999999999957367, 1.607695154586737507, -149.9806624327026157 ) ) ;
#8834=CARTESIAN_POINT ( 'NONE',  ( -5.999999999999963585, 8.134310703387671600E-14, -121.4136751345948255 ) ) ;
#8835=CARTESIAN_POINT ( 'NONE',  ( 0.000000000000000000, 0.000000000000000000, 0.000000000000000000 ) ) ;
#8837=CARTESIAN_POINT ( 'NONE',  ( 3.175426480543072749, -5.500000000000105693, -159.6250000000000284 ) ) ;
#8840=VECTOR ( 'NONE', #23000, 1000.000000000000000 ) ;
#8841=CARTESIAN_POINT ( 'NONE',  ( 6.350852961086080661, -9.614813431917819062E-14, -84.37500000000004263 ) ) ;
#8843=CARTESIAN_POINT ( 'NONE',  ( 0.000000000000000000, 5.499999999999991118, -70.50000000000000000 ) ) ;
#8844=EDGE_CURVE ( 'NONE', #6568, #25854, #25815, .T. ) ;
#8845=AXIS2_PLACEMENT_3D ( 'NONE', #15705, #20282, #29630 ) ;
#8846=CARTESIAN_POINT ( 'NONE',  ( 5.999999999999897859, 1.607695154586893826, -142.5193375672974128 ) ) ;
#8847=CARTESIAN_POINT ( 'NONE',  ( 3.464101615137757051, -5.999999999999979572, -174.9136751345948539 ) ) ;
#8849=CARTESIAN_POINT ( 'NONE',  ( 6.000000000000014211, -1.607695154586730180, -149.2306624327026441 ) ) ;
#8851=CARTESIAN_POINT ( 'NONE',  ( 0.000000000000000000, 5.999999999999977796, -118.7886751345948397 ) ) ;
#8853=CARTESIAN_POINT ( 'NONE',  ( -5.196152422706601826, 2.999999999999975131, -169.5386751345948539 ) ) ;
#8854=ORIENTED_EDGE ( 'NONE', *, *, #1861, .T. ) ;
#8856=DIRECTION ( 'NONE',  ( -7.147005652999508048E-36, 5.642372883946980038E-36, 1.000000000000000000 ) ) ;
#8858=CARTESIAN_POINT ( 'NONE',  ( 5.196152422706629359, 3.000000000000002665, -157.4613248654052029 ) ) ;
#8860=ORIENTED_EDGE ( 'NONE', *, *, #11015, .F. ) ;
#8863=CARTESIAN_POINT ( 'NONE',  ( -3.175426480542816510, 5.499999999999865885, -97.37499999999998579 ) ) ;
#8865=FACE_OUTER_BOUND ( 'NONE', #26, .T. ) ;
#8866=CARTESIAN_POINT ( 'NONE',  ( -7.216878364870328078, 0.000000000000000000, -111.0580127018922241 ) ) ;
#8867=CARTESIAN_POINT ( 'NONE',  ( 0.8029667472979687970, 10.97248951867538125, -19.05056182979571133 ) ) ;
#8869=EDGE_CURVE ( 'NONE', #24823, #14484, #15358, .T. ) ;
#8871=ORIENTED_EDGE ( 'NONE', *, *, #25362, .F. ) ;
#8872=CARTESIAN_POINT ( 'NONE',  ( -3.464101615137725076, 5.999999999999979572, -153.1636751345947971 ) ) ;
#8875=CARTESIAN_POINT ( 'NONE',  ( -6.350852961085760029, -1.281975124255709124E-13, -163.1249999999999716 ) ) ;
#8877=CARTESIAN_POINT ( 'NONE',  ( 6.350852961086080661, -9.614813431917819062E-14, -105.3750000000000426 ) ) ;
#8878=LINE ( 'NONE', #3478, #19310 ) ;
#8879=CARTESIAN_POINT ( 'NONE',  ( -5.196152422706573404, -3.000000000000002665, -122.7886751345948539 ) ) ;
#8880=CARTESIAN_POINT ( 'NONE',  ( 3.175426480543072749, -5.500000000000105693, -99.62500000000007105 ) ) ;
#8889=ORIENTED_EDGE ( 'NONE', *, *, #18932, .T. ) ;
#8890=CARTESIAN_POINT ( 'NONE',  ( -3.464101615137725076, 5.999999999999979572, -112.0863248654051887 ) ) ;
#8891=CARTESIAN_POINT ( 'NONE',  ( 5.412658773652739619, 3.124999999999988898, -86.81698729810783277 ) ) ;
#8893=CARTESIAN_POINT ( 'NONE',  ( 0.000000000000000000, -5.999999999999991118, -65.53867513459482552 ) ) ;
#8898=CARTESIAN_POINT ( 'NONE',  ( -4.763139720814407951, -2.750000000000016431, -121.0000000000000000 ) ) ;
#8900=CARTESIAN_POINT ( 'NONE',  ( -5.412658773652739619, 3.124999999999975131, -132.1830127018922667 ) ) ;
#8903=CARTESIAN_POINT ( 'NONE',  ( 3.608439182435180470, 6.249999999999982236, -124.1919872981078043 ) ) ;
#8904=CARTESIAN_POINT ( 'NONE',  ( -3.608439182435052128, -6.250000000000110134, -175.9419872981078754 ) ) ;
#8908=EDGE_CURVE ( 'NONE', #12739, #27786, #13058, .T. ) ;
#8909=EDGE_LOOP ( 'NONE', ( #12577, #26661, #1558, #238 ) ) ;
#8913=AXIS2_PLACEMENT_3D ( 'NONE', #24157, #12371, #10043 ) ;
#8915=CARTESIAN_POINT ( 'NONE',  ( -3.608439182435115633, 6.249999999999965361, -74.44198729810783277 ) ) ;
#8916=CARTESIAN_POINT ( 'NONE',  ( 5.412658773652712085, -3.125000000000086153, -63.06698729810783277 ) ) ;
#8918=CARTESIAN_POINT ( 'NONE',  ( 3.175426480543072749, -5.500000000000105693, -47.12500000000006395 ) ) ;
#8920=CARTESIAN_POINT ( 'NONE',  ( 3.464101615137757051, -5.999999999999979572, -123.3363248654051745 ) ) ;
#8922=CARTESIAN_POINT ( 'NONE',  ( -6.350852961085760029, -1.281975124255709124E-13, -122.6250000000000426 ) ) ;
#8923=CARTESIAN_POINT ( 'NONE',  ( -5.999999999999963585, 8.134310703387671600E-14, -145.4136751345948539 ) ) ;
#8924=ORIENTED_EDGE ( 'NONE', *, *, #23918, .F. ) ;
#8929=CARTESIAN_POINT ( 'NONE',  ( 5.196152422706629359, -2.999999999999988898, -147.7886751345948255 ) ) ;
#8932=CARTESIAN_POINT ( 'NONE',  ( -5.999999999999944933, 1.607695154586759934, -121.4806624327025872 ) ) ;
#8934=CARTESIAN_POINT ( 'NONE',  ( -7.216878364870328078, 0.000000000000000000, -113.1919872981078186 ) ) ;
#8939=VERTEX_POINT ( 'NONE', #27732 ) ;
#8940=CARTESIAN_POINT ( 'NONE',  ( 6.000000000000000888, -3.330669073875464691E-16, -7.560779664488942560E-35 ) ) ;
#8942=CARTESIAN_POINT ( 'NONE',  ( 2.775557561562891351E-14, 6.250000000000033751, -143.5669872981077901 ) ) ;
#8943=AXIS2_PLACEMENT_3D ( 'NONE', #13706, #11395, #4438 ) ;
#8944=CARTESIAN_POINT ( 'NONE',  ( 2.775557561562891351E-14, -11.00000000000001066, -31.00000000000002842 ) ) ;
#8947=CARTESIAN_POINT ( 'NONE',  ( -5.999999999999963585, 8.134310703387671600E-14, -119.9136751345948397 ) ) ;
#8948=CARTESIAN_POINT ( 'NONE',  ( -3.608439182435115633, 6.249999999999965361, -70.80801270189222407 ) ) ;
#8952=CARTESIAN_POINT ( 'NONE',  ( -5.196152422706601826, 2.999999999999975131, -73.53867513459483973 ) ) ;
#8958=CARTESIAN_POINT ( 'NONE',  ( 6.350852961086080661, -9.614813431917819062E-14, -127.8749999999999858 ) ) ;
#8959=CARTESIAN_POINT ( 'NONE',  ( 2.775557561562891351E-14, -6.250000000000061284, -145.1830127018922667 ) ) ;
#8962=CIRCLE ( 'NONE', #27556, 11.00000000000001599 ) ;
#8963=CARTESIAN_POINT ( 'NONE',  ( 6.350852961086080661, -9.614813431917819062E-14, -52.87500000000002842 ) ) ;
#8965=CARTESIAN_POINT ( 'NONE',  ( 0.000000000000000000, 0.000000000000000000, 0.000000000000000000 ) ) ;
#8966=LINE ( 'NONE', #30147, #28781 ) ;
#8967=ORIENTED_EDGE ( 'NONE', *, *, #716, .T. ) ;
#8971=LINE ( 'NONE', #11613, #21963 ) ;
#8972=EDGE_LOOP ( 'NONE', ( #8258, #2091, #26561, #28027 ) ) ;
#8973=CARTESIAN_POINT ( 'NONE',  ( 6.350852961086080661, -9.614813431917819062E-14, -135.3750000000000284 ) ) ;
#8975=VERTEX_POINT ( 'NONE', #4848 ) ;
#8976=CARTESIAN_POINT ( 'NONE',  ( 4.763139720814407951, 2.750000000000002665, -69.25000000000002842 ) ) ;
#8977=ADVANCED_FACE ( 'NONE', ( #6711 ), #4701, .T. ) ;
#8980=ORIENTED_EDGE ( 'NONE', *, *, #9084, .T. ) ;
#8982=CARTESIAN_POINT ( 'NONE',  ( -5.196152422706573404, -3.000000000000002665, -83.78867513459481131 ) ) ;
#8985=CARTESIAN_POINT ( 'NONE',  ( 4.763139720814407951, -2.749999999999988454, -150.5000000000000284 ) ) ;
#8986=DIRECTION ( 'NONE',  ( -7.147005652999508048E-36, 5.642372883946980038E-36, 1.000000000000000000 ) ) ;
#8987=CARTESIAN_POINT ( 'NONE',  ( -4.763139720814407951, -2.750000000000016431, -142.0000000000000284 ) ) ;
#8988=CARTESIAN_POINT ( 'NONE',  ( 2.775557561562891351E-14, 6.250000000000033751, -157.9330127018922383 ) ) ;
#8991=CARTESIAN_POINT ( 'NONE',  ( 3.175426480543072749, 5.499999999999865885, -76.62500000000001421 ) ) ;
#8993=CARTESIAN_POINT ( 'NONE',  ( 3.175426480543072749, 5.499999999999865885, -70.62500000000004263 ) ) ;
#8994=VECTOR ( 'NONE', #3071, 1000.000000000000000 ) ;
#8995=CARTESIAN_POINT ( 'NONE',  ( -5.196152422706573404, -3.000000000000002665, -74.78867513459486815 ) ) ;
#8998=CARTESIAN_POINT ( 'NONE',  ( 3.464101615137757051, -5.999999999999979572, -75.91367513459483973 ) ) ;
#9001=( BOUNDED_CURVE ( )  B_SPLINE_CURVE ( 2, ( #10049, #19428, #28905, #28755, #3251, #7724, #22017, #22173, #17429 ),
 .UNSPECIFIED., .F., .F. ) 
 B_SPLINE_CURVE_WITH_KNOTS ( ( 3, 2, 2, 2, 3 ),
 ( 0.1527777777777777901, 0.1537037037037036757, 0.1555555555555555580, 0.1574074074074074403, 0.1583333333333333259 ),
 .UNSPECIFIED. ) 
 CURVE ( )  GEOMETRIC_REPRESENTATION_ITEM ( )  RATIONAL_B_SPLINE_CURVE ( ( 0.9330127018922194093, 0.9330127018922194093, 1.000000000000000000, 0.8660254037844388186, 1.000000000000000000, 0.8660254037844388186, 1.000000000000000000, 0.9330127018922194093, 0.9330127018922194093 ) ) 
 REPRESENTATION_ITEM ( '' )  );
#9004=ORIENTED_EDGE ( 'NONE', *, *, #27026, .F. ) ;
#9008=ORIENTED_EDGE ( 'NONE', *, *, #6509, .F. ) ;
#9010=ORIENTED_EDGE ( 'NONE', *, *, #16133, .T. ) ;
#9011=CARTESIAN_POINT ( 'NONE',  ( -4.763139720814407951, -2.750000000000016431, -95.50000000000002842 ) ) ;
#9013=CARTESIAN_POINT ( 'NONE',  ( 2.775557561562891351E-14, 6.250000000000033751, -105.4330127018922525 ) ) ;
#9014=ORIENTED_EDGE ( 'NONE', *, *, #2191, .F. ) ;
#9015=DIRECTION ( 'NONE',  ( -7.147005652999508048E-36, 5.642372883946980038E-36, 1.000000000000000000 ) ) ;
#9018=CARTESIAN_POINT ( 'NONE',  ( 2.691259848637810315, -10.67213569177517485, -30.37695071776536793 ) ) ;
#9021=CARTESIAN_POINT ( 'NONE',  ( 0.000000000000000000, 5.499999999999991118, -175.5000000000000000 ) ) ;
#9023=CARTESIAN_POINT ( 'NONE',  ( -3.175426480542816510, 5.499999999999865885, -164.8750000000000568 ) ) ;
#9025=CARTESIAN_POINT ( 'NONE',  ( -3.175426480542816066, -5.500000000000057732, -108.8750000000000426 ) ) ;
#9027=CARTESIAN_POINT ( 'NONE',  ( 5.196152422706629359, -2.999999999999988898, -122.2886751345948539 ) ) ;
#9028=CARTESIAN_POINT ( 'NONE',  ( 3.175426480543072749, -5.500000000000105693, -93.62500000000002842 ) ) ;
#9034=CARTESIAN_POINT ( 'NONE',  ( -5.999999999999962697, 3.323446944526963891E-14, -161.9136751345948539 ) ) ;
#9036=CARTESIAN_POINT ( 'NONE',  ( -5.999999999999964473, 9.063946212346262433E-15, -173.9136751345948255 ) ) ;
#9037=( BOUNDED_CURVE ( )  B_SPLINE_CURVE ( 2, ( #28385, #11712, #9680, #4598, #6906, #16625, #21209, #14029, #27781 ),
 .UNSPECIFIED., .F., .T. ) 
 B_SPLINE_CURVE_WITH_KNOTS ( ( 3, 2, 2, 2, 3 ),
 ( 0.8861111111111110716, 0.8870370370370370683, 0.8888888888888888395, 0.8907407407407407218, 0.8916666666666666075 ),
 .UNSPECIFIED. ) 
 CURVE ( )  GEOMETRIC_REPRESENTATION_ITEM ( )  RATIONAL_B_SPLINE_CURVE ( ( 0.9330127018922194093, 0.9330127018922154125, 1.000000000000000000, 0.8660254037844388186, 1.000000000000000000, 0.8660254037844388186, 1.000000000000000000, 0.9330127018922234061, 0.9330127018922194093 ) ) 
 REPRESENTATION_ITEM ( '' )  );
#9039=EDGE_CURVE ( 'NONE', #11924, #21660, #4557, .T. ) ;
#9040=CARTESIAN_POINT ( 'NONE',  ( 5.412658773652712085, -3.125000000000086153, -90.06698729810780435 ) ) ;
#9042=CARTESIAN_POINT ( 'NONE',  ( 6.000000000000052403, -1.607695154586662678, -65.23066243270255882 ) ) ;
#9043=ORIENTED_EDGE ( 'NONE', *, *, #9291, .T. ) ;
#9046=CARTESIAN_POINT ( 'NONE',  ( 6.350852961086080661, -9.614813431917819062E-14, -124.8749999999999858 ) ) ;
#9049=CARTESIAN_POINT ( 'NONE',  ( -7.216878364870328078, 0.000000000000000000, -127.5580127018922241 ) ) ;
#9050=ORIENTED_EDGE ( 'NONE', *, *, #29771, .T. ) ;
#9051=DIRECTION ( 'NONE',  ( 1.000000000000000000, -5.551115123125773458E-17, -1.260129944081490338E-35 ) ) ;
#9052=CARTESIAN_POINT ( 'NONE',  ( 5.412658773652739619, 3.124999999999988898, -170.8169872981077901 ) ) ;
#9053=CARTESIAN_POINT ( 'NONE',  ( -5.412658773652739619, 3.124999999999975131, -173.3169872981078470 ) ) ;
#9055=DIRECTION ( 'NONE',  ( -7.147005652999508048E-36, 5.642372883946980038E-36, 1.000000000000000000 ) ) ;
#9060=CARTESIAN_POINT ( 'NONE',  ( 2.775557561562891351E-14, -6.250000000000061284, -73.81698729810781856 ) ) ;
#9061=CARTESIAN_POINT ( 'NONE',  ( -5.412658773652739619, 3.124999999999975131, -63.81698729810780435 ) ) ;
#9062=CARTESIAN_POINT ( 'NONE',  ( -3.175426480542816510, 5.499999999999865885, -49.37500000000000711 ) ) ;
#9064=CARTESIAN_POINT ( 'NONE',  ( 5.196152422706629359, -2.999999999999988898, -123.2113248654052029 ) ) ;
#9066=CARTESIAN_POINT ( 'NONE',  ( -2.775557561562891351E-14, -5.500000000000115463, -117.7500000000000284 ) ) ;
#9068=VERTEX_POINT ( 'NONE', #25434 ) ;
#9071=CARTESIAN_POINT ( 'NONE',  ( 6.000000000000000888, -3.330669073875464691E-16, -7.560779664488942560E-35 ) ) ;
#9072=VERTEX_POINT ( 'NONE', #20702 ) ;
#9074=CARTESIAN_POINT ( 'NONE',  ( 0.000000000000000000, 5.999999999999977796, -121.7886751345948539 ) ) ;
#9077=CARTESIAN_POINT ( 'NONE',  ( -5.412658773652684552, -3.125000000000099920, -110.0669872981078186 ) ) ;
#9078=CARTESIAN_POINT ( 'NONE',  ( 5.999999999999949374, 1.607695154586804565, -108.5966878364870496 ) ) ;
#9080=ORIENTED_EDGE ( 'NONE', *, *, #27707, .T. ) ;
#9084=EDGE_CURVE ( 'NONE', #2061, #7050, #13823, .T. ) ;
#9085=AXIS2_PLACEMENT_3D ( 'NONE', #646, #10030, #19407 ) ;
#9086=CARTESIAN_POINT ( 'NONE',  ( -5.412658773652684552, -3.125000000000099920, -140.0669872981078470 ) ) ;
#9087=CARTESIAN_POINT ( 'NONE',  ( -5.196152422706601826, 2.999999999999975131, -150.9613248654052597 ) ) ;
#9090=CARTESIAN_POINT ( 'NONE',  ( 0.000000000000000000, -5.999999999999991118, -137.5386751345948255 ) ) ;
#9091=CARTESIAN_POINT ( 'NONE',  ( 5.412658773652739619, 3.124999999999988898, -68.18301270189225249 ) ) ;
#9094=CARTESIAN_POINT ( 'NONE',  ( 3.464101615137852974, 5.999999999999884537, -73.91367513459483973 ) ) ;
#9095=CARTESIAN_POINT ( 'NONE',  ( 3.464101615137852974, 5.999999999999884537, -165.4136751345947687 ) ) ;
#9099=DIRECTION ( 'NONE',  ( -7.147005652999508048E-36, 5.642372883946980038E-36, 1.000000000000000000 ) ) ;
#9100=CARTESIAN_POINT ( 'NONE',  ( -6.350852961085760029, -1.281975124255709124E-13, -127.1249999999999858 ) ) ;
#9101=CARTESIAN_POINT ( 'NONE',  ( -5.999999999999963585, 1.780251999655701777E-13, -53.33632486540522422 ) ) ;
#9102=CARTESIAN_POINT ( 'NONE',  ( -7.216878364870328078, 0.000000000000000000, -142.5580127018922667 ) ) ;
#9104=CARTESIAN_POINT ( 'NONE',  ( 0.000000000000000000, 0.000000000000000000, 0.000000000000000000 ) ) ;
#9106=CARTESIAN_POINT ( 'NONE',  ( 4.763139720814407951, 2.750000000000002665, -51.25000000000001421 ) ) ;
#9114=EDGE_CURVE ( 'NONE', #14484, #20574, #4632, .T. ) ;
#9117=CIRCLE ( 'NONE', #12564, 0.9999999999999991118 ) ;
#9119=CARTESIAN_POINT ( 'NONE',  ( 4.763139720814407951, 2.750000000000002665, -135.2500000000000284 ) ) ;
#9122=ORIENTED_EDGE ( 'NONE', *, *, #4067, .F. ) ;
#9123=CARTESIAN_POINT ( 'NONE',  ( 0.000000000000000000, 5.499999999999991118, -66.00000000000000000 ) ) ;
#9125=( BOUNDED_CURVE ( )  B_SPLINE_CURVE ( 2, ( #1065, #3061, #12779, #19524, #3201, #21824, #28858, #10454, #26847 ),
 .UNSPECIFIED., .F., .T. ) 
 B_SPLINE_CURVE_WITH_KNOTS ( ( 3, 2, 2, 2, 3 ),
 ( 0.9750000000000000888, 0.9759259259259259744, 0.9777777777777777457, 0.9796296296296296280, 0.9805555555555555136 ),
 .UNSPECIFIED. ) 
 CURVE ( )  GEOMETRIC_REPRESENTATION_ITEM ( )  RATIONAL_B_SPLINE_CURVE ( ( 0.9330127018922194093, 0.9330127018922234061, 1.000000000000000000, 0.8660254037844388186, 1.000000000000000000, 0.8660254037844388186, 1.000000000000000000, 0.9330127018922234061, 0.9330127018922194093 ) ) 
 REPRESENTATION_ITEM ( '' )  );
#9126=EDGE_LOOP ( 'NONE', ( #2017, #13123, #12746, #15508 ) ) ;
#9127=CARTESIAN_POINT ( 'NONE',  ( -5.999999999999963585, 1.780251999655701777E-13, -57.83632486540521711 ) ) ;
#9129=CARTESIAN_POINT ( 'NONE',  ( 5.999999999999988454, 1.607695154586737729, -150.5966878364870638 ) ) ;
#9132=CARTESIAN_POINT ( 'NONE',  ( -2.775557561562891351E-14, -5.500000000000115463, -146.2500000000000000 ) ) ;
#9134=CARTESIAN_POINT ( 'NONE',  ( 3.175426480543072749, 5.499999999999865885, -142.6250000000000000 ) ) ;
#9135=CARTESIAN_POINT ( 'NONE',  ( 5.412658773652739619, 3.124999999999988898, -162.6830127018922383 ) ) ;
#9136=CARTESIAN_POINT ( 'NONE',  ( 20.99177011976446749, 10.49588505988222842, 1.500282997124228146E-34 ) ) ;
#9137=CARTESIAN_POINT ( 'NONE',  ( 5.196152422706629359, 3.000000000000002665, -89.96132486540520290 ) ) ;
#9138=VECTOR ( 'NONE', #17735, 1000.000000000000000 ) ;
#9139=CARTESIAN_POINT ( 'NONE',  ( -3.175426480542816066, -5.500000000000057732, -75.87500000000001421 ) ) ;
#9141=CARTESIAN_POINT ( 'NONE',  ( -2.775557561562891351E-14, -5.500000000000115463, -74.25000000000004263 ) ) ;
#9143=CARTESIAN_POINT ( 'NONE',  ( -5.196152422706573404, -3.000000000000002665, -88.28867513459482552 ) ) ;
#9148=CARTESIAN_POINT ( 'NONE',  ( 5.999999999999949374, 1.607695154586804565, -95.09668783648706381 ) ) ;
#9151=EDGE_CURVE ( 'NONE', #23842, #30226, #4809, .T. ) ;
#9152=VERTEX_POINT ( 'NONE', #840 ) ;
#9154=CARTESIAN_POINT ( 'NONE',  ( 3.464101615137757051, -5.999999999999979572, -156.9136751345947971 ) ) ;
#9158=ORIENTED_EDGE ( 'NONE', *, *, #12894, .F. ) ;
#9160=CARTESIAN_POINT ( 'NONE',  ( -6.350852961085760029, -1.281975124255709124E-13, -88.12500000000000000 ) ) ;
#9161=CARTESIAN_POINT ( 'NONE',  ( 2.775557561562891351E-14, 6.250000000000033751, -108.4330127018922099 ) ) ;
#9162=VERTEX_POINT ( 'NONE', #19160 ) ;
#9163=CARTESIAN_POINT ( 'NONE',  ( 3.979146954363714350, 10.25926384964410509, -20.49296196285818894 ) ) ;
#9164=CARTESIAN_POINT ( 'NONE',  ( 6.000000000000000888, -3.330669073875464691E-16, -7.560779664488942560E-35 ) ) ;
#9165=CARTESIAN_POINT ( 'NONE',  ( 5.959171229995800623, -9.246457381727758218, -25.80348449789765297 ) ) ;
#9167=DIRECTION ( 'NONE',  ( 1.000000000000000000, -5.551115123125773458E-17, -1.260129944081490338E-35 ) ) ;
#9168=CARTESIAN_POINT ( 'NONE',  ( 0.000000000000000000, 5.499999999999991118, -169.4999999999999716 ) ) ;
#9170=CARTESIAN_POINT ( 'NONE',  ( 4.763139720814407951, -2.749999999999988454, -165.4999999999999716 ) ) ;
#9173=CARTESIAN_POINT ( 'NONE',  ( -6.350852961085760029, -1.281975124255709124E-13, -100.1250000000000568 ) ) ;
#9174=CARTESIAN_POINT ( 'NONE',  ( 3.464101615137757051, -5.999999999999979572, -165.9136751345947403 ) ) ;
#9175=CARTESIAN_POINT ( 'NONE',  ( 6.350852961086080661, -9.614813431917819062E-14, -100.8750000000000000 ) ) ;
#9179=CIRCLE ( 'NONE', #13646, 11.00000000000001599 ) ;
#9183=CARTESIAN_POINT ( 'NONE',  ( 3.464101615137852974, 5.999999999999884537, -130.3363248654052029 ) ) ;
#9191=CARTESIAN_POINT ( 'NONE',  ( 6.000000000000052403, -1.607695154586662678, -75.15331216351297883 ) ) ;
#9195=CARTESIAN_POINT ( 'NONE',  ( -4.763139720814407951, -2.750000000000016431, -111.9999999999999858 ) ) ;
#9197=CARTESIAN_POINT ( 'NONE',  ( 3.608439182435180470, -6.249999999999997335, -133.0580127018922667 ) ) ;
#9199=DIRECTION ( 'NONE',  ( -7.147005652999508048E-36, 5.642372883946980038E-36, 1.000000000000000000 ) ) ;
#9200=CARTESIAN_POINT ( 'NONE',  ( 3.608439182435180470, -6.249999999999997335, -168.1919872981078470 ) ) ;
#9201=CARTESIAN_POINT ( 'NONE',  ( -3.608439182435052128, -6.250000000000110134, -178.9419872981078470 ) ) ;
#9202=VECTOR ( 'NONE', #10748, 1000.000000000000000 ) ;
#9203=CARTESIAN_POINT ( 'NONE',  ( 0.000000000000000000, 0.000000000000000000, 0.000000000000000000 ) ) ;
#9204=ORIENTED_EDGE ( 'NONE', *, *, #5209, .T. ) ;
#9206=CARTESIAN_POINT ( 'NONE',  ( -5.999999999999963585, -1.487416814333745711E-14, -128.9136751345948539 ) ) ;
#9211=CARTESIAN_POINT ( 'NONE',  ( 2.775557561562891351E-14, 6.250000000000033751, -73.06698729810784698 ) ) ;
#9212=CARTESIAN_POINT ( 'NONE',  ( -5.412658773652684552, -3.125000000000099920, -63.56698729810783277 ) ) ;
#9213=EDGE_CURVE ( 'NONE', #14750, #891, #21335, .T. ) ;
#9214=CARTESIAN_POINT ( 'NONE',  ( 3.175426480543072749, 5.499999999999865885, -49.62500000000001421 ) ) ;
#9218=( BOUNDED_CURVE ( )  B_SPLINE_CURVE ( 2, ( #26792, #5756, #24503, #1932, #30188, #9154, #18547, #11338, #23453 ),
 .UNSPECIFIED., .F., .T. ) 
 B_SPLINE_CURVE_WITH_KNOTS ( ( 3, 2, 2, 2, 3 ),
 ( 0.1805555555555555525, 0.1814814814814814936, 0.1833333333333333204, 0.1851851851851851749, 0.1861111111111111160 ),
 .UNSPECIFIED. ) 
 CURVE ( )  GEOMETRIC_REPRESENTATION_ITEM ( )  RATIONAL_B_SPLINE_CURVE ( ( 0.9330127018922196314, 0.9330127018922185211, 1.000000000000000000, 0.8660254037844388186, 1.000000000000000000, 0.8660254037844388186, 1.000000000000000000, 0.9330127018922184101, 0.9330127018922194093 ) ) 
 REPRESENTATION_ITEM ( '' )  );
#9219=CARTESIAN_POINT ( 'NONE',  ( 4.763139720814407951, -2.749999999999988454, -123.5000000000000568 ) ) ;
#9223=EDGE_CURVE ( 'NONE', #28281, #1984, #1483, .T. ) ;
#9227=CARTESIAN_POINT ( 'NONE',  ( 3.464101615137757051, -5.999999999999979572, -114.9136751345948255 ) ) ;
#9228=CARTESIAN_POINT ( 'NONE',  ( -3.608439182435115633, 6.249999999999965361, -108.9419872981077901 ) ) ;
#9229=CARTESIAN_POINT ( 'NONE',  ( -5.999999999999962697, 3.323446944526963891E-14, -158.3363248654052313 ) ) ;
#9231=ORIENTED_EDGE ( 'NONE', *, *, #29804, .T. ) ;
#9232=CARTESIAN_POINT ( 'NONE',  ( -5.196152422706573404, -3.000000000000002665, -142.2886751345948539 ) ) ;
#9234=ORIENTED_EDGE ( 'NONE', *, *, #28099, .F. ) ;
#9235=CARTESIAN_POINT ( 'NONE',  ( 2.775557561562891351E-14, 6.250000000000033751, -136.0669872981078470 ) ) ;
#9237=CARTESIAN_POINT ( 'NONE',  ( 6.000000000000000888, -1.859271017917181981E-14, -93.08632486540523132 ) ) ;
#9240=CARTESIAN_POINT ( 'NONE',  ( 3.608439182435180470, 6.249999999999982236, -68.05801270189226670 ) ) ;
#9246=ADVANCED_FACE ( 'NONE', ( #10537 ), #6062, .T. ) ;
#9250=CARTESIAN_POINT ( 'NONE',  ( 6.000000000000000888, 1.743066579297358182E-13, -94.58632486540521711 ) ) ;
#9251=CARTESIAN_POINT ( 'NONE',  ( 4.763139720814407951, 2.750000000000002665, -123.2500000000000284 ) ) ;
#9253=CARTESIAN_POINT ( 'NONE',  ( -3.608439182435052128, -6.250000000000110134, -143.8080127018922667 ) ) ;
#9254=CARTESIAN_POINT ( 'NONE',  ( -5.196152422706601826, 2.999999999999975131, -148.5386751345948539 ) ) ;
#9255=LINE ( 'NONE', #18650, #16137 ) ;
#9257=CARTESIAN_POINT ( 'NONE',  ( 3.175426480543072749, -5.500000000000105693, -56.12500000000004263 ) ) ;
#9258=CARTESIAN_POINT ( 'NONE',  ( 3.464101615137757051, -5.999999999999979572, -154.8363248654052029 ) ) ;
#9260=CARTESIAN_POINT ( 'NONE',  ( -3.464101615137725076, 5.999999999999979572, -121.0863248654051461 ) ) ;
#9261=EDGE_CURVE ( 'NONE', #15213, #899, #3433, .T. ) ;
#9263=EDGE_LOOP ( 'NONE', ( #8223, #6965, #28842, #28387 ) ) ;
#9266=CARTESIAN_POINT ( 'NONE',  ( 3.608439182435180470, 6.249999999999982236, -106.1919872981078612 ) ) ;
#9269=CYLINDRICAL_SURFACE ( 'NONE', #18046, 6.000000000000000888 ) ;
#9270=CARTESIAN_POINT ( 'NONE',  ( 3.175426480543072749, 5.499999999999865885, -139.6250000000000000 ) ) ;
#9271=VERTEX_POINT ( 'NONE', #8199 ) ;
#9273=ORIENTED_EDGE ( 'NONE', *, *, #29373, .T. ) ;
#9274=CARTESIAN_POINT ( 'NONE',  ( 4.763139720814407951, -2.749999999999988454, -65.00000000000000000 ) ) ;
#9275=DIRECTION ( 'NONE',  ( -7.147005652999508048E-36, 5.642372883946980038E-36, 1.000000000000000000 ) ) ;
#9276=CARTESIAN_POINT ( 'NONE',  ( 5.196152422706629359, -2.999999999999988898, -123.7886751345948539 ) ) ;
#9277=VERTEX_POINT ( 'NONE', #27243 ) ;
#9281=CARTESIAN_POINT ( 'NONE',  ( 0.000000000000000000, 0.000000000000000000, 0.000000000000000000 ) ) ;
#9283=CARTESIAN_POINT ( 'NONE',  ( 0.000000000000000000, 5.499999999999991118, -148.5000000000000284 ) ) ;
#9285=CARTESIAN_POINT ( 'NONE',  ( 0.000000000000000000, 5.499999999999991118, -135.0000000000000000 ) ) ;
#9286=CARTESIAN_POINT ( 'NONE',  ( -3.608439182435115633, 6.249999999999965361, -163.8080127018922667 ) ) ;
#9287=CARTESIAN_POINT ( 'NONE',  ( 20.99177011976446394, -10.49588505988223730, 2.684716942222302368E-34 ) ) ;
#9288=CARTESIAN_POINT ( 'NONE',  ( 0.000000000000000000, 5.999999999999977796, -89.71132486540523132 ) ) ;
#9289=CARTESIAN_POINT ( 'NONE',  ( -6.350852961085760029, -1.281975124255709124E-13, -79.12500000000001421 ) ) ;
#9290=CARTESIAN_POINT ( 'NONE',  ( -6.000000000000023093, 1.607695154586625819, -173.4033121635129646 ) ) ;
#9291=EDGE_CURVE ( 'NONE', #856, #18552, #94, .T. ) ;
#9292=CARTESIAN_POINT ( 'NONE',  ( -3.175426480542816510, -5.500000000000057732, -66.87500000000002842 ) ) ;
#9293=EDGE_CURVE ( 'NONE', #25418, #18127, #22203, .T. ) ;
#9296=FACE_OUTER_BOUND ( 'NONE', #23818, .T. ) ;
#9300=CARTESIAN_POINT ( 'NONE',  ( -5.999999999999919176, 1.607695154586804565, -94.48066243270258724 ) ) ;
#9304=( BOUNDED_CURVE ( )  B_SPLINE_CURVE ( 2, ( #7397, #4921, #28268, #24123, #21690, #179, #2773, #23837, #23692 ),
 .UNSPECIFIED., .F., .F. ) 
 B_SPLINE_CURVE_WITH_KNOTS ( ( 3, 2, 2, 2, 3 ),
 ( 0.7416666666666666963, 0.7425925925925925819, 0.7444444444444444642, 0.7462962962962962354, 0.7472222222222222321 ),
 .UNSPECIFIED. ) 
 CURVE ( )  GEOMETRIC_REPRESENTATION_ITEM ( )  RATIONAL_B_SPLINE_CURVE ( ( 0.9330127018922194093, 0.9330127018922234061, 1.000000000000000000, 0.8660254037844388186, 1.000000000000000000, 0.8660254037844388186, 1.000000000000000000, 0.9330127018922194093, 0.9330127018922194093 ) ) 
 REPRESENTATION_ITEM ( '' )  );
#9305=EDGE_LOOP ( 'NONE', ( #309, #10357, #2403, #1728 ) ) ;
#9310=CYLINDRICAL_SURFACE ( 'NONE', #13653, 6.000000000000000888 ) ;
#9312=ORIENTED_EDGE ( 'NONE', *, *, #18397, .T. ) ;
#9313=( BOUNDED_CURVE ( )  B_SPLINE_CURVE ( 2, ( #7970, #12332, #12937, #24555, #29005, #17232, #17533, #29313, #22273 ),
 .UNSPECIFIED., .F., .T. ) 
 B_SPLINE_CURVE_WITH_KNOTS ( ( 3, 2, 2, 2, 3 ),
 ( 0.1027777777777777735, 0.1037037037037037007, 0.1055555555555555552, 0.1074074074074074098, 0.1083333333333333370 ),
 .UNSPECIFIED. ) 
 CURVE ( )  GEOMETRIC_REPRESENTATION_ITEM ( )  RATIONAL_B_SPLINE_CURVE ( ( 0.9330127018922194093, 0.9330127018922194093, 1.000000000000000000, 0.8660254037844388186, 1.000000000000000000, 0.8660254037844388186, 1.000000000000000000, 0.9330127018922194093, 0.9330127018922194093 ) ) 
 REPRESENTATION_ITEM ( '' )  );
#9314=ORIENTED_EDGE ( 'NONE', *, *, #5980, .F. ) ;
#9315=CARTESIAN_POINT ( 'NONE',  ( 3.175426480543072749, 5.499999999999865885, -91.62500000000001421 ) ) ;
#9316=CARTESIAN_POINT ( 'NONE',  ( -3.608439182435115633, 6.249999999999965361, -103.8080127018922525 ) ) ;
#9317=ORIENTED_EDGE ( 'NONE', *, *, #7241, .T. ) ;
#9318=CARTESIAN_POINT ( 'NONE',  ( 4.763867271839615114, 9.917884865257411420, -21.33175192690179856 ) ) ;
#9320=CARTESIAN_POINT ( 'NONE',  ( 0.000000000000000000, 5.499999999999991118, -165.0000000000000284 ) ) ;
#9321=ADVANCED_FACE ( 'NONE', ( #3588 ), #10705, .T. ) ;
#9323=ORIENTED_EDGE ( 'NONE', *, *, #11444, .F. ) ;
#9325=VECTOR ( 'NONE', #5736, 1000.000000000000000 ) ;
#9326=CARTESIAN_POINT ( 'NONE',  ( -4.763139720814407951, 2.749999999999946709, -175.2500000000000284 ) ) ;
#9327=CARTESIAN_POINT ( 'NONE',  ( 3.175426480543072749, -5.500000000000105693, -152.1250000000000568 ) ) ;
#9328=AXIS2_PLACEMENT_3D ( 'NONE', #29636, #24876, #22285 ) ;
#9331=CARTESIAN_POINT ( 'NONE',  ( 0.000000000000000000, -5.999999999999991118, -166.0386751345947971 ) ) ;
#9333=CARTESIAN_POINT ( 'NONE',  ( 4.763139720814407951, 2.750000000000002665, -94.75000000000000000 ) ) ;
#9344=CARTESIAN_POINT ( 'NONE',  ( -6.000000000000000888, 1.067854986875958443E-15, 7.560779664488942560E-35 ) ) ;
#9347=VECTOR ( 'NONE', #17343, 1000.000000000000000 ) ;
#9352=VERTEX_POINT ( 'NONE', #24332 ) ;
#9353=CARTESIAN_POINT ( 'NONE',  ( -2.775557561562891351E-14, -5.500000000000115463, -116.2500000000000142 ) ) ;
#9355=CARTESIAN_POINT ( 'NONE',  ( -3.608439182435052128, -6.250000000000110134, -131.8080127018922383 ) ) ;
#9356=ORIENTED_EDGE ( 'NONE', *, *, #3289, .T. ) ;
#9357=CYLINDRICAL_SURFACE ( 'NONE', #8292, 6.000000000000000888 ) ;
#9358=CARTESIAN_POINT ( 'NONE',  ( -5.412658773652684552, -3.125000000000099920, -168.5669872981078186 ) ) ;
#9360=EDGE_CURVE ( 'NONE', #12840, #17900, #3286, .T. ) ;
#9362=CARTESIAN_POINT ( 'NONE',  ( 5.999999999999949374, 1.607695154586804565, -96.01933756729745539 ) ) ;
#9366=CARTESIAN_POINT ( 'NONE',  ( -5.412658773652739619, 3.124999999999975131, -175.6830127018922383 ) ) ;
#9368=CARTESIAN_POINT ( 'NONE',  ( 3.464101615137757051, -5.999999999999979572, -48.33632486540521711 ) ) ;
#9370=CARTESIAN_POINT ( 'NONE',  ( -5.999999999999957367, 1.607695154586737507, -158.9806624327025872 ) ) ;
#9371=CARTESIAN_POINT ( 'NONE',  ( -3.175426480542816510, 5.499999999999865885, -122.8749999999999858 ) ) ;
#9374=CARTESIAN_POINT ( 'NONE',  ( 3.464101615137852974, 5.999999999999884537, -145.9136751345947687 ) ) ;
#9375=ORIENTED_EDGE ( 'NONE', *, *, #4146, .F. ) ;
#9381=DIRECTION ( 'NONE',  ( -7.147005652999508048E-36, 5.642372883946980038E-36, 1.000000000000000000 ) ) ;
#9382=CARTESIAN_POINT ( 'NONE',  ( -5.412658773652684552, -3.125000000000099920, -111.5669872981078186 ) ) ;
#9384=CARTESIAN_POINT ( 'NONE',  ( 0.000000000000000000, -5.999999999999991118, -95.53867513459479710 ) ) ;
#9386=ORIENTED_EDGE ( 'NONE', *, *, #15018, .F. ) ;
#9390=( GEOMETRIC_REPRESENTATION_CONTEXT ( 3 ) GLOBAL_UNCERTAINTY_ASSIGNED_CONTEXT ( ( #23802 ) ) GLOBAL_UNIT_ASSIGNED_CONTEXT ( ( #29198, #27206, #24765 ) ) REPRESENTATION_CONTEXT ( 'NONE', 'WORKASPACE' ) );
#9391=CARTESIAN_POINT ( 'NONE',  ( -5.412658773652739619, 3.124999999999975131, -140.3169872981078186 ) ) ;
#9396=CARTESIAN_POINT ( 'NONE',  ( 3.464101615137852974, 5.999999999999884537, -151.3363248654051745 ) ) ;
#9398=CARTESIAN_POINT ( 'NONE',  ( 0.000000000000000000, -5.999999999999991118, -171.4613248654052313 ) ) ;
#9399=CARTESIAN_POINT ( 'NONE',  ( -5.999999999999963585, 8.134310703387671600E-14, -120.8363248654052171 ) ) ;
#9400=( BOUNDED_CURVE ( )  B_SPLINE_CURVE ( 2, ( #8538, #22533, #15650, #27258, #10877, #6230, #13197, #29581, #597 ),
 .UNSPECIFIED., .F., .T. ) 
 B_SPLINE_CURVE_WITH_KNOTS ( ( 3, 2, 2, 2, 3 ),
 ( 0.06944444444444444753, 0.07037037037037037479, 0.07222222222222221544, 0.07407407407407406996, 0.07499999999999999722 ),
 .UNSPECIFIED. ) 
 CURVE ( )  GEOMETRIC_REPRESENTATION_ITEM ( )  RATIONAL_B_SPLINE_CURVE ( ( 0.9330127018922194093, 0.9330127018922194093, 1.000000000000000000, 0.8660254037844388186, 1.000000000000000000, 0.8660254037844388186, 1.000000000000000000, 0.9330127018922194093, 0.9330127018922194093 ) ) 
 REPRESENTATION_ITEM ( '' )  );
#9401=EDGE_CURVE ( 'NONE', #21672, #4124, #30323, .T. ) ;
#9405=CARTESIAN_POINT ( 'NONE',  ( 5.999999999999999112, 2.951592740943527306E-14, -160.5863248654052029 ) ) ;
#9406=CARTESIAN_POINT ( 'NONE',  ( 6.000000000000000888, -1.607695154586752384, -146.2306624327026441 ) ) ;
#9415=CARTESIAN_POINT ( 'NONE',  ( 4.763139720814407951, 2.750000000000002665, -57.25000000000002132 ) ) ;
#9416=CYLINDRICAL_SURFACE ( 'NONE', #4600, 6.000000000000000888 ) ;
#9417=CARTESIAN_POINT ( 'NONE',  ( 6.000000000000000888, 7.762456499804234384E-14, -121.5863248654052455 ) ) ;
#9422=CARTESIAN_POINT ( 'NONE',  ( 5.412658773652712085, -3.125000000000086153, -102.0669872981078186 ) ) ;
#9429=CARTESIAN_POINT ( 'NONE',  ( -6.350852961085760029, -1.281975124255709124E-13, -139.1250000000000000 ) ) ;
#9430=ORIENTED_EDGE ( 'NONE', *, *, #4106, .F. ) ;
#9432=CARTESIAN_POINT ( 'NONE',  ( 3.175426480543072749, -5.500000000000105693, -66.62500000000002842 ) ) ;
#9435=CARTESIAN_POINT ( 'NONE',  ( -3.464101615137757051, -5.999999999999979572, -179.6636751345948255 ) ) ;
#9437=CARTESIAN_POINT ( 'NONE',  ( -3.608439182435115633, 6.249999999999965361, -84.30801270189222407 ) ) ;
#9439=CARTESIAN_POINT ( 'NONE',  ( 5.196152422706629359, -2.999999999999988898, -100.7113248654052313 ) ) ;
#9440=CARTESIAN_POINT ( 'NONE',  ( -5.999999999999971578, 1.607695154586715303, -139.4806624327025872 ) ) ;
#9442=CARTESIAN_POINT ( 'NONE',  ( 0.000000000000000000, 0.000000000000000000, -43.99152654425658682 ) ) ;
#9443=CARTESIAN_POINT ( 'NONE',  ( 0.000000000000000000, 0.000000000000000000, 0.000000000000000000 ) ) ;
#9445=CARTESIAN_POINT ( 'NONE',  ( -3.175426480542816066, -5.500000000000057732, -147.8750000000000284 ) ) ;
#9447=CARTESIAN_POINT ( 'NONE',  ( -7.216878364870328078, 0.000000000000000000, -160.5580127018922099 ) ) ;
#9448=CARTESIAN_POINT ( 'NONE',  ( 21.99999999999998934, 10.99999999999992184, -14.99152654425661879 ) ) ;
#9451=CARTESIAN_POINT ( 'NONE',  ( 0.000000000000000000, 5.499999999999991118, -82.50000000000001421 ) ) ;
#9453=CARTESIAN_POINT ( 'NONE',  ( -3.175426480542816510, -5.500000000000057732, -62.37500000000001421 ) ) ;
#9454=CARTESIAN_POINT ( 'NONE',  ( 5.999999999999988454, 1.607695154586737729, -155.0966878364871206 ) ) ;
#9455=CARTESIAN_POINT ( 'NONE',  ( 6.000000000000000888, 1.743066579297358182E-13, -87.66367513459482552 ) ) ;
#9459=CARTESIAN_POINT ( 'NONE',  ( -5.999999999999956479, -1.607695154586745057, -50.26933756729746250 ) ) ;
#9468=ORIENTED_EDGE ( 'NONE', *, *, #16847, .T. ) ;
#9472=CARTESIAN_POINT ( 'NONE',  ( -6.350852961085760029, -1.281975124255709124E-13, -92.62500000000001421 ) ) ;
#9474=CARTESIAN_POINT ( 'NONE',  ( 5.412658773652712085, -3.125000000000086153, -110.4330127018922099 ) ) ;
#9476=CARTESIAN_POINT ( 'NONE',  ( 5.196152422706629359, 3.000000000000002665, -68.03867513459482552 ) ) ;
#9479=CARTESIAN_POINT ( 'NONE',  ( -4.763139720814407951, -2.750000000000016431, -166.0000000000000284 ) ) ;
#9480=CARTESIAN_POINT ( 'NONE',  ( -3.464101615137757051, -5.999999999999979572, -106.1636751345948539 ) ) ;
#9482=CARTESIAN_POINT ( 'NONE',  ( 6.000000000000000888, -1.859271017917181981E-14, -67.58632486540523132 ) ) ;
#9483=CARTESIAN_POINT ( 'NONE',  ( -6.350852961085760029, -1.281975124255709124E-13, -169.1249999999999716 ) ) ;
#9485=CARTESIAN_POINT ( 'NONE',  ( -6.350852961085760029, -1.281975124255709124E-13, -151.1250000000000568 ) ) ;
#9487=CARTESIAN_POINT ( 'NONE',  ( 3.175426480543072749, -5.500000000000105693, -101.1249999999999858 ) ) ;
#9488=CARTESIAN_POINT ( 'NONE',  ( -5.196152422706573404, -3.000000000000002665, -159.7113248654052313 ) ) ;
#9490=( BOUNDED_CURVE ( )  B_SPLINE_CURVE ( 2, ( #22282, #1072, #18004, #8279, #14924 ),
 .UNSPECIFIED., .F., .F. ) 
 B_SPLINE_CURVE_WITH_KNOTS ( ( 3, 2, 3 ),
 ( 0.000000000000000000, 0.001851851851851882280, 0.002777777777777768343 ),
 .UNSPECIFIED. ) 
 CURVE ( )  GEOMETRIC_REPRESENTATION_ITEM ( )  RATIONAL_B_SPLINE_CURVE ( ( 1.000000000000000000, 0.8660254037844388186, 1.000000000000000000, 0.9330127018922194093, 0.9330127018922194093 ) ) 
 REPRESENTATION_ITEM ( '' )  );
#9491=CARTESIAN_POINT ( 'NONE',  ( -6.350852961085760029, -1.281975124255709124E-13, -157.1250000000000284 ) ) ;
#9492=CARTESIAN_POINT ( 'NONE',  ( 0.000000000000000000, 5.499999999999991118, -88.50000000000002842 ) ) ;
#9501=( BOUNDED_CURVE ( )  B_SPLINE_CURVE ( 2, ( #25244, #20671, #8995, #30024, #27699, #24650, #3597, #15795, #1457 ),
 .UNSPECIFIED., .F., .T. ) 
 B_SPLINE_CURVE_WITH_KNOTS ( ( 3, 2, 2, 2, 3 ),
 ( 0.7916666666666666297, 0.7925925925925926263, 0.7944444444444443976, 0.7962962962962962798, 0.7972222222222222765 ),
 .UNSPECIFIED. ) 
 CURVE ( )  GEOMETRIC_REPRESENTATION_ITEM ( )  RATIONAL_B_SPLINE_CURVE ( ( 0.9330127018922194093, 0.9330127018922154125, 1.000000000000000000, 0.8660254037844388186, 1.000000000000000000, 0.8660254037844388186, 1.000000000000000000, 0.9330127018922154125, 0.9330127018922194093 ) ) 
 REPRESENTATION_ITEM ( '' )  );
#9502=ORIENTED_EDGE ( 'NONE', *, *, #15131, .F. ) ;
#9504=DIRECTION ( 'NONE',  ( -7.147005652999508048E-36, 5.642372883946980038E-36, 1.000000000000000000 ) ) ;
#9508=CARTESIAN_POINT ( 'NONE',  ( 6.000000000000052403, -1.607695154586662678, -52.65331216351295041 ) ) ;
#9509=AXIS2_PLACEMENT_3D ( 'NONE', #3631, #13068, #22399 ) ;
#9511=VERTEX_POINT ( 'NONE', #25558 ) ;
#9512=CARTESIAN_POINT ( 'NONE',  ( 3.175426480543072749, 5.499999999999865885, -114.1249999999999858 ) ) ;
#9515=CARTESIAN_POINT ( 'NONE',  ( 2.775557561562891351E-14, -6.250000000000061284, -130.1830127018922667 ) ) ;
#9516=ORIENTED_EDGE ( 'NONE', *, *, #8222, .T. ) ;
#9517=CARTESIAN_POINT ( 'NONE',  ( 0.000000000000000000, 0.000000000000000000, 0.000000000000000000 ) ) ;
#9518=CARTESIAN_POINT ( 'NONE',  ( 5.412658773652712085, -3.125000000000086153, -168.0669872981078186 ) ) ;
#9523=CARTESIAN_POINT ( 'NONE',  ( -3.464101615137725076, 5.999999999999979572, -136.6636751345948539 ) ) ;
#9524=CARTESIAN_POINT ( 'NONE',  ( 4.763139720814407951, 2.750000000000002665, -177.2500000000000284 ) ) ;
#9526=CARTESIAN_POINT ( 'NONE',  ( 2.775557561562891351E-14, 6.250000000000033751, -175.9330127018922099 ) ) ;
#9528=CARTESIAN_POINT ( 'NONE',  ( -3.464101615137725076, 5.999999999999979572, -123.1636751345947971 ) ) ;
#9529=CARTESIAN_POINT ( 'NONE',  ( 6.350852961086080661, -9.614813431917819062E-14, -112.8750000000000568 ) ) ;
#9530=CARTESIAN_POINT ( 'NONE',  ( -3.464101615137725076, 5.999999999999979572, -145.6636751345947687 ) ) ;
#9536=ORIENTED_EDGE ( 'NONE', *, *, #23492, .F. ) ;
#9538=EDGE_CURVE ( 'NONE', #3881, #4074, #11925, .T. ) ;
#9539=CARTESIAN_POINT ( 'NONE',  ( 3.464101615137757051, -5.999999999999979572, -176.4136751345947403 ) ) ;
#9540=CARTESIAN_POINT ( 'NONE',  ( 0.000000000000000000, -5.999999999999991118, -125.5386751345948255 ) ) ;
#9545=EDGE_LOOP ( 'NONE', ( #4319, #25213, #27559, #2757 ) ) ;
#9548=ORIENTED_EDGE ( 'NONE', *, *, #3918, .F. ) ;
#9549=CARTESIAN_POINT ( 'NONE',  ( 5.412658773652739619, 3.124999999999988898, -136.3169872981078186 ) ) ;
#9550=CARTESIAN_POINT ( 'NONE',  ( 6.000000000000000888, -3.330669073875464691E-16, -7.560779664488942560E-35 ) ) ;
#9552=CARTESIAN_POINT ( 'NONE',  ( -6.000000000000007105, -1.607695154586655129, -93.76933756729741276 ) ) ;
#9555=CARTESIAN_POINT ( 'NONE',  ( 6.000000000000000888, -1.859271017917181981E-14, -137.1636751345948255 ) ) ;
#9556=DIRECTION ( 'NONE',  ( -7.147005652999508048E-36, 5.642372883946980038E-36, 1.000000000000000000 ) ) ;
#9558=CARTESIAN_POINT ( 'NONE',  ( -5.999999999999963585, -1.487416814333745711E-14, -101.9136751345948397 ) ) ;
#9559=CARTESIAN_POINT ( 'NONE',  ( 5.999999999999949374, 1.607695154586804565, -74.09668783648706381 ) ) ;
#9561=CARTESIAN_POINT ( 'NONE',  ( -6.000000000000007105, -1.607695154586655129, -69.76933756729741276 ) ) ;
#9564=CARTESIAN_POINT ( 'NONE',  ( -5.999999999999962697, 3.323446944526963891E-14, -148.4136751345948255 ) ) ;
#9565=ORIENTED_EDGE ( 'NONE', *, *, #28445, .F. ) ;
#9566=CARTESIAN_POINT ( 'NONE',  ( 6.350852961086080661, -9.614813431917819062E-14, -55.87500000000003553 ) ) ;
#9567=CARTESIAN_POINT ( 'NONE',  ( -5.196152422706573404, -3.000000000000002665, -133.2886751345948539 ) ) ;
#9568=CARTESIAN_POINT ( 'NONE',  ( -5.999999999999919176, 1.607695154586804565, -62.40331216351300725 ) ) ;
#9569=DIRECTION ( 'NONE',  ( -7.147005652999508048E-36, 5.642372883946980038E-36, 1.000000000000000000 ) ) ;
#9574=CARTESIAN_POINT ( 'NONE',  ( 5.412658773652739619, 3.124999999999988898, -101.8169872981078470 ) ) ;
#9579=CARTESIAN_POINT ( 'NONE',  ( -3.175426480542816510, -5.500000000000057732, -128.3750000000000000 ) ) ;
#9580=( BOUNDED_CURVE ( )  B_SPLINE_CURVE ( 2, ( #3564, #1426, #8497, #17903, #12995, #25072, #24923, #10512, #22493 ),
 .UNSPECIFIED., .F., .T. ) 
 B_SPLINE_CURVE_WITH_KNOTS ( ( 3, 2, 2, 2, 3 ),
 ( 0.4694444444444444420, 0.4703703703703703831, 0.4722222222222222099, 0.4740740740740740922, 0.4750000000000000333 ),
 .UNSPECIFIED. ) 
 CURVE ( )  GEOMETRIC_REPRESENTATION_ITEM ( )  RATIONAL_B_SPLINE_CURVE ( ( 0.9330127018922194093, 0.9330127018922194093, 1.000000000000000000, 0.8660254037844388186, 1.000000000000000000, 0.8660254037844388186, 1.000000000000000000, 0.9330127018922174109, 0.9330127018922194093 ) ) 
 REPRESENTATION_ITEM ( '' )  );
#9583=CARTESIAN_POINT ( 'NONE',  ( 5.999999999999999112, 2.951592740943527306E-14, -163.5863248654052313 ) ) ;
#9585=CARTESIAN_POINT ( 'NONE',  ( -2.775557561562891351E-14, -5.500000000000115463, -66.75000000000002842 ) ) ;
#9586=CARTESIAN_POINT ( 'NONE',  ( -3.464101615137725076, 5.999999999999979572, -115.6636751345948255 ) ) ;
#9588=CARTESIAN_POINT ( 'NONE',  ( -7.216878364870328078, 0.000000000000000000, -79.55801270189225249 ) ) ;
#9589=CARTESIAN_POINT ( 'NONE',  ( 0.000000000000000000, -5.999999999999991118, -113.5386751345948113 ) ) ;
#9594=CARTESIAN_POINT ( 'NONE',  ( 4.763139720814407951, 2.750000000000002665, -139.7500000000000284 ) ) ;
#9595=CARTESIAN_POINT ( 'NONE',  ( -3.464101615137757051, -5.999999999999979572, -105.5863248654052171 ) ) ;
#9597=CARTESIAN_POINT ( 'NONE',  ( 5.412658773652739619, 3.124999999999988898, -155.1830127018922667 ) ) ;
#9599=CARTESIAN_POINT ( 'NONE',  ( 3.175426480543072749, 5.499999999999865885, -82.62500000000004263 ) ) ;
#9600=CARTESIAN_POINT ( 'NONE',  ( 5.999999999999949374, 1.607695154586804565, -174.0193375672974412 ) ) ;
#9601=CARTESIAN_POINT ( 'NONE',  ( 4.763139720814407951, 2.750000000000002665, -61.75000000000002842 ) ) ;
#9604=CARTESIAN_POINT ( 'NONE',  ( -5.999999999999962697, 3.323446944526963891E-14, -148.4136751345948255 ) ) ;
#9608=LINE ( 'NONE', #16703, #27802 ) ;
#9610=DIRECTION ( 'NONE',  ( 1.000000000000000000, -5.551115123125773458E-17, -1.260129944081490338E-35 ) ) ;
#9615=ORIENTED_EDGE ( 'NONE', *, *, #30294, .F. ) ;
#9617=VERTEX_POINT ( 'NONE', #14391 ) ;
#9618=CARTESIAN_POINT ( 'NONE',  ( 3.175426480543072749, 5.499999999999865885, -93.12500000000002842 ) ) ;
#9620=CARTESIAN_POINT ( 'NONE',  ( -3.608439182435052128, -6.250000000000110134, -100.3080127018922241 ) ) ;
#9621=ORIENTED_EDGE ( 'NONE', *, *, #24746, .F. ) ;
#9623=VECTOR ( 'NONE', #20326, 1000.000000000000000 ) ;
#9626=CARTESIAN_POINT ( 'NONE',  ( 0.000000000000000000, -5.999999999999991118, -67.96132486540523132 ) ) ;
#9628=CARTESIAN_POINT ( 'NONE',  ( -2.775557561562891351E-14, -5.500000000000115463, -173.2500000000000284 ) ) ;
#9630=CARTESIAN_POINT ( 'NONE',  ( 3.175426480543072749, -5.500000000000105693, -158.1250000000000284 ) ) ;
#9632=CARTESIAN_POINT ( 'NONE',  ( -6.000000000000007105, -1.607695154586655129, -104.2693375672974128 ) ) ;
#9633=EDGE_CURVE ( 'NONE', #20687, #11659, #21575, .T. ) ;
#9634=CARTESIAN_POINT ( 'NONE',  ( -4.763139720814407951, -2.750000000000016431, -104.5000000000000426 ) ) ;
#9637=CARTESIAN_POINT ( 'NONE',  ( 4.763139720814407951, -2.749999999999988454, -155.0000000000000284 ) ) ;
#9638=CARTESIAN_POINT ( 'NONE',  ( -4.763139720814407951, -2.750000000000016431, -86.50000000000002842 ) ) ;
#9640=DIRECTION ( 'NONE',  ( -7.147005652999508048E-36, 5.642372883946980038E-36, 1.000000000000000000 ) ) ;
#9641=EDGE_LOOP ( 'NONE', ( #25227, #11847, #3577, #17335 ) ) ;
#9647=EDGE_CURVE ( 'NONE', #448, #30239, #11120, .T. ) ;
#9648=CARTESIAN_POINT ( 'NONE',  ( -3.464101615137725076, 5.999999999999979572, -78.16367513459485394 ) ) ;
#9650=EDGE_CURVE ( 'NONE', #2096, #23551, #25633, .T. ) ;
#9651=VERTEX_POINT ( 'NONE', #22481 ) ;
#9652=FACE_OUTER_BOUND ( 'NONE', #5809, .T. ) ;
#9653=ORIENTED_EDGE ( 'NONE', *, *, #27468, .T. ) ;
#9657=CARTESIAN_POINT ( 'NONE',  ( 4.763139720814407951, 2.750000000000002665, -109.7500000000000142 ) ) ;
#9660=CARTESIAN_POINT ( 'NONE',  ( -3.608439182435052128, -6.250000000000110134, -124.3080127018922099 ) ) ;
#9663=CARTESIAN_POINT ( 'NONE',  ( -7.216878364870328078, 0.000000000000000000, -165.6919872981078186 ) ) ;
#9667=( BOUNDED_CURVE ( )  B_SPLINE_CURVE ( 2, ( #3073, #12497, #22598, #24731, #1380, #13258, #13107, #1531, #25024 ),
 .UNSPECIFIED., .F., .T. ) 
 B_SPLINE_CURVE_WITH_KNOTS ( ( 3, 2, 2, 2, 3 ),
 ( 0.9305555555555555802, 0.9314814814814814659, 0.9333333333333333481, 0.9351851851851852304, 0.9361111111111111160 ),
 .UNSPECIFIED. ) 
 CURVE ( )  GEOMETRIC_REPRESENTATION_ITEM ( )  RATIONAL_B_SPLINE_CURVE ( ( 0.9330127018922194093, 0.9330127018922234061, 1.000000000000000000, 0.8660254037844388186, 1.000000000000000000, 0.8660254037844388186, 1.000000000000000000, 0.9330127018922194093, 0.9330127018922194093 ) ) 
 REPRESENTATION_ITEM ( '' )  );
#9668=CARTESIAN_POINT ( 'NONE',  ( -4.871333033796909184, 9.863307416503793945, -21.49176472276548111 ) ) ;
#9670=CARTESIAN_POINT ( 'NONE',  ( -2.775557561562891351E-14, -5.500000000000115463, -176.2500000000000284 ) ) ;
#9672=CARTESIAN_POINT ( 'NONE',  ( 7.216878364870455975, -6.409875621278545621E-14, -173.3080127018922667 ) ) ;
#9673=CARTESIAN_POINT ( 'NONE',  ( -5.999999999999971578, 1.607695154586715303, -75.90331216351297883 ) ) ;
#9675=CARTESIAN_POINT ( 'NONE',  ( -3.464101615137757051, -5.999999999999979572, -101.6636751345948255 ) ) ;
#9678=CARTESIAN_POINT ( 'NONE',  ( -4.763139720814407951, 2.749999999999946709, -110.7500000000000142 ) ) ;
#9680=CARTESIAN_POINT ( 'NONE',  ( -5.196152422706601826, 2.999999999999975131, -165.9613248654052029 ) ) ;
#9681=CARTESIAN_POINT ( 'NONE',  ( 3.464101615137852974, 5.999999999999884537, -88.91367513459483973 ) ) ;
#9682=ORIENTED_EDGE ( 'NONE', *, *, #19452, .F. ) ;
#9684=LINE ( 'NONE', #21059, #26069 ) ;
#9685=CARTESIAN_POINT ( 'NONE',  ( 6.000000000000000888, -1.859271017917181981E-14, -168.6636751345947971 ) ) ;
#9686=AXIS2_PLACEMENT_3D ( 'NONE', #14831, #24175, #28914 ) ;
#9692=CARTESIAN_POINT ( 'NONE',  ( -5.999999999999963585, -1.487416814333745711E-14, -127.4136751345948113 ) ) ;
#9693=FACE_OUTER_BOUND ( 'NONE', #22563, .T. ) ;
#9694=CARTESIAN_POINT ( 'NONE',  ( 3.464101615137757051, -5.999999999999979572, -77.41367513459478289 ) ) ;
#9695=CYLINDRICAL_SURFACE ( 'NONE', #24540, 6.000000000000000888 ) ;
#9696=( GEOMETRIC_REPRESENTATION_CONTEXT ( 3 ) GLOBAL_UNCERTAINTY_ASSIGNED_CONTEXT ( ( #13185 ) ) GLOBAL_UNIT_ASSIGNED_CONTEXT ( ( #23922, #29255, #19910 ) ) REPRESENTATION_CONTEXT ( 'NONE', 'WORKASPACE' ) );
#9697=VERTEX_POINT ( 'NONE', #4297 ) ;
#9698=CARTESIAN_POINT ( 'NONE',  ( 0.000000000000000000, 5.999999999999977796, -141.2886751345947971 ) ) ;
#9700=VERTEX_POINT ( 'NONE', #26742 ) ;
#9701=CARTESIAN_POINT ( 'NONE',  ( -3.608439182435115633, 6.249999999999965361, -143.4419872981078470 ) ) ;
#9703=AXIS2_PLACEMENT_3D ( 'NONE', #20239, #15814, #15657 ) ;
#9705=CARTESIAN_POINT ( 'NONE',  ( 6.000000000000000888, -1.607695154586752384, -116.2306624327026157 ) ) ;
#9707=CARTESIAN_POINT ( 'NONE',  ( 6.000000000000000888, -3.330669073875464691E-16, -7.560779664488942560E-35 ) ) ;
#9709=CARTESIAN_POINT ( 'NONE',  ( 5.196152422706629359, -2.999999999999988898, -56.28867513459484684 ) ) ;
#9710=CARTESIAN_POINT ( 'NONE',  ( -3.464101615137725076, 5.999999999999979572, -92.58632486540521711 ) ) ;
#9712=CARTESIAN_POINT ( 'NONE',  ( 0.000000000000000000, 5.999999999999977796, -60.28867513459484684 ) ) ;
#9713=DIRECTION ( 'NONE',  ( -7.147005652999508048E-36, 5.642372883946980038E-36, 1.000000000000000000 ) ) ;
#9718=CARTESIAN_POINT ( 'NONE',  ( 3.464101615137852974, 5.999999999999884537, -148.9136751345947687 ) ) ;
#9719=VERTEX_POINT ( 'NONE', #8325 ) ;
#9722=CARTESIAN_POINT ( 'NONE',  ( 3.464101615137852974, 5.999999999999884537, -88.33632486540521711 ) ) ;
#9724=CARTESIAN_POINT ( 'NONE',  ( -5.999999999999919176, 1.607695154586804565, -78.90331216351299304 ) ) ;
#9725=CARTESIAN_POINT ( 'NONE',  ( -5.999999999999963585, 9.296355089585909904E-15, -164.3363248654052313 ) ) ;
#9728=CARTESIAN_POINT ( 'NONE',  ( 3.608439182435180470, -6.249999999999997335, -105.1919872981078470 ) ) ;
#9731=AXIS2_PLACEMENT_3D ( 'NONE', #22215, #13488, #11020 ) ;
#9734=CARTESIAN_POINT ( 'NONE',  ( -6.350852961085760029, -1.281975124255709124E-13, -125.6250000000000426 ) ) ;
#9736=CARTESIAN_POINT ( 'NONE',  ( -4.763139720814407951, 2.749999999999946709, -56.75000000000002132 ) ) ;
#9738=CARTESIAN_POINT ( 'NONE',  ( 2.775557561562891351E-14, -6.250000000000061284, -85.18301270189220986 ) ) ;
#9739=UNCERTAINTY_MEASURE_WITH_UNIT (LENGTH_MEASURE( 1.000000000000000082E-05 ), #1638, 'distance_accuracy_value', 'NONE');
#9744=EDGE_CURVE ( 'NONE', #25601, #10258, #325, .T. ) ;
#9747=CARTESIAN_POINT ( 'NONE',  ( -6.350852961085760029, -1.281975124255709124E-13, -140.6250000000000000 ) ) ;
#9749=CARTESIAN_POINT ( 'NONE',  ( 3.608439182435180470, 6.249999999999982236, -155.0580127018922383 ) ) ;
#9750=SURFACE_STYLE_FILL_AREA ( #16247 ) ;
#9751=CARTESIAN_POINT ( 'NONE',  ( 3.175426480543072749, -5.500000000000105693, -69.62500000000004263 ) ) ;
#9752=CARTESIAN_POINT ( 'NONE',  ( 4.763139720814407951, -2.749999999999988454, -63.50000000000000000 ) ) ;
#9766=CARTESIAN_POINT ( 'NONE',  ( 5.999999999999999112, 2.951592740943527306E-14, -158.1636751345948539 ) ) ;
#9768=CARTESIAN_POINT ( 'NONE',  ( -3.175426480542816510, 5.499999999999865885, -181.3750000000000000 ) ) ;
#9770=CARTESIAN_POINT ( 'NONE',  ( -3.608439182435115633, 6.249999999999965361, -153.9419872981078186 ) ) ;
#9772=CARTESIAN_POINT ( 'NONE',  ( 4.763139720814407951, -2.749999999999988454, -80.00000000000001421 ) ) ;
#9773=CARTESIAN_POINT ( 'NONE',  ( -3.608439182435115633, 6.249999999999965361, -102.3080127018922383 ) ) ;
#9774=ORIENTED_EDGE ( 'NONE', *, *, #24019, .F. ) ;
#9778=CARTESIAN_POINT ( 'NONE',  ( 6.000000000000000888, -1.859271017917181981E-14, -72.66367513459482552 ) ) ;
#9781=CARTESIAN_POINT ( 'NONE',  ( 4.763139720814407951, -2.749999999999988454, -161.0000000000000284 ) ) ;
#9782=CARTESIAN_POINT ( 'NONE',  ( 5.196152422706629359, 3.000000000000002665, -58.46132486540523132 ) ) ;
#9783=CARTESIAN_POINT ( 'NONE',  ( -2.775557561562891351E-14, -5.500000000000115463, -155.2500000000000000 ) ) ;
#9786=CARTESIAN_POINT ( 'NONE',  ( -3.175426480542816066, 5.499999999999865885, -103.3750000000000142 ) ) ;
#9788=CARTESIAN_POINT ( 'NONE',  ( 3.175426480543072749, 5.499999999999865885, -88.62500000000001421 ) ) ;
#9789=CARTESIAN_POINT ( 'NONE',  ( 0.000000000000000000, 0.000000000000000000, 0.000000000000000000 ) ) ;
#9792=CARTESIAN_POINT ( 'NONE',  ( 0.000000000000000000, -5.999999999999991118, -66.46132486540523132 ) ) ;
#9795=ORIENTED_EDGE ( 'NONE', *, *, #7508, .T. ) ;
#9796=CYLINDRICAL_SURFACE ( 'NONE', #19538, 6.000000000000000888 ) ;
#9800=ORIENTED_EDGE ( 'NONE', *, *, #3778, .F. ) ;
#9802=ORIENTED_EDGE ( 'NONE', *, *, #4170, .T. ) ;
#9804=CARTESIAN_POINT ( 'NONE',  ( -2.775557561562891351E-14, -5.500000000000115463, -113.2500000000000142 ) ) ;
#9806=CARTESIAN_POINT ( 'NONE',  ( 3.608439182435180470, 6.249999999999982236, -120.5580127018922667 ) ) ;
#9807=VERTEX_POINT ( 'NONE', #12678 ) ;
#9808=CARTESIAN_POINT ( 'NONE',  ( 0.000000000000000000, -5.999999999999991118, -68.53867513459482552 ) ) ;
#9809=MECHANICAL_DESIGN_GEOMETRIC_PRESENTATION_REPRESENTATION('',(#17673),#29892);
#9810=CARTESIAN_POINT ( 'NONE',  ( 7.216878364870455975, -6.409875621278545621E-14, -158.9419872981077901 ) ) ;
#9817=CARTESIAN_POINT ( 'NONE',  ( -5.196152422706601826, 2.999999999999975131, -137.4613248654051745 ) ) ;
#9818=CARTESIAN_POINT ( 'NONE',  ( 6.350852961086080661, -9.614813431917819062E-14, -177.3750000000000284 ) ) ;
#9820=CARTESIAN_POINT ( 'NONE',  ( -5.999999999999956479, -1.607695154586745057, -113.2693375672974128 ) ) ;
#9821=CARTESIAN_POINT ( 'NONE',  ( 2.775557561562891351E-14, -6.250000000000061284, -179.6830127018922383 ) ) ;
#9822=CARTESIAN_POINT ( 'NONE',  ( 5.196152422706629359, 3.000000000000002665, -76.46132486540524553 ) ) ;
#9823=CARTESIAN_POINT ( 'NONE',  ( 4.763139720814407951, -2.749999999999988454, -128.0000000000000000 ) ) ;
#9825=CARTESIAN_POINT ( 'NONE',  ( -3.175426480542816510, 5.499999999999865885, -112.3750000000000426 ) ) ;
#9831=CARTESIAN_POINT ( 'NONE',  ( -3.464101615137757051, -5.999999999999979572, -137.0863248654051745 ) ) ;
#9835=CARTESIAN_POINT ( 'NONE',  ( -4.763139720814407951, 2.749999999999946709, -178.2500000000000284 ) ) ;
#9837=ORIENTED_EDGE ( 'NONE', *, *, #13594, .F. ) ;
#9846=ORIENTED_EDGE ( 'NONE', *, *, #29723, .F. ) ;
#9847=CARTESIAN_POINT ( 'NONE',  ( -5.412658773652739619, 3.124999999999975131, -128.3169872981078186 ) ) ;
#9854=CARTESIAN_POINT ( 'NONE',  ( 3.464101615137757051, -5.999999999999979572, -129.9136751345947687 ) ) ;
#9855=EDGE_CURVE ( 'NONE', #16482, #29957, #18392, .T. ) ;
#9856=CARTESIAN_POINT ( 'NONE',  ( 6.000000000000000888, -1.859271017917181981E-14, -147.0863248654052313 ) ) ;
#9857=( BOUNDED_CURVE ( )  B_SPLINE_CURVE ( 2, ( #12370, #21719, #9439, #10041, #28743, #7715, #18822, #28148, #7116 ),
 .UNSPECIFIED., .F., .F. ) 
 B_SPLINE_CURVE_WITH_KNOTS ( ( 3, 2, 2, 2, 3 ),
 ( 0.4027777777777777901, 0.4037037037037036757, 0.4055555555555555580, 0.4074074074074074403, 0.4083333333333333259 ),
 .UNSPECIFIED. ) 
 CURVE ( )  GEOMETRIC_REPRESENTATION_ITEM ( )  RATIONAL_B_SPLINE_CURVE ( ( 0.9330127018922194093, 0.9330127018922194093, 1.000000000000000000, 0.8660254037844388186, 1.000000000000000000, 0.8660254037844388186, 1.000000000000000000, 0.9330127018922194093, 0.9330127018922194093 ) ) 
 REPRESENTATION_ITEM ( '' )  );
#9862=CARTESIAN_POINT ( 'NONE',  ( -5.196152422706573404, -3.000000000000002665, -140.2113248654052313 ) ) ;
#9867=CARTESIAN_POINT ( 'NONE',  ( 5.196152422706629359, -2.999999999999988898, -142.7113248654052313 ) ) ;
#9868=CARTESIAN_POINT ( 'NONE',  ( -6.350852961085760029, -1.281975124255709124E-13, -139.1250000000000000 ) ) ;
#9871=ORIENTED_EDGE ( 'NONE', *, *, #14063, .F. ) ;
#9877=CARTESIAN_POINT ( 'NONE',  ( -3.608439182435052128, -6.250000000000110134, -106.9419872981077901 ) ) ;
#9878=STYLED_ITEM ( 'NONE', ( #5855 ), #28673 ) ;
#9882=VECTOR ( 'NONE', #28236, 1000.000000000000000 ) ;
#9884=CARTESIAN_POINT ( 'NONE',  ( -4.763139720814407951, -2.750000000000016431, -127.0000000000000000 ) ) ;
#9888=CARTESIAN_POINT ( 'NONE',  ( 3.175426480543072749, 5.499999999999865885, -54.12500000000003553 ) ) ;
#9889=CARTESIAN_POINT ( 'NONE',  ( -5.196152422706573404, -3.000000000000002665, -179.7886751345948539 ) ) ;
#9890=LINE ( 'NONE', #19264, #26444 ) ;
#9891=EDGE_CURVE ( 'NONE', #12627, #23669, #12927, .T. ) ;
#9892=CARTESIAN_POINT ( 'NONE',  ( -5.412658773652684552, -3.125000000000099920, -83.93301270189223828 ) ) ;
#9894=( BOUNDED_CURVE ( )  B_SPLINE_CURVE ( 2, ( #17729, #6020, #29822, #1871, #29520, #19849, #27357, #20320, #8158 ),
 .UNSPECIFIED., .F., .F. ) 
 B_SPLINE_CURVE_WITH_KNOTS ( ( 3, 2, 2, 2, 3 ),
 ( 0.03055555555555556149, 0.03148148148148147835, 0.03333333333333333287, 0.03518518518518518740, 0.03611111111111110772 ),
 .UNSPECIFIED. ) 
 CURVE ( )  GEOMETRIC_REPRESENTATION_ITEM ( )  RATIONAL_B_SPLINE_CURVE ( ( 0.9330127018922194093, 0.9330127018922198534, 1.000000000000000000, 0.8660254037844388186, 1.000000000000000000, 0.8660254037844388186, 1.000000000000000000, 0.9330127018922196314, 0.9330127018922194093 ) ) 
 REPRESENTATION_ITEM ( '' )  );
#9896=CARTESIAN_POINT ( 'NONE',  ( -6.000000000000000888, 1.067854986875958443E-15, 7.560779664488942560E-35 ) ) ;
#9899=CARTESIAN_POINT ( 'NONE',  ( 3.175426480543072749, -5.500000000000105693, -137.1250000000000568 ) ) ;
#9900=CARTESIAN_POINT ( 'NONE',  ( 3.464101615137757051, -5.999999999999979572, -105.3363248654052171 ) ) ;
#9902=CARTESIAN_POINT ( 'NONE',  ( 5.412658773652739619, 3.124999999999988898, -156.6830127018922099 ) ) ;
#9904=CARTESIAN_POINT ( 'NONE',  ( -3.175426480542816066, 5.499999999999865885, -74.87500000000000000 ) ) ;
#9905=CARTESIAN_POINT ( 'NONE',  ( -6.350852961085760029, -1.281975124255709124E-13, -65.62500000000002842 ) ) ;
#9909=CARTESIAN_POINT ( 'NONE',  ( -5.999999999999963585, -1.487416814333745711E-14, -97.41367513459481131 ) ) ;
#9910=CARTESIAN_POINT ( 'NONE',  ( -6.000000000000007105, -1.607695154586655129, -58.34668783648704959 ) ) ;
#9912=CARTESIAN_POINT ( 'NONE',  ( 0.000000000000000000, 0.000000000000000000, 0.000000000000000000 ) ) ;
#9917=VECTOR ( 'NONE', #13135, 1000.000000000000000 ) ;
#9918=EDGE_CURVE ( 'NONE', #23551, #23148, #2309, .T. ) ;
#9919=EDGE_CURVE ( 'NONE', #12844, #2708, #28742, .T. ) ;
#9920=DIRECTION ( 'NONE',  ( -7.147005652999508048E-36, 5.642372883946980038E-36, 1.000000000000000000 ) ) ;
#9921=CARTESIAN_POINT ( 'NONE',  ( -3.608439182435115633, 6.249999999999965361, -47.44198729810783277 ) ) ;
#9924=CARTESIAN_POINT ( 'NONE',  ( -3.175426480542816510, 5.499999999999865885, -79.37500000000001421 ) ) ;
#9925=CARTESIAN_POINT ( 'NONE',  ( 3.608439182435180470, -6.249999999999997335, -98.55801270189222407 ) ) ;
#9926=ORIENTED_EDGE ( 'NONE', *, *, #4629, .F. ) ;
#9928=CYLINDRICAL_SURFACE ( 'NONE', #19627, 6.000000000000000888 ) ;
#9929=CARTESIAN_POINT ( 'NONE',  ( -5.999999999999919176, 1.607695154586804565, -58.48066243270260856 ) ) ;
#9931=CARTESIAN_POINT ( 'NONE',  ( 0.000000000000000000, -5.999999999999991118, -58.96132486540523132 ) ) ;
#9932=PRESENTATION_STYLE_ASSIGNMENT (( #12119 ) ) ;
#9933=CARTESIAN_POINT ( 'NONE',  ( 6.350852961086080661, -9.614813431917819062E-14, -165.3750000000000568 ) ) ;
#9935=CARTESIAN_POINT ( 'NONE',  ( -3.175426480542816510, -5.500000000000057732, -158.3750000000000284 ) ) ;
#9937=CARTESIAN_POINT ( 'NONE',  ( -3.175426480542816066, -5.500000000000057732, -90.87500000000001421 ) ) ;
#9938=CARTESIAN_POINT ( 'NONE',  ( -5.999999999999971578, 1.607695154586715303, -125.4033121635129930 ) ) ;
#9940=CARTESIAN_POINT ( 'NONE',  ( -3.175426480542816510, -5.500000000000057732, -90.87500000000001421 ) ) ;
#9941=( BOUNDED_CURVE ( )  B_SPLINE_CURVE ( 2, ( #8428, #17834, #761, #10145, #28848, #19516, #24547, #7806, #3498 ),
 .UNSPECIFIED., .F., .F. ) 
 B_SPLINE_CURVE_WITH_KNOTS ( ( 3, 2, 2, 2, 3 ),
 ( 0.2750000000000000222, 0.2759259259259259078, 0.2777777777777777901, 0.2796296296296296169, 0.2805555555555555580 ),
 .UNSPECIFIED. ) 
 CURVE ( )  GEOMETRIC_REPRESENTATION_ITEM ( )  RATIONAL_B_SPLINE_CURVE ( ( 0.9330127018922194093, 0.9330127018922214077, 1.000000000000000000, 0.8660254037844388186, 1.000000000000000000, 0.8660254037844388186, 1.000000000000000000, 0.9330127018922194093, 0.9330127018922194093 ) ) 
 REPRESENTATION_ITEM ( '' )  );
#9946=DIRECTION ( 'NONE',  ( 1.000000000000000000, -5.551115123125773458E-17, -1.260129944081490338E-35 ) ) ;
#9948=VERTEX_POINT ( 'NONE', #20905 ) ;
#9949=CARTESIAN_POINT ( 'NONE',  ( -5.999999999999963585, 1.780251999655701777E-13, -58.41367513459482552 ) ) ;
#9950=DIRECTION ( 'NONE',  ( -7.147005652999508048E-36, 5.642372883946980038E-36, 1.000000000000000000 ) ) ;
#9954=ORIENTED_EDGE ( 'NONE', *, *, #713, .T. ) ;
#9956=CARTESIAN_POINT ( 'NONE',  ( 3.175426480543072749, -5.500000000000105693, -107.1250000000000284 ) ) ;
#9958=CARTESIAN_POINT ( 'NONE',  ( 3.175426480543072749, 5.499999999999865885, -150.1250000000000284 ) ) ;
#9959=CARTESIAN_POINT ( 'NONE',  ( 3.608439182435180470, -6.249999999999997335, -125.5580127018922383 ) ) ;
#9960=VERTEX_POINT ( 'NONE', #12605 ) ;
#9961=CYLINDRICAL_SURFACE ( 'NONE', #14255, 6.000000000000000888 ) ;
#9962=CARTESIAN_POINT ( 'NONE',  ( 5.412658773652712085, -3.125000000000086153, -160.5669872981078186 ) ) ;
#9965=CARTESIAN_POINT ( 'NONE',  ( -3.608439182435052128, -6.250000000000110134, -56.80801270189228092 ) ) ;
#9966=VERTEX_POINT ( 'NONE', #10132 ) ;
#9967=CARTESIAN_POINT ( 'NONE',  ( 3.464101615137852974, 5.999999999999884537, -167.8363248654051745 ) ) ;
#9970=CARTESIAN_POINT ( 'NONE',  ( -3.175426480542816510, 5.499999999999865885, -179.8750000000000000 ) ) ;
#9973=CARTESIAN_POINT ( 'NONE',  ( 5.412658773652739619, 3.124999999999988898, -179.1830127018922383 ) ) ;
#9975=CARTESIAN_POINT ( 'NONE',  ( 0.000000000000000000, -5.999999999999991118, -48.46132486540521711 ) ) ;
#9976=CARTESIAN_POINT ( 'NONE',  ( -3.175426480542816066, -5.500000000000057732, -117.8750000000000142 ) ) ;
#9978=CARTESIAN_POINT ( 'NONE',  ( 4.763139720814407951, 2.750000000000002665, -117.2500000000000142 ) ) ;
#9980=CARTESIAN_POINT ( 'NONE',  ( -5.999999999999963585, 8.134310703387671600E-14, -131.9136751345948255 ) ) ;
#9981=ORIENTED_EDGE ( 'NONE', *, *, #9918, .T. ) ;
#9985=CARTESIAN_POINT ( 'NONE',  ( -5.999999999999971578, 1.607695154586715303, -167.9806624327025872 ) ) ;
#9988=CARTESIAN_POINT ( 'NONE',  ( -3.175426480542816066, 5.499999999999865885, -176.8750000000000568 ) ) ;
#9992=CARTESIAN_POINT ( 'NONE',  ( 6.000000000000000888, -1.859271017917181981E-14, -125.1636751345948397 ) ) ;
#9995=ORIENTED_EDGE ( 'NONE', *, *, #13141, .F. ) ;
#9998=ORIENTED_EDGE ( 'NONE', *, *, #24053, .F. ) ;
#10000=CARTESIAN_POINT ( 'NONE',  ( 5.412658773652712085, -3.125000000000086153, -132.0669872981078470 ) ) ;
#10001=DIRECTION ( 'NONE',  ( -7.147005652999508048E-36, 5.642372883946980038E-36, 1.000000000000000000 ) ) ;
#10002=DIRECTION ( 'NONE',  ( -7.147005652999508048E-36, 5.642372883946980038E-36, 1.000000000000000000 ) ) ;
#10004=VERTEX_POINT ( 'NONE', #28674 ) ;
#10007=CARTESIAN_POINT ( 'NONE',  ( 6.000000000000000888, -1.859271017917181981E-14, -136.5863248654051745 ) ) ;
#10009=CARTESIAN_POINT ( 'NONE',  ( 6.000000000000000888, -3.330669073875464691E-16, -7.560779664488942560E-35 ) ) ;
#10013=CARTESIAN_POINT ( 'NONE',  ( 3.175426480543072749, -5.500000000000105693, -137.1250000000000568 ) ) ;
#10016=EDGE_LOOP ( 'NONE', ( #11036, #22124, #7520, #18285 ) ) ;
#10019=CARTESIAN_POINT ( 'NONE',  ( 6.000000000000000888, 1.743066579297358182E-13, -76.58632486540523132 ) ) ;
#10025=CARTESIAN_POINT ( 'NONE',  ( -3.608439182435115633, 6.249999999999965361, -93.94198729810786119 ) ) ;
#10027=EDGE_CURVE ( 'NONE', #16677, #21329, #20522, .T. ) ;
#10030=DIRECTION ( 'NONE',  ( -7.147005652999508048E-36, 5.642372883946980038E-36, 1.000000000000000000 ) ) ;
#10032=CARTESIAN_POINT ( 'NONE',  ( -3.175426480542816510, 5.499999999999865885, -127.3750000000000000 ) ) ;
#10033=( BOUNDED_CURVE ( )  B_SPLINE_CURVE ( 2, ( #3214, #12637, #19822, #24572, #27025, #15238, #3521, #21982, #5671 ),
 .UNSPECIFIED., .F., .T. ) 
 B_SPLINE_CURVE_WITH_KNOTS ( ( 3, 2, 2, 2, 3 ),
 ( 0.3972222222222222543, 0.3981481481481481399, 0.4000000000000000222, 0.4018518518518518490, 0.4027777777777777901 ),
 .UNSPECIFIED. ) 
 CURVE ( )  GEOMETRIC_REPRESENTATION_ITEM ( )  RATIONAL_B_SPLINE_CURVE ( ( 0.9330127018922194093, 0.9330127018922214077, 1.000000000000000000, 0.8660254037844388186, 1.000000000000000000, 0.8660254037844388186, 1.000000000000000000, 0.9330127018922194093, 0.9330127018922194093 ) ) 
 REPRESENTATION_ITEM ( '' )  );
#10034=VERTEX_POINT ( 'NONE', #21655 ) ;
#10035=VERTEX_POINT ( 'NONE', #590 ) ;
#10036=CARTESIAN_POINT ( 'NONE',  ( 4.763139720814407951, -2.749999999999988454, -57.49999999999999289 ) ) ;
#10037=DIRECTION ( 'NONE',  ( 3.330669073875465184E-16, -0.8660254037844377084, 0.5000000000000016653 ) ) ;
#10038=CARTESIAN_POINT ( 'NONE',  ( 6.000000000000000888, 1.743066579297358182E-13, -66.66367513459481131 ) ) ;
#10040=CARTESIAN_POINT ( 'NONE',  ( -3.608439182435052128, -6.250000000000110134, -82.30801270189228092 ) ) ;
#10041=CARTESIAN_POINT ( 'NONE',  ( 3.464101615137757051, -5.999999999999979572, -100.8363248654051887 ) ) ;
#10043=DIRECTION ( 'NONE',  ( 1.000000000000000000, -5.551115123125774690E-17, 0.000000000000000000 ) ) ;
#10046=CARTESIAN_POINT ( 'NONE',  ( -3.175426480542816066, -5.500000000000057732, -138.8750000000000568 ) ) ;
#10048=CARTESIAN_POINT ( 'NONE',  ( 5.412658773652739619, 3.124999999999988898, -150.6830127018922099 ) ) ;
#10049=CARTESIAN_POINT ( 'NONE',  ( -5.999999999999963585, -1.487416814333745711E-14, -66.83632486540523132 ) ) ;
#10053=AXIS2_PLACEMENT_3D ( 'NONE', #3531, #5837, #8781 ) ;
#10054=CARTESIAN_POINT ( 'NONE',  ( -4.763139720814407951, -2.750000000000016431, -73.00000000000001421 ) ) ;
#10055=CARTESIAN_POINT ( 'NONE',  ( 3.464101615137852974, 5.999999999999884537, -114.4136751345948255 ) ) ;
#10056=CARTESIAN_POINT ( 'NONE',  ( -4.763139720814407951, 2.749999999999946709, -56.75000000000002132 ) ) ;
#10057=CARTESIAN_POINT ( 'NONE',  ( -5.999999999999919176, 1.607695154586804565, -53.40331216351298593 ) ) ;
#10060=CARTESIAN_POINT ( 'NONE',  ( -5.196152422706601826, 2.999999999999975131, -126.9613248654052313 ) ) ;
#10062=CARTESIAN_POINT ( 'NONE',  ( 5.196152422706629359, -2.999999999999988898, -104.2886751345948255 ) ) ;
#10067=ORIENTED_EDGE ( 'NONE', *, *, #6007, .T. ) ;
#10069=VECTOR ( 'NONE', #18164, 1000.000000000000000 ) ;
#10071=CARTESIAN_POINT ( 'NONE',  ( 3.175426480543072749, 5.499999999999865885, -180.1250000000000000 ) ) ;
#10074=CARTESIAN_POINT ( 'NONE',  ( 3.175426480543072749, -5.500000000000105693, -78.62500000000001421 ) ) ;
#10075=CARTESIAN_POINT ( 'NONE',  ( -7.216878364870328078, 0.000000000000000000, -100.5580127018922241 ) ) ;
#10078=CARTESIAN_POINT ( 'NONE',  ( 6.000000000000000888, 7.762456499804234384E-14, -127.5863248654052171 ) ) ;
#10079=CARTESIAN_POINT ( 'NONE',  ( -4.763139720814407951, -2.750000000000016431, -167.4999999999999716 ) ) ;
#10081=CARTESIAN_POINT ( 'NONE',  ( 4.871333033796958922, -9.863307416503765523, -21.49176472276546690 ) ) ;
#10084=CARTESIAN_POINT ( 'NONE',  ( 3.175426480543072749, -5.500000000000105693, -164.1249999999999716 ) ) ;
#10086=CARTESIAN_POINT ( 'NONE',  ( 3.175426480543072749, 5.499999999999865885, -148.6250000000000284 ) ) ;
#10088=CARTESIAN_POINT ( 'NONE',  ( -5.999999999999963585, -1.487416814333745711E-14, -59.33632486540522422 ) ) ;
#10091=CARTESIAN_POINT ( 'NONE',  ( 4.763139720814407951, 2.750000000000002665, -97.75000000000000000 ) ) ;
#10094=CARTESIAN_POINT ( 'NONE',  ( -3.175426480542816510, 5.499999999999865885, -92.87500000000002842 ) ) ;
#10102=CARTESIAN_POINT ( 'NONE',  ( 3.464101615137852974, 5.999999999999884537, -178.9136751345947971 ) ) ;
#10103=CARTESIAN_POINT ( 'NONE',  ( 5.999999999999949374, 1.607695154586804565, -83.09668783648704959 ) ) ;
#10105=ORIENTED_EDGE ( 'NONE', *, *, #19056, .T. ) ;
#10107=ORIENTED_EDGE ( 'NONE', *, *, #4387, .T. ) ;
#10109=CARTESIAN_POINT ( 'NONE',  ( 6.350852961086080661, -9.614813431917819062E-14, -102.3750000000000000 ) ) ;
#10111=CARTESIAN_POINT ( 'NONE',  ( 5.412658773652712085, -3.125000000000086153, -119.4330127018922099 ) ) ;
#10113=CARTESIAN_POINT ( 'NONE',  ( 5.196152422706629359, -2.999999999999988898, -60.78867513459484684 ) ) ;
#10114=CARTESIAN_POINT ( 'NONE',  ( 2.775557561562891351E-14, -6.250000000000061284, -162.3169872981078470 ) ) ;
#10117=CARTESIAN_POINT ( 'NONE',  ( -7.216878364870328078, 0.000000000000000000, -57.05801270189221697 ) ) ;
#10123=CARTESIAN_POINT ( 'NONE',  ( 4.763139720814407951, -2.749999999999988454, -168.4999999999999716 ) ) ;
#10127=CARTESIAN_POINT ( 'NONE',  ( 3.608439182435180470, -6.249999999999997335, -166.0580127018922099 ) ) ;
#10131=CARTESIAN_POINT ( 'NONE',  ( -3.175426480542816066, -5.500000000000057732, -119.3750000000000284 ) ) ;
#10132=CARTESIAN_POINT ( 'NONE',  ( 6.000000000000000888, -1.859271017917181981E-14, -54.66367513459481842 ) ) ;
#10134=CARTESIAN_POINT ( 'NONE',  ( -2.775557561562891351E-14, -5.500000000000115463, -114.7500000000000142 ) ) ;
#10140=CARTESIAN_POINT ( 'NONE',  ( 6.000000000000000888, 1.607695154586715303, -109.5193375672974270 ) ) ;
#10141=ORIENTED_EDGE ( 'NONE', *, *, #2860, .T. ) ;
#10143=CARTESIAN_POINT ( 'NONE',  ( 4.763139720814407951, -2.749999999999988454, -179.0000000000000568 ) ) ;
#10145=CARTESIAN_POINT ( 'NONE',  ( 3.464101615137852974, 5.999999999999884537, -144.4136751345947687 ) ) ;
#10147=ORIENTED_EDGE ( 'NONE', *, *, #27824, .F. ) ;
#10151=CARTESIAN_POINT ( 'NONE',  ( 3.608439182435180470, -6.249999999999997335, -129.1919872981078186 ) ) ;
#10152=CYLINDRICAL_SURFACE ( 'NONE', #24360, 6.000000000000000888 ) ;
#10153=DIRECTION ( 'NONE',  ( 1.000000000000000000, -5.551115123125773458E-17, -1.260129944081490338E-35 ) ) ;
#10155=CARTESIAN_POINT ( 'NONE',  ( -5.999999999999963585, 1.780251999655701777E-13, -56.33632486540525264 ) ) ;
#10156=CARTESIAN_POINT ( 'NONE',  ( -5.999999999999963585, -1.487416814333745711E-14, -139.4136751345948255 ) ) ;
#10160=CARTESIAN_POINT ( 'NONE',  ( 6.000000000000000888, -3.330669073875464691E-16, -7.560779664488942560E-35 ) ) ;
#10161=FACE_OUTER_BOUND ( 'NONE', #20193, .T. ) ;
#10167=EDGE_CURVE ( 'NONE', #16117, #9352, #20547, .T. ) ;
#10168=CARTESIAN_POINT ( 'NONE',  ( 3.175426480543072749, 5.499999999999865885, -141.1250000000000000 ) ) ;
#10172=CARTESIAN_POINT ( 'NONE',  ( 3.175426480543072749, 5.499999999999865885, -49.62500000000000000 ) ) ;
#10175=VECTOR ( 'NONE', #13493, 1000.000000000000000 ) ;
#10178=CARTESIAN_POINT ( 'NONE',  ( -3.608439182435052128, -6.250000000000110134, -99.44198729810781856 ) ) ;
#10179=CARTESIAN_POINT ( 'NONE',  ( 3.464101615137757051, -5.999999999999979572, -78.33632486540520290 ) ) ;
#10181=CARTESIAN_POINT ( 'NONE',  ( -3.464101615137725076, 5.999999999999979572, -77.58632486540523132 ) ) ;
#10182=VECTOR ( 'NONE', #12392, 1000.000000000000000 ) ;
#10183=CARTESIAN_POINT ( 'NONE',  ( -3.175426480542816510, 5.499999999999865885, -125.8749999999999858 ) ) ;
#10187=CARTESIAN_POINT ( 'NONE',  ( -5.999999999999963585, 1.780251999655701777E-13, -83.33632486540520290 ) ) ;
#10188=EDGE_CURVE ( 'NONE', #28549, #12504, #8878, .T. ) ;
#10189=CARTESIAN_POINT ( 'NONE',  ( -4.763139720814407951, 2.749999999999946709, -53.75000000000002132 ) ) ;
#10191=CARTESIAN_POINT ( 'NONE',  ( -3.464101615137757051, -5.999999999999979572, -134.6636751345948539 ) ) ;
#10193=CARTESIAN_POINT ( 'NONE',  ( -5.412658773652684552, -3.125000000000099920, -76.43301270189223828 ) ) ;
#10195=COLOUR_RGB ( '', 0.31764706, 0.68627451, 0.89019608) ;
#10197=CARTESIAN_POINT ( 'NONE',  ( 3.464101615137852974, 5.999999999999884537, -79.91367513459479710 ) ) ;
#10199=CARTESIAN_POINT ( 'NONE',  ( 0.000000000000000000, 0.000000000000000000, 0.000000000000000000 ) ) ;
#10201=CARTESIAN_POINT ( 'NONE',  ( -3.175426480542816066, -5.500000000000057732, -140.3750000000000568 ) ) ;
#10202=CARTESIAN_POINT ( 'NONE',  ( 6.000000000000000888, 5.577813053751546416E-15, -177.0863248654052597 ) ) ;
#10203=CARTESIAN_POINT ( 'NONE',  ( 5.412658773652712085, -3.125000000000086153, -153.9330127018922383 ) ) ;
#10204=CARTESIAN_POINT ( 'NONE',  ( 3.464101615137757051, -5.999999999999979572, -70.83632486540518869 ) ) ;
#10206=CARTESIAN_POINT ( 'NONE',  ( 6.350852961086080661, -9.614813431917819062E-14, -67.87500000000002842 ) ) ;
#10209=CARTESIAN_POINT ( 'NONE',  ( -2.775557561562891351E-14, -5.500000000000115463, -57.75000000000002132 ) ) ;
#10210=( BOUNDED_CURVE ( )  B_SPLINE_CURVE ( 2, ( #19028, #28635, #21166, #16584, #2556, #28346, #7322, #19165, #4999 ),
 .UNSPECIFIED., .F., .T. ) 
 B_SPLINE_CURVE_WITH_KNOTS ( ( 3, 2, 2, 2, 3 ),
 ( 0.09722222222222220989, 0.09814814814814809552, 0.09999999999999997780, 0.1018518518518518601, 0.1027777777777777457 ),
 .UNSPECIFIED. ) 
 CURVE ( )  GEOMETRIC_REPRESENTATION_ITEM ( )  RATIONAL_B_SPLINE_CURVE ( ( 0.9330127018922194093, 0.9330127018922194093, 1.000000000000000000, 0.8660254037844388186, 1.000000000000000000, 0.8660254037844388186, 1.000000000000000000, 0.9330127018922234061, 0.9330127018922194093 ) ) 
 REPRESENTATION_ITEM ( '' )  );
#10217=CARTESIAN_POINT ( 'NONE',  ( -5.196152422706573404, -3.000000000000002665, -104.7886751345948397 ) ) ;
#10219=( BOUNDED_CURVE ( )  B_SPLINE_CURVE ( 2, ( #15787, #29392, #25091, #12709, #6057, #8360, #26772, #5738, #8194 ),
 .UNSPECIFIED., .F., .T. ) 
 B_SPLINE_CURVE_WITH_KNOTS ( ( 3, 2, 2, 2, 3 ),
 ( 0.6694444444444443976, 0.6703703703703703942, 0.6722222222222222765, 0.6740740740740740478, 0.6750000000000000444 ),
 .UNSPECIFIED. ) 
 CURVE ( )  GEOMETRIC_REPRESENTATION_ITEM ( )  RATIONAL_B_SPLINE_CURVE ( ( 0.9330127018922194093, 0.9330127018922154125, 1.000000000000000000, 0.8660254037844388186, 1.000000000000000000, 0.8660254037844388186, 1.000000000000000000, 0.9330127018922154125, 0.9330127018922194093 ) ) 
 REPRESENTATION_ITEM ( '' )  );
#10224=CARTESIAN_POINT ( 'NONE',  ( 3.608439182435180470, 6.249999999999982236, -46.19198729810782567 ) ) ;
#10226=CARTESIAN_POINT ( 'NONE',  ( 3.608439182435180470, -6.249999999999997335, -153.1919872981078186 ) ) ;
#10228=ADVANCED_FACE ( 'NONE', ( #15365 ), #24689, .T. ) ;
#10229=CARTESIAN_POINT ( 'NONE',  ( 3.175426480543072749, -5.500000000000105693, -84.62499999999998579 ) ) ;
#10231=CARTESIAN_POINT ( 'NONE',  ( -7.216878364870328078, 0.000000000000000000, -97.55801270189222407 ) ) ;
#10234=CARTESIAN_POINT ( 'NONE',  ( 5.195867772253143890, -9.698547982442518034, -21.97454809331924608 ) ) ;
#10238=ADVANCED_FACE ( 'NONE', ( #6715 ), #1957, .T. ) ;
#10239=CARTESIAN_POINT ( 'NONE',  ( 0.000000000000000000, 5.499999999999991118, -165.0000000000000284 ) ) ;
#10241=CARTESIAN_POINT ( 'NONE',  ( 6.350852961086080661, -9.614813431917819062E-14, -144.3750000000000568 ) ) ;
#10245=CARTESIAN_POINT ( 'NONE',  ( 0.000000000000000000, 5.499999999999991118, -91.50000000000002842 ) ) ;
#10246=CARTESIAN_POINT ( 'NONE',  ( -5.196152422706601826, 2.999999999999975131, -125.4613248654052313 ) ) ;
#10248=CARTESIAN_POINT ( 'NONE',  ( -3.175426480542816510, 5.499999999999865885, -83.87500000000004263 ) ) ;
#10249=CARTESIAN_POINT ( 'NONE',  ( 5.196152422706629359, 3.000000000000002665, -143.9613248654052597 ) ) ;
#10250=CARTESIAN_POINT ( 'NONE',  ( -3.464101615137725076, 5.999999999999979572, -124.6636751345948113 ) ) ;
#10251=CARTESIAN_POINT ( 'NONE',  ( -3.464101615137757051, -5.999999999999979572, -74.08632486540518869 ) ) ;
#10252=FACE_OUTER_BOUND ( 'NONE', #7796, .T. ) ;
#10255=CARTESIAN_POINT ( 'NONE',  ( -3.464101615137725076, 5.999999999999979572, -178.6636751345948255 ) ) ;
#10256=ORIENTED_EDGE ( 'NONE', *, *, #25458, .F. ) ;
#10257=ORIENTED_EDGE ( 'NONE', *, *, #25965, .F. ) ;
#10258=VERTEX_POINT ( 'NONE', #25758 ) ;
#10260=CARTESIAN_POINT ( 'NONE',  ( 0.000000000000000000, 5.499999999999991118, -107.9999999999999858 ) ) ;
#10262=CARTESIAN_POINT ( 'NONE',  ( -3.608439182435115633, 6.249999999999965361, -121.8080127018921957 ) ) ;
#10264=CARTESIAN_POINT ( 'NONE',  ( 6.000000000000000888, -1.607695154586752384, -110.2306624327026157 ) ) ;
#10265=CARTESIAN_POINT ( 'NONE',  ( -3.608439182435052128, -6.250000000000110134, -159.4419872981077617 ) ) ;
#10267=CARTESIAN_POINT ( 'NONE',  ( 5.412658773652739619, 3.124999999999988898, -62.18301270189224539 ) ) ;
#10270=EDGE_CURVE ( 'NONE', #16308, #3499, #15249, .T. ) ;
#10271=CARTESIAN_POINT ( 'NONE',  ( -5.999999999999982236, -1.607695154586700426, -119.8466878364870496 ) ) ;
#10272=CARTESIAN_POINT ( 'NONE',  ( 0.000000000000000000, 0.000000000000000000, 0.000000000000000000 ) ) ;
#10273=CARTESIAN_POINT ( 'NONE',  ( 6.000000000000000000, 2.951592740943527306E-14, -160.5863248654052313 ) ) ;
#10274=CARTESIAN_POINT ( 'NONE',  ( -6.350852961085760029, -1.281975124255709124E-13, -170.6250000000000284 ) ) ;
#10277=CARTESIAN_POINT ( 'NONE',  ( -3.608439182435052128, -6.250000000000110134, -166.3080127018922667 ) ) ;
#10278=CARTESIAN_POINT ( 'NONE',  ( 0.000000000000000000, 5.999999999999977796, -48.28867513459483973 ) ) ;
#10280=CARTESIAN_POINT ( 'NONE',  ( -6.350852961085760029, -1.281975124255709124E-13, -115.1250000000000000 ) ) ;
#10282=CARTESIAN_POINT ( 'NONE',  ( 3.175426480543072749, -5.500000000000105693, -105.6250000000000142 ) ) ;
#10286=CARTESIAN_POINT ( 'NONE',  ( -5.196152422706601826, 2.999999999999975131, -86.46132486540525974 ) ) ;
#10287=ORIENTED_EDGE ( 'NONE', *, *, #18222, .T. ) ;
#10288=CARTESIAN_POINT ( 'NONE',  ( -3.608439182435115633, 6.249999999999965361, -80.44198729810779014 ) ) ;
#10290=ORIENTED_EDGE ( 'NONE', *, *, #21025, .F. ) ;
#10294=ORIENTED_EDGE ( 'NONE', *, *, #24589, .T. ) ;
#10297=EDGE_CURVE ( 'NONE', #11265, #7855, #24626, .T. ) ;
#10298=( BOUNDED_CURVE ( )  B_SPLINE_CURVE ( 2, ( #447, #21811, #14903, #19078, #19214, #7804, #7961, #304, #17220 ),
 .UNSPECIFIED., .F., .T. ) 
 B_SPLINE_CURVE_WITH_KNOTS ( ( 3, 2, 2, 2, 3 ),
 ( 0.5305555555555555580, 0.5314814814814814437, 0.5333333333333333259, 0.5351851851851852082, 0.5361111111111110938 ),
 .UNSPECIFIED. ) 
 CURVE ( )  GEOMETRIC_REPRESENTATION_ITEM ( )  RATIONAL_B_SPLINE_CURVE ( ( 0.9330127018922194093, 0.9330127018922194093, 1.000000000000000000, 0.8660254037844388186, 1.000000000000000000, 0.8660254037844388186, 1.000000000000000000, 0.9330127018922234061, 0.9330127018922194093 ) ) 
 REPRESENTATION_ITEM ( '' )  );
#10300=CARTESIAN_POINT ( 'NONE',  ( 5.412658773652739619, 3.124999999999988898, -133.3169872981078186 ) ) ;
#10305=CARTESIAN_POINT ( 'NONE',  ( 6.000000000000026645, -1.607695154586707753, -138.7306624327025872 ) ) ;
#10306=CYLINDRICAL_SURFACE ( 'NONE', #21098, 6.000000000000000888 ) ;
#10309=CARTESIAN_POINT ( 'NONE',  ( 7.216878364870455975, -6.409875621278545621E-14, -65.94198729810784698 ) ) ;
#10310=CARTESIAN_POINT ( 'NONE',  ( 7.216878364870455975, -6.409875621278545621E-14, -53.94198729810779724 ) ) ;
#10311=CARTESIAN_POINT ( 'NONE',  ( 6.000000000000000888, 7.762456499804234384E-14, -128.1636751345948539 ) ) ;
#10313=CARTESIAN_POINT ( 'NONE',  ( -5.196152422706601826, 2.999999999999975131, -74.46132486540524553 ) ) ;
#10314=AXIS2_PLACEMENT_3D ( 'NONE', #7161, #18865, #9167 ) ;
#10315=CARTESIAN_POINT ( 'NONE',  ( -4.763139720814407951, 2.749999999999946709, -140.7500000000000284 ) ) ;
#10320=CARTESIAN_POINT ( 'NONE',  ( -4.763139720814407951, 2.749999999999946709, -50.75000000000001421 ) ) ;
#10328=CARTESIAN_POINT ( 'NONE',  ( -3.608439182435052128, -6.250000000000110134, -93.44198729810786119 ) ) ;
#10329=CARTESIAN_POINT ( 'NONE',  ( -5.196152422706573404, -3.000000000000002665, -78.71132486540521711 ) ) ;
#10333=CARTESIAN_POINT ( 'NONE',  ( 5.196152422706629359, 3.000000000000002665, -77.96132486540518869 ) ) ;
#10339=CARTESIAN_POINT ( 'NONE',  ( 4.763139720814407951, -2.749999999999988454, -60.50000000000000000 ) ) ;
#10340=CARTESIAN_POINT ( 'NONE',  ( -3.464101615137757051, -5.999999999999979572, -51.58632486540522422 ) ) ;
#10342=CARTESIAN_POINT ( 'NONE',  ( -3.608439182435052128, -6.250000000000110134, -74.80801270189222407 ) ) ;
#10345=CARTESIAN_POINT ( 'NONE',  ( -5.999999999999963585, 9.296355089585909904E-15, -168.8363248654052029 ) ) ;
#10346=CARTESIAN_POINT ( 'NONE',  ( 6.000000000000000888, -1.859271017917181981E-14, -80.16367513459481131 ) ) ;
#10348=CARTESIAN_POINT ( 'NONE',  ( -5.196152422706573404, -3.000000000000002665, -94.28867513459482552 ) ) ;
#10349=CARTESIAN_POINT ( 'NONE',  ( 4.763139720814407951, 2.750000000000002665, -135.2500000000000284 ) ) ;
#10351=CARTESIAN_POINT ( 'NONE',  ( 6.000000000000000888, -1.859271017917181981E-14, -170.1636751345948539 ) ) ;
#10354=CARTESIAN_POINT ( 'NONE',  ( -4.763139720814407951, 2.749999999999946709, -70.25000000000002842 ) ) ;
#10355=CARTESIAN_POINT ( 'NONE',  ( -3.175426480542816510, -5.500000000000057732, -60.87500000000000000 ) ) ;
#10356=AXIS2_PLACEMENT_3D ( 'NONE', #21911, #22057, #17466 ) ;
#10357=ORIENTED_EDGE ( 'NONE', *, *, #19213, .T. ) ;
#10361=CARTESIAN_POINT ( 'NONE',  ( -5.999999999999963585, -1.487416814333745711E-14, -126.8363248654052171 ) ) ;
#10364=CARTESIAN_POINT ( 'NONE',  ( 5.196152422706629359, -2.999999999999988898, -57.78867513459484684 ) ) ;
#10365=ORIENTED_EDGE ( 'NONE', *, *, #22387, .T. ) ;
#10367=CARTESIAN_POINT ( 'NONE',  ( 6.000000000000000888, 7.762456499804235646E-14, -140.1636751345948255 ) ) ;
#10369=DIRECTION ( 'NONE',  ( 1.000000000000000000, -5.551115123125773458E-17, -1.260129944081490338E-35 ) ) ;
#10370=ADVANCED_FACE ( 'NONE', ( #12868 ), #8369, .T. ) ;
#10371=CARTESIAN_POINT ( 'NONE',  ( 6.350852961086080661, -9.614813431917819062E-14, -180.3750000000000284 ) ) ;
#10373=CARTESIAN_POINT ( 'NONE',  ( 3.608439182435180470, 6.249999999999982236, -146.6919872981078470 ) ) ;
#10374=CARTESIAN_POINT ( 'NONE',  ( -4.763139720814407951, -2.750000000000016431, -83.50000000000001421 ) ) ;
#10375=VECTOR ( 'NONE', #1600, 1000.000000000000000 ) ;
#10376=CARTESIAN_POINT ( 'NONE',  ( -5.412658773652684552, -3.125000000000099920, -92.93301270189225249 ) ) ;
#10377=ORIENTED_EDGE ( 'NONE', *, *, #14457, .T. ) ;
#10381=CARTESIAN_POINT ( 'NONE',  ( -5.196152422706573404, -3.000000000000002665, -151.2886751345948824 ) ) ;
#10382=CARTESIAN_POINT ( 'NONE',  ( 6.000000000000000888, -1.859271017917181981E-14, -120.0863248654052313 ) ) ;
#10384=( BOUNDED_CURVE ( )  B_SPLINE_CURVE ( 2, ( #21390, #2628, #18952, #5072, #9712, #12049, #322, #14500, #19094 ),
 .UNSPECIFIED., .F., .T. ) 
 B_SPLINE_CURVE_WITH_KNOTS ( ( 3, 2, 2, 2, 3 ),
 ( 0.8972222222222222543, 0.8981481481481481399, 0.9000000000000000222, 0.9018518518518519045, 0.9027777777777777901 ),
 .UNSPECIFIED. ) 
 CURVE ( )  GEOMETRIC_REPRESENTATION_ITEM ( )  RATIONAL_B_SPLINE_CURVE ( ( 0.9330127018922194093, 0.9330127018922234061, 1.000000000000000000, 0.8660254037844388186, 1.000000000000000000, 0.8660254037844388186, 1.000000000000000000, 0.9330127018922194093, 0.9330127018922194093 ) ) 
 REPRESENTATION_ITEM ( '' )  );
#10385=CARTESIAN_POINT ( 'NONE',  ( -4.763139720814407951, 2.749999999999946709, -164.7500000000000000 ) ) ;
#10386=DIRECTION ( 'NONE',  ( -7.147005652999508048E-36, 5.642372883946980038E-36, 1.000000000000000000 ) ) ;
#10388=CARTESIAN_POINT ( 'NONE',  ( 4.763139720814407951, 2.750000000000002665, -144.2500000000000000 ) ) ;
#10390=CARTESIAN_POINT ( 'NONE',  ( 5.196152422706629359, -2.999999999999988898, -92.28867513459482552 ) ) ;
#10392=CARTESIAN_POINT ( 'NONE',  ( -3.175426480542816066, -5.500000000000057732, -95.37500000000002842 ) ) ;
#10393=CARTESIAN_POINT ( 'NONE',  ( 0.000000000000000000, -5.999999999999991118, -130.9613248654052313 ) ) ;
#10394=CARTESIAN_POINT ( 'NONE',  ( -3.175426480542816510, 5.499999999999865885, -85.37500000000004263 ) ) ;
#10396=CARTESIAN_POINT ( 'NONE',  ( 3.464101615137757051, -5.999999999999979572, -108.3363248654052171 ) ) ;
#10400=CARTESIAN_POINT ( 'NONE',  ( 5.196152422706629359, 3.000000000000002665, -128.9613248654052313 ) ) ;
#10401=CARTESIAN_POINT ( 'NONE',  ( 0.000000000000000000, 5.999999999999977796, -174.2886751345948255 ) ) ;
#10404=CYLINDRICAL_SURFACE ( 'NONE', #21444, 6.000000000000000888 ) ;
#10405=CARTESIAN_POINT ( 'NONE',  ( -5.999999999999919176, 1.607695154586804565, -82.48066243270260145 ) ) ;
#10407=CARTESIAN_POINT ( 'NONE',  ( -5.999999999999963585, 8.134310703387671600E-14, -116.3363248654052313 ) ) ;
#10408=EDGE_LOOP ( 'NONE', ( #25282, #5474, #25802, #2325 ) ) ;
#10411=AXIS2_PLACEMENT_3D ( 'NONE', #24943, #20049, #3894 ) ;
#10412=CARTESIAN_POINT ( 'NONE',  ( -6.350852961085760029, -1.281975124255709124E-13, -101.6250000000000000 ) ) ;
#10413=CARTESIAN_POINT ( 'NONE',  ( -3.608439182435052128, -6.250000000000110134, -115.3080127018922241 ) ) ;
#10414=ORIENTED_EDGE ( 'NONE', *, *, #27826, .T. ) ;
#10416=CARTESIAN_POINT ( 'NONE',  ( -3.608439182435115633, 6.249999999999965361, -161.4419872981077901 ) ) ;
#10418=CARTESIAN_POINT ( 'NONE',  ( -5.412658773652739619, 3.124999999999975131, -58.68301270189224539 ) ) ;
#10419=VERTEX_POINT ( 'NONE', #22667 ) ;
#10424=CARTESIAN_POINT ( 'NONE',  ( 4.763139720814407951, 2.750000000000002665, -171.2500000000000000 ) ) ;
#10428=CARTESIAN_POINT ( 'NONE',  ( -3.608439182435115633, 6.249999999999965361, -171.3080127018922383 ) ) ;
#10432=CARTESIAN_POINT ( 'NONE',  ( 4.763139720814407951, 2.750000000000002665, -112.7500000000000142 ) ) ;
#10434=CARTESIAN_POINT ( 'NONE',  ( 6.350852961086080661, -9.614813431917819062E-14, -102.3750000000000000 ) ) ;
#10435=CARTESIAN_POINT ( 'NONE',  ( 6.000000000000000888, -1.859271017917181981E-14, -145.5863248654052029 ) ) ;
#10441=CARTESIAN_POINT ( 'NONE',  ( -4.763139720814407951, 2.749999999999946709, -160.2500000000000000 ) ) ;
#10442=CARTESIAN_POINT ( 'NONE',  ( 2.775557561562891351E-14, -6.250000000000061284, -81.31698729810781856 ) ) ;
#10445=EDGE_CURVE ( 'NONE', #22536, #18017, #497, .T. ) ;
#10450=CARTESIAN_POINT ( 'NONE',  ( -5.412658773652684552, -3.125000000000099920, -142.4330127018922383 ) ) ;
#10451=ORIENTED_EDGE ( 'NONE', *, *, #28736, .T. ) ;
#10452=CARTESIAN_POINT ( 'NONE',  ( -3.608439182435052128, -6.250000000000110134, -135.4419872981078186 ) ) ;
#10454=CARTESIAN_POINT ( 'NONE',  ( -5.999999999999919176, 1.607695154586804565, -49.48066243270260856 ) ) ;
#10456=VERTEX_POINT ( 'NONE', #3109 ) ;
#10460=CARTESIAN_POINT ( 'NONE',  ( 6.000000000000000888, 5.577813053751546416E-15, -165.6636751345948255 ) ) ;
#10463=CARTESIAN_POINT ( 'NONE',  ( -5.412658773652684552, -3.125000000000099920, -65.06698729810783277 ) ) ;
#10464=CARTESIAN_POINT ( 'NONE',  ( 3.608439182435180470, -6.249999999999997335, -51.19198729810784698 ) ) ;
#10469=CARTESIAN_POINT ( 'NONE',  ( 4.763139720814407951, -2.749999999999988454, -128.0000000000000000 ) ) ;
#10471=CARTESIAN_POINT ( 'NONE',  ( -3.464101615137725076, 5.999999999999979572, -166.6636751345947971 ) ) ;
#10478=EDGE_CURVE ( 'NONE', #21171, #14517, #6787, .T. ) ;
#10481=ORIENTED_EDGE ( 'NONE', *, *, #5311, .T. ) ;
#10485=CARTESIAN_POINT ( 'NONE',  ( -5.412658773652684552, -3.125000000000099920, -96.56698729810780435 ) ) ;
#10486=CARTESIAN_POINT ( 'NONE',  ( 6.000000000000000888, 1.607695154586715303, -173.0966878364870354 ) ) ;
#10494=CARTESIAN_POINT ( 'NONE',  ( 0.000000000000000000, 5.499999999999991118, -48.00000000000004263 ) ) ;
#10495=CARTESIAN_POINT ( 'NONE',  ( 6.000000000000052403, -1.607695154586662678, -51.15331216351301435 ) ) ;
#10496=CARTESIAN_POINT ( 'NONE',  ( 2.775557561562891351E-14, -6.250000000000061284, -77.68301270189226670 ) ) ;
#10498=CARTESIAN_POINT ( 'NONE',  ( -5.999999999999963585, 8.134310703387671600E-14, -141.8363248654052029 ) ) ;
#10502=CARTESIAN_POINT ( 'NONE',  ( -3.175426480542816066, -5.500000000000057732, -128.3750000000000000 ) ) ;
#10504=CARTESIAN_POINT ( 'NONE',  ( -3.608439182435052128, -6.250000000000110134, -148.3080127018922667 ) ) ;
#10505=CARTESIAN_POINT ( 'NONE',  ( -5.999999999999962697, 3.323446944526963260E-14, -158.3363248654052313 ) ) ;
#10506=CARTESIAN_POINT ( 'NONE',  ( 0.000000000000000000, 5.499999999999991118, -64.50000000000000000 ) ) ;
#10507=CARTESIAN_POINT ( 'NONE',  ( -3.175426480542816510, -5.500000000000057732, -56.37500000000004263 ) ) ;
#10508=EDGE_CURVE ( 'NONE', #14874, #19083, #13117, .T. ) ;
#10510=ORIENTED_EDGE ( 'NONE', *, *, #8328, .T. ) ;
#10512=CARTESIAN_POINT ( 'NONE',  ( 6.000000000000026645, -1.607695154586707753, -117.7306624327026299 ) ) ;
#10515=CARTESIAN_POINT ( 'NONE',  ( 0.000000000000000000, -5.999999999999991118, -58.03867513459481842 ) ) ;
#10521=CARTESIAN_POINT ( 'NONE',  ( 4.763139720814407951, -2.749999999999988454, -147.5000000000000284 ) ) ;
#10522=CARTESIAN_POINT ( 'NONE',  ( 7.216878364870455975, -6.409875621278545621E-14, -49.44198729810784698 ) ) ;
#10524=ORIENTED_EDGE ( 'NONE', *, *, #7774, .F. ) ;
#10525=CARTESIAN_POINT ( 'NONE',  ( -5.412658773652739619, 3.124999999999975131, -146.3169872981078186 ) ) ;
#10526=CARTESIAN_POINT ( 'NONE',  ( 0.000000000000000000, 5.499999999999991118, -70.50000000000000000 ) ) ;
#10528=CARTESIAN_POINT ( 'NONE',  ( -3.608439182435115633, 6.249999999999965361, -91.80801270189225249 ) ) ;
#10534=FACE_OUTER_BOUND ( 'NONE', #5930, .T. ) ;
#10536=CARTESIAN_POINT ( 'NONE',  ( 6.350852961086080661, -9.614813431917819062E-14, -156.3750000000000000 ) ) ;
#10537=FACE_OUTER_BOUND ( 'NONE', #24066, .T. ) ;
#10538=CARTESIAN_POINT ( 'NONE',  ( -3.175426480542816510, 5.499999999999865885, -143.8750000000000000 ) ) ;
#10540=CARTESIAN_POINT ( 'NONE',  ( 6.000000000000052403, -1.607695154586662678, -92.23066243270260145 ) ) ;
#10541=CARTESIAN_POINT ( 'NONE',  ( 4.763139720814407951, 2.750000000000002665, -90.25000000000005684 ) ) ;
#10542=CARTESIAN_POINT ( 'NONE',  ( 6.000000000000000888, 1.743066579297358182E-13, -66.08632486540521711 ) ) ;
#10543=CARTESIAN_POINT ( 'NONE',  ( -6.350852961085760029, -1.281975124255709124E-13, -77.62500000000001421 ) ) ;
#10544=ADVANCED_FACE ( 'NONE', ( #3867 ), #22326, .T. ) ;
#10547=CARTESIAN_POINT ( 'NONE',  ( 6.000000000000000888, -1.859271017917181981E-14, -109.5863248654052029 ) ) ;
#10548=CARTESIAN_POINT ( 'NONE',  ( -5.999999999999963585, 1.780251999655701777E-13, -98.33632486540520290 ) ) ;
#10549=CARTESIAN_POINT ( 'NONE',  ( 6.000000000000000888, 1.607695154586715303, -135.0193375672974412 ) ) ;
#10550=CARTESIAN_POINT ( 'NONE',  ( 6.000000000000001776, 5.345404176511898156E-15, -174.6636751345948539 ) ) ;
#10554=DIRECTION ( 'NONE',  ( -7.147005652999508048E-36, 5.642372883946980038E-36, 1.000000000000000000 ) ) ;
#10557=ORIENTED_EDGE ( 'NONE', *, *, #3195, .T. ) ;
#10558=ORIENTED_EDGE ( 'NONE', *, *, #20957, .T. ) ;
#10559=CARTESIAN_POINT ( 'NONE',  ( 0.000000000000000000, 5.499999999999991118, -106.5000000000000426 ) ) ;
#10563=CARTESIAN_POINT ( 'NONE',  ( 5.412658773652712085, -3.125000000000086153, -117.9330127018922667 ) ) ;
#10564=VERTEX_POINT ( 'NONE', #17739 ) ;
#10569=AXIS2_PLACEMENT_3D ( 'NONE', #29755, #18121, #1498 ) ;
#10571=CARTESIAN_POINT ( 'NONE',  ( 5.412658773652712085, -3.125000000000086153, -50.43301270189226670 ) ) ;
#10573=CARTESIAN_POINT ( 'NONE',  ( -5.196152422706601826, 2.999999999999975131, -167.4613248654052029 ) ) ;
#10574=CARTESIAN_POINT ( 'NONE',  ( 0.000000000000000000, -5.999999999999991118, -56.53867513459481842 ) ) ;
#10575=CARTESIAN_POINT ( 'NONE',  ( 6.000000000000052403, -1.607695154586662678, -61.65331216351297883 ) ) ;
#10577=CARTESIAN_POINT ( 'NONE',  ( 4.763139720814407951, 2.750000000000002665, -174.2500000000000284 ) ) ;
#10579=CARTESIAN_POINT ( 'NONE',  ( -5.196152422706601826, 2.999999999999975131, -107.4613248654052171 ) ) ;
#10580=CARTESIAN_POINT ( 'NONE',  ( 2.775557561562891351E-14, 6.250000000000033751, -168.4330127018922667 ) ) ;
#10582=AXIS2_PLACEMENT_3D ( 'NONE', #24357, #8541, #15653 ) ;
#10583=CARTESIAN_POINT ( 'NONE',  ( -3.175426480542816066, -5.500000000000057732, -114.8749999999999858 ) ) ;
#10585=EDGE_CURVE ( 'NONE', #29768, #23369, #16262, .T. ) ;
#10586=CARTESIAN_POINT ( 'NONE',  ( 6.350852961086080661, -9.614813431917819062E-14, -106.8750000000000142 ) ) ;
#10587=CARTESIAN_POINT ( 'NONE',  ( -5.196152422706601826, 2.999999999999975131, -142.5386751345948255 ) ) ;
#10588=FILL_AREA_STYLE_COLOUR ( '', #21094 ) ;
#10594=CARTESIAN_POINT ( 'NONE',  ( -6.000000000000007105, -1.607695154586655129, -146.2693375672974412 ) ) ;
#10596=CARTESIAN_POINT ( 'NONE',  ( 6.000000000000000888, 1.743066579297358182E-13, -66.08632486540521711 ) ) ;
#10597=CARTESIAN_POINT ( 'NONE',  ( -5.412658773652684552, -3.125000000000099920, -78.56698729810784698 ) ) ;
#10599=ORIENTED_EDGE ( 'NONE', *, *, #14582, .T. ) ;
#10603=CARTESIAN_POINT ( 'NONE',  ( 5.412658773652712085, -3.125000000000086153, -140.4330127018922383 ) ) ;
#10605=CARTESIAN_POINT ( 'NONE',  ( 5.412658773652712085, -3.125000000000086153, -124.5669872981078328 ) ) ;
#10606=CARTESIAN_POINT ( 'NONE',  ( -4.763139720814407951, -2.750000000000016431, -173.5000000000000000 ) ) ;
#10607=CARTESIAN_POINT ( 'NONE',  ( -5.196152422706601826, 2.999999999999975131, -83.46132486540524553 ) ) ;
#10612=DIRECTION ( 'NONE',  ( 1.000000000000000000, -5.551115123125773458E-17, -1.260129944081490338E-35 ) ) ;
#10613=DIRECTION ( 'NONE',  ( 1.000000000000000000, -5.551115123125773458E-17, -1.260129944081490338E-35 ) ) ;
#10614=DIRECTION ( 'NONE',  ( -7.147005652999508048E-36, 5.642372883946980038E-36, 1.000000000000000000 ) ) ;
#10619=CARTESIAN_POINT ( 'NONE',  ( 3.608439182435180470, -6.249999999999997335, -66.19198729810779014 ) ) ;
#10621=CARTESIAN_POINT ( 'NONE',  ( 3.608439182435180470, 6.249999999999982236, -53.69198729810779724 ) ) ;
#10623=CARTESIAN_POINT ( 'NONE',  ( 0.000000000000000000, -5.999999999999991118, -64.03867513459482552 ) ) ;
#10626=ADVANCED_FACE ( 'NONE', ( #29988 ), #14071, .T. ) ;
#10627=CARTESIAN_POINT ( 'NONE',  ( -6.350852961085760029, -1.281975124255709124E-13, -125.6250000000000426 ) ) ;
#10633=CARTESIAN_POINT ( 'NONE',  ( 0.000000000000000000, 5.999999999999977796, -119.7113248654052597 ) ) ;
#10638=CARTESIAN_POINT ( 'NONE',  ( -5.196152422706601826, 2.999999999999975131, -71.46132486540524553 ) ) ;
#10639=CARTESIAN_POINT ( 'NONE',  ( 3.608439182435180470, -6.249999999999997335, -99.19198729810781856 ) ) ;
#10643=EDGE_LOOP ( 'NONE', ( #4230, #1863, #572, #28648 ) ) ;
#10644=CARTESIAN_POINT ( 'NONE',  ( -5.999999999999963585, 1.780251999655701777E-13, -77.33632486540524553 ) ) ;
#10648=CARTESIAN_POINT ( 'NONE',  ( -4.763139720814407951, 2.749999999999946709, -49.25000000000001421 ) ) ;
#10652=CARTESIAN_POINT ( 'NONE',  ( -5.999999999999963585, 1.780251999655701777E-13, -62.91367513459483973 ) ) ;
#10653=DIRECTION ( 'NONE',  ( 1.000000000000000000, -5.551115123125773458E-17, -1.260129944081490338E-35 ) ) ;
#10654=CARTESIAN_POINT ( 'NONE',  ( -3.608439182435052128, -6.250000000000110134, -71.80801270189222407 ) ) ;
#10658=CARTESIAN_POINT ( 'NONE',  ( 0.000000000000000000, 0.000000000000000000, 0.000000000000000000 ) ) ;
#10660=CARTESIAN_POINT ( 'NONE',  ( 5.999999999999999112, 2.951592740943527306E-14, -152.1636751345948255 ) ) ;
#10662=CARTESIAN_POINT ( 'NONE',  ( 3.464101615137852974, 5.999999999999884537, -104.8363248654052029 ) ) ;
#10663=ADVANCED_FACE ( 'NONE', ( #23406 ), #9416, .T. ) ;
#10665=CARTESIAN_POINT ( 'NONE',  ( 6.350852961086080661, -9.614813431917819062E-14, -133.8750000000000284 ) ) ;
#10668=LINE ( 'NONE', #1257, #9623 ) ;
#10670=CARTESIAN_POINT ( 'NONE',  ( 0.000000000000000000, 5.499999999999991118, -60.00000000000005684 ) ) ;
#10671=CARTESIAN_POINT ( 'NONE',  ( 4.763139720814407951, -2.749999999999988454, -57.49999999999999289 ) ) ;
#10672=( BOUNDED_CURVE ( )  B_SPLINE_CURVE ( 2, ( #18655, #16219, #14072, #27974, #4934, #30, #14365, #28131, #23104 ),
 .UNSPECIFIED., .F., .T. ) 
 B_SPLINE_CURVE_WITH_KNOTS ( ( 3, 2, 2, 2, 3 ),
 ( 0.9805555555555555136, 0.9814814814814815103, 0.9833333333333332815, 0.9851851851851851638, 0.9861111111111111605 ),
 .UNSPECIFIED. ) 
 CURVE ( )  GEOMETRIC_REPRESENTATION_ITEM ( )  RATIONAL_B_SPLINE_CURVE ( ( 0.9330127018922194093, 0.9330127018922154125, 1.000000000000000000, 0.8660254037844388186, 1.000000000000000000, 0.8660254037844388186, 1.000000000000000000, 0.9330127018922154125, 0.9330127018922194093 ) ) 
 REPRESENTATION_ITEM ( '' )  );
#10673=CARTESIAN_POINT ( 'NONE',  ( -6.000000000000007105, -1.607695154586655129, -174.7693375672974412 ) ) ;
#10674=ORIENTED_EDGE ( 'NONE', *, *, #14755, .F. ) ;
#10686=CARTESIAN_POINT ( 'NONE',  ( 5.196152422706629359, -2.999999999999988898, -121.7113248654052597 ) ) ;
#10688=CARTESIAN_POINT ( 'NONE',  ( 3.175426480543072749, -5.500000000000105693, -147.6250000000000284 ) ) ;
#10690=ORIENTED_EDGE ( 'NONE', *, *, #8183, .T. ) ;
#10691=CARTESIAN_POINT ( 'NONE',  ( -7.216878364870328078, 0.000000000000000000, -146.1919872981078470 ) ) ;
#10692=CARTESIAN_POINT ( 'NONE',  ( -4.763139720814407951, 2.749999999999946709, -70.25000000000002842 ) ) ;
#10693=EDGE_CURVE ( 'NONE', #18702, #3793, #19369, .T. ) ;
#10694=EDGE_CURVE ( 'NONE', #10419, #13111, #10949, .T. ) ;
#10695=CARTESIAN_POINT ( 'NONE',  ( 5.412658773652712085, -3.125000000000086153, -90.93301270189225249 ) ) ;
#10697=CARTESIAN_POINT ( 'NONE',  ( -5.799430203125090166, -9.347489878302569721, -23.41021253818530923 ) ) ;
#10698=CARTESIAN_POINT ( 'NONE',  ( 0.000000000000000000, -5.999999999999991118, -96.46132486540520290 ) ) ;
#10700=CARTESIAN_POINT ( 'NONE',  ( -6.000000000000007105, -1.607695154586655129, -86.84668783648706381 ) ) ;
#10701=DIRECTION ( 'NONE',  ( 1.000000000000000000, -5.551115123125773458E-17, -1.260129944081490338E-35 ) ) ;
#10704=CARTESIAN_POINT ( 'NONE',  ( -6.350852961085760029, -1.281975124255709124E-13, -154.1250000000000568 ) ) ;
#10705=CYLINDRICAL_SURFACE ( 'NONE', #10411, 6.000000000000000888 ) ;
#10706=CARTESIAN_POINT ( 'NONE',  ( -2.775557561562891351E-14, -5.500000000000115463, -149.2500000000000000 ) ) ;
#10709=CARTESIAN_POINT ( 'NONE',  ( 6.350852961086080661, -9.614813431917819062E-14, -82.87500000000004263 ) ) ;
#10710=FACE_OUTER_BOUND ( 'NONE', #28557, .T. ) ;
#10711=CARTESIAN_POINT ( 'NONE',  ( -6.350852961085760029, -1.281975124255709124E-13, -83.62499999999998579 ) ) ;
#10712=DIRECTION ( 'NONE',  ( -7.147005652999508048E-36, 5.642372883946980038E-36, 1.000000000000000000 ) ) ;
#10716=VECTOR ( 'NONE', #24206, 1000.000000000000000 ) ;
#10717=( BOUNDED_CURVE ( )  B_SPLINE_CURVE ( 2, ( #24031, #14979, #16997, #12103, #26323, #21442, #375, #21745, #9766 ),
 .UNSPECIFIED., .F., .F. ) 
 B_SPLINE_CURVE_WITH_KNOTS ( ( 3, 2, 2, 2, 3 ),
 ( 0.1694444444444444253, 0.1703703703703703665, 0.1722222222222222210, 0.1740740740740740755, 0.1750000000000000167 ),
 .UNSPECIFIED. ) 
 CURVE ( )  GEOMETRIC_REPRESENTATION_ITEM ( )  RATIONAL_B_SPLINE_CURVE ( ( 0.9330127018922196314, 0.9330127018922185211, 1.000000000000000000, 0.8660254037844388186, 1.000000000000000000, 0.8660254037844388186, 1.000000000000000000, 0.9330127018922184101, 0.9330127018922194093 ) ) 
 REPRESENTATION_ITEM ( '' )  );
#10720=( BOUNDED_CURVE ( )  B_SPLINE_CURVE ( 2, ( #26087, #28823, #9817, #5327, #875, #21501, #21938, #285, #3032 ),
 .UNSPECIFIED., .F., .F. ) 
 B_SPLINE_CURVE_WITH_KNOTS ( ( 3, 2, 2, 2, 3 ),
 ( 0.6750000000000000444, 0.6759259259259259300, 0.6777777777777778123, 0.6796296296296295836, 0.6805555555555555802 ),
 .UNSPECIFIED. ) 
 CURVE ( )  GEOMETRIC_REPRESENTATION_ITEM ( )  RATIONAL_B_SPLINE_CURVE ( ( 0.9330127018922194093, 0.9330127018922234061, 1.000000000000000000, 0.8660254037844388186, 1.000000000000000000, 0.8660254037844388186, 1.000000000000000000, 0.9330127018922154125, 0.9330127018922194093 ) ) 
 REPRESENTATION_ITEM ( '' )  );
#10723=ORIENTED_EDGE ( 'NONE', *, *, #5209, .F. ) ;
#10725=CARTESIAN_POINT ( 'NONE',  ( 6.000000000000052403, -1.607695154586662678, -78.73066243270262987 ) ) ;
#10727=ORIENTED_EDGE ( 'NONE', *, *, #19259, .F. ) ;
#10729=CARTESIAN_POINT ( 'NONE',  ( -4.763139720814407951, -2.750000000000016431, -101.5000000000000284 ) ) ;
#10730=FACE_OUTER_BOUND ( 'NONE', #10643, .T. ) ;
#10731=ADVANCED_FACE ( 'NONE', ( #11288 ), #27669, .T. ) ;
#10732=CARTESIAN_POINT ( 'NONE',  ( 5.412658773652712085, -3.125000000000086153, -111.9330127018922667 ) ) ;
#10734=CARTESIAN_POINT ( 'NONE',  ( 6.000000000000000888, -1.859271017917181981E-14, -141.0863248654051745 ) ) ;
#10736=STYLED_ITEM ( 'NONE', ( #7918 ), #17567 ) ;
#10737=LINE ( 'NONE', #19630, #14092 ) ;
#10738=CARTESIAN_POINT ( 'NONE',  ( 2.775557561562891351E-14, -6.250000000000061284, -50.68301270189223828 ) ) ;
#10743=DIRECTION ( 'NONE',  ( -7.147005652999508048E-36, 5.642372883946980038E-36, 1.000000000000000000 ) ) ;
#10744=CARTESIAN_POINT ( 'NONE',  ( 3.175426480543072749, -5.500000000000105693, -170.1250000000000000 ) ) ;
#10747=CARTESIAN_POINT ( 'NONE',  ( -3.608439182435115633, 6.249999999999965361, -172.8080127018922667 ) ) ;
#10748=DIRECTION ( 'NONE',  ( -7.147005652999508048E-36, 5.642372883946980038E-36, 1.000000000000000000 ) ) ;
#10749=CARTESIAN_POINT ( 'NONE',  ( 3.175426480543072749, -5.500000000000105693, -107.1250000000000284 ) ) ;
#10751=CARTESIAN_POINT ( 'NONE',  ( -4.763139720814407951, -2.750000000000016431, -101.5000000000000284 ) ) ;
#10756=CARTESIAN_POINT ( 'NONE',  ( -5.999999999999963585, 1.780251999655701777E-13, -90.83632486540521711 ) ) ;
#10758=ORIENTED_EDGE ( 'NONE', *, *, #21100, .F. ) ;
#10759=CARTESIAN_POINT ( 'NONE',  ( -6.350852961085760029, -1.281975124255709124E-13, -161.6250000000000284 ) ) ;
#10760=CARTESIAN_POINT ( 'NONE',  ( 5.999999999999999112, 2.951592740943527306E-14, -156.6636751345948255 ) ) ;
#10762=EDGE_CURVE ( 'NONE', #9352, #25369, #14113, .T. ) ;
#10763=CARTESIAN_POINT ( 'NONE',  ( -5.412658773652684552, -3.125000000000099920, -83.06698729810779014 ) ) ;
#10765=VERTEX_POINT ( 'NONE', #10019 ) ;
#10769=CARTESIAN_POINT ( 'NONE',  ( -4.763139720814407951, -2.750000000000016431, -119.5000000000000568 ) ) ;
#10770=EDGE_CURVE ( 'NONE', #16190, #22104, #17224, .T. ) ;
#10771=CARTESIAN_POINT ( 'NONE',  ( 2.775557561562891351E-14, -6.250000000000061284, -137.6830127018922099 ) ) ;
#10774=CARTESIAN_POINT ( 'NONE',  ( 5.412658773652739619, 3.124999999999988898, -125.8169872981078612 ) ) ;
#10775=CARTESIAN_POINT ( 'NONE',  ( 6.000000000000000888, -1.859271017917181981E-14, -135.0863248654052029 ) ) ;
#10776=CARTESIAN_POINT ( 'NONE',  ( -2.775557561562891351E-14, -5.500000000000115463, -173.2500000000000284 ) ) ;
#10781=CARTESIAN_POINT ( 'NONE',  ( -5.999999999999963585, -1.487416814333745711E-14, -92.33632486540518869 ) ) ;
#10782=CARTESIAN_POINT ( 'NONE',  ( 6.000000000000000888, 1.743066579297358182E-13, -90.66367513459483973 ) ) ;
#10786=CARTESIAN_POINT ( 'NONE',  ( -3.608439182435115633, 6.249999999999965361, -63.94198729810785409 ) ) ;
#10790=CARTESIAN_POINT ( 'NONE',  ( 3.175426480543072749, -5.500000000000105693, -132.6250000000000000 ) ) ;
#10791=CARTESIAN_POINT ( 'NONE',  ( -5.196152422706601826, 2.999999999999975131, -138.0386751345948255 ) ) ;
#10792=ORIENTED_EDGE ( 'NONE', *, *, #30040, .T. ) ;
#10797=VECTOR ( 'NONE', #24119, 1000.000000000000000 ) ;
#10803=CARTESIAN_POINT ( 'NONE',  ( -7.216878364870328078, 0.000000000000000000, -116.1919872981078328 ) ) ;
#10809=EDGE_CURVE ( 'NONE', #23669, #2929, #20339, .T. ) ;
#10811=ORIENTED_EDGE ( 'NONE', *, *, #21983, .T. ) ;
#10812=VERTEX_POINT ( 'NONE', #7691 ) ;
#10814=CARTESIAN_POINT ( 'NONE',  ( -4.763139720814407951, -2.750000000000016431, -47.49999999999998579 ) ) ;
#10817=CARTESIAN_POINT ( 'NONE',  ( -5.412658773652739619, 3.124999999999975131, -75.18301270189226670 ) ) ;
#10821=CARTESIAN_POINT ( 'NONE',  ( -5.196152422706573404, -3.000000000000002665, -178.2886751345948539 ) ) ;
#10824=CARTESIAN_POINT ( 'NONE',  ( 6.350852961086080661, -9.614813431917819062E-14, -132.3750000000000284 ) ) ;
#10827=CARTESIAN_POINT ( 'NONE',  ( 3.464101615137852974, 5.999999999999884537, -178.3363248654052313 ) ) ;
#10829=CARTESIAN_POINT ( 'NONE',  ( -4.763139720814407951, 2.749999999999946709, -64.25000000000002842 ) ) ;
#10830=CARTESIAN_POINT ( 'NONE',  ( 3.464101615137852974, 5.999999999999884537, -70.33632486540518869 ) ) ;
#10832=ORIENTED_EDGE ( 'NONE', *, *, #16099, .F. ) ;
#10837=ADVANCED_FACE ( 'NONE', ( #12349 ), #28573, .T. ) ;
#10839=ORIENTED_EDGE ( 'NONE', *, *, #4741, .F. ) ;
#10845=CARTESIAN_POINT ( 'NONE',  ( -3.175426480542816510, -5.500000000000057732, -141.8750000000000568 ) ) ;
#10846=ORIENTED_EDGE ( 'NONE', *, *, #4940, .F. ) ;
#10848=ORIENTED_EDGE ( 'NONE', *, *, #21609, .T. ) ;
#10849=CARTESIAN_POINT ( 'NONE',  ( -6.350852961085760029, -1.281975124255709124E-13, -76.12500000000000000 ) ) ;
#10850=( BOUNDED_CURVE ( )  B_SPLINE_CURVE ( 2, ( #6605, #16179, #28086, #11564, #23216, #11713, #16329, #2457, #23368 ),
 .UNSPECIFIED., .F., .T. ) 
 B_SPLINE_CURVE_WITH_KNOTS ( ( 3, 2, 2, 2, 3 ),
 ( 0.7972222222222222765, 0.7981481481481481621, 0.8000000000000000444, 0.8018518518518518157, 0.8027777777777778123 ),
 .UNSPECIFIED. ) 
 CURVE ( )  GEOMETRIC_REPRESENTATION_ITEM ( )  RATIONAL_B_SPLINE_CURVE ( ( 0.9330127018922194093, 0.9330127018922234061, 1.000000000000000000, 0.8660254037844388186, 1.000000000000000000, 0.8660254037844388186, 1.000000000000000000, 0.9330127018922154125, 0.9330127018922194093 ) ) 
 REPRESENTATION_ITEM ( '' )  );
#10851=CARTESIAN_POINT ( 'NONE',  ( 5.412658773652739619, 3.124999999999988898, -93.68301270189222407 ) ) ;
#10852=CARTESIAN_POINT ( 'NONE',  ( -6.000000000000000888, 1.067854986875958443E-15, 7.560779664488942560E-35 ) ) ;
#10855=CARTESIAN_POINT ( 'NONE',  ( 6.000000000000052403, -1.607695154586662678, -86.23066243270258724 ) ) ;
#10858=( BOUNDED_CURVE ( )  B_SPLINE_CURVE ( 2, ( #1545, #17871, #10638, #19834, #15252, #12962, #20303, #22457, #8464 ),
 .UNSPECIFIED., .F., .F. ) 
 B_SPLINE_CURVE_WITH_KNOTS ( ( 3, 2, 2, 2, 3 ),
 ( 0.1861111111111111160, 0.1870370370370370017, 0.1888888888888888840, 0.1907407407407407662, 0.1916666666666666519 ),
 .UNSPECIFIED. ) 
 CURVE ( )  GEOMETRIC_REPRESENTATION_ITEM ( )  RATIONAL_B_SPLINE_CURVE ( ( 0.9330127018922194093, 0.9330127018922194093, 1.000000000000000000, 0.8660254037844388186, 1.000000000000000000, 0.8660254037844388186, 1.000000000000000000, 0.9330127018922194093, 0.9330127018922194093 ) ) 
 REPRESENTATION_ITEM ( '' )  );
#10859=CARTESIAN_POINT ( 'NONE',  ( 4.763139720814407951, 2.750000000000002665, -159.2500000000000000 ) ) ;
#10862=CARTESIAN_POINT ( 'NONE',  ( 6.350852961086080661, -9.614813431917819062E-14, -85.87500000000004263 ) ) ;
#10863=CARTESIAN_POINT ( 'NONE',  ( -3.464101615137757051, -5.999999999999979572, -140.6636751345948255 ) ) ;
#10865=CARTESIAN_POINT ( 'NONE',  ( 6.350852961086080661, -9.614813431917819062E-14, -82.87500000000004263 ) ) ;
#10866=VECTOR ( 'NONE', #9099, 1000.000000000000000 ) ;
#10867=CARTESIAN_POINT ( 'NONE',  ( -5.999999999999971578, 1.607695154586715303, -105.9033121635130072 ) ) ;
#10872=CARTESIAN_POINT ( 'NONE',  ( -5.999999999999963585, 1.780251999655701777E-13, -74.91367513459485394 ) ) ;
#10873=EDGE_CURVE ( 'NONE', #23894, #12844, #23497, .T. ) ;
#10877=CARTESIAN_POINT ( 'NONE',  ( 0.000000000000000000, -5.999999999999991118, -172.0386751345947971 ) ) ;
#10880=ORIENTED_EDGE ( 'NONE', *, *, #384, .T. ) ;
#10881=AXIS2_PLACEMENT_3D ( 'NONE', #11994, #5012, #14443 ) ;
#10882=ORIENTED_EDGE ( 'NONE', *, *, #26186, .F. ) ;
#10883=CARTESIAN_POINT ( 'NONE',  ( -3.175426480542816510, -5.500000000000057732, -95.37500000000004263 ) ) ;
#10885=CARTESIAN_POINT ( 'NONE',  ( 3.608439182435180470, -6.249999999999997335, -118.0580127018922525 ) ) ;
#10886=VERTEX_POINT ( 'NONE', #17705 ) ;
#10887=CARTESIAN_POINT ( 'NONE',  ( 0.000000000000000000, 5.999999999999977796, -140.7113248654052313 ) ) ;
#10888=LINE ( 'NONE', #2101, #22107 ) ;
#10890=CARTESIAN_POINT ( 'NONE',  ( 3.608439182435180470, -6.249999999999997335, -50.55801270189225249 ) ) ;
#10892=DIRECTION ( 'NONE',  ( -7.147005652999508048E-36, 5.642372883946980038E-36, 1.000000000000000000 ) ) ;
#10895=CARTESIAN_POINT ( 'NONE',  ( -4.763139720814407951, 2.749999999999946709, -163.2500000000000000 ) ) ;
#10899=CARTESIAN_POINT ( 'NONE',  ( -2.775557561562891351E-14, -5.500000000000115463, -110.2500000000000142 ) ) ;
#10901=CARTESIAN_POINT ( 'NONE',  ( -4.763139720814407951, 2.749999999999946709, -106.2500000000000142 ) ) ;
#10910=ORIENTED_EDGE ( 'NONE', *, *, #24703, .F. ) ;
#10911=CARTESIAN_POINT ( 'NONE',  ( -5.999999999999963585, -1.487416814333745711E-14, -127.4136751345948113 ) ) ;
#10913=CARTESIAN_POINT ( 'NONE',  ( 7.216878364870455975, -6.409875621278545621E-14, -91.44198729810784698 ) ) ;
#10917=CYLINDRICAL_SURFACE ( 'NONE', #15011, 6.000000000000000888 ) ;
#10919=ORIENTED_EDGE ( 'NONE', *, *, #12820, .F. ) ;
#10923=CARTESIAN_POINT ( 'NONE',  ( -6.350852961085760029, -1.281975124255709124E-13, -122.6250000000000426 ) ) ;
#10925=CARTESIAN_POINT ( 'NONE',  ( 5.196152422706629359, 3.000000000000002665, -161.0386751345948539 ) ) ;
#10926=CARTESIAN_POINT ( 'NONE',  ( 2.775557561562891351E-14, -6.250000000000061284, -123.3169872981078043 ) ) ;
#10927=CARTESIAN_POINT ( 'NONE',  ( 5.412658773652739619, 3.124999999999988898, -175.3169872981078470 ) ) ;
#10928=CARTESIAN_POINT ( 'NONE',  ( -6.350852961085760029, -1.281975124255709124E-13, -175.1250000000000284 ) ) ;
#10930=CARTESIAN_POINT ( 'NONE',  ( -5.999999999999963585, 1.780251999655701777E-13, -47.33632486540523132 ) ) ;
#10931=VERTEX_POINT ( 'NONE', #29335 ) ;
#10936=CARTESIAN_POINT ( 'NONE',  ( 2.775557561562891351E-14, 6.250000000000033751, -65.56698729810783277 ) ) ;
#10937=CARTESIAN_POINT ( 'NONE',  ( -7.216878364870328078, 0.000000000000000000, -54.69198729810780435 ) ) ;
#10939=CARTESIAN_POINT ( 'NONE',  ( -5.999999999999963585, 1.780251999655701777E-13, -110.3363248654052029 ) ) ;
#10940=CARTESIAN_POINT ( 'NONE',  ( 0.000000000000000000, 5.499999999999991118, -51.00000000000004263 ) ) ;
#10942=CARTESIAN_POINT ( 'NONE',  ( 0.000000000000000000, 0.000000000000000000, 0.000000000000000000 ) ) ;
#10943=CARTESIAN_POINT ( 'NONE',  ( 0.000000000000000000, 5.499999999999991118, -132.0000000000000000 ) ) ;
#10944=EDGE_LOOP ( 'NONE', ( #10290, #24501, #9317, #17702 ) ) ;
#10946=DIRECTION ( 'NONE',  ( 1.000000000000000000, -5.551115123125773458E-17, -1.260129944081490338E-35 ) ) ;
#10948=CARTESIAN_POINT ( 'NONE',  ( 6.000000000000000888, -1.859271017917181981E-14, -147.6636751345948255 ) ) ;
#10949=( BOUNDED_CURVE ( )  B_SPLINE_CURVE ( 2, ( #11126, #27514, #6492, #20474, #18197, #1882, #18353, #13599, #22943 ),
 .UNSPECIFIED., .F., .T. ) 
 B_SPLINE_CURVE_WITH_KNOTS ( ( 3, 2, 2, 2, 3 ),
 ( 0.2027777777777777790, 0.2037037037037036924, 0.2055555555555555469, 0.2074074074074074014, 0.2083333333333333426 ),
 .UNSPECIFIED. ) 
 CURVE ( )  GEOMETRIC_REPRESENTATION_ITEM ( )  RATIONAL_B_SPLINE_CURVE ( ( 0.9330127018922194093, 0.9330127018922194093, 1.000000000000000000, 0.8660254037844388186, 1.000000000000000000, 0.8660254037844388186, 1.000000000000000000, 0.9330127018922184101, 0.9330127018922194093 ) ) 
 REPRESENTATION_ITEM ( '' )  );
#10950=EDGE_CURVE ( 'NONE', #28820, #7308, #12800, .T. ) ;
#10954=DIRECTION ( 'NONE',  ( -7.147005652999508048E-36, 5.642372883946980038E-36, 1.000000000000000000 ) ) ;
#10955=CARTESIAN_POINT ( 'NONE',  ( 5.412658773652712085, -3.125000000000086153, -117.0669872981078328 ) ) ;
#10956=CARTESIAN_POINT ( 'NONE',  ( 0.000000000000000000, -5.999999999999991118, -109.9613248654052171 ) ) ;
#10963=ORIENTED_EDGE ( 'NONE', *, *, #2004, .F. ) ;
#10965=CARTESIAN_POINT ( 'NONE',  ( 6.000000000000000888, 1.743066579297358182E-13, -107.1636751345948539 ) ) ;
#10969=CARTESIAN_POINT ( 'NONE',  ( -5.412658773652739619, 3.124999999999975131, -64.68301270189225249 ) ) ;
#10978=MECHANICAL_DESIGN_GEOMETRIC_PRESENTATION_REPRESENTATION('',(#637),#26601);
#10979=CARTESIAN_POINT ( 'NONE',  ( -3.175426480542816066, 5.499999999999865885, -130.3750000000000284 ) ) ;
#10980=CARTESIAN_POINT ( 'NONE',  ( 3.608439182435180470, -6.249999999999997335, -148.0580127018922383 ) ) ;
#10983=CARTESIAN_POINT ( 'NONE',  ( -4.763139720814407951, 2.749999999999946709, -61.25000000000002842 ) ) ;
#10984=EDGE_CURVE ( 'NONE', #11104, #3131, #2487, .T. ) ;
#10985=ORIENTED_EDGE ( 'NONE', *, *, #2547, .T. ) ;
#10992=AXIS2_PLACEMENT_3D ( 'NONE', #13985, #2115, #7017 ) ;
#10995=CARTESIAN_POINT ( 'NONE',  ( 6.350852961086080661, -9.614813431917819062E-14, -148.8750000000000284 ) ) ;
#10999=CARTESIAN_POINT ( 'NONE',  ( -2.775557561562891351E-14, -5.500000000000115463, -77.25000000000004263 ) ) ;
#11001=ORIENTED_EDGE ( 'NONE', *, *, #12894, .T. ) ;
#11003=ADVANCED_FACE ( 'NONE', ( #20146 ), #8459, .T. ) ;
#11004=CARTESIAN_POINT ( 'NONE',  ( -5.196152422706601826, 2.999999999999975131, -150.0386751345948539 ) ) ;
#11008=SHAPE_DEFINITION_REPRESENTATION ( #15587, #13689 ) ;
#11009=CARTESIAN_POINT ( 'NONE',  ( -3.175426480542816066, 5.499999999999865885, -158.8750000000000000 ) ) ;
#11011=CARTESIAN_POINT ( 'NONE',  ( -3.175426480542816066, 5.499999999999865885, -88.37500000000001421 ) ) ;
#11012=CARTESIAN_POINT ( 'NONE',  ( 3.464101615137757051, -5.999999999999979572, -140.4136751345948255 ) ) ;
#11014=CARTESIAN_POINT ( 'NONE',  ( 6.350852961086080661, -9.614813431917819062E-14, -70.87500000000004263 ) ) ;
#11015=EDGE_CURVE ( 'NONE', #10886, #18250, #20911, .T. ) ;
#11016=CARTESIAN_POINT ( 'NONE',  ( -5.196152422706601826, 2.999999999999975131, -105.9613248654052171 ) ) ;
#11017=CARTESIAN_POINT ( 'NONE',  ( -6.000000000000007105, -1.607695154586655129, -108.7693375672974412 ) ) ;
#11019=CARTESIAN_POINT ( 'NONE',  ( -5.999999999999971578, 1.607695154586715303, -54.90331216351302146 ) ) ;
#11020=DIRECTION ( 'NONE',  ( 1.000000000000000000, -5.551115123125773458E-17, -1.260129944081490338E-35 ) ) ;
#11021=CYLINDRICAL_SURFACE ( 'NONE', #22845, 6.000000000000000888 ) ;
#11022=VERTEX_POINT ( 'NONE', #23372 ) ;
#11028=CARTESIAN_POINT ( 'NONE',  ( 0.000000000000000000, 5.499999999999991118, -100.5000000000000284 ) ) ;
#11029=DIRECTION ( 'NONE',  ( -7.147005652999508048E-36, 5.642372883946980038E-36, 1.000000000000000000 ) ) ;
#11030=CARTESIAN_POINT ( 'NONE',  ( 2.775557561562891351E-14, 6.250000000000033751, -115.9330127018922667 ) ) ;
#11031=CARTESIAN_POINT ( 'NONE',  ( -5.999999999999963585, 1.780251999655701777E-13, -110.3363248654052029 ) ) ;
#11033=CARTESIAN_POINT ( 'NONE',  ( -5.999999999999963585, 1.780251999655701777E-13, -107.9136751345948397 ) ) ;
#11034=ADVANCED_FACE ( 'NONE', ( #30107 ), #25653, .T. ) ;
#11035=CARTESIAN_POINT ( 'NONE',  ( -5.412658773652739619, 3.124999999999975131, -55.68301270189224539 ) ) ;
#11036=ORIENTED_EDGE ( 'NONE', *, *, #19209, .F. ) ;
#11037=CARTESIAN_POINT ( 'NONE',  ( -5.999999999999971578, 1.607695154586715303, -159.9033121635130499 ) ) ;
#11038=DIRECTION ( 'NONE',  ( 0.000000000000000000, 0.000000000000000000, 1.000000000000000000 ) ) ;
#11039=CARTESIAN_POINT ( 'NONE',  ( -5.196152422706573404, -3.000000000000002665, -167.2113248654052313 ) ) ;
#11040=CARTESIAN_POINT ( 'NONE',  ( 0.000000000000000000, 5.499999999999991118, -165.0000000000000284 ) ) ;
#11043=CARTESIAN_POINT ( 'NONE',  ( 6.350852961086080661, -9.614813431917819062E-14, -108.3750000000000426 ) ) ;
#11046=EDGE_CURVE ( 'NONE', #6403, #22416, #20299, .T. ) ;
#11047=CARTESIAN_POINT ( 'NONE',  ( 4.763139720814407951, -2.749999999999988454, -98.00000000000002842 ) ) ;
#11050=VERTEX_POINT ( 'NONE', #29645 ) ;
#11053=ORIENTED_EDGE ( 'NONE', *, *, #15719, .F. ) ;
#11054=CARTESIAN_POINT ( 'NONE',  ( 5.999999999999949374, 1.607695154586804565, -112.5193375672973986 ) ) ;
#11056=CARTESIAN_POINT ( 'NONE',  ( 5.412658773652739619, 3.124999999999988898, -89.81698729810783277 ) ) ;
#11057=CARTESIAN_POINT ( 'NONE',  ( -5.196152422706573404, -3.000000000000002665, -129.7113248654052029 ) ) ;
#11058=ORIENTED_EDGE ( 'NONE', *, *, #23492, .T. ) ;
#11059=CARTESIAN_POINT ( 'NONE',  ( -4.384309399116673944, 10.08956758734764136, -29.10056064752988547 ) ) ;
#11060=CARTESIAN_POINT ( 'NONE',  ( 4.763139720814407951, 2.750000000000002665, -151.7500000000000568 ) ) ;
#11061=ORIENTED_EDGE ( 'NONE', *, *, #12403, .T. ) ;
#11065=CARTESIAN_POINT ( 'NONE',  ( 0.000000000000000000, 5.499999999999991118, -120.0000000000000000 ) ) ;
#11066=CARTESIAN_POINT ( 'NONE',  ( 7.216878364870455975, -6.409875621278545621E-14, -137.3080127018922667 ) ) ;
#11067=ORIENTED_EDGE ( 'NONE', *, *, #15317, .F. ) ;
#11068=CARTESIAN_POINT ( 'NONE',  ( 3.464101615137757051, -5.999999999999979572, -57.33632486540520290 ) ) ;
#11069=CARTESIAN_POINT ( 'NONE',  ( 7.216878364870455975, -6.409875621278545621E-14, -119.9419872981078470 ) ) ;
#11070=CARTESIAN_POINT ( 'NONE',  ( -4.763139720814407951, 2.749999999999946709, -170.7500000000000000 ) ) ;
#11073=DIRECTION ( 'NONE',  ( 1.000000000000000000, -5.551115123125773458E-17, -1.260129944081490338E-35 ) ) ;
#11074=( BOUNDED_CURVE ( )  B_SPLINE_CURVE ( 2, ( #16087, #27996, #7117, #25863, #9589, #25391, #14238, #11471, #203 ),
 .UNSPECIFIED., .F., .F. ) 
 B_SPLINE_CURVE_WITH_KNOTS ( ( 3, 2, 2, 2, 3 ),
 ( 0.5027777777777777679, 0.5037037037037036535, 0.5055555555555555358, 0.5074074074074074181, 0.5083333333333334147 ),
 .UNSPECIFIED. ) 
 CURVE ( )  GEOMETRIC_REPRESENTATION_ITEM ( )  RATIONAL_B_SPLINE_CURVE ( ( 0.9330127018922194093, 0.9330127018922194093, 1.000000000000000000, 0.8660254037844388186, 1.000000000000000000, 0.8660254037844388186, 1.000000000000000000, 0.9330127018922154125, 0.9330127018922194093 ) ) 
 REPRESENTATION_ITEM ( '' )  );
#11075=ADVANCED_FACE ( 'NONE', ( #3986 ), #13409, .T. ) ;
#11079=EDGE_CURVE ( 'NONE', #9960, #10034, #22157, .T. ) ;
#11083=CARTESIAN_POINT ( 'NONE',  ( 2.775557561562891351E-14, -6.250000000000061284, -76.81698729810781856 ) ) ;
#11084=CARTESIAN_POINT ( 'NONE',  ( 2.775557561562891351E-14, -6.250000000000061284, -61.81698729810780435 ) ) ;
#11086=CARTESIAN_POINT ( 'NONE',  ( -6.350852961085760029, -1.281975124255709124E-13, -52.12500000000002132 ) ) ;
#11089=CARTESIAN_POINT ( 'NONE',  ( 3.175426480543072749, -5.500000000000105693, -125.1250000000000426 ) ) ;
#11092=CARTESIAN_POINT ( 'NONE',  ( 0.000000000000000000, 5.999999999999977796, -132.2886751345947971 ) ) ;
#11094=CARTESIAN_POINT ( 'NONE',  ( 0.000000000000000000, 0.000000000000000000, 0.000000000000000000 ) ) ;
#11096=ORIENTED_EDGE ( 'NONE', *, *, #2050, .T. ) ;
#11100=CARTESIAN_POINT ( 'NONE',  ( 2.775557561562891351E-14, -6.250000000000061284, -114.3169872981077901 ) ) ;
#11101=CARTESIAN_POINT ( 'NONE',  ( -5.196152422706573404, -3.000000000000002665, -173.7886751345948255 ) ) ;
#11104=VERTEX_POINT ( 'NONE', #27476 ) ;
#11106=ORIENTED_EDGE ( 'NONE', *, *, #6128, .T. ) ;
#11109=AXIS2_PLACEMENT_3D ( 'NONE', #20978, #18682, #211 ) ;
#11110=CARTESIAN_POINT ( 'NONE',  ( 6.000000000000000888, -3.330669073875464691E-16, -7.560779664488942560E-35 ) ) ;
#11113=CARTESIAN_POINT ( 'NONE',  ( -5.412658773652739619, 3.124999999999975131, -69.18301270189225249 ) ) ;
#11116=DIRECTION ( 'NONE',  ( -7.147005652999508048E-36, 5.642372883946980038E-36, 1.000000000000000000 ) ) ;
#11117=CARTESIAN_POINT ( 'NONE',  ( -3.464101615137725076, 5.999999999999979572, -165.1636751345948255 ) ) ;
#11120=( BOUNDED_CURVE ( )  B_SPLINE_CURVE ( 2, ( #23578, #11944, #209, #9900, #18985, #9595, #19124, #28455, #16835 ),
 .UNSPECIFIED., .F., .T. ) 
 B_SPLINE_CURVE_WITH_KNOTS ( ( 3, 2, 2, 2, 3 ),
 ( 0.4361111111111111160, 0.4370370370370370017, 0.4388888888888888840, 0.4407407407407407662, 0.4416666666666666519 ),
 .UNSPECIFIED. ) 
 CURVE ( )  GEOMETRIC_REPRESENTATION_ITEM ( )  RATIONAL_B_SPLINE_CURVE ( ( 0.9330127018922194093, 0.9330127018922194093, 1.000000000000000000, 0.8660254037844388186, 1.000000000000000000, 0.8660254037844388186, 1.000000000000000000, 0.9330127018922194093, 0.9330127018922194093 ) ) 
 REPRESENTATION_ITEM ( '' )  );
#11121=CARTESIAN_POINT ( 'NONE',  ( -3.175426480542816066, 5.499999999999865885, -125.8749999999999858 ) ) ;
#11123=CARTESIAN_POINT ( 'NONE',  ( 6.000000000000000888, -1.859271017917181981E-14, -159.0863248654052313 ) ) ;
#11124=EDGE_LOOP ( 'NONE', ( #20346, #24518, #5734, #17736 ) ) ;
#11125=CARTESIAN_POINT ( 'NONE',  ( 4.763139720814407951, 2.750000000000002665, -63.25000000000002842 ) ) ;
#11126=CARTESIAN_POINT ( 'NONE',  ( -5.999999999999963585, -1.487416814333745711E-14, -154.4136751345947971 ) ) ;
#11127=CARTESIAN_POINT ( 'NONE',  ( 5.196152422706629359, 3.000000000000002665, -70.46132486540524553 ) ) ;
#11131=CYLINDRICAL_SURFACE ( 'NONE', #596, 6.000000000000000888 ) ;
#11139=CARTESIAN_POINT ( 'NONE',  ( -3.175426480542816510, -5.500000000000057732, -143.3750000000000000 ) ) ;
#11144=CARTESIAN_POINT ( 'NONE',  ( 3.175426480543072749, 5.499999999999865885, -72.12500000000005684 ) ) ;
#11146=CARTESIAN_POINT ( 'NONE',  ( 7.216878364870455975, -6.409875621278545621E-14, -87.80801270189223828 ) ) ;
#11148=CARTESIAN_POINT ( 'NONE',  ( -4.520081486476279053, -10.03271082534599401, -28.96438617129773618 ) ) ;
#11149=CARTESIAN_POINT ( 'NONE',  ( 5.999999999999949374, 1.607695154586804565, -107.0966878364870638 ) ) ;
#11150=DIRECTION ( 'NONE',  ( 1.000000000000000000, -5.551115123125774690E-17, 0.000000000000000000 ) ) ;
#11153=CARTESIAN_POINT ( 'NONE',  ( -3.175426480542816066, -5.500000000000057732, -159.8750000000000284 ) ) ;
#11158=CARTESIAN_POINT ( 'NONE',  ( -4.763139720814407951, -2.750000000000016431, -86.50000000000002842 ) ) ;
#11159=VECTOR ( 'NONE', #29374, 1000.000000000000000 ) ;
#11160=VECTOR ( 'NONE', #12022, 1000.000000000000000 ) ;
#11162=CARTESIAN_POINT ( 'NONE',  ( -6.350852961085760029, -1.281975124255709124E-13, -73.12500000000005684 ) ) ;
#11164=CARTESIAN_POINT ( 'NONE',  ( 6.000000000000000888, 7.762456499804234384E-14, -142.5863248654051745 ) ) ;
#11172=CARTESIAN_POINT ( 'NONE',  ( 0.000000000000000000, 5.999999999999977796, -134.7113248654052597 ) ) ;
#11173=CARTESIAN_POINT ( 'NONE',  ( 3.464101615137852974, 5.999999999999884537, -169.9136751345948255 ) ) ;
#11179=CARTESIAN_POINT ( 'NONE',  ( 0.000000000000000000, 5.999999999999977796, -157.2113248654052313 ) ) ;
#11183=CARTESIAN_POINT ( 'NONE',  ( -3.175426480542816510, 5.499999999999865885, -95.87500000000002842 ) ) ;
#11184=VECTOR ( 'NONE', #28882, 1000.000000000000000 ) ;
#11185=CARTESIAN_POINT ( 'NONE',  ( 5.196152422706629359, 3.000000000000002665, -71.03867513459482552 ) ) ;
#11186=ADVANCED_FACE ( 'NONE', ( #7370 ), #26101, .T. ) ;
#11187=CARTESIAN_POINT ( 'NONE',  ( 2.775557561562891351E-14, -6.250000000000061284, -109.1830127018922383 ) ) ;
#11190=CARTESIAN_POINT ( 'NONE',  ( 0.000000000000000000, -5.999999999999991118, -143.5386751345948255 ) ) ;
#11191=CARTESIAN_POINT ( 'NONE',  ( -3.175426480542816510, 5.499999999999865885, -166.3750000000000568 ) ) ;
#11192=CARTESIAN_POINT ( 'NONE',  ( 3.608439182435180470, 6.249999999999982236, -47.05801270189223118 ) ) ;
#11193=DIRECTION ( 'NONE',  ( 1.000000000000000000, -5.551115123125773458E-17, -1.260129944081490338E-35 ) ) ;
#11195=CARTESIAN_POINT ( 'NONE',  ( 6.000000000000052403, -1.607695154586662678, -56.23066243270260856 ) ) ;
#11196=CARTESIAN_POINT ( 'NONE',  ( 6.000000000000000888, -3.330669073875464691E-16, -7.560779664488942560E-35 ) ) ;
#11197=CARTESIAN_POINT ( 'NONE',  ( 0.000000000000000000, 5.499999999999991118, -160.5000000000000284 ) ) ;
#11200=CARTESIAN_POINT ( 'NONE',  ( 3.175426480543072749, -5.500000000000105693, -111.6249999999999858 ) ) ;
#11203=CARTESIAN_POINT ( 'NONE',  ( -2.775557561562891351E-14, -5.500000000000115463, -99.75000000000000000 ) ) ;
#11207=ORIENTED_EDGE ( 'NONE', *, *, #18747, .F. ) ;
#11214=CARTESIAN_POINT ( 'NONE',  ( -3.608439182435052128, -6.250000000000110134, -88.94198729810783277 ) ) ;
#11215=EDGE_CURVE ( 'NONE', #23369, #29507, #8778, .T. ) ;
#11216=DIRECTION ( 'NONE',  ( -7.147005652999508048E-36, 5.642372883946980038E-36, 1.000000000000000000 ) ) ;
#11220=ORIENTED_EDGE ( 'NONE', *, *, #29407, .T. ) ;
#11222=CARTESIAN_POINT ( 'NONE',  ( 3.175426480543072749, -5.500000000000105693, -125.1250000000000426 ) ) ;
#11224=CARTESIAN_POINT ( 'NONE',  ( 7.216878364870455975, -6.409875621278545621E-14, -128.3080127018922383 ) ) ;
#11226=LINE ( 'NONE', #15696, #23447 ) ;
#11227=CARTESIAN_POINT ( 'NONE',  ( -5.412658773652684552, -3.125000000000099920, -123.5669872981078328 ) ) ;
#11228=CARTESIAN_POINT ( 'NONE',  ( -7.216878364870328078, 0.000000000000000000, -177.6919872981078186 ) ) ;
#11234=FACE_OUTER_BOUND ( 'NONE', #6199, .T. ) ;
#11235=CARTESIAN_POINT ( 'NONE',  ( 3.464101615137852974, 5.999999999999884537, -90.41367513459483973 ) ) ;
#11239=CARTESIAN_POINT ( 'NONE',  ( 2.775557561562891351E-14, 6.250000000000033751, -76.06698729810779014 ) ) ;
#11240=CARTESIAN_POINT ( 'NONE',  ( -3.608439182435115633, 6.249999999999965361, -62.44198729810783988 ) ) ;
#11241=CARTESIAN_POINT ( 'NONE',  ( 4.763139720814407951, 2.750000000000002665, -46.75000000000001421 ) ) ;
#11242=CARTESIAN_POINT ( 'NONE',  ( 5.196152422706629359, -2.999999999999988898, -111.2113248654051887 ) ) ;
#11244=CARTESIAN_POINT ( 'NONE',  ( 4.763139720814407951, -2.749999999999988454, -120.5000000000000568 ) ) ;
#11245=CARTESIAN_POINT ( 'NONE',  ( -6.000000000000000888, 1.067854986875958443E-15, 7.560779664488942560E-35 ) ) ;
#11250=CARTESIAN_POINT ( 'NONE',  ( 6.000000000000000888, -3.330669073875464691E-16, -7.560779664488942560E-35 ) ) ;
#11252=ORIENTED_EDGE ( 'NONE', *, *, #16785, .T. ) ;
#11254=CARTESIAN_POINT ( 'NONE',  ( 6.000000000000000888, -1.607695154586752384, -114.7306624327026157 ) ) ;
#11256=CARTESIAN_POINT ( 'NONE',  ( 3.608439182435180470, -6.249999999999997335, -117.1919872981078470 ) ) ;
#11257=EDGE_CURVE ( 'NONE', #12739, #15355, #18835, .T. ) ;
#11259=ADVANCED_FACE ( 'NONE', ( #300 ), #30411, .T. ) ;
#11265=VERTEX_POINT ( 'NONE', #16479 ) ;
#11266=CARTESIAN_POINT ( 'NONE',  ( 7.216878364870455975, -6.409875621278545621E-14, -149.9419872981078186 ) ) ;
#11271=CARTESIAN_POINT ( 'NONE',  ( 2.775557561562891351E-14, -6.250000000000061284, -64.18301270189225249 ) ) ;
#11275=DIRECTION ( 'NONE',  ( -7.147005652999508048E-36, 5.642372883946980038E-36, 1.000000000000000000 ) ) ;
#11276=CARTESIAN_POINT ( 'NONE',  ( 5.196152422706629359, -2.999999999999988898, -155.2886751345948824 ) ) ;
#11278=CARTESIAN_POINT ( 'NONE',  ( 5.999999999999949374, 1.607695154586804565, -115.5193375672974412 ) ) ;
#11282=CARTESIAN_POINT ( 'NONE',  ( -4.763139720814407951, 2.749999999999946709, -125.7500000000000284 ) ) ;
#11283=CARTESIAN_POINT ( 'NONE',  ( 6.000000000000000888, 1.743066579297358182E-13, -92.16367513459482552 ) ) ;
#11284=CARTESIAN_POINT ( 'NONE',  ( -3.608439182435052128, -6.250000000000110134, -145.3080127018922383 ) ) ;
#11285=CARTESIAN_POINT ( 'NONE',  ( -6.000000000000000888, 1.067854986875958443E-15, 7.560779664488942560E-35 ) ) ;
#11286=ORIENTED_EDGE ( 'NONE', *, *, #2588, .T. ) ;
#11287=CARTESIAN_POINT ( 'NONE',  ( -4.763139720814407951, -2.750000000000016431, -56.49999999999999289 ) ) ;
#11288=FACE_OUTER_BOUND ( 'NONE', #7095, .T. ) ;
#11290=ORIENTED_EDGE ( 'NONE', *, *, #8658, .T. ) ;
#11300=CARTESIAN_POINT ( 'NONE',  ( 0.000000000000000000, 5.499999999999991118, -136.5000000000000000 ) ) ;
#11302=ORIENTED_EDGE ( 'NONE', *, *, #14781, .F. ) ;
#11304=ORIENTED_EDGE ( 'NONE', *, *, #12034, .F. ) ;
#11305=CARTESIAN_POINT ( 'NONE',  ( -4.763139720814407951, 2.749999999999946709, -65.75000000000002842 ) ) ;
#11307=LINE ( 'NONE', #4042, #19969 ) ;
#11308=CARTESIAN_POINT ( 'NONE',  ( -3.608439182435115633, 6.249999999999965361, -90.30801270189225249 ) ) ;
#11309=( BOUNDED_CURVE ( )  B_SPLINE_CURVE ( 2, ( #27116, #8390, #11185, #20534, #17798, #24826, #3773, #22538, #3917 ),
 .UNSPECIFIED., .F., .T. ) 
 B_SPLINE_CURVE_WITH_KNOTS ( ( 3, 2, 2, 2, 3 ),
 ( 0.8194444444444445308, 0.8203703703703704164, 0.8222222222222221877, 0.8240740740740740700, 0.8249999999999999556 ),
 .UNSPECIFIED. ) 
 CURVE ( )  GEOMETRIC_REPRESENTATION_ITEM ( )  RATIONAL_B_SPLINE_CURVE ( ( 0.9330127018922194093, 0.9330127018922234061, 1.000000000000000000, 0.8660254037844388186, 1.000000000000000000, 0.8660254037844388186, 1.000000000000000000, 0.9330127018922234061, 0.9330127018922194093 ) ) 
 REPRESENTATION_ITEM ( '' )  );
#11311=DIRECTION ( 'NONE',  ( -7.147005652999508048E-36, 5.642372883946980038E-36, 1.000000000000000000 ) ) ;
#11313=DIRECTION ( 'NONE',  ( -7.147005652999508048E-36, 5.642372883946980038E-36, 1.000000000000000000 ) ) ;
#11316=CARTESIAN_POINT ( 'NONE',  ( 4.763139720814407951, 2.750000000000002665, -151.7500000000000568 ) ) ;
#11318=CARTESIAN_POINT ( 'NONE',  ( -3.175426480542816510, -5.500000000000057732, -141.8750000000000568 ) ) ;
#11319=CARTESIAN_POINT ( 'NONE',  ( 5.412658773652712085, -3.125000000000086153, -161.4330127018922667 ) ) ;
#11321=CARTESIAN_POINT ( 'NONE',  ( 0.000000000000000000, 0.000000000000000000, 0.000000000000000000 ) ) ;
#11322=ADVANCED_FACE ( 'NONE', ( #3442 ), #1147, .T. ) ;
#11323=CARTESIAN_POINT ( 'NONE',  ( 4.763139720814407951, 2.750000000000002665, -76.74999999999998579 ) ) ;
#11324=LINE ( 'NONE', #17930, #27700 ) ;
#11325=CARTESIAN_POINT ( 'NONE',  ( 3.175426480543072749, -5.500000000000105693, -72.62500000000005684 ) ) ;
#11327=CARTESIAN_POINT ( 'NONE',  ( -5.999999999999963585, 1.780251999655701777E-13, -64.41367513459483973 ) ) ;
#11328=CARTESIAN_POINT ( 'NONE',  ( -5.196152422706573404, -3.000000000000002665, -71.78867513459485394 ) ) ;
#11332=CARTESIAN_POINT ( 'NONE',  ( -5.999999999999971578, 1.607695154586715303, -118.4806624327026299 ) ) ;
#11334=CARTESIAN_POINT ( 'NONE',  ( 3.464101615137852974, 5.999999999999884537, -139.3363248654051745 ) ) ;
#11338=CARTESIAN_POINT ( 'NONE',  ( 6.000000000000014211, -1.607695154586730180, -156.7306624327026157 ) ) ;
#11340=CARTESIAN_POINT ( 'NONE',  ( 5.196152422706629359, 3.000000000000002665, -179.9613248654052313 ) ) ;
#11341=ORIENTED_EDGE ( 'NONE', *, *, #21025, .T. ) ;
#11343=EDGE_LOOP ( 'NONE', ( #22230, #2880, #3376, #29173 ) ) ;
#11344=CARTESIAN_POINT ( 'NONE',  ( -2.775557561562891351E-14, -5.500000000000115463, -95.25000000000000000 ) ) ;
#11345=CARTESIAN_POINT ( 'NONE',  ( 2.775557561562891351E-14, 6.250000000000033751, -103.9330127018922525 ) ) ;
#11346=ORIENTED_EDGE ( 'NONE', *, *, #14818, .T. ) ;
#11347=VECTOR ( 'NONE', #25662, 1000.000000000000000 ) ;
#11350=CARTESIAN_POINT ( 'NONE',  ( 3.175426480543072749, -5.500000000000105693, -162.6250000000000284 ) ) ;
#11351=CARTESIAN_POINT ( 'NONE',  ( -5.999999999999963585, 1.780251999655701777E-13, -63.83632486540523132 ) ) ;
#11352=VERTEX_POINT ( 'NONE', #10547 ) ;
#11353=CARTESIAN_POINT ( 'NONE',  ( 0.000000000000000000, 0.000000000000000000, 0.000000000000000000 ) ) ;
#11355=CARTESIAN_POINT ( 'NONE',  ( -3.175426480542816066, 5.499999999999865885, -170.8750000000000853 ) ) ;
#11357=CARTESIAN_POINT ( 'NONE',  ( -2.775557561562891351E-14, -5.500000000000115463, -165.7500000000000000 ) ) ;
#11361=CARTESIAN_POINT ( 'NONE',  ( -4.763139720814407951, -2.750000000000016431, -111.9999999999999858 ) ) ;
#11362=CARTESIAN_POINT ( 'NONE',  ( -5.999999999999962697, 3.323446944526963260E-14, -159.8363248654052597 ) ) ;
#11364=CARTESIAN_POINT ( 'NONE',  ( 4.763139720814407951, -2.749999999999988454, -95.00000000000002842 ) ) ;
#11369=LINE ( 'NONE', #15414, #24192 ) ;
#11373=CARTESIAN_POINT ( 'NONE',  ( 6.000000000000052403, -1.607695154586662678, -85.65331216351297883 ) ) ;
#11379=CARTESIAN_POINT ( 'NONE',  ( -5.412658773652684552, -3.125000000000099920, -90.56698729810786119 ) ) ;
#11380=ORIENTED_EDGE ( 'NONE', *, *, #26482, .T. ) ;
#11383=ORIENTED_EDGE ( 'NONE', *, *, #14195, .T. ) ;
#11384=CARTESIAN_POINT ( 'NONE',  ( -3.175426480542816510, -5.500000000000057732, -125.3749999999999858 ) ) ;
#11386=CARTESIAN_POINT ( 'NONE',  ( 3.608439182435180470, 6.249999999999982236, -128.0580127018922383 ) ) ;
#11387=ORIENTED_EDGE ( 'NONE', *, *, #7474, .F. ) ;
#11388=CARTESIAN_POINT ( 'NONE',  ( 0.000000000000000000, 5.999999999999977796, -160.7886751345948255 ) ) ;
#11389=CARTESIAN_POINT ( 'NONE',  ( -3.608439182435115633, 6.249999999999965361, -168.9419872981078186 ) ) ;
#11390=CARTESIAN_POINT ( 'NONE',  ( 3.608439182435180470, 6.249999999999982236, -173.6919872981077901 ) ) ;
#11392=AXIS2_PLACEMENT_3D ( 'NONE', #4781, #6635, #27959 ) ;
#11395=DIRECTION ( 'NONE',  ( -7.147005652999508048E-36, 5.642372883946980038E-36, 1.000000000000000000 ) ) ;
#11396=DIRECTION ( 'NONE',  ( 1.779758311459930738E-16, 1.000000000000000000, -5.642372883946978702E-36 ) ) ;
#11398=CARTESIAN_POINT ( 'NONE',  ( -7.216878364870328078, 0.000000000000000000, -75.69198729810783277 ) ) ;
#11400=CARTESIAN_POINT ( 'NONE',  ( -3.608439182435115633, 6.249999999999965361, -57.94198729810781145 ) ) ;
#11401=CARTESIAN_POINT ( 'NONE',  ( -3.175426480542816510, 5.499999999999865885, -50.87500000000001421 ) ) ;
#11404=CARTESIAN_POINT ( 'NONE',  ( -5.999999999999904965, -1.607695154586834541, -123.7693375672974554 ) ) ;
#11406=( BOUNDED_CURVE ( )  B_SPLINE_CURVE ( 2, ( #24721, #27015, #17689, #1372, #13250, #29158, #8758, #27456, #15553 ),
 .UNSPECIFIED., .F., .T. ) 
 B_SPLINE_CURVE_WITH_KNOTS ( ( 3, 2, 2, 2, 3 ),
 ( 0.7527777777777777679, 0.7537037037037037646, 0.7555555555555555358, 0.7574074074074074181, 0.7583333333333333037 ),
 .UNSPECIFIED. ) 
 CURVE ( )  GEOMETRIC_REPRESENTATION_ITEM ( )  RATIONAL_B_SPLINE_CURVE ( ( 0.9330127018922194093, 0.9330127018922154125, 1.000000000000000000, 0.8660254037844388186, 1.000000000000000000, 0.8660254037844388186, 1.000000000000000000, 0.9330127018922234061, 0.9330127018922194093 ) ) 
 REPRESENTATION_ITEM ( '' )  );
#11407=CARTESIAN_POINT ( 'NONE',  ( -6.350852961085760029, -1.281975124255709124E-13, -118.1250000000000142 ) ) ;
#11408=CARTESIAN_POINT ( 'NONE',  ( 6.350852961086080661, -9.614813431917819062E-14, -154.8750000000000000 ) ) ;
#11410=ORIENTED_EDGE ( 'NONE', *, *, #22789, .F. ) ;
#11414=EDGE_CURVE ( 'NONE', #10456, #18174, #3088, .T. ) ;
#11416=EDGE_LOOP ( 'NONE', ( #19181, #7503, #30039, #13377 ) ) ;
#11421=CARTESIAN_POINT ( 'NONE',  ( 3.608439182435180470, 6.249999999999982236, -107.6919872981077901 ) ) ;
#11422=CARTESIAN_POINT ( 'NONE',  ( -5.999999999999919176, 1.607695154586804565, -107.9806624327026299 ) ) ;
#11424=ORIENTED_EDGE ( 'NONE', *, *, #23392, .F. ) ;
#11425=ORIENTED_EDGE ( 'NONE', *, *, #25577, .T. ) ;
#11428=CARTESIAN_POINT ( 'NONE',  ( 3.608439182435180470, -6.249999999999997335, -49.69198729810783988 ) ) ;
#11430=CARTESIAN_POINT ( 'NONE',  ( 7.216878364870455975, -6.409875621278545621E-14, -137.9419872981078186 ) ) ;
#11432=CARTESIAN_POINT ( 'NONE',  ( -5.999999999999971578, 1.607695154586715303, -150.9033121635130499 ) ) ;
#11434=CARTESIAN_POINT ( 'NONE',  ( 6.000000000000000888, 1.607695154586715303, -120.5966878364870212 ) ) ;
#11435=CARTESIAN_POINT ( 'NONE',  ( -5.412658773652684552, -3.125000000000099920, -64.43301270189222407 ) ) ;
#11439=CARTESIAN_POINT ( 'NONE',  ( 3.464101615137757051, -5.999999999999979572, -160.8363248654052313 ) ) ;
#11442=CARTESIAN_POINT ( 'NONE',  ( 6.000000000000000888, -1.859271017917181981E-14, -115.5863248654052171 ) ) ;
#11444=EDGE_CURVE ( 'NONE', #3959, #18433, #19793, .T. ) ;
#11445=CARTESIAN_POINT ( 'NONE',  ( 2.000000000000003109, -1.110223024625156540E-16, -2.520259888162984417E-35 ) ) ;
#11447=CARTESIAN_POINT ( 'NONE',  ( 4.763139720814407951, 2.750000000000002665, -120.2500000000000284 ) ) ;
#11448=CARTESIAN_POINT ( 'NONE',  ( 3.464101615137757051, -5.999999999999979572, -92.41367513459485394 ) ) ;
#11449=CARTESIAN_POINT ( 'NONE',  ( -3.608439182435115633, 6.249999999999965361, -142.8080127018922383 ) ) ;
#11452=CARTESIAN_POINT ( 'NONE',  ( -2.775557561562891351E-14, -5.500000000000115463, -56.25000000000002132 ) ) ;
#11453=CARTESIAN_POINT ( 'NONE',  ( 5.999999999999999112, 2.951592740943527306E-14, -154.5863248654052029 ) ) ;
#11460=CARTESIAN_POINT ( 'NONE',  ( 6.000000000000000888, 1.743066579297358182E-13, -91.58632486540523132 ) ) ;
#11464=CARTESIAN_POINT ( 'NONE',  ( 4.763139720814407951, -2.749999999999988454, -141.5000000000000284 ) ) ;
#11465=ORIENTED_EDGE ( 'NONE', *, *, #21231, .T. ) ;
#11468=CARTESIAN_POINT ( 'NONE',  ( -6.350852961085760029, -1.281975124255709124E-13, -65.62500000000002842 ) ) ;
#11469=LINE ( 'NONE', #20814, #23898 ) ;
#11470=CARTESIAN_POINT ( 'NONE',  ( 2.775557561562891351E-14, -6.250000000000061284, -89.68301270189226670 ) ) ;
#11471=CARTESIAN_POINT ( 'NONE',  ( 6.000000000000052403, -1.607695154586662678, -113.2306624327025872 ) ) ;
#11473=CARTESIAN_POINT ( 'NONE',  ( 0.000000000000000000, 0.000000000000000000, -180.0000000000000568 ) ) ;
#11475=FACE_OUTER_BOUND ( 'NONE', #7629, .T. ) ;
#11479=CARTESIAN_POINT ( 'NONE',  ( -4.763139720814407951, -2.750000000000016431, -146.5000000000000284 ) ) ;
#11481=CARTESIAN_POINT ( 'NONE',  ( 5.412658773652712085, -3.125000000000086153, -162.9330127018922667 ) ) ;
#11482=FACE_OUTER_BOUND ( 'NONE', #9126, .T. ) ;
#11483=CARTESIAN_POINT ( 'NONE',  ( -6.350852961085760029, -1.281975124255709124E-13, -76.12500000000002842 ) ) ;
#11484=CYLINDRICAL_SURFACE ( 'NONE', #20359, 6.000000000000000888 ) ;
#11485=CARTESIAN_POINT ( 'NONE',  ( 4.763139720814407951, 2.750000000000002665, -76.74999999999998579 ) ) ;
#11486=CARTESIAN_POINT ( 'NONE',  ( 5.999999999999999112, 2.951592740943527306E-14, -156.0863248654052597 ) ) ;
#11492=CARTESIAN_POINT ( 'NONE',  ( 3.464101615137852974, 5.999999999999884537, -94.91367513459479710 ) ) ;
#11493=DIRECTION ( 'NONE',  ( -7.147005652999508048E-36, 5.642372883946980038E-36, 1.000000000000000000 ) ) ;
#11494=( BOUNDED_CURVE ( )  B_SPLINE_CURVE ( 2, ( #20946, #2636, #30296, #9260, #18654, #16517, #2353, #11754, #9417 ),
 .UNSPECIFIED., .F., .T. ) 
 B_SPLINE_CURVE_WITH_KNOTS ( ( 3, 2, 2, 2, 3 ),
 ( 0.5527777777777778123, 0.5537037037037036979, 0.5555555555555555802, 0.5574074074074073515, 0.5583333333333333481 ),
 .UNSPECIFIED. ) 
 CURVE ( )  GEOMETRIC_REPRESENTATION_ITEM ( )  RATIONAL_B_SPLINE_CURVE ( ( 0.9330127018922194093, 0.9330127018922234061, 1.000000000000000000, 0.8660254037844388186, 1.000000000000000000, 0.8660254037844388186, 1.000000000000000000, 0.9330127018922154125, 0.9330127018922194093 ) ) 
 REPRESENTATION_ITEM ( '' )  );
#11495=CARTESIAN_POINT ( 'NONE',  ( 5.412658773652739619, 3.124999999999988898, -110.8169872981078470 ) ) ;
#11496=VERTEX_POINT ( 'NONE', #6685 ) ;
#11501=ORIENTED_EDGE ( 'NONE', *, *, #28374, .F. ) ;
#11503=( BOUNDED_CURVE ( )  B_SPLINE_CURVE ( 2, ( #27270, #2102, #11509, #22696, #20848, #25597, #20379, #8713, #6242 ),
 .UNSPECIFIED., .F., .T. ) 
 B_SPLINE_CURVE_WITH_KNOTS ( ( 3, 2, 2, 2, 3 ),
 ( 0.04166666666666674068, 0.04259259259259262631, 0.04444444444444439757, 0.04629629629629627985, 0.04722222222222216548 ),
 .UNSPECIFIED. ) 
 CURVE ( )  GEOMETRIC_REPRESENTATION_ITEM ( )  RATIONAL_B_SPLINE_CURVE ( ( 0.9330127018922194093, 0.9330127018922234061, 1.000000000000000000, 0.8660254037844388186, 1.000000000000000000, 0.8660254037844388186, 1.000000000000000000, 0.9330127018922234061, 0.9330127018922194093 ) ) 
 REPRESENTATION_ITEM ( '' )  );
#11506=CARTESIAN_POINT ( 'NONE',  ( 3.175426480543072749, 5.499999999999865885, -88.62500000000001421 ) ) ;
#11507=CARTESIAN_POINT ( 'NONE',  ( -5.412658773652739619, 3.124999999999975131, -105.1830127018922383 ) ) ;
#11508=DIRECTION ( 'NONE',  ( -7.147005652999508048E-36, 5.642372883946980038E-36, 1.000000000000000000 ) ) ;
#11509=CARTESIAN_POINT ( 'NONE',  ( -5.196152422706601826, 2.999999999999975131, -51.96132486540522422 ) ) ;
#11510=CARTESIAN_POINT ( 'NONE',  ( 5.682342569962902878, -9.420267146893145593, -26.96534570410896592 ) ) ;
#11511=ORIENTED_EDGE ( 'NONE', *, *, #8183, .F. ) ;
#11512=CARTESIAN_POINT ( 'NONE',  ( 6.000000000000000888, 1.743066579297358182E-13, -56.16367513459481842 ) ) ;
#11513=EDGE_CURVE ( 'NONE', #26144, #9352, #20984, .T. ) ;
#11514=CARTESIAN_POINT ( 'NONE',  ( -2.775557561562891351E-14, -5.500000000000115463, -171.7500000000000000 ) ) ;
#11516=CARTESIAN_POINT ( 'NONE',  ( 3.175426480543072749, 5.499999999999865885, -162.1250000000000284 ) ) ;
#11518=CARTESIAN_POINT ( 'NONE',  ( 4.763139720814407951, 2.750000000000002665, -105.2500000000000142 ) ) ;
#11519=CARTESIAN_POINT ( 'NONE',  ( 3.464101615137757051, -5.999999999999979572, -159.3363248654052313 ) ) ;
#11520=CARTESIAN_POINT ( 'NONE',  ( -3.464101615137757051, -5.999999999999979572, -122.6636751345948113 ) ) ;
#11521=CARTESIAN_POINT ( 'NONE',  ( -3.175426480542816510, -5.500000000000057732, -95.37500000000004263 ) ) ;
#11523=LINE ( 'NONE', #23330, #18007 ) ;
#11528=ORIENTED_EDGE ( 'NONE', *, *, #15719, .T. ) ;
#11531=ORIENTED_EDGE ( 'NONE', *, *, #16481, .T. ) ;
#11533=ADVANCED_FACE ( 'NONE', ( #19285, #14678 ), #26022, .F. ) ;
#11534=VERTEX_POINT ( 'NONE', #19436 ) ;
#11536=ORIENTED_EDGE ( 'NONE', *, *, #29300, .F. ) ;
#11538=CARTESIAN_POINT ( 'NONE',  ( -3.175426480542816510, -5.500000000000057732, -114.8749999999999858 ) ) ;
#11540=CARTESIAN_POINT ( 'NONE',  ( -7.216878364870328078, 0.000000000000000000, -135.0580127018922667 ) ) ;
#11543=CARTESIAN_POINT ( 'NONE',  ( 5.412658773652712085, -3.125000000000086153, -172.5669872981078186 ) ) ;
#11544=CARTESIAN_POINT ( 'NONE',  ( 2.775557561562891351E-14, 6.250000000000033751, -179.5669872981078186 ) ) ;
#11546=CARTESIAN_POINT ( 'NONE',  ( -3.464101615137725076, 5.999999999999979572, -147.1636751345947687 ) ) ;
#11549=EDGE_CURVE ( 'NONE', #87, #13381, #20168, .T. ) ;
#11554=DIRECTION ( 'NONE',  ( -1.000000000000000000, 1.779758311459930738E-16, 0.000000000000000000 ) ) ;
#11555=CARTESIAN_POINT ( 'NONE',  ( -7.216878364870328078, 0.000000000000000000, -72.69198729810781856 ) ) ;
#11556=CARTESIAN_POINT ( 'NONE',  ( -7.216878364870328078, 0.000000000000000000, -60.69198729810782567 ) ) ;
#11557=CARTESIAN_POINT ( 'NONE',  ( -4.763139720814407951, 2.749999999999946709, -52.25000000000002132 ) ) ;
#11559=CARTESIAN_POINT ( 'NONE',  ( -5.196152422706573404, -3.000000000000002665, -153.7113248654052313 ) ) ;
#11562=CARTESIAN_POINT ( 'NONE',  ( -4.763139720814407951, 2.749999999999946709, -118.2500000000000284 ) ) ;
#11564=CARTESIAN_POINT ( 'NONE',  ( -3.464101615137725076, 5.999999999999979572, -154.0863248654051745 ) ) ;
#11566=CARTESIAN_POINT ( 'NONE',  ( -5.999999999999919176, 1.607695154586804565, -104.9806624327026014 ) ) ;
#11569=FACE_OUTER_BOUND ( 'NONE', #5792, .T. ) ;
#11571=CARTESIAN_POINT ( 'NONE',  ( 5.412658773652712085, -3.125000000000086153, -109.5669872981078186 ) ) ;
#11574=ORIENTED_EDGE ( 'NONE', *, *, #15132, .F. ) ;
#11577=EDGE_CURVE ( 'NONE', #12780, #9068, #6413, .T. ) ;
#11578=AXIS2_PLACEMENT_3D ( 'NONE', #25627, #23344, #30380 ) ;
#11579=CARTESIAN_POINT ( 'NONE',  ( -5.412658773652684552, -3.125000000000099920, -137.0669872981078470 ) ) ;
#11583=CARTESIAN_POINT ( 'NONE',  ( 0.000000000000000000, 0.000000000000000000, 0.000000000000000000 ) ) ;
#11585=FACE_OUTER_BOUND ( 'NONE', #20800, .T. ) ;
#11586=CARTESIAN_POINT ( 'NONE',  ( 3.608439182435180470, 6.249999999999982236, -66.55801270189226670 ) ) ;
#11591=CARTESIAN_POINT ( 'NONE',  ( 3.464101615137852974, 5.999999999999884537, -102.4136751345948255 ) ) ;
#11592=CARTESIAN_POINT ( 'NONE',  ( -5.196152422706573404, -3.000000000000002665, -161.2113248654052313 ) ) ;
#11594=VECTOR ( 'NONE', #2085, 1000.000000000000000 ) ;
#11598=CARTESIAN_POINT ( 'NONE',  ( -2.775557561562891351E-14, -5.500000000000115463, -125.2500000000000284 ) ) ;
#11600=CARTESIAN_POINT ( 'NONE',  ( 6.000000000000000888, -1.859271017917181981E-14, -169.5863248654052029 ) ) ;
#11602=CARTESIAN_POINT ( 'NONE',  ( -4.763139720814407951, 2.749999999999946709, -55.25000000000002132 ) ) ;
#11603=CARTESIAN_POINT ( 'NONE',  ( -5.999999999999963585, -1.487416814333745711E-14, -123.8363248654052171 ) ) ;
#11604=CARTESIAN_POINT ( 'NONE',  ( -5.999999999999963585, 1.780251999655701777E-13, -78.83632486540523132 ) ) ;
#11610=CARTESIAN_POINT ( 'NONE',  ( 2.775557561562891351E-14, -6.250000000000061284, -102.3169872981078470 ) ) ;
#11613=CARTESIAN_POINT ( 'NONE',  ( 6.000000000000000888, -3.330669073875464691E-16, -7.560779664488942560E-35 ) ) ;
#11616=CARTESIAN_POINT ( 'NONE',  ( -3.175426480542816510, -5.500000000000057732, -134.3750000000000284 ) ) ;
#11619=CARTESIAN_POINT ( 'NONE',  ( 3.175426480543072749, -5.500000000000105693, -63.62500000000001421 ) ) ;
#11621=CARTESIAN_POINT ( 'NONE',  ( -5.999999999999963585, -1.487416814333745711E-14, -124.4136751345948255 ) ) ;
#11623=CARTESIAN_POINT ( 'NONE',  ( 3.608439182435180470, 6.249999999999982236, -89.05801270189225249 ) ) ;
#11629=CARTESIAN_POINT ( 'NONE',  ( -6.350852961085760029, -1.281975124255709124E-13, -151.1250000000000284 ) ) ;
#11630=CARTESIAN_POINT ( 'NONE',  ( 0.000000000000000000, 0.000000000000000000, -200.0000000000000000 ) ) ;
#11631=CARTESIAN_POINT ( 'NONE',  ( -6.350852961085760029, -1.281975124255709124E-13, -134.6250000000000284 ) ) ;
#11632=CARTESIAN_POINT ( 'NONE',  ( 5.412658773652739619, 3.124999999999988898, -164.1830127018922383 ) ) ;
#11633=CYLINDRICAL_SURFACE ( 'NONE', #11109, 6.000000000000000888 ) ;
#11634=( BOUNDED_CURVE ( )  B_SPLINE_CURVE ( 2, ( #6850, #14661, #9476, #17272, #3240, #19416, #14953, #12667, #26592 ),
 .UNSPECIFIED., .F., .F. ) 
 B_SPLINE_CURVE_WITH_KNOTS ( ( 3, 2, 2, 2, 3 ),
 ( 0.8416666666666666741, 0.8425925925925925597, 0.8444444444444444420, 0.8462962962962963243, 0.8472222222222222099 ),
 .UNSPECIFIED. ) 
 CURVE ( )  GEOMETRIC_REPRESENTATION_ITEM ( )  RATIONAL_B_SPLINE_CURVE ( ( 0.9330127018922194093, 0.9330127018922194093, 1.000000000000000000, 0.8660254037844388186, 1.000000000000000000, 0.8660254037844388186, 1.000000000000000000, 0.9330127018922194093, 0.9330127018922194093 ) ) 
 REPRESENTATION_ITEM ( '' )  );
#11635=CARTESIAN_POINT ( 'NONE',  ( -6.350852961085760029, -1.281975124255709124E-13, -82.12500000000001421 ) ) ;
#11637=CARTESIAN_POINT ( 'NONE',  ( 4.763139720814407951, 2.750000000000002665, -64.75000000000002842 ) ) ;
#11638=CARTESIAN_POINT ( 'NONE',  ( -5.999999999999904965, -1.607695154586834541, -156.7693375672974128 ) ) ;
#11640=CARTESIAN_POINT ( 'NONE',  ( -3.464101615137757051, -5.999999999999979572, -114.5863248654051745 ) ) ;
#11645=CARTESIAN_POINT ( 'NONE',  ( 5.196152422706629359, 3.000000000000002665, -95.03867513459485394 ) ) ;
#11649=EDGE_LOOP ( 'NONE', ( #18195, #25893, #24712, #2576 ) ) ;
#11653=CARTESIAN_POINT ( 'NONE',  ( -6.350852961085760029, -1.281975124255709124E-13, -154.1250000000000568 ) ) ;
#11654=EDGE_CURVE ( 'NONE', #3053, #26392, #13896, .T. ) ;
#11655=CARTESIAN_POINT ( 'NONE',  ( 5.453341115157027907, 2.554536117543700247, -179.9798858605075509 ) ) ;
#11657=VERTEX_POINT ( 'NONE', #5716 ) ;
#11658=ADVANCED_FACE ( 'NONE', ( #12837 ), #11131, .T. ) ;
#11659=VERTEX_POINT ( 'NONE', #24458 ) ;
#11660=CARTESIAN_POINT ( 'NONE',  ( 3.175426480543072749, -5.500000000000105693, -90.62500000000001421 ) ) ;
#11661=CARTESIAN_POINT ( 'NONE',  ( -7.216878364870328078, 0.000000000000000000, -105.0580127018922525 ) ) ;
#11666=CARTESIAN_POINT ( 'NONE',  ( 6.000249633052443521, -9.219381998443749282, -24.80704692217345197 ) ) ;
#11668=CARTESIAN_POINT ( 'NONE',  ( -5.999999999999971578, 1.607695154586715303, -92.98066243270261566 ) ) ;
#11670=CARTESIAN_POINT ( 'NONE',  ( 6.350852961086080661, -9.614813431917819062E-14, -174.3750000000000284 ) ) ;
#11671=CARTESIAN_POINT ( 'NONE',  ( 0.000000000000000000, -5.999999999999991118, -80.53867513459483973 ) ) ;
#11672=CARTESIAN_POINT ( 'NONE',  ( 6.350852961086080661, -9.614813431917819062E-14, -156.3750000000000000 ) ) ;
#11674=CARTESIAN_POINT ( 'NONE',  ( -5.999999999999963585, 1.780251999655701777E-13, -86.91367513459485394 ) ) ;
#11676=CARTESIAN_POINT ( 'NONE',  ( -4.763139720814407951, -2.750000000000016431, -95.50000000000002842 ) ) ;
#11683=CARTESIAN_POINT ( 'NONE',  ( 6.000000000000000888, -3.330669073875464691E-16, -7.560779664488942560E-35 ) ) ;
#11684=( BOUNDED_CURVE ( )  B_SPLINE_CURVE ( 2, ( #11486, #20828, #18534, #6826, #25568, #2236, #18837, #11638, #14248 ),
 .UNSPECIFIED., .F., .T. ) 
 B_SPLINE_CURVE_WITH_KNOTS ( ( 3, 2, 2, 2, 3 ),
 ( 0.8138888888888888840, 0.8148148148148148806, 0.8166666666666666519, 0.8185185185185185341, 0.8194444444444444198 ),
 .UNSPECIFIED. ) 
 CURVE ( )  GEOMETRIC_REPRESENTATION_ITEM ( )  RATIONAL_B_SPLINE_CURVE ( ( 0.9330127018922194093, 0.9330127018922154125, 1.000000000000000000, 0.8660254037844388186, 1.000000000000000000, 0.8660254037844388186, 1.000000000000000000, 0.9330127018922234061, 0.9330127018922194093 ) ) 
 REPRESENTATION_ITEM ( '' )  );
#11685=VERTEX_POINT ( 'NONE', #20479 ) ;
#11695=CARTESIAN_POINT ( 'NONE',  ( 6.350852961086080661, -9.614813431917819062E-14, -115.8750000000000000 ) ) ;
#11697=CARTESIAN_POINT ( 'NONE',  ( 3.608439182435180470, 6.249999999999982236, -132.5580127018922383 ) ) ;
#11700=CARTESIAN_POINT ( 'NONE',  ( -5.412658773652684552, -3.125000000000099920, -173.0669872981078186 ) ) ;
#11703=CARTESIAN_POINT ( 'NONE',  ( 0.000000000000000000, 5.499999999999991118, -180.0000000000000568 ) ) ;
#11706=CARTESIAN_POINT ( 'NONE',  ( 2.775557561562891351E-14, -6.250000000000061284, -175.1830127018922383 ) ) ;
#11708=CARTESIAN_POINT ( 'NONE',  ( 3.464101615137757051, -5.999999999999979572, -101.4136751345948255 ) ) ;
#11710=CARTESIAN_POINT ( 'NONE',  ( 0.000000000000000000, 5.999999999999977796, -159.2886751345948255 ) ) ;
#11711=CARTESIAN_POINT ( 'NONE',  ( -4.763139720814407951, 2.749999999999946709, -121.2500000000000284 ) ) ;
#11712=CARTESIAN_POINT ( 'NONE',  ( -6.000000000000023093, 1.607695154586625819, -165.9033121635129646 ) ) ;
#11713=CARTESIAN_POINT ( 'NONE',  ( 3.464101615137852974, 5.999999999999884537, -154.3363248654052029 ) ) ;
#11714=ORIENTED_EDGE ( 'NONE', *, *, #6164, .T. ) ;
#11716=EDGE_CURVE ( 'NONE', #22223, #4758, #22796, .T. ) ;
#11719=DIRECTION ( 'NONE',  ( -7.147005652999508048E-36, 5.642372883946980038E-36, 1.000000000000000000 ) ) ;
#11722=CARTESIAN_POINT ( 'NONE',  ( 6.000000000000000888, 7.762456499804234384E-14, -122.1636751345948397 ) ) ;
#11723=CARTESIAN_POINT ( 'NONE',  ( -5.412658773652739619, 3.124999999999975131, -108.8169872981078470 ) ) ;
#11725=CARTESIAN_POINT ( 'NONE',  ( -3.464101615137757051, -5.999999999999979572, -125.6636751345948113 ) ) ;
#11727=CARTESIAN_POINT ( 'NONE',  ( 0.000000000000000000, 0.000000000000000000, 0.000000000000000000 ) ) ;
#11732=CARTESIAN_POINT ( 'NONE',  ( 2.775557561562891351E-14, -6.250000000000061284, -139.8169872981078186 ) ) ;
#11733=CARTESIAN_POINT ( 'NONE',  ( -6.000000000000000888, 1.067854986875958443E-15, 7.560779664488942560E-35 ) ) ;
#11736=CARTESIAN_POINT ( 'NONE',  ( -3.464101615137757051, -5.999999999999979572, -130.1636751345948539 ) ) ;
#11737=DIRECTION ( 'NONE',  ( -7.147005652999508048E-36, 5.642372883946980038E-36, 1.000000000000000000 ) ) ;
#11738=CARTESIAN_POINT ( 'NONE',  ( -7.216878364870328078, 0.000000000000000000, -63.05801270189225249 ) ) ;
#11739=CARTESIAN_POINT ( 'NONE',  ( 0.000000000000000000, 0.000000000000000000, 0.000000000000000000 ) ) ;
#11743=CARTESIAN_POINT ( 'NONE',  ( -5.196152422706573404, -3.000000000000002665, -146.7886751345948255 ) ) ;
#11745=CARTESIAN_POINT ( 'NONE',  ( 5.196152422706629359, 3.000000000000002665, -113.9613248654052171 ) ) ;
#11747=CARTESIAN_POINT ( 'NONE',  ( 6.000000000000052403, -1.607695154586662678, -94.65331216351297883 ) ) ;
#11750=VERTEX_POINT ( 'NONE', #1736 ) ;
#11751=EDGE_CURVE ( 'NONE', #25219, #12504, #9580, .T. ) ;
#11752=CARTESIAN_POINT ( 'NONE',  ( 0.000000000000000000, 5.499999999999991118, -55.49999999999999289 ) ) ;
#11754=CARTESIAN_POINT ( 'NONE',  ( 6.000000000000052403, 1.607695154586625819, -121.5193375672974412 ) ) ;
#11755=CARTESIAN_POINT ( 'NONE',  ( -5.196152422706573404, -3.000000000000002665, -152.2113248654052313 ) ) ;
#11756=AXIS2_PLACEMENT_3D ( 'NONE', #989, #18350, #15913 ) ;
#11760=CARTESIAN_POINT ( 'NONE',  ( 7.216878364870455975, -6.409875621278545621E-14, -104.9419872981078470 ) ) ;
#11761=CARTESIAN_POINT ( 'NONE',  ( 6.000000000000000888, 1.607695154586715303, -177.0193375672974696 ) ) ;
#11766=CARTESIAN_POINT ( 'NONE',  ( -3.175426480542816510, -5.500000000000057732, -140.3750000000000568 ) ) ;
#11770=CARTESIAN_POINT ( 'NONE',  ( 3.175426480543072749, 5.499999999999865885, -67.62500000000002842 ) ) ;
#11771=CARTESIAN_POINT ( 'NONE',  ( 6.000000000000014211, -1.607695154586730180, -164.2306624327026157 ) ) ;
#11772=LINE ( 'NONE', #7277, #22546 ) ;
#11773=CARTESIAN_POINT ( 'NONE',  ( 7.216878364870455975, -6.409875621278545621E-14, -80.30801270189225249 ) ) ;
#11777=DIRECTION ( 'NONE',  ( -7.147005652999508048E-36, 5.642372883946980038E-36, 1.000000000000000000 ) ) ;
#11778=DIRECTION ( 'NONE',  ( 1.000000000000000000, -5.551115123125773458E-17, -1.260129944081490338E-35 ) ) ;
#11780=CARTESIAN_POINT ( 'NONE',  ( -4.763139720814407951, -2.750000000000016431, -145.0000000000000284 ) ) ;
#11782=CARTESIAN_POINT ( 'NONE',  ( -4.763139720814407951, 2.749999999999946709, -139.2499999999999716 ) ) ;
#11783=CARTESIAN_POINT ( 'NONE',  ( 5.412658773652739619, 3.124999999999988898, -161.1830127018922667 ) ) ;
#11784=CARTESIAN_POINT ( 'NONE',  ( 5.196152422706629359, 3.000000000000002665, -116.9613248654052313 ) ) ;
#11785=DIRECTION ( 'NONE',  ( -7.147005652999508048E-36, 5.642372883946980038E-36, 1.000000000000000000 ) ) ;
#11787=CARTESIAN_POINT ( 'NONE',  ( -4.763139720814407951, -2.750000000000016431, -77.50000000000001421 ) ) ;
#11789=CARTESIAN_POINT ( 'NONE',  ( -4.763139720814407951, -2.750000000000016431, -62.50000000000000000 ) ) ;
#11792=CARTESIAN_POINT ( 'NONE',  ( 6.000000000000000888, -3.330669073875464691E-16, -7.560779664488942560E-35 ) ) ;
#11793=FACE_OUTER_BOUND ( 'NONE', #2016, .T. ) ;
#11796=CARTESIAN_POINT ( 'NONE',  ( 6.000000000000052403, -1.607695154586662678, -49.65331216351296462 ) ) ;
#11799=ADVANCED_FACE ( 'NONE', ( #20024 ), #17590, .T. ) ;
#11800=CARTESIAN_POINT ( 'NONE',  ( -6.000000000000007105, -1.607695154586655129, -98.26933756729742697 ) ) ;
#11801=ORIENTED_EDGE ( 'NONE', *, *, #21426, .F. ) ;
#11802=VECTOR ( 'NONE', #16800, 1000.000000000000000 ) ;
#11804=LINE ( 'NONE', #25111, #10175 ) ;
#11806=AXIS2_PLACEMENT_3D ( 'NONE', #3067, #22848, #28863 ) ;
#11807=CARTESIAN_POINT ( 'NONE',  ( -5.999999999999919176, 1.607695154586804565, -179.4033121635130215 ) ) ;
#11809=ORIENTED_EDGE ( 'NONE', *, *, #21231, .F. ) ;
#11811=ORIENTED_EDGE ( 'NONE', *, *, #8908, .T. ) ;
#11812=CARTESIAN_POINT ( 'NONE',  ( -2.775557561562891351E-14, -5.500000000000115463, -86.25000000000004263 ) ) ;
#11813=CARTESIAN_POINT ( 'NONE',  ( -3.608439182435115633, 6.249999999999965361, -106.8080127018922667 ) ) ;
#11815=CARTESIAN_POINT ( 'NONE',  ( 3.199609099280345870, 10.52573284576699386, -30.07939160056614014 ) ) ;
#11817=( BOUNDED_CURVE ( )  B_SPLINE_CURVE ( 2, ( #4951, #18978, #51, #23427, #6669, #2656, #6813, #9440, #21264 ),
 .UNSPECIFIED., .F., .F. ) 
 B_SPLINE_CURVE_WITH_KNOTS ( ( 3, 2, 2, 2, 3 ),
 ( 0.3083333333333333481, 0.3092592592592592338, 0.3111111111111111160, 0.3129629629629629428, 0.3138888888888888840 ),
 .UNSPECIFIED. ) 
 CURVE ( )  GEOMETRIC_REPRESENTATION_ITEM ( )  RATIONAL_B_SPLINE_CURVE ( ( 0.9330127018922194093, 0.9330127018922214077, 1.000000000000000000, 0.8660254037844388186, 1.000000000000000000, 0.8660254037844388186, 1.000000000000000000, 0.9330127018922194093, 0.9330127018922194093 ) ) 
 REPRESENTATION_ITEM ( '' )  );
#11818=CARTESIAN_POINT ( 'NONE',  ( 5.412658773652712085, -3.125000000000086153, -47.43301270189226670 ) ) ;
#11822=CARTESIAN_POINT ( 'NONE',  ( -3.175426480542816066, 5.499999999999865885, -169.3750000000000568 ) ) ;
#11824=CARTESIAN_POINT ( 'NONE',  ( 0.000000000000000000, 5.499999999999991118, -151.5000000000000284 ) ) ;
#11828=CARTESIAN_POINT ( 'NONE',  ( 4.763139720814407951, 2.750000000000002665, -102.2500000000000142 ) ) ;
#11832=CARTESIAN_POINT ( 'NONE',  ( -6.350852961085760029, -1.281975124255709124E-13, -91.12500000000001421 ) ) ;
#11835=ORIENTED_EDGE ( 'NONE', *, *, #10508, .T. ) ;
#11840=DIRECTION ( 'NONE',  ( -7.147005652999508048E-36, 5.642372883946980038E-36, 1.000000000000000000 ) ) ;
#11841=ORIENTED_EDGE ( 'NONE', *, *, #16874, .F. ) ;
#11843=DIRECTION ( 'NONE',  ( -7.147005652999508048E-36, 5.642372883946980038E-36, 1.000000000000000000 ) ) ;
#11845=ORIENTED_EDGE ( 'NONE', *, *, #17517, .T. ) ;
#11846=CARTESIAN_POINT ( 'NONE',  ( -5.999999999999963585, 1.780251999655701777E-13, -53.33632486540522422 ) ) ;
#11847=ORIENTED_EDGE ( 'NONE', *, *, #7532, .F. ) ;
#11849=CARTESIAN_POINT ( 'NONE',  ( 6.350852961086080661, -9.614813431917819062E-14, -111.3750000000000568 ) ) ;
#11851=CARTESIAN_POINT ( 'NONE',  ( 3.608439182435180470, 6.249999999999982236, -131.0580127018922383 ) ) ;
#11853=CYLINDRICAL_SURFACE ( 'NONE', #14233, 6.000000000000000888 ) ;
#11854=CARTESIAN_POINT ( 'NONE',  ( 2.775557561562891351E-14, 6.250000000000033751, -169.0669872981078186 ) ) ;
#11857=ORIENTED_EDGE ( 'NONE', *, *, #14457, .F. ) ;
#11859=( BOUNDED_CURVE ( )  B_SPLINE_CURVE ( 2, ( #9604, #18994, #28317, #4968, #2667, #1227, #8929, #1698, #10948 ),
 .UNSPECIFIED., .F., .T. ) 
 B_SPLINE_CURVE_WITH_KNOTS ( ( 3, 2, 2, 2, 3 ),
 ( 0.2472222222222222043, 0.2481481481481481455, 0.2500000000000000000, 0.2518518518518518268, 0.2527777777777777679 ),
 .UNSPECIFIED. ) 
 CURVE ( )  GEOMETRIC_REPRESENTATION_ITEM ( )  RATIONAL_B_SPLINE_CURVE ( ( 0.9330127018922196314, 0.9330127018922185211, 1.000000000000000000, 0.8660254037844388186, 1.000000000000000000, 0.8660254037844388186, 1.000000000000000000, 0.9330127018922194093, 0.9330127018922194093 ) ) 
 REPRESENTATION_ITEM ( '' )  );
#11861=CARTESIAN_POINT ( 'NONE',  ( 6.000000000000000888, 1.607695154586715303, -137.0966878364870354 ) ) ;
#11862=CARTESIAN_POINT ( 'NONE',  ( 3.175426480543072749, -5.500000000000105693, -177.6250000000000284 ) ) ;
#11864=CARTESIAN_POINT ( 'NONE',  ( 5.412658773652712085, -3.125000000000086153, -179.4330127018922667 ) ) ;
#11870=CARTESIAN_POINT ( 'NONE',  ( -3.175426480542816510, -5.500000000000057732, -111.8750000000000568 ) ) ;
#11871=( BOUNDED_CURVE ( )  B_SPLINE_CURVE ( 2, ( #3869, #8170, #3721, #27516, #27368, #13601, #15761, #1884, #13150 ),
 .UNSPECIFIED., .F., .T. ) 
 B_SPLINE_CURVE_WITH_KNOTS ( ( 3, 2, 2, 2, 3 ),
 ( 0.1361111111111110994, 0.1370370370370370405, 0.1388888888888888951, 0.1407407407407407496, 0.1416666666666666907 ),
 .UNSPECIFIED. ) 
 CURVE ( )  GEOMETRIC_REPRESENTATION_ITEM ( )  RATIONAL_B_SPLINE_CURVE ( ( 0.9330127018922196314, 0.9330127018922185211, 1.000000000000000000, 0.8660254037844388186, 1.000000000000000000, 0.8660254037844388186, 1.000000000000000000, 0.9330127018922184101, 0.9330127018922194093 ) ) 
 REPRESENTATION_ITEM ( '' )  );
#11874=ORIENTED_EDGE ( 'NONE', *, *, #26530, .T. ) ;
#11877=CARTESIAN_POINT ( 'NONE',  ( 6.000000000000052403, -1.607695154586662678, -55.65331216351297172 ) ) ;
#11878=DIRECTION ( 'NONE',  ( 1.000000000000000000, -5.551115123125773458E-17, -1.260129944081490338E-35 ) ) ;
#11879=FACE_OUTER_BOUND ( 'NONE', #23164, .T. ) ;
#11884=CARTESIAN_POINT ( 'NONE',  ( -3.464101615137757051, -5.999999999999979572, -95.66367513459481131 ) ) ;
#11886=ORIENTED_EDGE ( 'NONE', *, *, #9891, .T. ) ;
#11891=CARTESIAN_POINT ( 'NONE',  ( -3.608439182435052128, -6.250000000000110134, -136.9419872981078186 ) ) ;
#11894=EDGE_CURVE ( 'NONE', #27647, #11657, #157, .T. ) ;
#11897=CARTESIAN_POINT ( 'NONE',  ( -5.999999999999956479, -1.607695154586745057, -137.8466878364870638 ) ) ;
#11909=CARTESIAN_POINT ( 'NONE',  ( -3.464101615137725076, 5.999999999999979572, -148.6636751345947403 ) ) ;
#11910=ORIENTED_EDGE ( 'NONE', *, *, #7985, .F. ) ;
#11913=CARTESIAN_POINT ( 'NONE',  ( -4.763139720814407951, 2.749999999999946709, -52.25000000000002132 ) ) ;
#11914=CARTESIAN_POINT ( 'NONE',  ( -5.196152422706601826, 2.999999999999975131, -87.96132486540520290 ) ) ;
#11915=DIRECTION ( 'NONE',  ( -7.147005652999508048E-36, 5.642372883946980038E-36, 1.000000000000000000 ) ) ;
#11917=ORIENTED_EDGE ( 'NONE', *, *, #22581, .T. ) ;
#11920=CARTESIAN_POINT ( 'NONE',  ( -5.412658773652739619, 3.124999999999975131, -99.81698729810784698 ) ) ;
#11924=VERTEX_POINT ( 'NONE', #17690 ) ;
#11925=CIRCLE ( 'NONE', #18768, 4.000000000000006217 ) ;
#11926=CARTESIAN_POINT ( 'NONE',  ( 0.000000000000000000, 5.499999999999991118, -141.0000000000000000 ) ) ;
#11929=EDGE_CURVE ( 'NONE', #25500, #9277, #7244, .T. ) ;
#11930=CARTESIAN_POINT ( 'NONE',  ( 3.175426480543072749, 5.499999999999865885, -64.62500000000001421 ) ) ;
#11931=AXIS2_PLACEMENT_3D ( 'NONE', #1719, #24764, #29357 ) ;
#11932=DIRECTION ( 'NONE',  ( -7.147005652999508048E-36, 5.642372883946980038E-36, 1.000000000000000000 ) ) ;
#11934=CARTESIAN_POINT ( 'NONE',  ( 5.412658773652739619, 3.124999999999988898, -80.18301270189220986 ) ) ;
#11939=CARTESIAN_POINT ( 'NONE',  ( -5.999999999999919176, 1.607695154586804565, -60.90331216351300725 ) ) ;
#11943=CARTESIAN_POINT ( 'NONE',  ( 3.175426480543072749, -5.500000000000105693, -147.6250000000000284 ) ) ;
#11944=CARTESIAN_POINT ( 'NONE',  ( 6.000000000000000888, -1.607695154586752384, -105.1533121635130215 ) ) ;
#11945=EDGE_CURVE ( 'NONE', #29849, #14641, #2537, .T. ) ;
#11946=CARTESIAN_POINT ( 'NONE',  ( -5.412658773652684552, -3.125000000000099920, -160.4330127018922667 ) ) ;
#11947=CARTESIAN_POINT ( 'NONE',  ( -3.464101615137725076, 5.999999999999979572, -89.58632486540521711 ) ) ;
#11948=AXIS2_PLACEMENT_3D ( 'NONE', #17867, #22606, #1541 ) ;
#11949=CARTESIAN_POINT ( 'NONE',  ( -4.763139720814407951, 2.749999999999946709, -77.74999999999998579 ) ) ;
#11950=CARTESIAN_POINT ( 'NONE',  ( 3.175426480543072749, -5.500000000000105693, -66.62500000000002842 ) ) ;
#11958=DIRECTION ( 'NONE',  ( -7.147005652999508048E-36, 5.642372883946980038E-36, 1.000000000000000000 ) ) ;
#11963=CARTESIAN_POINT ( 'NONE',  ( 4.763139720814407951, 2.750000000000002665, -153.2500000000000000 ) ) ;
#11966=CARTESIAN_POINT ( 'NONE',  ( 7.216878364870455975, -6.409875621278545621E-14, -154.4419872981078186 ) ) ;
#11968=EDGE_CURVE ( 'NONE', #14907, #28127, #4882, .T. ) ;
#11969=CARTESIAN_POINT ( 'NONE',  ( 4.763139720814407951, -2.749999999999988454, -93.50000000000002842 ) ) ;
#11973=CARTESIAN_POINT ( 'NONE',  ( 4.763139720814407951, -2.749999999999988454, -168.4999999999999716 ) ) ;
#11974=DIRECTION ( 'NONE',  ( -7.147005652999508048E-36, 5.642372883946980038E-36, 1.000000000000000000 ) ) ;
#11975=EDGE_CURVE ( 'NONE', #2318, #25700, #16868, .T. ) ;
#11976=ADVANCED_FACE ( 'NONE', ( #30395 ), #25472, .T. ) ;
#11977=CARTESIAN_POINT ( 'NONE',  ( 3.175426480543072749, 5.499999999999865885, -171.1250000000000000 ) ) ;
#11979=CARTESIAN_POINT ( 'NONE',  ( 3.175426480543072749, -5.500000000000105693, -153.6250000000000568 ) ) ;
#11980=CARTESIAN_POINT ( 'NONE',  ( -3.175426480542816066, 5.499999999999865885, -101.8750000000000142 ) ) ;
#11982=CARTESIAN_POINT ( 'NONE',  ( 4.763139720814407951, -2.749999999999988454, -156.5000000000000284 ) ) ;
#11983=CARTESIAN_POINT ( 'NONE',  ( 4.763139720814407951, 2.750000000000002665, -93.25000000000000000 ) ) ;
#11994=CARTESIAN_POINT ( 'NONE',  ( 0.000000000000000000, 0.000000000000000000, 0.000000000000000000 ) ) ;
#11995=ORIENTED_EDGE ( 'NONE', *, *, #19625, .F. ) ;
#11996=CARTESIAN_POINT ( 'NONE',  ( -5.999999999999956479, -1.607695154586745057, -141.7693375672974128 ) ) ;
#11998=VERTEX_POINT ( 'NONE', #12009 ) ;
#12000=CARTESIAN_POINT ( 'NONE',  ( -4.763139720814407951, 2.749999999999946709, -116.7500000000000142 ) ) ;
#12002=CARTESIAN_POINT ( 'NONE',  ( 5.412658773652739619, 3.124999999999988898, -120.6830127018922383 ) ) ;
#12004=DIRECTION ( 'NONE',  ( -7.147005652999508048E-36, 5.642372883946980038E-36, 1.000000000000000000 ) ) ;
#12005=CARTESIAN_POINT ( 'NONE',  ( 2.775557561562891351E-14, 6.250000000000033751, -166.0669872981078186 ) ) ;
#12007=ORIENTED_EDGE ( 'NONE', *, *, #26577, .F. ) ;
#12009=CARTESIAN_POINT ( 'NONE',  ( -5.999999999999962697, 3.323446944526963891E-14, -152.9136751345948255 ) ) ;
#12010=CARTESIAN_POINT ( 'NONE',  ( -6.350852961085760029, -1.281975124255709124E-13, -176.6250000000000568 ) ) ;
#12012=CARTESIAN_POINT ( 'NONE',  ( -5.412658773652684552, -3.125000000000099920, -173.9330127018922099 ) ) ;
#12016=CARTESIAN_POINT ( 'NONE',  ( -2.775557561562891351E-14, -5.500000000000115463, -111.7500000000000142 ) ) ;
#12018=CARTESIAN_POINT ( 'NONE',  ( 6.000000000000000888, -1.859271017917181981E-14, -89.16367513459485394 ) ) ;
#12019=VERTEX_POINT ( 'NONE', #9206 ) ;
#12022=DIRECTION ( 'NONE',  ( -7.147005652999508048E-36, 5.642372883946980038E-36, 1.000000000000000000 ) ) ;
#12023=CARTESIAN_POINT ( 'NONE',  ( 0.000000000000000000, 5.999999999999977796, -131.7113248654052029 ) ) ;
#12026=CARTESIAN_POINT ( 'NONE',  ( -4.763139720814407951, -2.750000000000016431, -179.5000000000000000 ) ) ;
#12028=CARTESIAN_POINT ( 'NONE',  ( -5.999999999999963585, 1.780251999655701777E-13, -77.91367513459482552 ) ) ;
#12029=CARTESIAN_POINT ( 'NONE',  ( 6.000000000000000888, 1.743066579297358182E-13, -57.66367513459481842 ) ) ;
#12034=EDGE_CURVE ( 'NONE', #28360, #22536, #18599, .T. ) ;
#12035=( BOUNDED_SURFACE ( )  B_SPLINE_SURFACE ( 2, 3, ( 
 ( #30326, #18528, #9448, #20824 ),
 ( #14245, #9287, #9136, #23729 ),
 ( #27853, #23437, #6822, #21270 ) ),
 .UNSPECIFIED., .F., .F., .T. ) 
 B_SPLINE_SURFACE_WITH_KNOTS ( ( 3, 3 ),
 ( 4, 4 ),
 ( 0.000000000000000000, 1.000000000000000000 ),
 ( 0.000000000000000000, 1.000000000000000000 ),
 .UNSPECIFIED. ) 
 GEOMETRIC_REPRESENTATION_ITEM ( )  RATIONAL_B_SPLINE_SURFACE ( (
 ( 1.000000000000000000, 0.3333333333333334259, 0.3333333333333334259, 1.000000000000000000),
 ( 1.000000000000000000, 0.3333333333333334259, 0.3333333333333334259, 1.000000000000000000),
 ( 1.000000000000000000, 0.3333333333333334259, 0.3333333333333334259, 1.000000000000000000) ) ) 
 REPRESENTATION_ITEM ( '' )  SURFACE ( )  );
#12038=CARTESIAN_POINT ( 'NONE',  ( 5.412658773652712085, -3.125000000000086153, -142.5669872981077901 ) ) ;
#12041=CARTESIAN_POINT ( 'NONE',  ( -3.464101615137725076, 5.999999999999979572, -129.1636751345948255 ) ) ;
#12046=CARTESIAN_POINT ( 'NONE',  ( -5.999999999999963585, 1.780251999655701777E-13, -56.91367513459483973 ) ) ;
#12047=CARTESIAN_POINT ( 'NONE',  ( 0.000000000000000000, -5.999999999999991118, -99.46132486540525974 ) ) ;
#12048=CARTESIAN_POINT ( 'NONE',  ( 11.00000000000001599, -6.106226635438360972E-16, -43.99152654425658682 ) ) ;
#12049=CARTESIAN_POINT ( 'NONE',  ( -3.464101615137725076, 5.999999999999979572, -60.16367513459481842 ) ) ;
#12052=CARTESIAN_POINT ( 'NONE',  ( -5.999999999999919176, 1.607695154586804565, -112.4806624327025872 ) ) ;
#12054=CARTESIAN_POINT ( 'NONE',  ( -6.000000000000007105, -1.607695154586655129, -107.2693375672974838 ) ) ;
#12057=ORIENTED_EDGE ( 'NONE', *, *, #29025, .F. ) ;
#12061=CARTESIAN_POINT ( 'NONE',  ( 5.412658773652712085, -3.125000000000086153, -105.0669872981078186 ) ) ;
#12062=CARTESIAN_POINT ( 'NONE',  ( 5.196152422706629359, 3.000000000000002665, -176.9613248654052313 ) ) ;
#12066=CARTESIAN_POINT ( 'NONE',  ( -3.175426480542816510, 5.499999999999865885, -133.3750000000000284 ) ) ;
#12070=ORIENTED_EDGE ( 'NONE', *, *, #7375, .F. ) ;
#12073=CARTESIAN_POINT ( 'NONE',  ( -3.175426480542816510, 5.499999999999865885, -56.87500000000004974 ) ) ;
#12076=CARTESIAN_POINT ( 'NONE',  ( -5.412658773652739619, 3.124999999999975131, -87.18301270189220986 ) ) ;
#12078=( BOUNDED_CURVE ( )  B_SPLINE_CURVE ( 2, ( #20934, #7247, #13904, #4327, #14351, #27809, #2186, #28267, #16356 ),
 .UNSPECIFIED., .F., .F. ) 
 B_SPLINE_CURVE_WITH_KNOTS ( ( 3, 2, 2, 2, 3 ),
 ( 0.8249999999999999556, 0.8259259259259259522, 0.8277777777777777235, 0.8296296296296296058, 0.8305555555555556024 ),
 .UNSPECIFIED. ) 
 CURVE ( )  GEOMETRIC_REPRESENTATION_ITEM ( )  RATIONAL_B_SPLINE_CURVE ( ( 0.9330127018922194093, 0.9330127018922154125, 1.000000000000000000, 0.8660254037844388186, 1.000000000000000000, 0.8660254037844388186, 1.000000000000000000, 0.9330127018922154125, 0.9330127018922194093 ) ) 
 REPRESENTATION_ITEM ( '' )  );
#12082=CARTESIAN_POINT ( 'NONE',  ( -2.775557561562891351E-14, -5.500000000000115463, -141.7500000000000568 ) ) ;
#12084=CARTESIAN_POINT ( 'NONE',  ( 5.412658773652712085, -3.125000000000086153, -150.9330127018922383 ) ) ;
#12085=CARTESIAN_POINT ( 'NONE',  ( -5.196152422706601826, 2.999999999999975131, -116.4613248654052313 ) ) ;
#12086=CARTESIAN_POINT ( 'NONE',  ( 0.000000000000000000, -5.999999999999991118, -73.03867513459482552 ) ) ;
#12087=CARTESIAN_POINT ( 'NONE',  ( -4.763139720814407951, 2.749999999999946709, -68.75000000000002842 ) ) ;
#12088=CARTESIAN_POINT ( 'NONE',  ( -5.999999999999919176, 1.607695154586804565, -85.48066243270261566 ) ) ;
#12090=CARTESIAN_POINT ( 'NONE',  ( 0.000000000000000000, 5.499999999999991118, -61.50000000000000000 ) ) ;
#12093=AXIS2_PLACEMENT_3D ( 'NONE', #26789, #20367, #22216 ) ;
#12099=ORIENTED_EDGE ( 'NONE', *, *, #21518, .T. ) ;
#12101=CARTESIAN_POINT ( 'NONE',  ( -3.175426480542816510, 5.499999999999865885, -154.3749999999999716 ) ) ;
#12103=CARTESIAN_POINT ( 'NONE',  ( -3.464101615137757051, -5.999999999999979572, -158.6636751345948255 ) ) ;
#12105=CARTESIAN_POINT ( 'NONE',  ( -4.763139720814407951, 2.749999999999946709, -181.2500000000000284 ) ) ;
#12107=ORIENTED_EDGE ( 'NONE', *, *, #21874, .F. ) ;
#12108=CARTESIAN_POINT ( 'NONE',  ( 5.412658773652739619, 3.124999999999988898, -154.3169872981078470 ) ) ;
#12111=CARTESIAN_POINT ( 'NONE',  ( 4.763139720814407951, 2.750000000000002665, -87.25000000000005684 ) ) ;
#12112=ORIENTED_EDGE ( 'NONE', *, *, #17767, .T. ) ;
#12117=CARTESIAN_POINT ( 'NONE',  ( 1.580833713216741820, -10.88751498504594473, -19.20858708930976277 ) ) ;
#12118=DIRECTION ( 'NONE',  ( 1.000000000000000000, -5.551115123125773458E-17, -1.260129944081490338E-35 ) ) ;
#12119=SURFACE_STYLE_USAGE ( .BOTH. , #2409 ) ;
#12120=CARTESIAN_POINT ( 'NONE',  ( 4.763139720814407951, 2.750000000000002665, -165.2500000000000000 ) ) ;
#12121=CARTESIAN_POINT ( 'NONE',  ( 6.350852961086080661, -9.614813431917819062E-14, -151.8749999999999716 ) ) ;
#12124=CARTESIAN_POINT ( 'NONE',  ( -4.763139720814407951, -2.750000000000016431, -101.5000000000000284 ) ) ;
#12127=CARTESIAN_POINT ( 'NONE',  ( 3.175426480543072749, 5.499999999999865885, -87.12500000000000000 ) ) ;
#12129=CARTESIAN_POINT ( 'NONE',  ( -5.999999999999963585, 8.134310703387671600E-14, -136.4136751345948255 ) ) ;
#12134=CARTESIAN_POINT ( 'NONE',  ( -5.999999999999971578, 1.607695154586715303, -71.98066243270261566 ) ) ;
#12138=CARTESIAN_POINT ( 'NONE',  ( -6.000000000000000888, 1.067854986875958443E-15, 7.560779664488942560E-35 ) ) ;
#12143=VERTEX_POINT ( 'NONE', #19077 ) ;
#12144=CARTESIAN_POINT ( 'NONE',  ( 3.175426480543072749, -5.500000000000105693, -116.1250000000000000 ) ) ;
#12146=CARTESIAN_POINT ( 'NONE',  ( -5.412658773652684552, -3.125000000000099920, -125.9330127018922809 ) ) ;
#12148=ORIENTED_EDGE ( 'NONE', *, *, #22431, .F. ) ;
#12150=CARTESIAN_POINT ( 'NONE',  ( -7.216878364870328078, 0.000000000000000000, -159.6919872981078754 ) ) ;
#12154=VERTEX_POINT ( 'NONE', #28394 ) ;
#12157=CARTESIAN_POINT ( 'NONE',  ( 4.763139720814407951, 2.750000000000002665, -175.7500000000000284 ) ) ;
#12160=CARTESIAN_POINT ( 'NONE',  ( -3.608439182435052128, -6.250000000000110134, -173.8080127018922383 ) ) ;
#12162=CARTESIAN_POINT ( 'NONE',  ( -6.350852961085760029, -1.281975124255709124E-13, -122.6250000000000426 ) ) ;
#12164=CARTESIAN_POINT ( 'NONE',  ( -4.763139720814407951, 2.749999999999946709, -116.7500000000000142 ) ) ;
#12166=CARTESIAN_POINT ( 'NONE',  ( 3.464101615137852974, 5.999999999999884537, -100.9136751345948255 ) ) ;
#12167=ORIENTED_EDGE ( 'NONE', *, *, #12719, .T. ) ;
#12170=EDGE_CURVE ( 'NONE', #7855, #12780, #7416, .T. ) ;
#12171=CARTESIAN_POINT ( 'NONE',  ( 0.000000000000000000, -5.999999999999991118, -136.9613248654052313 ) ) ;
#12175=ORIENTED_EDGE ( 'NONE', *, *, #7375, .T. ) ;
#12178=CARTESIAN_POINT ( 'NONE',  ( -3.175426480542816066, -5.500000000000057732, -177.8750000000000284 ) ) ;
#12190=CARTESIAN_POINT ( 'NONE',  ( 5.412658773652739619, 3.124999999999988898, -128.8169872981078186 ) ) ;
#12196=LINE ( 'NONE', #23977, #15725 ) ;
#12199=CARTESIAN_POINT ( 'NONE',  ( 3.464101615137757051, -5.999999999999979572, -99.33632486540518869 ) ) ;
#12202=CARTESIAN_POINT ( 'NONE',  ( 0.000000000000000000, 5.999999999999977796, -113.7113248654052455 ) ) ;
#12206=ORIENTED_EDGE ( 'NONE', *, *, #26065, .T. ) ;
#12207=EDGE_CURVE ( 'NONE', #19051, #16860, #5422, .T. ) ;
#12208=CARTESIAN_POINT ( 'NONE',  ( 3.175426480543072749, -5.500000000000105693, -47.12500000000006395 ) ) ;
#12216=CARTESIAN_POINT ( 'NONE',  ( 5.412658773652712085, -3.125000000000086153, -106.5669872981078186 ) ) ;
#12217=( BOUNDED_CURVE ( )  B_SPLINE_CURVE ( 2, ( #27201, #27500, #12977, #13131, #8633, #22469, #22311, #1563, #6014 ),
 .UNSPECIFIED., .F., .T. ) 
 B_SPLINE_CURVE_WITH_KNOTS ( ( 3, 2, 2, 2, 3 ),
 ( 0.2472222222222222321, 0.2481481481481481177, 0.2500000000000000000, 0.2518518518518518823, 0.2527777777777777679 ),
 .UNSPECIFIED. ) 
 CURVE ( )  GEOMETRIC_REPRESENTATION_ITEM ( )  RATIONAL_B_SPLINE_CURVE ( ( 0.9330127018922194093, 0.9330127018922194093, 1.000000000000000000, 0.8660254037844388186, 1.000000000000000000, 0.8660254037844388186, 1.000000000000000000, 0.9330127018922194093, 0.9330127018922194093 ) ) 
 REPRESENTATION_ITEM ( '' )  );
#12220=CARTESIAN_POINT ( 'NONE',  ( -4.763139720814407951, 2.749999999999946709, -131.7500000000000284 ) ) ;
#12223=ORIENTED_EDGE ( 'NONE', *, *, #19829, .F. ) ;
#12225=CARTESIAN_POINT ( 'NONE',  ( -3.175426480542816510, -5.500000000000057732, -57.87500000000004974 ) ) ;
#12226=CARTESIAN_POINT ( 'NONE',  ( -5.999999999999944933, 1.607695154586759934, -115.4806624327025872 ) ) ;
#12227=CARTESIAN_POINT ( 'NONE',  ( 6.000000000000000888, 5.577813053751546416E-15, -177.0863248654052597 ) ) ;
#12228=CARTESIAN_POINT ( 'NONE',  ( 5.412658773652739619, 3.124999999999988898, -84.68301270189226670 ) ) ;
#12234=CARTESIAN_POINT ( 'NONE',  ( -2.775557561562891351E-14, -5.500000000000115463, -138.7500000000000284 ) ) ;
#12236=CARTESIAN_POINT ( 'NONE',  ( -5.412658773652684552, -3.125000000000099920, -149.9330127018922383 ) ) ;
#12237=CARTESIAN_POINT ( 'NONE',  ( 6.000000000000000888, 1.743066579297358182E-13, -102.0863248654051887 ) ) ;
#12239=CARTESIAN_POINT ( 'NONE',  ( -2.775557561562891351E-14, -5.500000000000115463, -74.25000000000004263 ) ) ;
#12240=CARTESIAN_POINT ( 'NONE',  ( 6.350852961086080661, -9.614813431917819062E-14, -69.37500000000004263 ) ) ;
#12241=EDGE_CURVE ( 'NONE', #24992, #9072, #12558, .T. ) ;
#12242=CARTESIAN_POINT ( 'NONE',  ( -3.464101615137725076, 5.999999999999979572, -53.58632486540517448 ) ) ;
#12247=CARTESIAN_POINT ( 'NONE',  ( 3.464101615137757051, -5.999999999999979572, -147.3363248654051745 ) ) ;
#12249=CARTESIAN_POINT ( 'NONE',  ( -5.999999999999982236, -1.607695154586700426, -145.3466878364870354 ) ) ;
#12250=ORIENTED_EDGE ( 'NONE', *, *, #26126, .T. ) ;
#12255=CARTESIAN_POINT ( 'NONE',  ( 4.763139720814407951, -2.749999999999988454, -177.5000000000000000 ) ) ;
#12258=CARTESIAN_POINT ( 'NONE',  ( 6.350852961086080661, -9.614813431917819062E-14, -81.37500000000004263 ) ) ;
#12259=FACE_OUTER_BOUND ( 'NONE', #6722, .T. ) ;
#12261=CARTESIAN_POINT ( 'NONE',  ( -2.775557561562891351E-14, -5.500000000000115463, -168.7500000000000000 ) ) ;
#12262=CARTESIAN_POINT ( 'NONE',  ( 6.000000000000000888, 1.607695154586715303, -54.59668783648703538 ) ) ;
#12263=CARTESIAN_POINT ( 'NONE',  ( 5.196152422706629359, 3.000000000000002665, -59.03867513459481842 ) ) ;
#12266=CARTESIAN_POINT ( 'NONE',  ( -4.763139720814407951, 2.749999999999946709, -163.2500000000000000 ) ) ;
#12267=CARTESIAN_POINT ( 'NONE',  ( 0.000000000000000000, 5.999999999999977796, -161.7113248654051745 ) ) ;
#12268=CARTESIAN_POINT ( 'NONE',  ( -3.175426480542816510, 5.499999999999865885, -154.3749999999999716 ) ) ;
#12269=CARTESIAN_POINT ( 'NONE',  ( -5.196152422706601826, 2.999999999999975131, -76.53867513459483973 ) ) ;
#12272=CARTESIAN_POINT ( 'NONE',  ( 0.000000000000000000, 5.499999999999991118, -97.50000000000002842 ) ) ;
#12274=CARTESIAN_POINT ( 'NONE',  ( -4.763139720814407951, -2.750000000000016431, -88.00000000000002842 ) ) ;
#12275=EDGE_CURVE ( 'NONE', #1827, #9271, #24264, .T. ) ;
#12280=CARTESIAN_POINT ( 'NONE',  ( 6.000000000000000888, 1.607695154586715303, -126.5966878364870638 ) ) ;
#12281=CARTESIAN_POINT ( 'NONE',  ( 6.000000000000052403, -1.607695154586662678, -73.65331216351297883 ) ) ;
#12283=ORIENTED_EDGE ( 'NONE', *, *, #9647, .T. ) ;
#12284=SURFACE_STYLE_FILL_AREA ( #23776 ) ;
#12285=FACE_OUTER_BOUND ( 'NONE', #10944, .T. ) ;
#12289=CARTESIAN_POINT ( 'NONE',  ( -6.350852961085760029, -1.281975124255709124E-13, -106.1250000000000142 ) ) ;
#12292=CARTESIAN_POINT ( 'NONE',  ( 2.775557561562891351E-14, 6.250000000000033751, -121.9330127018922667 ) ) ;
#12293=ORIENTED_EDGE ( 'NONE', *, *, #5754, .T. ) ;
#12295=CARTESIAN_POINT ( 'NONE',  ( 5.412658773652739619, 3.124999999999988898, -161.8169872981078470 ) ) ;
#12299=EDGE_CURVE ( 'NONE', #14750, #11534, #1659, .T. ) ;
#12300=CARTESIAN_POINT ( 'NONE',  ( 7.216878364870455975, -6.409875621278545621E-14, -57.80801270189221697 ) ) ;
#12303=( BOUNDED_CURVE ( )  B_SPLINE_CURVE ( 2, ( #29883, #1629, #1473, #29729, #27562, #14518, #2947, #5091, #19410 ),
 .UNSPECIFIED., .F., .T. ) 
 B_SPLINE_CURVE_WITH_KNOTS ( ( 3, 2, 2, 2, 3 ),
 ( 0.6305555555555556468, 0.6314814814814815325, 0.6333333333333333037, 0.6351851851851851860, 0.6361111111111110716 ),
 .UNSPECIFIED. ) 
 CURVE ( )  GEOMETRIC_REPRESENTATION_ITEM ( )  RATIONAL_B_SPLINE_CURVE ( ( 0.9330127018922194093, 0.9330127018922234061, 1.000000000000000000, 0.8660254037844388186, 1.000000000000000000, 0.8660254037844388186, 1.000000000000000000, 0.9330127018922234061, 0.9330127018922194093 ) ) 
 REPRESENTATION_ITEM ( '' )  );
#12304=DIRECTION ( 'NONE',  ( -7.147005652999508048E-36, 5.642372883946980038E-36, 1.000000000000000000 ) ) ;
#12305=CARTESIAN_POINT ( 'NONE',  ( 6.000000000000000000, 2.951592740943527306E-14, -156.0863248654052597 ) ) ;
#12306=CARTESIAN_POINT ( 'NONE',  ( 4.763139720814407951, 2.750000000000002665, -180.2500000000000284 ) ) ;
#12308=CARTESIAN_POINT ( 'NONE',  ( -7.216878364870328078, 0.000000000000000000, -178.5580127018922383 ) ) ;
#12309=CARTESIAN_POINT ( 'NONE',  ( 6.000000000000000888, -6.507448562710137091E-15, -176.1636751345947971 ) ) ;
#12310=CARTESIAN_POINT ( 'NONE',  ( 0.000000000000000000, -5.999999999999991118, -101.5386751345947971 ) ) ;
#12311=CARTESIAN_POINT ( 'NONE',  ( -6.350852961085760029, -1.281975124255709124E-13, -113.6249999999999858 ) ) ;
#12312=CARTESIAN_POINT ( 'NONE',  ( -5.999999999999919176, 1.607695154586804565, -83.98066243270260145 ) ) ;
#12313=EDGE_CURVE ( 'NONE', #2458, #19518, #24099, .T. ) ;
#12314=CARTESIAN_POINT ( 'NONE',  ( -3.175426480542816510, -5.500000000000057732, -113.3750000000000568 ) ) ;
#12315=CARTESIAN_POINT ( 'NONE',  ( 6.000000000000000888, -1.607695154586752384, -131.2306624327026441 ) ) ;
#12319=CARTESIAN_POINT ( 'NONE',  ( 3.464101615137757051, -5.999999999999979572, -145.8363248654052029 ) ) ;
#12322=CARTESIAN_POINT ( 'NONE',  ( -5.999999999999956479, -1.607695154586745057, -126.7693375672974838 ) ) ;
#12323=CARTESIAN_POINT ( 'NONE',  ( 4.763139720814407951, 2.750000000000002665, -177.2500000000000284 ) ) ;
#12326=ORIENTED_EDGE ( 'NONE', *, *, #13916, .T. ) ;
#12327=CARTESIAN_POINT ( 'NONE',  ( -3.464101615137725076, 5.999999999999979572, -85.08632486540520290 ) ) ;
#12330=CARTESIAN_POINT ( 'NONE',  ( 3.608439182435180470, 6.249999999999982236, -131.6919872981078470 ) ) ;
#12332=CARTESIAN_POINT ( 'NONE',  ( -5.999999999999956479, -1.607695154586745057, -167.8466878364870354 ) ) ;
#12335=VERTEX_POINT ( 'NONE', #8573 ) ;
#12338=DIRECTION ( 'NONE',  ( -7.147005652999508048E-36, 5.642372883946980038E-36, 1.000000000000000000 ) ) ;
#12339=CARTESIAN_POINT ( 'NONE',  ( 6.000000000000000888, -1.859271017917181981E-14, -114.0863248654052029 ) ) ;
#12341=B_SPLINE_CURVE_WITH_KNOTS ( 'NONE', 3,
 ( #13011, #8831, #20496, #20206, #6207, #15783, #27534, #27086, #1283, #1749, #1444, #17920, #8356, #29389, #15934, #22808, #10697, #3886, #24936, #20659, #6511, #25229, #13174, #20043, #22659, #24637, #11148, #18070, #22512, #15312, #4200, #29556, #13617, #15627, #3583, #25089, #4045, #22964 ),
 .UNSPECIFIED., .F., .F.,
 ( 4, 2, 2, 2, 2, 2, 2, 2, 2, 2, 2, 2, 2, 2, 2, 2, 2, 2, 4 ),
 ( 0.01915730813553680537, 0.01975454893833630127, 0.02035178974113580064, 0.02154627134673479244, 0.02274075295233378424, 0.02393523455793277604, 0.02512971616353176785, 0.02632419776913075965, 0.02751867937472975145, 0.02871316098032874325, 0.02990764258592773506, 0.03110212419152672686, 0.03229660579712571866, 0.03349108740272471046, 0.03468556900832370227, 0.03528280981112319470, 0.03588005061392268713, 0.03707453221952168587, 0.03826901382512067074 ),
 .UNSPECIFIED. ) ;
#12343=CARTESIAN_POINT ( 'NONE',  ( -3.175426480542816510, -5.500000000000057732, -140.3750000000000568 ) ) ;
#12345=DIRECTION ( 'NONE',  ( -7.147005652999508048E-36, 5.642372883946980038E-36, 1.000000000000000000 ) ) ;
#12347=( BOUNDED_CURVE ( )  B_SPLINE_CURVE ( 2, ( #8012, #10495, #12522, #12976, #3392, #10340, #17420, #804, #3699 ),
 .UNSPECIFIED., .F., .F. ) 
 B_SPLINE_CURVE_WITH_KNOTS ( ( 3, 2, 2, 2, 3 ),
 ( 0.03611111111111109384, 0.03703703703703709049, 0.03888888888888886175, 0.04074074074074074403, 0.04166666666666674068 ),
 .UNSPECIFIED. ) 
 CURVE ( )  GEOMETRIC_REPRESENTATION_ITEM ( )  RATIONAL_B_SPLINE_CURVE ( ( 0.9330127018922194093, 0.9330127018922154125, 1.000000000000000000, 0.8660254037844388186, 1.000000000000000000, 0.8660254037844388186, 1.000000000000000000, 0.9330127018922154125, 0.9330127018922194093 ) ) 
 REPRESENTATION_ITEM ( '' )  );
#12348=CARTESIAN_POINT ( 'NONE',  ( -3.175426480542816066, -5.500000000000057732, -50.37500000000001421 ) ) ;
#12349=FACE_OUTER_BOUND ( 'NONE', #17494, .T. ) ;
#12350=CARTESIAN_POINT ( 'NONE',  ( -5.999999999999963585, 1.780251999655701777E-13, -102.8363248654052313 ) ) ;
#12354=CARTESIAN_POINT ( 'NONE',  ( 5.412658773652739619, 3.124999999999988898, -97.31698729810783277 ) ) ;
#12360=CARTESIAN_POINT ( 'NONE',  ( 4.763139720814407951, -2.749999999999988454, -128.0000000000000000 ) ) ;
#12361=ORIENTED_EDGE ( 'NONE', *, *, #22612, .F. ) ;
#12363=CARTESIAN_POINT ( 'NONE',  ( -2.775557561562891351E-14, -5.500000000000115463, -59.25000000000002842 ) ) ;
#12367=CARTESIAN_POINT ( 'NONE',  ( 5.999340830937940794, 9.219973438021412449, -24.59179872956898549 ) ) ;
#12369=CARTESIAN_POINT ( 'NONE',  ( 5.412658773652739619, 3.124999999999988898, -83.18301270189220986 ) ) ;
#12370=CARTESIAN_POINT ( 'NONE',  ( 6.000000000000000888, -1.859271017917181981E-14, -100.5863248654052171 ) ) ;
#12371=DIRECTION ( 'NONE',  ( -7.147005652999508048E-36, 5.642372883946980038E-36, 1.000000000000000000 ) ) ;
#12376=CARTESIAN_POINT ( 'NONE',  ( 0.000000000000000000, 5.499999999999991118, -136.5000000000000000 ) ) ;
#12379=CARTESIAN_POINT ( 'NONE',  ( 3.608439182435180470, -6.249999999999997335, -151.0580127018922951 ) ) ;
#12382=CARTESIAN_POINT ( 'NONE',  ( 0.000000000000000000, 5.499999999999991118, -67.50000000000000000 ) ) ;
#12383=CARTESIAN_POINT ( 'NONE',  ( 0.000000000000000000, 5.999999999999977796, -85.78867513459481131 ) ) ;
#12384=CARTESIAN_POINT ( 'NONE',  ( -4.763139720814407951, 2.749999999999946709, -59.75000000000002842 ) ) ;
#12385=( BOUNDED_CURVE ( )  B_SPLINE_CURVE ( 2, ( #4227, #22832, #23150, #15805, #4538, #27872, #13645, #6374, #18699 ),
 .UNSPECIFIED., .F., .F. ) 
 B_SPLINE_CURVE_WITH_KNOTS ( ( 3, 2, 2, 2, 3 ),
 ( 0.5361111111111110938, 0.5370370370370370905, 0.5388888888888888618, 0.5407407407407407440, 0.5416666666666667407 ),
 .UNSPECIFIED. ) 
 CURVE ( )  GEOMETRIC_REPRESENTATION_ITEM ( )  RATIONAL_B_SPLINE_CURVE ( ( 0.9330127018922194093, 0.9330127018922154125, 1.000000000000000000, 0.8660254037844388186, 1.000000000000000000, 0.8660254037844388186, 1.000000000000000000, 0.9330127018922154125, 0.9330127018922194093 ) ) 
 REPRESENTATION_ITEM ( '' )  );
#12386=CARTESIAN_POINT ( 'NONE',  ( 0.000000000000000000, 5.999999999999977796, -53.71132486540519579 ) ) ;
#12388=AXIS2_PLACEMENT_3D ( 'NONE', #20362, #20060, #27105 ) ;
#12391=VECTOR ( 'NONE', #10386, 1000.000000000000000 ) ;
#12392=DIRECTION ( 'NONE',  ( -7.147005652999508048E-36, 5.642372883946980038E-36, 1.000000000000000000 ) ) ;
#12394=ORIENTED_EDGE ( 'NONE', *, *, #7774, .T. ) ;
#12397=CARTESIAN_POINT ( 'NONE',  ( -5.196152422706601826, 2.999999999999975131, -63.96132486540523132 ) ) ;
#12398=CARTESIAN_POINT ( 'NONE',  ( 3.175426480543072749, 5.499999999999865885, -177.1250000000000284 ) ) ;
#12400=CARTESIAN_POINT ( 'NONE',  ( -5.412658773652684552, -3.125000000000099920, -153.5669872981077901 ) ) ;
#12402=CARTESIAN_POINT ( 'NONE',  ( 6.350852961086080661, -9.614813431917819062E-14, -79.87500000000001421 ) ) ;
#12403=EDGE_CURVE ( 'NONE', #3266, #22716, #14697, .T. ) ;
#12408=CARTESIAN_POINT ( 'NONE',  ( 0.000000000000000000, 5.499999999999991118, -168.0000000000000284 ) ) ;
#12410=CARTESIAN_POINT ( 'NONE',  ( 5.841785975170685319, -9.320713607846709436, -23.61690496628340341 ) ) ;
#12413=CARTESIAN_POINT ( 'NONE',  ( 0.000000000000000000, 5.499999999999991118, -166.4999999999999716 ) ) ;
#12414=CARTESIAN_POINT ( 'NONE',  ( -5.999999999999962697, 3.323446944526963260E-14, -161.3363248654052597 ) ) ;
#12415=CARTESIAN_POINT ( 'NONE',  ( 0.000000000000000000, 5.499999999999991118, -150.0000000000000284 ) ) ;
#12417=CARTESIAN_POINT ( 'NONE',  ( 6.350852961086080661, -9.614813431917819062E-14, -94.87500000000001421 ) ) ;
#12419=CARTESIAN_POINT ( 'NONE',  ( -3.175426480542816510, 5.499999999999865885, -88.37500000000000000 ) ) ;
#12421=CARTESIAN_POINT ( 'NONE',  ( -5.999999999999919176, 1.607695154586804565, -64.48066243270261566 ) ) ;
#12428=FACE_OUTER_BOUND ( 'NONE', #21178, .T. ) ;
#12429=CARTESIAN_POINT ( 'NONE',  ( -5.999999999999971578, 1.607695154586715303, -80.40331216351302146 ) ) ;
#12434=CARTESIAN_POINT ( 'NONE',  ( -4.763139720814407951, 2.749999999999946709, -103.2500000000000142 ) ) ;
#12437=CARTESIAN_POINT ( 'NONE',  ( 3.608439182435180470, -6.249999999999997335, -119.5580127018922525 ) ) ;
#12439=CARTESIAN_POINT ( 'NONE',  ( 4.763139720814407951, -2.749999999999988454, -152.0000000000000284 ) ) ;
#12441=CARTESIAN_POINT ( 'NONE',  ( 5.412658773652739619, 3.124999999999988898, -157.3169872981078470 ) ) ;
#12444=CARTESIAN_POINT ( 'NONE',  ( -5.412658773652684552, -3.125000000000099920, -56.93301270189221697 ) ) ;
#12450=CARTESIAN_POINT ( 'NONE',  ( 0.000000000000000000, 0.000000000000000000, 0.000000000000000000 ) ) ;
#12453=CARTESIAN_POINT ( 'NONE',  ( 5.412658773652739619, 3.124999999999988898, -168.6830127018922383 ) ) ;
#12456=CARTESIAN_POINT ( 'NONE',  ( -4.763139720814407951, 2.749999999999946709, -115.2500000000000142 ) ) ;
#12458=CARTESIAN_POINT ( 'NONE',  ( -6.350852961085760029, -1.281975124255709124E-13, -112.1249999999999858 ) ) ;
#12460=DIRECTION ( 'NONE',  ( -7.147005652999508048E-36, 5.642372883946980038E-36, 1.000000000000000000 ) ) ;
#12462=ORIENTED_EDGE ( 'NONE', *, *, #16059, .F. ) ;
#12466=AXIS2_PLACEMENT_3D ( 'NONE', #5079, #11915, #331 ) ;
#12467=CARTESIAN_POINT ( 'NONE',  ( 5.999999999999999112, 2.951592740943527306E-14, -153.0863248654052313 ) ) ;
#12470=ADVANCED_FACE ( 'NONE', ( #28058 ), #23923, .T. ) ;
#12472=ADVANCED_FACE ( 'NONE', ( #12285 ), #5308, .T. ) ;
#12473=CARTESIAN_POINT ( 'NONE',  ( -5.999999999999963585, -1.487416814333745711E-14, -166.4136751345948539 ) ) ;
#12476=( BOUNDED_CURVE ( )  B_SPLINE_CURVE ( 2, ( #3681, #13116, #22453, #30372, #15986, #9183, #1387, #4410, #27587 ),
 .UNSPECIFIED., .F., .T. ) 
 B_SPLINE_CURVE_WITH_KNOTS ( ( 3, 2, 2, 2, 3 ),
 ( 0.6194444444444444642, 0.6203703703703703498, 0.6222222222222222321, 0.6240740740740740033, 0.6250000000000000000 ),
 .UNSPECIFIED. ) 
 CURVE ( )  GEOMETRIC_REPRESENTATION_ITEM ( )  RATIONAL_B_SPLINE_CURVE ( ( 0.9330127018922194093, 0.9330127018922234061, 1.000000000000000000, 0.8660254037844388186, 1.000000000000000000, 0.8660254037844388186, 1.000000000000000000, 0.9330127018922194093, 0.9330127018922194093 ) ) 
 REPRESENTATION_ITEM ( '' )  );
#12477=ORIENTED_EDGE ( 'NONE', *, *, #18669, .F. ) ;
#12481=( BOUNDED_CURVE ( )  B_SPLINE_CURVE ( 2, ( #21410, #25855, #14231, #23567, #343, #21258, #2502, #198, #9583 ),
 .UNSPECIFIED., .F., .T. ) 
 B_SPLINE_CURVE_WITH_KNOTS ( ( 3, 2, 2, 2, 3 ),
 ( 0.8638888888888889284, 0.8648148148148148140, 0.8666666666666666963, 0.8685185185185184675, 0.8694444444444444642 ),
 .UNSPECIFIED. ) 
 CURVE ( )  GEOMETRIC_REPRESENTATION_ITEM ( )  RATIONAL_B_SPLINE_CURVE ( ( 0.9330127018922194093, 0.9330127018922234061, 1.000000000000000000, 0.8660254037844388186, 1.000000000000000000, 0.8660254037844388186, 1.000000000000000000, 0.9330127018922154125, 0.9330127018922194093 ) ) 
 REPRESENTATION_ITEM ( '' )  );
#12482=EDGE_CURVE ( 'NONE', #891, #14585, #562, .T. ) ;
#12484=CARTESIAN_POINT ( 'NONE',  ( 2.775557561562891351E-14, -6.250000000000061284, -133.8169872981078186 ) ) ;
#12486=CARTESIAN_POINT ( 'NONE',  ( 6.000000000000052403, 1.607695154586625819, -175.5193375672974412 ) ) ;
#12487=DIRECTION ( 'NONE',  ( -7.147005652999508048E-36, 5.642372883946980038E-36, 1.000000000000000000 ) ) ;
#12488=EDGE_LOOP ( 'NONE', ( #27422, #22960, #24997 ) ) ;
#12490=LINE ( 'NONE', #21828, #8313 ) ;
#12491=CARTESIAN_POINT ( 'NONE',  ( -5.999999999999956479, -1.607695154586745057, -92.26933756729744118 ) ) ;
#12496=CARTESIAN_POINT ( 'NONE',  ( 0.000000000000000000, -5.999999999999991118, -128.5386751345948255 ) ) ;
#12497=CARTESIAN_POINT ( 'NONE',  ( 5.999999999999949374, 1.607695154586804565, -56.09668783648702828 ) ) ;
#12498=CARTESIAN_POINT ( 'NONE',  ( -3.464101615137757051, -5.999999999999979572, -115.1636751345948255 ) ) ;
#12499=CARTESIAN_POINT ( 'NONE',  ( -2.775557561562891351E-14, -5.500000000000115463, -140.2500000000000000 ) ) ;
#12502=CARTESIAN_POINT ( 'NONE',  ( -2.775557561562891351E-14, -5.500000000000115463, -50.25000000000001421 ) ) ;
#12503=CARTESIAN_POINT ( 'NONE',  ( 6.000000000000026645, -1.607695154586707753, -132.7306624327025872 ) ) ;
#12504=VERTEX_POINT ( 'NONE', #2710 ) ;
#12508=CARTESIAN_POINT ( 'NONE',  ( 5.412658773652739619, 3.124999999999988898, -98.81698729810783277 ) ) ;
#12514=ADVANCED_FACE ( 'NONE', ( #9652 ), #28508, .T. ) ;
#12515=CARTESIAN_POINT ( 'NONE',  ( 4.763139720814407951, -2.749999999999988454, -131.0000000000000000 ) ) ;
#12516=EDGE_CURVE ( 'NONE', #137, #13496, #21180, .T. ) ;
#12517=ORIENTED_EDGE ( 'NONE', *, *, #1712, .T. ) ;
#12518=ORIENTED_EDGE ( 'NONE', *, *, #19056, .F. ) ;
#12519=CARTESIAN_POINT ( 'NONE',  ( -5.196152422706573404, -3.000000000000002665, -83.21132486540521711 ) ) ;
#12520=CARTESIAN_POINT ( 'NONE',  ( 3.175426480543072749, -5.500000000000105693, -54.62500000000003553 ) ) ;
#12522=CARTESIAN_POINT ( 'NONE',  ( 5.196152422706629359, -2.999999999999988898, -51.21132486540525264 ) ) ;
#12523=CARTESIAN_POINT ( 'NONE',  ( 2.687256737965279640, 10.66819377212462960, -30.36813770228161502 ) ) ;
#12524=CARTESIAN_POINT ( 'NONE',  ( -5.412658773652739619, 3.124999999999975131, -73.68301270189225249 ) ) ;
#12525=CARTESIAN_POINT ( 'NONE',  ( 0.000000000000000000, 0.000000000000000000, -14.99152654425661702 ) ) ;
#12529=CARTESIAN_POINT ( 'NONE',  ( 6.350852961086080661, -9.614813431917819062E-14, -139.8750000000000568 ) ) ;
#12533=CARTESIAN_POINT ( 'NONE',  ( 4.763139720814407951, -2.749999999999988454, -72.50000000000001421 ) ) ;
#12534=CARTESIAN_POINT ( 'NONE',  ( -4.763139720814407951, -2.750000000000016431, -59.50000000000000000 ) ) ;
#12535=EDGE_LOOP ( 'NONE', ( #12107, #9846, #3014, #28664 ) ) ;
#12538=CARTESIAN_POINT ( 'NONE',  ( 0.000000000000000000, 5.999999999999977796, -44.99152654425658682 ) ) ;
#12540=ADVANCED_FACE ( 'NONE', ( #14151 ), #23489, .T. ) ;
#12545=EDGE_CURVE ( 'NONE', #21702, #18178, #23777, .T. ) ;
#12547=CARTESIAN_POINT ( 'NONE',  ( 4.763139720814407951, -2.749999999999988454, -176.0000000000000568 ) ) ;
#12549=ORIENTED_EDGE ( 'NONE', *, *, #27826, .F. ) ;
#12551=CARTESIAN_POINT ( 'NONE',  ( -2.775557561562891351E-14, -5.500000000000115463, -81.74999999999998579 ) ) ;
#12552=ORIENTED_EDGE ( 'NONE', *, *, #21365, .F. ) ;
#12556=CARTESIAN_POINT ( 'NONE',  ( 3.675482141847883799, -10.37335300580274300, -20.24150316489820511 ) ) ;
#12557=CARTESIAN_POINT ( 'NONE',  ( -3.464101615137757051, -5.999999999999979572, -59.08632486540519579 ) ) ;
#12558=( BOUNDED_CURVE ( )  B_SPLINE_CURVE ( 2, ( #10760, #8254, #5794, #15209, #24852, #13228, #3341, #12767, #1189 ),
 .UNSPECIFIED., .F., .F. ) 
 B_SPLINE_CURVE_WITH_KNOTS ( ( 3, 2, 2, 2, 3 ),
 ( 0.1861111111111111160, 0.1870370370370370294, 0.1888888888888888840, 0.1907407407407407385, 0.1916666666666666519 ),
 .UNSPECIFIED. ) 
 CURVE ( )  GEOMETRIC_REPRESENTATION_ITEM ( )  RATIONAL_B_SPLINE_CURVE ( ( 0.9330127018922194093, 0.9330127018922204085, 1.000000000000000000, 0.8660254037844388186, 1.000000000000000000, 0.8660254037844388186, 1.000000000000000000, 0.9330127018922205195, 0.9330127018922196314 ) ) 
 REPRESENTATION_ITEM ( '' )  );
#12559=CARTESIAN_POINT ( 'NONE',  ( -6.350852961085760029, -1.281975124255709124E-13, -163.1249999999999716 ) ) ;
#12561=CARTESIAN_POINT ( 'NONE',  ( 4.763139720814407951, -2.749999999999988454, -144.5000000000000284 ) ) ;
#12564=AXIS2_PLACEMENT_3D ( 'NONE', #17939, #17629, #24657 ) ;
#12565=CARTESIAN_POINT ( 'NONE',  ( -2.775557561562891351E-14, -5.500000000000115463, -96.75000000000000000 ) ) ;
#12567=CYLINDRICAL_SURFACE ( 'NONE', #10356, 6.000000000000000888 ) ;
#12568=CARTESIAN_POINT ( 'NONE',  ( 4.763139720814407951, 2.750000000000002665, -78.25000000000004263 ) ) ;
#12570=FACE_OUTER_BOUND ( 'NONE', #5015, .T. ) ;
#12577=ORIENTED_EDGE ( 'NONE', *, *, #4283, .F. ) ;
#12581=CARTESIAN_POINT ( 'NONE',  ( -5.196152422706601826, 2.999999999999975131, -80.46132486540524553 ) ) ;
#12583=ORIENTED_EDGE ( 'NONE', *, *, #7532, .T. ) ;
#12586=CARTESIAN_POINT ( 'NONE',  ( 3.175426480543072749, 5.499999999999865885, -108.1250000000000284 ) ) ;
#12587=CARTESIAN_POINT ( 'NONE',  ( -7.216878364870328078, 0.000000000000000000, -124.5580127018922241 ) ) ;
#12589=CARTESIAN_POINT ( 'NONE',  ( -5.196152422706573404, -3.000000000000002665, -68.78867513459485394 ) ) ;
#12590=CARTESIAN_POINT ( 'NONE',  ( 3.608439182435180470, 6.249999999999982236, -163.1919872981078470 ) ) ;
#12593=CARTESIAN_POINT ( 'NONE',  ( 3.608439182435180470, -6.249999999999997335, -56.55801270189220986 ) ) ;
#12595=CARTESIAN_POINT ( 'NONE',  ( -4.380587382795368967, 10.09118633559235612, -20.89546095134608805 ) ) ;
#12597=CARTESIAN_POINT ( 'NONE',  ( 3.175426480543072749, 5.499999999999865885, -171.1250000000000000 ) ) ;
#12600=CARTESIAN_POINT ( 'NONE',  ( 0.000000000000000000, 5.999999999999977796, -100.2113248654052313 ) ) ;
#12601=CARTESIAN_POINT ( 'NONE',  ( -3.608439182435052128, -6.250000000000110134, -170.8080127018922383 ) ) ;
#12604=CARTESIAN_POINT ( 'NONE',  ( 4.763139720814407951, 2.750000000000002665, -117.2500000000000142 ) ) ;
#12605=CARTESIAN_POINT ( 'NONE',  ( -2.910268709469104432E-14, -11.00000000000000000, -14.99152654425661702 ) ) ;
#12606=AXIS2_PLACEMENT_3D ( 'NONE', #11473, #20970, #6968 ) ;
#12607=CARTESIAN_POINT ( 'NONE',  ( -4.763139720814407951, -2.750000000000016431, -103.0000000000000426 ) ) ;
#12608=CARTESIAN_POINT ( 'NONE',  ( -5.999999999999944933, 1.607695154586759934, -142.4806624327026441 ) ) ;
#12611=AXIS2_PLACEMENT_3D ( 'NONE', #19168, #9640, #14713 ) ;
#12616=CARTESIAN_POINT ( 'NONE',  ( 3.464101615137757051, -5.999999999999979572, -126.9136751345948113 ) ) ;
#12618=CARTESIAN_POINT ( 'NONE',  ( 5.412658773652712085, -3.125000000000086153, -84.06698729810780435 ) ) ;
#12623=CARTESIAN_POINT ( 'NONE',  ( 5.412658773652712085, -3.125000000000086153, -130.5669872981078470 ) ) ;
#12626=FACE_OUTER_BOUND ( 'NONE', #19717, .T. ) ;
#12627=VERTEX_POINT ( 'NONE', #13039 ) ;
#12629=CARTESIAN_POINT ( 'NONE',  ( 3.464101615137852974, 5.999999999999884537, -56.83632486540519579 ) ) ;
#12633=AXIS2_PLACEMENT_3D ( 'NONE', #26445, #25859, #5399 ) ;
#12634=EDGE_CURVE ( 'NONE', #16367, #16120, #4078, .T. ) ;
#12637=CARTESIAN_POINT ( 'NONE',  ( 5.999999999999974243, 1.607695154586759934, -128.0966878364870638 ) ) ;
#12638=CARTESIAN_POINT ( 'NONE',  ( 3.175426480543072749, 5.499999999999865885, -136.6250000000000568 ) ) ;
#12644=CARTESIAN_POINT ( 'NONE',  ( 4.763139720814407951, 2.750000000000002665, -49.75000000000001421 ) ) ;
#12647=( BOUNDED_CURVE ( )  B_SPLINE_CURVE ( 2, ( #18187, #27506, #25205, #22933, #4328, #1873, #11276, #20630, #13746 ),
 .UNSPECIFIED., .F., .F. ) 
 B_SPLINE_CURVE_WITH_KNOTS ( ( 3, 2, 2, 2, 3 ),
 ( 0.1916666666666666519, 0.1925925925925925930, 0.1944444444444444475, 0.1962962962962963021, 0.1972222222222222432 ),
 .UNSPECIFIED. ) 
 CURVE ( )  GEOMETRIC_REPRESENTATION_ITEM ( )  RATIONAL_B_SPLINE_CURVE ( ( 0.9330127018922196314, 0.9330127018922185211, 1.000000000000000000, 0.8660254037844388186, 1.000000000000000000, 0.8660254037844388186, 1.000000000000000000, 0.9330127018922184101, 0.9330127018922194093 ) ) 
 REPRESENTATION_ITEM ( '' )  );
#12648=ADVANCED_FACE ( 'NONE', ( #5912 ), #719, .T. ) ;
#12649=ORIENTED_EDGE ( 'NONE', *, *, #21742, .F. ) ;
#12651=CARTESIAN_POINT ( 'NONE',  ( -5.999999999999962697, 3.323446944526963891E-14, -158.9136751345948255 ) ) ;
#12652=CARTESIAN_POINT ( 'NONE',  ( 2.775557561562891351E-14, -6.250000000000061284, -96.31698729810783277 ) ) ;
#12653=DIRECTION ( 'NONE',  ( 1.000000000000000000, -5.551115123125773458E-17, -1.260129944081490338E-35 ) ) ;
#12663=CARTESIAN_POINT ( 'NONE',  ( 0.000000000000000000, -5.999999999999991118, -138.4613248654051745 ) ) ;
#12664=CARTESIAN_POINT ( 'NONE',  ( -6.350852961085760029, -1.281975124255709124E-13, -61.12500000000000711 ) ) ;
#12665=CARTESIAN_POINT ( 'NONE',  ( 5.999999999999949374, 1.607695154586804565, -69.59668783648703538 ) ) ;
#12667=CARTESIAN_POINT ( 'NONE',  ( -5.999999999999971578, 1.607695154586715303, -67.48066243270260145 ) ) ;
#12668=CARTESIAN_POINT ( 'NONE',  ( -7.216878364870328078, 0.000000000000000000, -78.05801270189225249 ) ) ;
#12672=DIRECTION ( 'NONE',  ( 0.7071067811865477948, 4.734329415645503570E-17, -0.7071067811865472397 ) ) ;
#12677=CARTESIAN_POINT ( 'NONE',  ( 3.175426480543072749, 5.499999999999865885, -142.6250000000000000 ) ) ;
#12678=CARTESIAN_POINT ( 'NONE',  ( 6.000000000000000888, 1.743066579297358182E-13, -87.66367513459482552 ) ) ;
#12679=CARTESIAN_POINT ( 'NONE',  ( 2.775557561562891351E-14, 6.250000000000033751, -147.4330127018922383 ) ) ;
#12680=CARTESIAN_POINT ( 'NONE',  ( 0.000000000000000000, 0.000000000000000000, 0.000000000000000000 ) ) ;
#12683=CARTESIAN_POINT ( 'NONE',  ( 6.350852961086080661, -9.614813431917819062E-14, -72.37500000000000000 ) ) ;
#12685=EDGE_CURVE ( 'NONE', #8576, #26834, #30381, .T. ) ;
#12686=CARTESIAN_POINT ( 'NONE',  ( -4.763139720814407951, 2.749999999999946709, -58.25000000000002132 ) ) ;
#12690=CARTESIAN_POINT ( 'NONE',  ( 5.999999999999949374, 1.607695154586804565, -98.09668783648704959 ) ) ;
#12699=CARTESIAN_POINT ( 'NONE',  ( 0.000000000000000000, 5.499999999999991118, -177.0000000000000568 ) ) ;
#12701=CARTESIAN_POINT ( 'NONE',  ( 3.608439182435180470, -6.249999999999997335, -147.1919872981078470 ) ) ;
#12703=CARTESIAN_POINT ( 'NONE',  ( 3.175426480543072749, 5.499999999999865885, -82.62500000000004263 ) ) ;
#12704=CARTESIAN_POINT ( 'NONE',  ( 3.608439182435180470, -6.249999999999997335, -92.55801270189225249 ) ) ;
#12709=CARTESIAN_POINT ( 'NONE',  ( -3.464101615137757051, -5.999999999999979572, -91.16367513459485394 ) ) ;
#12711=CARTESIAN_POINT ( 'NONE',  ( -4.763139720814407951, -2.750000000000016431, -161.5000000000000284 ) ) ;
#12712=CARTESIAN_POINT ( 'NONE',  ( 6.000000000000000888, -3.330669073875464691E-16, -7.560779664488942560E-35 ) ) ;
#12713=CARTESIAN_POINT ( 'NONE',  ( 6.350852961086080661, -9.614813431917819062E-14, -145.8750000000000284 ) ) ;
#12714=FACE_OUTER_BOUND ( 'NONE', #23380, .T. ) ;
#12715=CARTESIAN_POINT ( 'NONE',  ( 5.196152422706629359, -2.999999999999988898, -103.7113248654052455 ) ) ;
#12716=CARTESIAN_POINT ( 'NONE',  ( -4.763139720814407951, -2.750000000000016431, -95.50000000000002842 ) ) ;
#12719=EDGE_CURVE ( 'NONE', #11022, #24590, #934, .T. ) ;
#12720=CARTESIAN_POINT ( 'NONE',  ( 4.763139720814407951, 2.750000000000002665, -82.74999999999998579 ) ) ;
#12724=CARTESIAN_POINT ( 'NONE',  ( -5.999999999999919176, 1.607695154586804565, -155.4033121635129930 ) ) ;
#12725=CYLINDRICAL_SURFACE ( 'NONE', #5045, 6.000000000000000888 ) ;
#12726=CARTESIAN_POINT ( 'NONE',  ( 3.464101615137852974, 5.999999999999884537, -72.41367513459482552 ) ) ;
#12727=CARTESIAN_POINT ( 'NONE',  ( 6.000000000000000888, -1.859271017917181981E-14, -63.66367513459483973 ) ) ;
#12728=ORIENTED_EDGE ( 'NONE', *, *, #17846, .F. ) ;
#12729=CARTESIAN_POINT ( 'NONE',  ( 5.196152422706629359, 3.000000000000002665, -91.46132486540525974 ) ) ;
#12731=CARTESIAN_POINT ( 'NONE',  ( -3.464101615137725076, 5.999999999999979572, -82.66367513459479710 ) ) ;
#12733=CARTESIAN_POINT ( 'NONE',  ( -3.464101615137757051, -5.999999999999979572, -116.0863248654052171 ) ) ;
#12734=VERTEX_POINT ( 'NONE', #12884 ) ;
#12735=ORIENTED_EDGE ( 'NONE', *, *, #1467, .F. ) ;
#12736=CARTESIAN_POINT ( 'NONE',  ( 3.175426480543072749, 5.499999999999865885, -105.1250000000000284 ) ) ;
#12737=( BOUNDED_CURVE ( )  B_SPLINE_CURVE ( 2, ( #10346, #19707, #29052, #10197, #3552, #24447, #661, #22009, #17577 ),
 .UNSPECIFIED., .F., .T. ) 
 B_SPLINE_CURVE_WITH_KNOTS ( ( 3, 2, 2, 2, 3 ),
 ( 0.7527777777777777679, 0.7537037037037036535, 0.7555555555555555358, 0.7574074074074074181, 0.7583333333333333037 ),
 .UNSPECIFIED. ) 
 CURVE ( )  GEOMETRIC_REPRESENTATION_ITEM ( )  RATIONAL_B_SPLINE_CURVE ( ( 0.9330127018922194093, 0.9330127018922194093, 1.000000000000000000, 0.8660254037844388186, 1.000000000000000000, 0.8660254037844388186, 1.000000000000000000, 0.9330127018922234061, 0.9330127018922194093 ) ) 
 REPRESENTATION_ITEM ( '' )  );
#12738=CARTESIAN_POINT ( 'NONE',  ( -3.608439182435052128, -6.250000000000110134, -118.3080127018922383 ) ) ;
#12739=VERTEX_POINT ( 'NONE', #22221 ) ;
#12740=CARTESIAN_POINT ( 'NONE',  ( 7.216878364870455975, -6.409875621278545621E-14, -163.4419872981078186 ) ) ;
#12744=CARTESIAN_POINT ( 'NONE',  ( 3.608439182435180470, 6.249999999999982236, -59.05801270189222407 ) ) ;
#12746=ORIENTED_EDGE ( 'NONE', *, *, #13140, .T. ) ;
#12748=EDGE_CURVE ( 'NONE', #18178, #29147, #9400, .T. ) ;
#12749=CARTESIAN_POINT ( 'NONE',  ( -5.792970643771982786, 9.351264793308498469, -23.42496030963406284 ) ) ;
#12750=CYLINDRICAL_SURFACE ( 'NONE', #5941, 6.000000000000000888 ) ;
#12751=CARTESIAN_POINT ( 'NONE',  ( -4.763139720814407951, -2.750000000000016431, -169.0000000000000284 ) ) ;
#12753=CARTESIAN_POINT ( 'NONE',  ( -3.464101615137757051, -5.999999999999979572, -113.0863248654051745 ) ) ;
#12754=CARTESIAN_POINT ( 'NONE',  ( -3.608439182435115633, 6.249999999999965361, -166.8080127018922951 ) ) ;
#12755=CYLINDRICAL_SURFACE ( 'NONE', #16612, 6.000000000000000888 ) ;
#12757=CARTESIAN_POINT ( 'NONE',  ( 4.763139720814407951, -2.749999999999988454, -112.9999999999999858 ) ) ;
#12758=CARTESIAN_POINT ( 'NONE',  ( 4.763139720814407951, 2.750000000000002665, -106.7500000000000142 ) ) ;
#12764=LINE ( 'NONE', #1183, #18244 ) ;
#12765=LINE ( 'NONE', #4060, #18891 ) ;
#12766=ORIENTED_EDGE ( 'NONE', *, *, #29373, .F. ) ;
#12767=CARTESIAN_POINT ( 'NONE',  ( -5.999999999999957367, 1.607695154586737507, -155.9806624327026157 ) ) ;
#12768=CARTESIAN_POINT ( 'NONE',  ( 3.608439182435180470, -6.249999999999997335, -84.19198729810781856 ) ) ;
#12769=VECTOR ( 'NONE', #6929, 1000.000000000000000 ) ;
#12770=DIRECTION ( 'NONE',  ( -7.147005652999508048E-36, 5.642372883946980038E-36, 1.000000000000000000 ) ) ;
#12772=DIRECTION ( 'NONE',  ( 1.000000000000000000, -5.551115123125773458E-17, -1.260129944081490338E-35 ) ) ;
#12773=ORIENTED_EDGE ( 'NONE', *, *, #17425, .T. ) ;
#12774=ORIENTED_EDGE ( 'NONE', *, *, #25430, .F. ) ;
#12777=CARTESIAN_POINT ( 'NONE',  ( -3.608439182435052128, -6.250000000000110134, -132.4419872981078470 ) ) ;
#12779=CARTESIAN_POINT ( 'NONE',  ( 5.196152422706629359, 3.000000000000002665, -50.03867513459481131 ) ) ;
#12780=VERTEX_POINT ( 'NONE', #21515 ) ;
#12782=CARTESIAN_POINT ( 'NONE',  ( 5.196152422706629359, 3.000000000000002665, -135.5386751345948255 ) ) ;
#12784=ADVANCED_FACE ( 'NONE', ( #297 ), #14752, .F. ) ;
#12785=LINE ( 'NONE', #7679, #29897 ) ;
#12786=CARTESIAN_POINT ( 'NONE',  ( 6.000000000000000888, -1.859271017917181981E-14, -93.08632486540523132 ) ) ;
#12788=CARTESIAN_POINT ( 'NONE',  ( 7.216878364870455975, -6.409875621278545621E-14, -67.44198729810779014 ) ) ;
#12789=CARTESIAN_POINT ( 'NONE',  ( 2.775557561562891351E-14, -6.250000000000061284, -51.31698729810785409 ) ) ;
#12791=CARTESIAN_POINT ( 'NONE',  ( 3.464101615137757051, -5.999999999999979572, -128.4136751345948255 ) ) ;
#12795=CARTESIAN_POINT ( 'NONE',  ( 6.350852961086080661, -9.614813431917819062E-14, -132.3750000000000284 ) ) ;
#12799=CARTESIAN_POINT ( 'NONE',  ( 3.464101615137852974, 5.999999999999884537, -119.8363248654051603 ) ) ;
#12800=LINE ( 'NONE', #17552, #28969 ) ;
#12806=CARTESIAN_POINT ( 'NONE',  ( 5.412658773652712085, -3.125000000000086153, -97.56698729810780435 ) ) ;
#12807=CARTESIAN_POINT ( 'NONE',  ( 6.000000000000000888, -1.859271017917181981E-14, -173.1636751345948539 ) ) ;
#12811=FACE_OUTER_BOUND ( 'NONE', #17230, .T. ) ;
#12812=EDGE_CURVE ( 'NONE', #26042, #2934, #9684, .T. ) ;
#12813=VECTOR ( 'NONE', #19152, 1000.000000000000000 ) ;
#12816=CARTESIAN_POINT ( 'NONE',  ( 0.000000000000000000, 5.499999999999991118, -49.49999999999998579 ) ) ;
#12818=CARTESIAN_POINT ( 'NONE',  ( -5.196152422706573404, -3.000000000000002665, -62.78867513459485394 ) ) ;
#12819=CARTESIAN_POINT ( 'NONE',  ( 2.775557561562891351E-14, -6.250000000000061284, -73.18301270189225249 ) ) ;
#12820=EDGE_CURVE ( 'NONE', #9948, #9152, #4754, .T. ) ;
#12821=CARTESIAN_POINT ( 'NONE',  ( -3.464101615137757051, -5.999999999999979572, -173.0863248654051745 ) ) ;
#12823=CARTESIAN_POINT ( 'NONE',  ( 0.000000000000000000, 0.000000000000000000, 0.000000000000000000 ) ) ;
#12825=( BOUNDED_CURVE ( )  B_SPLINE_CURVE ( 2, ( #9980, #15043, #28985, #21512, #26391, #17208, #26536, #12315, #23805 ),
 .UNSPECIFIED., .F., .T. ) 
 B_SPLINE_CURVE_WITH_KNOTS ( ( 3, 2, 2, 2, 3 ),
 ( 0.3694444444444444087, 0.3703703703703703498, 0.3722222222222222321, 0.3740740740740740589, 0.3750000000000000000 ),
 .UNSPECIFIED. ) 
 CURVE ( )  GEOMETRIC_REPRESENTATION_ITEM ( )  RATIONAL_B_SPLINE_CURVE ( ( 0.9330127018922194093, 0.9330127018922174109, 1.000000000000000000, 0.8660254037844388186, 1.000000000000000000, 0.8660254037844388186, 1.000000000000000000, 0.9330127018922194093, 0.9330127018922194093 ) ) 
 REPRESENTATION_ITEM ( '' )  );
#12826=CARTESIAN_POINT ( 'NONE',  ( 3.175426480543072749, -5.500000000000105693, -131.1250000000000284 ) ) ;
#12830=CARTESIAN_POINT ( 'NONE',  ( -3.175426480542816066, -5.500000000000057732, -60.87500000000000000 ) ) ;
#12831=CARTESIAN_POINT ( 'NONE',  ( 0.000000000000000000, 5.499999999999991118, -57.00000000000004974 ) ) ;
#12834=CARTESIAN_POINT ( 'NONE',  ( -6.000000000000000888, 1.067854986875958443E-15, 7.560779664488942560E-35 ) ) ;
#12837=FACE_OUTER_BOUND ( 'NONE', #1228, .T. ) ;
#12840=VERTEX_POINT ( 'NONE', #30408 ) ;
#12844=VERTEX_POINT ( 'NONE', #18769 ) ;
#12845=EDGE_CURVE ( 'NONE', #18063, #11022, #2315, .T. ) ;
#12846=CARTESIAN_POINT ( 'NONE',  ( 4.763139720814407951, -2.749999999999988454, -146.0000000000000284 ) ) ;
#12849=CARTESIAN_POINT ( 'NONE',  ( -5.412658773652739619, 3.124999999999975131, -144.8169872981078186 ) ) ;
#12850=CARTESIAN_POINT ( 'NONE',  ( -3.175426480542816510, -5.500000000000057732, -78.87500000000002842 ) ) ;
#12851=VECTOR ( 'NONE', #21720, 1000.000000000000000 ) ;
#12854=CARTESIAN_POINT ( 'NONE',  ( -3.608439182435052128, -6.250000000000110134, -92.80801270189226670 ) ) ;
#12857=CARTESIAN_POINT ( 'NONE',  ( 3.464101615137852974, 5.999999999999884537, -175.9136751345948539 ) ) ;
#12860=CARTESIAN_POINT ( 'NONE',  ( -5.999999999999963585, 8.134310703387671600E-14, -115.4136751345948397 ) ) ;
#12863=CARTESIAN_POINT ( 'NONE',  ( -4.763139720814407951, 2.749999999999946709, -154.2500000000000000 ) ) ;
#12865=VECTOR ( 'NONE', #29798, 1000.000000000000000 ) ;
#12866=CARTESIAN_POINT ( 'NONE',  ( -4.763139720814407951, -2.750000000000016431, -143.5000000000000284 ) ) ;
#12867=CARTESIAN_POINT ( 'NONE',  ( 4.763139720814407951, 2.750000000000002665, -96.25000000000000000 ) ) ;
#12868=FACE_OUTER_BOUND ( 'NONE', #4908, .T. ) ;
#12869=CARTESIAN_POINT ( 'NONE',  ( 6.000000000000000888, -3.330669073875464691E-16, -7.560779664488942560E-35 ) ) ;
#12870=CARTESIAN_POINT ( 'NONE',  ( 4.763139720814407951, 2.750000000000002665, -79.74999999999998579 ) ) ;
#12873=CARTESIAN_POINT ( 'NONE',  ( -5.196152422706601826, 2.999999999999975131, -164.4613248654052029 ) ) ;
#12878=AXIS2_PLACEMENT_3D ( 'NONE', #14313, #17200, #23793 ) ;
#12880=FACE_OUTER_BOUND ( 'NONE', #5076, .T. ) ;
#12883=CARTESIAN_POINT ( 'NONE',  ( 5.196152422706629359, 3.000000000000002665, -73.46132486540524553 ) ) ;
#12884=CARTESIAN_POINT ( 'NONE',  ( -5.999999999999963585, 8.134310703387671600E-14, -119.9136751345948397 ) ) ;
#12886=EDGE_CURVE ( 'NONE', #4790, #27647, #2897, .T. ) ;
#12887=CYLINDRICAL_SURFACE ( 'NONE', #10582, 6.000000000000000888 ) ;
#12888=ORIENTED_EDGE ( 'NONE', *, *, #12313, .T. ) ;
#12891=CARTESIAN_POINT ( 'NONE',  ( 4.763139720814407951, -2.749999999999988454, -104.0000000000000426 ) ) ;
#12892=CARTESIAN_POINT ( 'NONE',  ( 3.464101615137757051, -5.999999999999979572, -89.41367513459483973 ) ) ;
#12894=EDGE_CURVE ( 'NONE', #11685, #11657, #26099, .T. ) ;
#12896=CARTESIAN_POINT ( 'NONE',  ( 3.464101615137852974, 5.999999999999884537, -140.8363248654051745 ) ) ;
#12898=CARTESIAN_POINT ( 'NONE',  ( 0.000000000000000000, 5.999999999999977796, -63.28867513459479710 ) ) ;
#12899=CARTESIAN_POINT ( 'NONE',  ( 5.412658773652712085, -3.125000000000086153, -54.93301270189221697 ) ) ;
#12901=CARTESIAN_POINT ( 'NONE',  ( -5.999999999999944933, 1.607695154586759934, -116.9806624327026299 ) ) ;
#12903=CARTESIAN_POINT ( 'NONE',  ( -6.000000000000007105, -1.607695154586655129, -62.26933756729742697 ) ) ;
#12905=CARTESIAN_POINT ( 'NONE',  ( -2.775557561562891351E-14, -5.500000000000115463, -167.2500000000000000 ) ) ;
#12907=CARTESIAN_POINT ( 'NONE',  ( -5.412658773652684552, -3.125000000000099920, -169.4330127018922667 ) ) ;
#12908=LINE ( 'NONE', #1030, #9202 ) ;
#12909=CARTESIAN_POINT ( 'NONE',  ( -2.775557561562891351E-14, -5.500000000000115463, -116.2500000000000142 ) ) ;
#12910=DIRECTION ( 'NONE',  ( -7.147005652999508048E-36, 5.642372883946980038E-36, 1.000000000000000000 ) ) ;
#12911=CARTESIAN_POINT ( 'NONE',  ( -6.350852961085760029, -1.281975124255709124E-13, -106.1250000000000142 ) ) ;
#12913=CARTESIAN_POINT ( 'NONE',  ( 6.000000000000000888, 1.743066579297358182E-13, -87.08632486540520290 ) ) ;
#12914=CARTESIAN_POINT ( 'NONE',  ( -5.999999999999963585, -1.487416814333745711E-14, -117.8363248654052313 ) ) ;
#12915=VERTEX_POINT ( 'NONE', #14473 ) ;
#12920=CARTESIAN_POINT ( 'NONE',  ( -2.775557561562891351E-14, -5.500000000000115463, -159.7500000000000568 ) ) ;
#12922=CARTESIAN_POINT ( 'NONE',  ( 5.412658773652739619, 3.124999999999988898, -77.81698729810781856 ) ) ;
#12923=EDGE_CURVE ( 'NONE', #22416, #10004, #17764, .T. ) ;
#12924=CARTESIAN_POINT ( 'NONE',  ( -5.999999999999963585, 8.134310703387671600E-14, -129.8363248654052313 ) ) ;
#12925=ORIENTED_EDGE ( 'NONE', *, *, #27026, .T. ) ;
#12926=DIRECTION ( 'NONE',  ( -7.147005652999508048E-36, 5.642372883946980038E-36, 1.000000000000000000 ) ) ;
#12927=( BOUNDED_CURVE ( )  B_SPLINE_CURVE ( 2, ( #4447, #30100, #18915, #16623, #2158, #7363, #27930, #18458, #4889 ),
 .UNSPECIFIED., .F., .F. ) 
 B_SPLINE_CURVE_WITH_KNOTS ( ( 3, 2, 2, 2, 3 ),
 ( 0.9472222222222221877, 0.9481481481481481843, 0.9499999999999999556, 0.9518518518518518379, 0.9527777777777778345 ),
 .UNSPECIFIED. ) 
 CURVE ( )  GEOMETRIC_REPRESENTATION_ITEM ( )  RATIONAL_B_SPLINE_CURVE ( ( 0.9330127018922194093, 0.9330127018922154125, 1.000000000000000000, 0.8660254037844388186, 1.000000000000000000, 0.8660254037844388186, 1.000000000000000000, 0.9330127018922154125, 0.9330127018922194093 ) ) 
 REPRESENTATION_ITEM ( '' )  );
#12931=EDGE_CURVE ( 'NONE', #16922, #5496, #12764, .T. ) ;
#12933=CARTESIAN_POINT ( 'NONE',  ( 5.412658773652712085, -3.125000000000086153, -138.9330127018922383 ) ) ;
#12935=CARTESIAN_POINT ( 'NONE',  ( 7.216878364870455975, -6.409875621278545621E-14, -124.4419872981078328 ) ) ;
#12936=CARTESIAN_POINT ( 'NONE',  ( 6.350852961086080661, -9.614813431917819062E-14, -171.3750000000000000 ) ) ;
#12937=CARTESIAN_POINT ( 'NONE',  ( -5.196152422706573404, -3.000000000000002665, -167.7886751345948255 ) ) ;
#12942=DIRECTION ( 'NONE',  ( -7.147005652999508048E-36, 5.642372883946980038E-36, 1.000000000000000000 ) ) ;
#12946=CARTESIAN_POINT ( 'NONE',  ( 2.775557561562891351E-14, -6.250000000000061284, -69.31698729810781856 ) ) ;
#12947=CARTESIAN_POINT ( 'NONE',  ( -7.216878364870328078, 0.000000000000000000, -57.69198729810781856 ) ) ;
#12948=LINE ( 'NONE', #6596, #3398 ) ;
#12952=CARTESIAN_POINT ( 'NONE',  ( -3.175426480542816510, -5.500000000000057732, -129.8750000000000284 ) ) ;
#12955=CARTESIAN_POINT ( 'NONE',  ( -6.000000000000000888, 1.067854986875958443E-15, 7.560779664488942560E-35 ) ) ;
#12957=CARTESIAN_POINT ( 'NONE',  ( 6.000000000000000888, 1.743066579297358182E-13, -97.58632486540524553 ) ) ;
#12958=CARTESIAN_POINT ( 'NONE',  ( 6.000000000000052403, -1.607695154586662678, -99.73066243270258724 ) ) ;
#12960=ORIENTED_EDGE ( 'NONE', *, *, #9360, .F. ) ;
#12962=CARTESIAN_POINT ( 'NONE',  ( 3.464101615137852974, 5.999999999999884537, -71.83632486540520290 ) ) ;
#12963=CARTESIAN_POINT ( 'NONE',  ( 5.412658773652712085, -3.125000000000086153, -93.06698729810780435 ) ) ;
#12974=CARTESIAN_POINT ( 'NONE',  ( 6.350852961086080661, -9.614813431917819062E-14, -48.37500000000000711 ) ) ;
#12976=CARTESIAN_POINT ( 'NONE',  ( 3.464101615137757051, -5.999999999999979572, -51.33632486540523843 ) ) ;
#12977=CARTESIAN_POINT ( 'NONE',  ( 5.196152422706629359, -2.999999999999988898, -79.71132486540521711 ) ) ;
#12978=CARTESIAN_POINT ( 'NONE',  ( -3.608439182435115633, 6.249999999999965361, -75.30801270189223828 ) ) ;
#12979=CYLINDRICAL_SURFACE ( 'NONE', #28550, 6.000000000000000888 ) ;
#12985=CARTESIAN_POINT ( 'NONE',  ( -4.763139720814407951, 2.749999999999946709, -133.2500000000000284 ) ) ;
#12987=CARTESIAN_POINT ( 'NONE',  ( -5.412658773652739619, 3.124999999999975131, -147.1830127018922667 ) ) ;
#12990=CARTESIAN_POINT ( 'NONE',  ( 4.763139720814407951, 2.750000000000002665, -61.75000000000002842 ) ) ;
#12991=CARTESIAN_POINT ( 'NONE',  ( 0.000000000000000000, 5.499999999999991118, -58.50000000000000000 ) ) ;
#12992=CARTESIAN_POINT ( 'NONE',  ( -3.464101615137725076, 5.999999999999979572, -170.5863248654052029 ) ) ;
#12995=CARTESIAN_POINT ( 'NONE',  ( 0.000000000000000000, -5.999999999999991118, -118.0386751345948113 ) ) ;
#12996=DIRECTION ( 'NONE',  ( -7.147005652999508048E-36, 5.642372883946980038E-36, 1.000000000000000000 ) ) ;
#12998=ADVANCED_FACE ( 'NONE', ( #24695 ), #8249, .T. ) ;
#12999=EDGE_LOOP ( 'NONE', ( #19099, #25929, #19409, #26318 ) ) ;
#13002=CARTESIAN_POINT ( 'NONE',  ( -2.775557561562891351E-14, -5.500000000000115463, -147.7500000000000568 ) ) ;
#13003=CARTESIAN_POINT ( 'NONE',  ( -3.608439182435052128, -6.250000000000110134, -49.94198729810783988 ) ) ;
#13006=CARTESIAN_POINT ( 'NONE',  ( 2.775557561562891351E-14, -6.250000000000061284, -147.3169872981078186 ) ) ;
#13007=CARTESIAN_POINT ( 'NONE',  ( -3.175426480542816510, 5.499999999999865885, -74.87500000000000000 ) ) ;
#13010=CARTESIAN_POINT ( 'NONE',  ( -3.608439182435115633, 6.249999999999965361, -97.80801270189222407 ) ) ;
#13011=CARTESIAN_POINT ( 'NONE',  ( 2.676951800742168933E-14, -11.00000000000000000, -19.00000000000002132 ) ) ;
#13013=CARTESIAN_POINT ( 'NONE',  ( -5.999999999999963585, 1.780251999655701777E-13, -86.91367513459485394 ) ) ;
#13014=AXIS2_PLACEMENT_3D ( 'NONE', #13021, #22975, #6518 ) ;
#13015=LINE ( 'NONE', #15937, #5847 ) ;
#13018=CARTESIAN_POINT ( 'NONE',  ( 4.763139720814407951, -2.749999999999988454, -153.5000000000000284 ) ) ;
#13020=CARTESIAN_POINT ( 'NONE',  ( 4.763139720814407951, 2.750000000000002665, -148.7500000000000568 ) ) ;
#13021=CARTESIAN_POINT ( 'NONE',  ( 2.775557561562891351E-14, 5.874999999999977796, -46.71650635094615467 ) ) ;
#13022=EDGE_CURVE ( 'NONE', #6076, #11685, #23318, .T. ) ;
#13023=CARTESIAN_POINT ( 'NONE',  ( -2.775557561562891351E-14, -5.500000000000115463, -83.25000000000004263 ) ) ;
#13025=CARTESIAN_POINT ( 'NONE',  ( -4.763139720814407951, -2.750000000000016431, -85.00000000000001421 ) ) ;
#13031=AXIS2_PLACEMENT_3D ( 'NONE', #22053, #1138, #3288 ) ;
#13032=CARTESIAN_POINT ( 'NONE',  ( -5.999999999999904965, -1.607695154586834541, -165.7693375672973559 ) ) ;
#13034=CARTESIAN_POINT ( 'NONE',  ( -5.999999999999963585, 1.780251999655701777E-13, -77.91367513459482552 ) ) ;
#13039=CARTESIAN_POINT ( 'NONE',  ( -5.999999999999963585, 1.780251999655701777E-13, -53.91367513459482552 ) ) ;
#13042=ORIENTED_EDGE ( 'NONE', *, *, #27603, .F. ) ;
#13043=AXIS2_PLACEMENT_3D ( 'NONE', #3844, #25042, #1554 ) ;
#13045=ORIENTED_EDGE ( 'NONE', *, *, #13697, .T. ) ;
#13046=CARTESIAN_POINT ( 'NONE',  ( -4.763139720814407951, 2.749999999999946709, -100.2500000000000000 ) ) ;
#13049=CARTESIAN_POINT ( 'NONE',  ( 2.775557561562891351E-14, -6.250000000000061284, -115.1830127018922383 ) ) ;
#13054=AXIS2_PLACEMENT_3D ( 'NONE', #218, #4825, #19831 ) ;
#13055=CARTESIAN_POINT ( 'NONE',  ( -3.608439182435052128, -6.250000000000110134, -49.30801270189224539 ) ) ;
#13056=ORIENTED_EDGE ( 'NONE', *, *, #1895, .F. ) ;
#13057=CARTESIAN_POINT ( 'NONE',  ( 6.000000000000000888, 7.762456499804234384E-14, -119.1636751345948113 ) ) ;
#13058=LINE ( 'NONE', #22391, #26259 ) ;
#13059=FACE_OUTER_BOUND ( 'NONE', #29315, .T. ) ;
#13060=CARTESIAN_POINT ( 'NONE',  ( -4.763139720814407951, 2.749999999999946709, -173.7500000000000284 ) ) ;
#13061=( BOUNDED_CURVE ( )  B_SPLINE_CURVE ( 2, ( #8480, #6180, #22630, #11591, #4780, #4919, #29972, #23090, #9558 ),
 .UNSPECIFIED., .F., .F. ) 
 B_SPLINE_CURVE_WITH_KNOTS ( ( 3, 2, 2, 2, 3 ),
 ( 0.5861111111111111382, 0.5870370370370370239, 0.5888888888888889062, 0.5907407407407407884, 0.5916666666666666741 ),
 .UNSPECIFIED. ) 
 CURVE ( )  GEOMETRIC_REPRESENTATION_ITEM ( )  RATIONAL_B_SPLINE_CURVE ( ( 0.9330127018922194093, 0.9330127018922234061, 1.000000000000000000, 0.8660254037844388186, 1.000000000000000000, 0.8660254037844388186, 1.000000000000000000, 0.9330127018922194093, 0.9330127018922194093 ) ) 
 REPRESENTATION_ITEM ( '' )  );
#13064=CARTESIAN_POINT ( 'NONE',  ( 3.608439182435180470, 6.249999999999982236, -170.0580127018922383 ) ) ;
#13067=CARTESIAN_POINT ( 'NONE',  ( 4.763139720814407951, 2.750000000000002665, -108.2500000000000142 ) ) ;
#13068=DIRECTION ( 'NONE',  ( -7.147005652999508048E-36, 5.642372883946980038E-36, 1.000000000000000000 ) ) ;
#13069=CARTESIAN_POINT ( 'NONE',  ( 4.763139720814407951, -2.749999999999988454, -104.0000000000000426 ) ) ;
#13071=CARTESIAN_POINT ( 'NONE',  ( 0.000000000000000000, 0.000000000000000000, 0.000000000000000000 ) ) ;
#13073=VERTEX_POINT ( 'NONE', #14664 ) ;
#13075=CARTESIAN_POINT ( 'NONE',  ( 0.000000000000000000, -5.999999999999991118, -90.46132486540525974 ) ) ;
#13078=EDGE_CURVE ( 'NONE', #19519, #23669, #22318, .T. ) ;
#13080=CARTESIAN_POINT ( 'NONE',  ( -4.763139720814407951, -2.750000000000016431, -158.5000000000000284 ) ) ;
#13081=CARTESIAN_POINT ( 'NONE',  ( -5.999999999999919176, 1.607695154586804565, -65.40331216351300725 ) ) ;
#13083=CARTESIAN_POINT ( 'NONE',  ( 7.216878364870455975, -6.409875621278545621E-14, -85.44198729810781856 ) ) ;
#13085=ORIENTED_EDGE ( 'NONE', *, *, #4895, .F. ) ;
#13089=CARTESIAN_POINT ( 'NONE',  ( 4.763139720814407951, 2.750000000000002665, -129.2500000000000284 ) ) ;
#13090=CARTESIAN_POINT ( 'NONE',  ( 5.412658773652712085, -3.125000000000086153, -135.9330127018922383 ) ) ;
#13091=ORIENTED_EDGE ( 'NONE', *, *, #8411, .F. ) ;
#13092=CARTESIAN_POINT ( 'NONE',  ( -5.196152422706573404, -3.000000000000002665, -57.71132486540520290 ) ) ;
#13093=CARTESIAN_POINT ( 'NONE',  ( 2.775557561562891351E-14, 6.250000000000033751, -125.5669872981078328 ) ) ;
#13094=CARTESIAN_POINT ( 'NONE',  ( 4.763139720814407951, -2.749999999999988454, -170.0000000000000284 ) ) ;
#13100=CYLINDRICAL_SURFACE ( 'NONE', #29000, 6.000000000000000888 ) ;
#13103=CARTESIAN_POINT ( 'NONE',  ( 2.775557561562891351E-14, 6.250000000000033751, -64.06698729810783277 ) ) ;
#13105=CARTESIAN_POINT ( 'NONE',  ( 3.608439182435180470, 6.249999999999982236, -52.19198729810779014 ) ) ;
#13107=CARTESIAN_POINT ( 'NONE',  ( -5.196152422706601826, 2.999999999999975131, -55.53867513459487526 ) ) ;
#13108=EDGE_CURVE ( 'NONE', #20574, #8576, #12737, .T. ) ;
#13110=CARTESIAN_POINT ( 'NONE',  ( -2.775557561562891351E-14, -5.500000000000115463, -131.2500000000000284 ) ) ;
#13111=VERTEX_POINT ( 'NONE', #19420 ) ;
#13114=CARTESIAN_POINT ( 'NONE',  ( -5.196152422706601826, 2.999999999999975131, -96.96132486540520290 ) ) ;
#13116=CARTESIAN_POINT ( 'NONE',  ( -5.999999999999919176, 1.607695154586804565, -129.9033121635129930 ) ) ;
#13117=( BOUNDED_CURVE ( )  B_SPLINE_CURVE ( 2, ( #18989, #510, #21730, #10055, #669, #28314, #4965, #14396, #23732 ),
 .UNSPECIFIED., .F., .T. ) 
 B_SPLINE_CURVE_WITH_KNOTS ( ( 3, 2, 2, 2, 3 ),
 ( 0.4972222222222222321, 0.4981481481481481732, 0.5000000000000000000, 0.5018518518518518823, 0.5027777777777777679 ),
 .UNSPECIFIED. ) 
 CURVE ( )  GEOMETRIC_REPRESENTATION_ITEM ( )  RATIONAL_B_SPLINE_CURVE ( ( 0.9330127018922194093, 0.9330127018922194093, 1.000000000000000000, 0.8660254037844388186, 1.000000000000000000, 0.8660254037844388186, 1.000000000000000000, 0.9330127018922194093, 0.9330127018922194093 ) ) 
 REPRESENTATION_ITEM ( '' )  );
#13118=ORIENTED_EDGE ( 'NONE', *, *, #2889, .T. ) ;
#13120=CARTESIAN_POINT ( 'NONE',  ( -3.608439182435052128, -6.250000000000110134, -118.9419872981078612 ) ) ;
#13123=ORIENTED_EDGE ( 'NONE', *, *, #11079, .T. ) ;
#13124=DIRECTION ( 'NONE',  ( -7.147005652999508048E-36, 5.642372883946980038E-36, 1.000000000000000000 ) ) ;
#13126=CARTESIAN_POINT ( 'NONE',  ( -3.464101615137757051, -5.999999999999979572, -138.5863248654051745 ) ) ;
#13127=CARTESIAN_POINT ( 'NONE',  ( 0.000000000000000000, 5.499999999999991118, -52.49999999999999289 ) ) ;
#13131=CARTESIAN_POINT ( 'NONE',  ( 3.464101615137757051, -5.999999999999979572, -79.83632486540523132 ) ) ;
#13132=CARTESIAN_POINT ( 'NONE',  ( -5.412658773652739619, 3.124999999999975131, -76.68301270189226670 ) ) ;
#13133=CARTESIAN_POINT ( 'NONE',  ( 6.000000000000000888, -1.607695154586752384, -172.6533121635129930 ) ) ;
#13135=DIRECTION ( 'NONE',  ( -7.147005652999508048E-36, 5.642372883946980038E-36, 1.000000000000000000 ) ) ;
#13136=SURFACE_STYLE_FILL_AREA ( #29823 ) ;
#13140=EDGE_CURVE ( 'NONE', #10034, #17588, #4959, .T. ) ;
#13141=EDGE_CURVE ( 'NONE', #11998, #13496, #28392, .T. ) ;
#13142=CARTESIAN_POINT ( 'NONE',  ( -6.350852961085760029, -1.281975124255709124E-13, -130.1250000000000284 ) ) ;
#13145=CYLINDRICAL_SURFACE ( 'NONE', #25804, 6.000000000000000888 ) ;
#13147=CARTESIAN_POINT ( 'NONE',  ( -2.775557561562891351E-14, -5.500000000000115463, -59.25000000000002842 ) ) ;
#13149=CARTESIAN_POINT ( 'NONE',  ( 6.000000000000000888, 1.607695154586715303, -172.5193375672974412 ) ) ;
#13150=CARTESIAN_POINT ( 'NONE',  ( 5.999999999999999112, 2.951592740943527306E-14, -162.6636751345948824 ) ) ;
#13157=CARTESIAN_POINT ( 'NONE',  ( -3.464101615137757051, -5.999999999999979572, -49.16367513459483973 ) ) ;
#13158=VECTOR ( 'NONE', #23558, 1000.000000000000000 ) ;
#13162=CARTESIAN_POINT ( 'NONE',  ( -5.999999999999963585, 1.780251999655701777E-13, -73.41367513459483973 ) ) ;
#13163=ORIENTED_EDGE ( 'NONE', *, *, #25430, .T. ) ;
#13165=CARTESIAN_POINT ( 'NONE',  ( -6.350852961085760029, -1.281975124255709124E-13, -143.6250000000000000 ) ) ;
#13167=CARTESIAN_POINT ( 'NONE',  ( -3.608439182435115633, 6.249999999999965361, -50.44198729810784698 ) ) ;
#13169=ORIENTED_EDGE ( 'NONE', *, *, #11414, .T. ) ;
#13170=CARTESIAN_POINT ( 'NONE',  ( -3.175426480542816510, 5.499999999999865885, -76.37500000000001421 ) ) ;
#13172=CARTESIAN_POINT ( 'NONE',  ( 2.775557561562891351E-14, 6.250000000000033751, -94.93301270189225249 ) ) ;
#13174=CARTESIAN_POINT ( 'NONE',  ( -5.687368478357993418, -9.417270245429932629, -26.95189157943835667 ) ) ;
#13175=CARTESIAN_POINT ( 'NONE',  ( 3.464101615137757051, -5.999999999999979572, -83.41367513459481131 ) ) ;
#13178=CARTESIAN_POINT ( 'NONE',  ( -6.000000000000007105, -1.607695154586655129, -65.26933756729742697 ) ) ;
#13181=CARTESIAN_POINT ( 'NONE',  ( -3.175426480542816066, -5.500000000000057732, -155.3750000000000000 ) ) ;
#13183=CARTESIAN_POINT ( 'NONE',  ( 6.350852961086080661, -9.614813431917819062E-14, -141.3750000000000568 ) ) ;
#13184=DIRECTION ( 'NONE',  ( 1.000000000000000000, -5.551115123125773458E-17, -1.260129944081490338E-35 ) ) ;
#13185=UNCERTAINTY_MEASURE_WITH_UNIT (LENGTH_MEASURE( 1.000000000000000082E-05 ), #23922, 'distance_accuracy_value', 'NONE');
#13186=CARTESIAN_POINT ( 'NONE',  ( -4.763139720814407951, 2.749999999999946709, -88.25000000000005684 ) ) ;
#13188=CARTESIAN_POINT ( 'NONE',  ( 4.763139720814407951, -2.749999999999988454, -81.50000000000001421 ) ) ;
#13193=DIRECTION ( 'NONE',  ( -7.147005652999508048E-36, 5.642372883946980038E-36, 1.000000000000000000 ) ) ;
#13197=CARTESIAN_POINT ( 'NONE',  ( 5.196152422706629359, -2.999999999999988898, -171.7886751345948255 ) ) ;
#13201=( BOUNDED_CURVE ( )  B_SPLINE_CURVE ( 2, ( #28640, #994, #17468, #19748, #17323, #7611, #26639, #16881, #14855 ),
 .UNSPECIFIED., .F., .T. ) 
 B_SPLINE_CURVE_WITH_KNOTS ( ( 3, 2, 2, 2, 3 ),
 ( 0.1916666666666666519, 0.1925925925925925375, 0.1944444444444444198, 0.1962962962962963021, 0.1972222222222222987 ),
 .UNSPECIFIED. ) 
 CURVE ( )  GEOMETRIC_REPRESENTATION_ITEM ( )  RATIONAL_B_SPLINE_CURVE ( ( 0.9330127018922194093, 0.9330127018922194093, 1.000000000000000000, 0.8660254037844388186, 1.000000000000000000, 0.8660254037844388186, 1.000000000000000000, 0.9330127018922154125, 0.9330127018922194093 ) ) 
 REPRESENTATION_ITEM ( '' )  );
#13202=ORIENTED_EDGE ( 'NONE', *, *, #18843, .T. ) ;
#13203=EDGE_CURVE ( 'NONE', #11924, #16705, #19020, .T. ) ;
#13204=CARTESIAN_POINT ( 'NONE',  ( -3.175426480542816510, 5.499999999999865885, -94.37500000000002842 ) ) ;
#13205=DIRECTION ( 'NONE',  ( 1.000000000000000000, -5.551115123125773458E-17, -1.260129944081490338E-35 ) ) ;
#13206=CARTESIAN_POINT ( 'NONE',  ( 5.412658773652712085, -3.125000000000086153, -116.4330127018922099 ) ) ;
#13207=( BOUNDED_CURVE ( )  B_SPLINE_CURVE ( 2, ( #4295, #20433, #20591, #25479, #27466, #13871, #4137, #16326, #23055 ),
 .UNSPECIFIED., .F., .T. ) 
 B_SPLINE_CURVE_WITH_KNOTS ( ( 3, 2, 2, 2, 3 ),
 ( 0.9916666666666665853, 0.9925925925925925819, 0.9944444444444444642, 0.9962962962962963465, 0.9972222222222222321 ),
 .UNSPECIFIED. ) 
 CURVE ( )  GEOMETRIC_REPRESENTATION_ITEM ( )  RATIONAL_B_SPLINE_CURVE ( ( 0.9330127018922194093, 0.9330127018922154125, 1.000000000000000000, 0.8660254037844388186, 1.000000000000000000, 0.8660254037844388186, 1.000000000000000000, 0.9330127018922194093, 0.9330127018922194093 ) ) 
 REPRESENTATION_ITEM ( '' )  );
#13208=ORIENTED_EDGE ( 'NONE', *, *, #4974, .F. ) ;
#13210=CARTESIAN_POINT ( 'NONE',  ( 7.216878364870455975, -6.409875621278545621E-14, -51.80801270189225960 ) ) ;
#13211=ORIENTED_EDGE ( 'NONE', *, *, #1587, .F. ) ;
#13216=CARTESIAN_POINT ( 'NONE',  ( -6.350852961085760029, -1.281975124255709124E-13, -173.6250000000000284 ) ) ;
#13218=CARTESIAN_POINT ( 'NONE',  ( 5.196152422706629359, 3.000000000000002665, -107.9613248654052171 ) ) ;
#13219=CARTESIAN_POINT ( 'NONE',  ( 6.000000000000000888, 1.743066579297358182E-13, -87.08632486540520290 ) ) ;
#13221=CARTESIAN_POINT ( 'NONE',  ( 3.175426480543072749, 5.499999999999865885, -108.1250000000000284 ) ) ;
#13222=CARTESIAN_POINT ( 'NONE',  ( 5.196152422706629359, 3.000000000000002665, -162.5386751345948539 ) ) ;
#13223=CARTESIAN_POINT ( 'NONE',  ( 6.000000000000052403, -1.607695154586662678, -81.73066243270260145 ) ) ;
#13224=EDGE_LOOP ( 'NONE', ( #4576, #30349, #21010, #6043 ) ) ;
#13227=ORIENTED_EDGE ( 'NONE', *, *, #12634, .T. ) ;
#13228=CARTESIAN_POINT ( 'NONE',  ( -3.464101615137725076, 5.999999999999979572, -156.1636751345947687 ) ) ;
#13229=CARTESIAN_POINT ( 'NONE',  ( -3.608439182435052128, -6.250000000000110134, -78.44198729810779014 ) ) ;
#13232=CARTESIAN_POINT ( 'NONE',  ( -5.999999999999956479, -1.607695154586745057, -75.76933756729744118 ) ) ;
#13234=VERTEX_POINT ( 'NONE', #6021 ) ;
#13237=CARTESIAN_POINT ( 'NONE',  ( 4.763139720814407951, -2.749999999999988454, -125.0000000000000000 ) ) ;
#13238=CARTESIAN_POINT ( 'NONE',  ( -5.412658773652684552, -3.125000000000099920, -137.9330127018922383 ) ) ;
#13239=ORIENTED_EDGE ( 'NONE', *, *, #4003, .T. ) ;
#13240=CARTESIAN_POINT ( 'NONE',  ( 5.999999999999949374, 1.607695154586804565, -57.59668783648704249 ) ) ;
#13241=CARTESIAN_POINT ( 'NONE',  ( 7.216878364870455975, -6.409875621278545621E-14, -121.4419872981078043 ) ) ;
#13242=CARTESIAN_POINT ( 'NONE',  ( -5.412658773652684552, -3.125000000000099920, -179.0669872981078186 ) ) ;
#13243=CARTESIAN_POINT ( 'NONE',  ( -3.175426480542816510, 5.499999999999865885, -172.3750000000000000 ) ) ;
#13246=VERTEX_POINT ( 'NONE', #24766 ) ;
#13250=CARTESIAN_POINT ( 'NONE',  ( 0.000000000000000000, 5.999999999999977796, -148.2113248654052313 ) ) ;
#13254=CARTESIAN_POINT ( 'NONE',  ( 5.412658773652712085, -3.125000000000086153, -67.56698729810783277 ) ) ;
#13255=CARTESIAN_POINT ( 'NONE',  ( 2.775557561562891351E-14, -6.250000000000061284, -55.81698729810780435 ) ) ;
#13257=CARTESIAN_POINT ( 'NONE',  ( -3.175426480542816510, -5.500000000000057732, -47.37500000000000000 ) ) ;
#13258=CARTESIAN_POINT ( 'NONE',  ( -3.464101615137725076, 5.999999999999979572, -55.66367513459481131 ) ) ;
#13259=CARTESIAN_POINT ( 'NONE',  ( -2.775557561562891351E-14, -5.500000000000115463, -129.7500000000000284 ) ) ;
#13260=CARTESIAN_POINT ( 'NONE',  ( 6.000000000000000888, -1.859271017917181981E-14, -115.5863248654052171 ) ) ;
#13261=VERTEX_POINT ( 'NONE', #1413 ) ;
#13265=CARTESIAN_POINT ( 'NONE',  ( 3.464101615137852974, 5.999999999999884537, -97.33632486540517448 ) ) ;
#13270=CARTESIAN_POINT ( 'NONE',  ( 3.608439182435180470, -6.249999999999997335, -118.6919872981078612 ) ) ;
#13273=ORIENTED_EDGE ( 'NONE', *, *, #22012, .T. ) ;
#13279=CARTESIAN_POINT ( 'NONE',  ( 4.763139720814407951, -2.749999999999988454, -53.00000000000004974 ) ) ;
#13282=FACE_OUTER_BOUND ( 'NONE', #16753, .T. ) ;
#13285=CARTESIAN_POINT ( 'NONE',  ( 2.775557561562891351E-14, 6.250000000000033751, -69.43301270189222407 ) ) ;
#13289=CARTESIAN_POINT ( 'NONE',  ( 6.000000000000007105, -1.607695154586741060, -177.7306624327026157 ) ) ;
#13291=CARTESIAN_POINT ( 'NONE',  ( -6.000000000000007105, -1.607695154586655129, -94.34668783648703538 ) ) ;
#13292=( BOUNDED_CURVE ( )  B_SPLINE_CURVE ( 2, ( #17519, #15686, #3496, #3646, #8103, #18126, #8426, #27441, #13376 ),
 .UNSPECIFIED., .F., .T. ) 
 B_SPLINE_CURVE_WITH_KNOTS ( ( 3, 2, 2, 2, 3 ),
 ( 0.6250000000000000000, 0.6259259259259258856, 0.6277777777777777679, 0.6296296296296296502, 0.6305555555555556468 ),
 .UNSPECIFIED. ) 
 CURVE ( )  GEOMETRIC_REPRESENTATION_ITEM ( )  RATIONAL_B_SPLINE_CURVE ( ( 0.9330127018922194093, 0.9330127018922194093, 1.000000000000000000, 0.8660254037844388186, 1.000000000000000000, 0.8660254037844388186, 1.000000000000000000, 0.9330127018922154125, 0.9330127018922194093 ) ) 
 REPRESENTATION_ITEM ( '' )  );
#13293=CARTESIAN_POINT ( 'NONE',  ( 3.175426480543072749, 5.499999999999865885, -130.6250000000000284 ) ) ;
#13294=ORIENTED_EDGE ( 'NONE', *, *, #23855, .F. ) ;
#13295=CARTESIAN_POINT ( 'NONE',  ( -2.775557561562891351E-14, -5.500000000000115463, -66.75000000000002842 ) ) ;
#13296=DIRECTION ( 'NONE',  ( -7.147005652999508048E-36, 5.642372883946980038E-36, 1.000000000000000000 ) ) ;
#13304=CARTESIAN_POINT ( 'NONE',  ( 6.000000000000000888, 1.743066579297358182E-13, -48.66367513459482552 ) ) ;
#13308=CARTESIAN_POINT ( 'NONE',  ( -3.464101615137757051, -5.999999999999979572, -122.0863248654051745 ) ) ;
#13312=CARTESIAN_POINT ( 'NONE',  ( -3.175426480542816510, -5.500000000000057732, -144.8750000000000853 ) ) ;
#13315=CARTESIAN_POINT ( 'NONE',  ( 3.175426480543072749, -5.500000000000105693, -69.62500000000004263 ) ) ;
#13317=CARTESIAN_POINT ( 'NONE',  ( 5.412658773652712085, -3.125000000000086153, -96.93301270189225249 ) ) ;
#13319=CARTESIAN_POINT ( 'NONE',  ( -5.999999999999968026, -1.607695154586722186, -151.3466878364870354 ) ) ;
#13321=CARTESIAN_POINT ( 'NONE',  ( -5.196152422706573404, -3.000000000000002665, -65.21132486540520290 ) ) ;
#13323=CIRCLE ( 'NONE', #26508, 4.000000000000006217 ) ;
#13324=CARTESIAN_POINT ( 'NONE',  ( -4.763139720814407951, 2.749999999999946709, -152.7500000000000568 ) ) ;
#13325=DIRECTION ( 'NONE',  ( -7.147005652999508048E-36, 5.642372883946980038E-36, 1.000000000000000000 ) ) ;
#13326=CARTESIAN_POINT ( 'NONE',  ( -5.511802646642890657, 2.338480655328711855, -180.0000000000001137 ) ) ;
#13327=CARTESIAN_POINT ( 'NONE',  ( -2.775557561562891351E-14, -5.500000000000115463, -89.25000000000005684 ) ) ;
#13330=CARTESIAN_POINT ( 'NONE',  ( -4.763139720814407951, 2.749999999999946709, -71.75000000000004263 ) ) ;
#13332=CARTESIAN_POINT ( 'NONE',  ( 3.464101615137757051, -5.999999999999979572, -120.3363248654051461 ) ) ;
#13333=CARTESIAN_POINT ( 'NONE',  ( -3.464101615137725076, 5.999999999999979572, -142.0863248654052029 ) ) ;
#13335=( BOUNDED_CURVE ( )  B_SPLINE_CURVE ( 2, ( #28311, #7289, #16692, #23730, #12086, #21425, #19279, #5710, #5263 ),
 .UNSPECIFIED., .F., .F. ) 
 B_SPLINE_CURVE_WITH_KNOTS ( ( 3, 2, 2, 2, 3 ),
 ( 0.8027777777777777013, 0.8037037037037036979, 0.8055555555555555802, 0.8074074074074074625, 0.8083333333333333481 ),
 .UNSPECIFIED. ) 
 CURVE ( )  GEOMETRIC_REPRESENTATION_ITEM ( )  RATIONAL_B_SPLINE_CURVE ( ( 0.9330127018922194093, 0.9330127018922154125, 1.000000000000000000, 0.8660254037844388186, 1.000000000000000000, 0.8660254037844388186, 1.000000000000000000, 0.9330127018922194093, 0.9330127018922194093 ) ) 
 REPRESENTATION_ITEM ( '' )  );
#13337=CARTESIAN_POINT ( 'NONE',  ( -3.464101615137725076, 5.999999999999979572, -174.1636751345948255 ) ) ;
#13338=ORIENTED_EDGE ( 'NONE', *, *, #22539, .T. ) ;
#13340=CARTESIAN_POINT ( 'NONE',  ( 6.000000000000000888, -1.859271017917181981E-14, -137.1636751345948255 ) ) ;
#13343=ORIENTED_EDGE ( 'NONE', *, *, #5140, .T. ) ;
#13344=EDGE_CURVE ( 'NONE', #15139, #14585, #10384, .T. ) ;
#13347=CARTESIAN_POINT ( 'NONE',  ( 3.175426480543072749, -5.500000000000105693, -101.1250000000000000 ) ) ;
#13348=CARTESIAN_POINT ( 'NONE',  ( 3.608439182435180470, -6.249999999999997335, -113.5580127018922383 ) ) ;
#13350=CARTESIAN_POINT ( 'NONE',  ( -5.196152422706601826, 2.999999999999975131, -91.53867513459485394 ) ) ;
#13354=CARTESIAN_POINT ( 'NONE',  ( -3.608439182435115633, 6.249999999999965361, -52.80801270189225960 ) ) ;
#13356=CARTESIAN_POINT ( 'NONE',  ( -4.763139720814407951, -2.750000000000016431, -163.0000000000000284 ) ) ;
#13358=CARTESIAN_POINT ( 'NONE',  ( -5.999999999999963585, 1.780251999655701777E-13, -78.83632486540523132 ) ) ;
#13360=CARTESIAN_POINT ( 'NONE',  ( -3.175426480542816066, 5.499999999999865885, -107.8750000000000284 ) ) ;
#13363=CARTESIAN_POINT ( 'NONE',  ( 4.763139720814407951, -2.749999999999988454, -101.0000000000000284 ) ) ;
#13364=CARTESIAN_POINT ( 'NONE',  ( -5.999999999999957367, 1.607695154586737507, -151.4806624327026157 ) ) ;
#13366=CARTESIAN_POINT ( 'NONE',  ( -5.999999999999963585, 1.780251999655701777E-13, -84.83632486540523132 ) ) ;
#13372=( BOUNDED_CURVE ( )  B_SPLINE_CURVE ( 2, ( #10156, #19529, #28862, #7822, #26564, #3205, #21975, #10305, #8444 ),
 .UNSPECIFIED., .F., .T. ) 
 B_SPLINE_CURVE_WITH_KNOTS ( ( 3, 2, 2, 2, 3 ),
 ( 0.3138888888888888840, 0.3148148148148148251, 0.3166666666666666519, 0.3185185185185185341, 0.3194444444444444753 ),
 .UNSPECIFIED. ) 
 CURVE ( )  GEOMETRIC_REPRESENTATION_ITEM ( )  RATIONAL_B_SPLINE_CURVE ( ( 0.9330127018922194093, 0.9330127018922194093, 1.000000000000000000, 0.8660254037844388186, 1.000000000000000000, 0.8660254037844388186, 1.000000000000000000, 0.9330127018922174109, 0.9330127018922194093 ) ) 
 REPRESENTATION_ITEM ( '' )  );
#13374=CARTESIAN_POINT ( 'NONE',  ( 0.000000000000000000, -5.999999999999991118, -169.9613248654052029 ) ) ;
#13376=CARTESIAN_POINT ( 'NONE',  ( 6.000000000000000888, 1.743066579297358182E-13, -96.66367513459479710 ) ) ;
#13377=ORIENTED_EDGE ( 'NONE', *, *, #2588, .F. ) ;
#13378=CARTESIAN_POINT ( 'NONE',  ( -3.033369321062190593, 10.57893614291643125, -30.19141222485917808 ) ) ;
#13380=( BOUNDED_CURVE ( )  B_SPLINE_CURVE ( 2, ( #1253, #20174, #29360, #22011, #947, #10662, #17732, #6022, #22478 ),
 .UNSPECIFIED., .F., .T. ) 
 B_SPLINE_CURVE_WITH_KNOTS ( ( 3, 2, 2, 2, 3 ),
 ( 0.4305555555555555802, 0.4314814814814814659, 0.4333333333333333481, 0.4351851851851852304, 0.4361111111111111160 ),
 .UNSPECIFIED. ) 
 CURVE ( )  GEOMETRIC_REPRESENTATION_ITEM ( )  RATIONAL_B_SPLINE_CURVE ( ( 0.9330127018922194093, 0.9330127018922234061, 1.000000000000000000, 0.8660254037844388186, 1.000000000000000000, 0.8660254037844388186, 1.000000000000000000, 0.9330127018922194093, 0.9330127018922194093 ) ) 
 REPRESENTATION_ITEM ( '' )  );
#13381=VERTEX_POINT ( 'NONE', #14206 ) ;
#13384=CARTESIAN_POINT ( 'NONE',  ( 3.175426480543072749, 5.499999999999865885, -121.6250000000000284 ) ) ;
#13385=CARTESIAN_POINT ( 'NONE',  ( 7.216878364870455975, -6.409875621278545621E-14, -141.8080127018922099 ) ) ;
#13386=EDGE_LOOP ( 'NONE', ( #19204, #26842, #1423, #27153 ) ) ;
#13387=CARTESIAN_POINT ( 'NONE',  ( -5.999999999999957367, 1.607695154586737507, -160.4806624327025872 ) ) ;
#13388=CARTESIAN_POINT ( 'NONE',  ( 3.608439182435180470, 6.249999999999982236, -127.1919872981078186 ) ) ;
#13389=CARTESIAN_POINT ( 'NONE',  ( 2.775557561562891351E-14, -6.250000000000061284, -178.8169872981077901 ) ) ;
#13390=CARTESIAN_POINT ( 'NONE',  ( -2.775557561562891351E-14, -5.500000000000115463, -171.7500000000000000 ) ) ;
#13399=CARTESIAN_POINT ( 'NONE',  ( -5.412658773652739619, 3.124999999999975131, -77.31698729810781856 ) ) ;
#13400=CARTESIAN_POINT ( 'NONE',  ( -5.196152422706601826, 2.999999999999975131, -110.4613248654052171 ) ) ;
#13401=CARTESIAN_POINT ( 'NONE',  ( -2.775557561562891351E-14, -5.500000000000115463, -47.25000000000001421 ) ) ;
#13403=CARTESIAN_POINT ( 'NONE',  ( -5.999999999999963585, -1.487416814333745711E-14, -153.8363248654052313 ) ) ;
#13404=CARTESIAN_POINT ( 'NONE',  ( -3.175426480542816510, 5.499999999999865885, -128.8750000000000000 ) ) ;
#13405=ORIENTED_EDGE ( 'NONE', *, *, #30195, .F. ) ;
#13406=CARTESIAN_POINT ( 'NONE',  ( -3.464101615137757051, -5.999999999999979572, -119.0863248654052171 ) ) ;
#13408=CARTESIAN_POINT ( 'NONE',  ( -5.999999999999963585, 0.000000000000000000, -179.3363248654052313 ) ) ;
#13409=CYLINDRICAL_SURFACE ( 'NONE', #18252, 6.000000000000000888 ) ;
#13414=CARTESIAN_POINT ( 'NONE',  ( 2.775557561562891351E-14, 6.250000000000033751, -112.0669872981078186 ) ) ;
#13418=ORIENTED_EDGE ( 'NONE', *, *, #13974, .F. ) ;
#13421=ORIENTED_EDGE ( 'NONE', *, *, #26025, .T. ) ;
#13424=CARTESIAN_POINT ( 'NONE',  ( -3.175426480542816510, -5.500000000000057732, -51.87500000000002132 ) ) ;
#13426=DIRECTION ( 'NONE',  ( -7.147005652999508048E-36, 5.642372883946980038E-36, 1.000000000000000000 ) ) ;
#13428=CARTESIAN_POINT ( 'NONE',  ( -3.608439182435052128, -6.250000000000110134, -65.80801270189225249 ) ) ;
#13431=CARTESIAN_POINT ( 'NONE',  ( -5.999999999999963585, 1.780251999655701777E-13, -77.33632486540524553 ) ) ;
#13432=CARTESIAN_POINT ( 'NONE',  ( -21.99999999999993605, 11.00000000000003730, -14.99152654425661879 ) ) ;
#13435=CARTESIAN_POINT ( 'NONE',  ( -2.775557561562891351E-14, -5.500000000000115463, -129.7500000000000284 ) ) ;
#13437=CARTESIAN_POINT ( 'NONE',  ( 0.000000000000000000, 0.000000000000000000, 0.000000000000000000 ) ) ;
#13438=CARTESIAN_POINT ( 'NONE',  ( -5.999999999999963585, 3.021315404115421074E-15, -177.8363248654052029 ) ) ;
#13439=ORIENTED_EDGE ( 'NONE', *, *, #26102, .T. ) ;
#13441=CARTESIAN_POINT ( 'NONE',  ( -3.175426480542816066, 5.499999999999865885, -61.37500000000000711 ) ) ;
#13442=DIRECTION ( 'NONE',  ( 1.000000000000000000, -5.551115123125773458E-17, -1.260129944081490338E-35 ) ) ;
#13444=CARTESIAN_POINT ( 'NONE',  ( -3.464101615137757051, -5.999999999999979572, -174.5863248654051745 ) ) ;
#13450=LINE ( 'NONE', #22495, #26339 ) ;
#13458=CARTESIAN_POINT ( 'NONE',  ( 0.000000000000000000, 5.499999999999991118, -144.0000000000000284 ) ) ;
#13461=VERTEX_POINT ( 'NONE', #21089 ) ;
#13462=CARTESIAN_POINT ( 'NONE',  ( -6.350852961085760029, -1.281975124255709124E-13, -74.62500000000000000 ) ) ;
#13463=CARTESIAN_POINT ( 'NONE',  ( 3.608439182435180470, -6.249999999999997335, -88.05801270189223828 ) ) ;
#13464=( BOUNDED_CURVE ( )  B_SPLINE_CURVE ( 2, ( #27282, #5785, #29440, #6256, #17819, #24984, #3934, #13364, #1650 ),
 .UNSPECIFIED., .F., .T. ) 
 B_SPLINE_CURVE_WITH_KNOTS ( ( 3, 2, 2, 2, 3 ),
 ( 0.2194444444444444697, 0.2203703703703703831, 0.2222222222222222099, 0.2240740740740740644, 0.2249999999999999778 ),
 .UNSPECIFIED. ) 
 CURVE ( )  GEOMETRIC_REPRESENTATION_ITEM ( )  RATIONAL_B_SPLINE_CURVE ( ( 0.9330127018922194093, 0.9330127018922204085, 1.000000000000000000, 0.8660254037844388186, 1.000000000000000000, 0.8660254037844388186, 1.000000000000000000, 0.9330127018922205195, 0.9330127018922196314 ) ) 
 REPRESENTATION_ITEM ( '' )  );
#13467=CARTESIAN_POINT ( 'NONE',  ( 5.196152422706629359, 3.000000000000002665, -150.5386751345948539 ) ) ;
#13468=CARTESIAN_POINT ( 'NONE',  ( 6.000000000000000888, 1.743066579297358182E-13, -53.16367513459481131 ) ) ;
#13470=CARTESIAN_POINT ( 'NONE',  ( 0.000000000000000000, 0.000000000000000000, 0.000000000000000000 ) ) ;
#13472=CARTESIAN_POINT ( 'NONE',  ( 0.000000000000000000, 5.499999999999991118, -157.5000000000000284 ) ) ;
#13476=EDGE_CURVE ( 'NONE', #30226, #2399, #21956, .T. ) ;
#13477=CARTESIAN_POINT ( 'NONE',  ( 6.350852961086080661, -9.614813431917819062E-14, -90.37500000000001421 ) ) ;
#13479=CARTESIAN_POINT ( 'NONE',  ( 4.763139720814407951, -2.749999999999988454, -69.50000000000000000 ) ) ;
#13480=CYLINDRICAL_SURFACE ( 'NONE', #13882, 6.000000000000000888 ) ;
#13482=CARTESIAN_POINT ( 'NONE',  ( 0.000000000000000000, 5.999999999999977796, -164.7113248654051745 ) ) ;
#13483=CARTESIAN_POINT ( 'NONE',  ( 6.000000000000000888, -3.330669073875464691E-16, -7.560779664488942560E-35 ) ) ;
#13485=CARTESIAN_POINT ( 'NONE',  ( 5.196152422706629359, 3.000000000000002665, -104.0386751345948539 ) ) ;
#13487=CARTESIAN_POINT ( 'NONE',  ( -3.464101615137725076, 5.999999999999979572, -94.66367513459479710 ) ) ;
#13488=DIRECTION ( 'NONE',  ( -7.147005652999508048E-36, 5.642372883946980038E-36, 1.000000000000000000 ) ) ;
#13489=ADVANCED_FACE ( 'NONE', ( #10161 ), #28867, .T. ) ;
#13491=ORIENTED_EDGE ( 'NONE', *, *, #29132, .T. ) ;
#13493=DIRECTION ( 'NONE',  ( -7.147005652999508048E-36, 5.642372883946980038E-36, 1.000000000000000000 ) ) ;
#13495=CARTESIAN_POINT ( 'NONE',  ( 6.000000000000000888, -1.859271017917181981E-14, -147.6636751345948255 ) ) ;
#13496=VERTEX_POINT ( 'NONE', #15077 ) ;
#13498=CARTESIAN_POINT ( 'NONE',  ( -3.175426480542816510, -5.500000000000057732, -99.87500000000000000 ) ) ;
#13501=CARTESIAN_POINT ( 'NONE',  ( 5.412658773652712085, -3.125000000000086153, -105.9330127018922667 ) ) ;
#13503=CARTESIAN_POINT ( 'NONE',  ( 2.799076333356274106E-14, 11.00000000000000000, -19.00000000000002132 ) ) ;
#13505=CARTESIAN_POINT ( 'NONE',  ( -4.763139720814407951, 2.749999999999946709, -166.2500000000000000 ) ) ;
#13506=CARTESIAN_POINT ( 'NONE',  ( -3.608439182435052128, -6.250000000000110134, -53.80801270189219565 ) ) ;
#13507=CARTESIAN_POINT ( 'NONE',  ( -5.999999999999963585, 1.780251999655701777E-13, -56.33632486540525264 ) ) ;
#13508=ORIENTED_EDGE ( 'NONE', *, *, #27367, .F. ) ;
#13510=CARTESIAN_POINT ( 'NONE',  ( 5.196152422706629359, -2.999999999999988898, -166.7113248654051745 ) ) ;
#13511=CARTESIAN_POINT ( 'NONE',  ( -2.775557561562891351E-14, -5.500000000000115463, -159.7500000000000568 ) ) ;
#13513=DIRECTION ( 'NONE',  ( 1.000000000000000000, -5.551115123125773458E-17, -1.260129944081490338E-35 ) ) ;
#13514=( BOUNDED_CURVE ( )  B_SPLINE_CURVE ( 2, ( #17390, #3362, #7827, #8452, #12496, #12791, #26705, #5988, #10311 ),
 .UNSPECIFIED., .F., .F. ) 
 B_SPLINE_CURVE_WITH_KNOTS ( ( 3, 2, 2, 2, 3 ),
 ( 0.3916666666666666630, 0.3925925925925926041, 0.3944444444444444309, 0.3962962962962963132, 0.3972222222222222543 ),
 .UNSPECIFIED. ) 
 CURVE ( )  GEOMETRIC_REPRESENTATION_ITEM ( )  RATIONAL_B_SPLINE_CURVE ( ( 0.9330127018922194093, 0.9330127018922194093, 1.000000000000000000, 0.8660254037844388186, 1.000000000000000000, 0.8660254037844388186, 1.000000000000000000, 0.9330127018922174109, 0.9330127018922194093 ) ) 
 REPRESENTATION_ITEM ( '' )  );
#13515=ADVANCED_FACE ( 'NONE', ( #26859 ), #21542, .T. ) ;
#13516=CARTESIAN_POINT ( 'NONE',  ( -2.775557561562891351E-14, -5.500000000000115463, -105.7500000000000142 ) ) ;
#13518=CARTESIAN_POINT ( 'NONE',  ( 6.000000000000000888, 1.743066579297358182E-13, -87.66367513459482552 ) ) ;
#13520=CARTESIAN_POINT ( 'NONE',  ( 3.175426480543072749, -5.500000000000105693, -98.12500000000004263 ) ) ;
#13523=ORIENTED_EDGE ( 'NONE', *, *, #4523, .T. ) ;
#13531=CARTESIAN_POINT ( 'NONE',  ( 3.608439182435180470, 6.249999999999982236, -91.19198729810783277 ) ) ;
#13534=ORIENTED_EDGE ( 'NONE', *, *, #22809, .F. ) ;
#13536=ORIENTED_EDGE ( 'NONE', *, *, #1921, .T. ) ;
#13537=VECTOR ( 'NONE', #30374, 1000.000000000000000 ) ;
#13538=CARTESIAN_POINT ( 'NONE',  ( -3.175426480542816510, -5.500000000000057732, -117.8750000000000142 ) ) ;
#13539=CARTESIAN_POINT ( 'NONE',  ( 2.775557561562891351E-14, 6.250000000000033751, -139.9330127018922383 ) ) ;
#13542=CARTESIAN_POINT ( 'NONE',  ( 7.216878364870455975, -6.409875621278545621E-14, -125.9419872981078186 ) ) ;
#13543=CARTESIAN_POINT ( 'NONE',  ( -3.608439182435052128, -6.250000000000110134, -177.4419872981078470 ) ) ;
#13548=CARTESIAN_POINT ( 'NONE',  ( 0.000000000000000000, 0.000000000000000000, 0.000000000000000000 ) ) ;
#13549=AXIS2_PLACEMENT_3D ( 'NONE', #6621, #13124, #20613 ) ;
#13551=DIRECTION ( 'NONE',  ( 1.000000000000000000, -5.551115123125773458E-17, 0.000000000000000000 ) ) ;
#13552=CARTESIAN_POINT ( 'NONE',  ( 3.608439182435180470, -6.249999999999997335, -61.69198729810783988 ) ) ;
#13553=CARTESIAN_POINT ( 'NONE',  ( -3.464101615137757051, -5.999999999999979572, -170.6636751345948255 ) ) ;
#13554=CARTESIAN_POINT ( 'NONE',  ( 6.350852961086080661, -9.614813431917819062E-14, -49.87500000000001421 ) ) ;
#13556=FACE_OUTER_BOUND ( 'NONE', #9545, .T. ) ;
#13557=( BOUNDED_CURVE ( )  B_SPLINE_CURVE ( 2, ( #10939, #3977, #13400, #20430, #29789, #25169, #18758, #1992, #4886 ),
 .UNSPECIFIED., .F., .T. ) 
 B_SPLINE_CURVE_WITH_KNOTS ( ( 3, 2, 2, 2, 3 ),
 ( 0.4750000000000000888, 0.4759259259259259744, 0.4777777777777777457, 0.4796296296296296280, 0.4805555555555555136 ),
 .UNSPECIFIED. ) 
 CURVE ( )  GEOMETRIC_REPRESENTATION_ITEM ( )  RATIONAL_B_SPLINE_CURVE ( ( 0.9330127018922194093, 0.9330127018922234061, 1.000000000000000000, 0.8660254037844388186, 1.000000000000000000, 0.8660254037844388186, 1.000000000000000000, 0.9330127018922234061, 0.9330127018922194093 ) ) 
 REPRESENTATION_ITEM ( '' )  );
#13559=CARTESIAN_POINT ( 'NONE',  ( 3.175426480543072749, 5.499999999999865885, -120.1250000000000284 ) ) ;
#13562=ORIENTED_EDGE ( 'NONE', *, *, #7947, .F. ) ;
#13571=CARTESIAN_POINT ( 'NONE',  ( 2.775557561562891351E-14, 6.250000000000033751, -113.5669872981078186 ) ) ;
#13572=CARTESIAN_POINT ( 'NONE',  ( 6.000000000000000888, -1.859271017917181981E-14, -109.5863248654052029 ) ) ;
#13575=ORIENTED_EDGE ( 'NONE', *, *, #399, .F. ) ;
#13577=CARTESIAN_POINT ( 'NONE',  ( 6.000000000000000888, -1.859271017917181981E-14, -126.0863248654052171 ) ) ;
#13579=CARTESIAN_POINT ( 'NONE',  ( 7.216878364870455975, -6.409875621278545621E-14, -145.4419872981078470 ) ) ;
#13580=CARTESIAN_POINT ( 'NONE',  ( -5.999999999999962697, 3.323446944526963891E-14, -157.4136751345948539 ) ) ;
#13588=CARTESIAN_POINT ( 'NONE',  ( 7.216878364870455975, -6.409875621278545621E-14, -68.30801270189220986 ) ) ;
#13590=CARTESIAN_POINT ( 'NONE',  ( 5.196152422706629359, -2.999999999999988898, -177.7886751345948539 ) ) ;
#13591=CARTESIAN_POINT ( 'NONE',  ( -20.99177011976446394, 10.49588505988223375, -1.500282997124227719E-34 ) ) ;
#13592=CARTESIAN_POINT ( 'NONE',  ( -5.999999999999962697, 3.323446944526963891E-14, -156.8363248654052313 ) ) ;
#13594=EDGE_CURVE ( 'NONE', #4124, #19006, #3264, .T. ) ;
#13595=CARTESIAN_POINT ( 'NONE',  ( 3.175426480543072749, -5.500000000000105693, -120.6250000000000284 ) ) ;
#13598=CARTESIAN_POINT ( 'NONE',  ( 4.763139720814407951, 2.750000000000002665, -52.75000000000002132 ) ) ;
#13599=CARTESIAN_POINT ( 'NONE',  ( 6.000000000000014211, -1.607695154586730180, -153.7306624327026157 ) ) ;
#13600=FACE_OUTER_BOUND ( 'NONE', #904, .T. ) ;
#13601=CARTESIAN_POINT ( 'NONE',  ( 3.464101615137757051, -5.999999999999979572, -162.9136751345947971 ) ) ;
#13610=CARTESIAN_POINT ( 'NONE',  ( -6.350852961085760029, -1.281975124255709124E-13, -140.6249999999999716 ) ) ;
#13613=ORIENTED_EDGE ( 'NONE', *, *, #17212, .F. ) ;
#13615=CARTESIAN_POINT ( 'NONE',  ( 6.350852961086080661, -9.614813431917819062E-14, -73.87500000000000000 ) ) ;
#13617=CARTESIAN_POINT ( 'NONE',  ( -2.511346088334902138, -10.71107091704336156, -30.45263927933804027 ) ) ;
#13618=CARTESIAN_POINT ( 'NONE',  ( -5.999999999999963585, -1.487416814333745711E-14, -134.3363248654052313 ) ) ;
#13620=CYLINDRICAL_SURFACE ( 'NONE', #2971, 6.000000000000000888 ) ;
#13622=EDGE_CURVE ( 'NONE', #15775, #9719, #27174, .T. ) ;
#13624=CARTESIAN_POINT ( 'NONE',  ( -6.350852961085760029, -1.281975124255709124E-13, -146.6250000000000284 ) ) ;
#13626=CARTESIAN_POINT ( 'NONE',  ( 5.412658773652712085, -3.125000000000086153, -164.4330127018922667 ) ) ;
#13628=TOROIDAL_SURFACE ( 'NONE', #12633, 9.999999999999998224, 1.000000000000000000 ) ;
#13629=CARTESIAN_POINT ( 'NONE',  ( 6.350852961086080661, -9.614813431917819062E-14, -87.37500000000005684 ) ) ;
#13633=CARTESIAN_POINT ( 'NONE',  ( 0.000000000000000000, 5.499999999999991118, -75.00000000000001421 ) ) ;
#13634=LINE ( 'NONE', #22981, #15214 ) ;
#13637=CARTESIAN_POINT ( 'NONE',  ( 0.000000000000000000, -5.999999999999991118, -71.53867513459482552 ) ) ;
#13641=CARTESIAN_POINT ( 'NONE',  ( 6.000000000000000888, 7.762456499804234384E-14, -139.5863248654051745 ) ) ;
#13642=( BOUNDED_CURVE ( )  B_SPLINE_CURVE ( 2, ( #25090, #30320, #18522 ),
 .UNSPECIFIED., .F., .F. ) 
 B_SPLINE_CURVE_WITH_KNOTS ( ( 3, 3 ),
 ( 0.01327334991652243112, 0.01388888888888888465 ),
 .UNSPECIFIED. ) 
 CURVE ( )  GEOMETRIC_REPRESENTATION_ITEM ( )  RATIONAL_B_SPLINE_CURVE ( ( 0.9626167487138490575, 0.9330127018922196314, 0.9330127018922194093 ) ) 
 REPRESENTATION_ITEM ( '' )  );
#13643=ORIENTED_EDGE ( 'NONE', *, *, #16133, .F. ) ;
#13645=CARTESIAN_POINT ( 'NONE',  ( 5.196152422706629359, -2.999999999999988898, -108.7886751345948397 ) ) ;
#13646=AXIS2_PLACEMENT_3D ( 'NONE', #18395, #8856, #4071 ) ;
#13652=( BOUNDED_CURVE ( )  B_SPLINE_CURVE ( 2, ( #6003, #24749, #27037, #15421, #7763, #20066, #12729, #29412, #29102 ),
 .UNSPECIFIED., .F., .T. ) 
 B_SPLINE_CURVE_WITH_KNOTS ( ( 3, 2, 2, 2, 3 ),
 ( 0.3305555555555556024, 0.3314814814814814881, 0.3333333333333333703, 0.3351851851851851416, 0.3361111111111110272 ),
 .UNSPECIFIED. ) 
 CURVE ( )  GEOMETRIC_REPRESENTATION_ITEM ( )  RATIONAL_B_SPLINE_CURVE ( ( 0.9330127018922194093, 0.9330127018922234061, 1.000000000000000000, 0.8660254037844388186, 1.000000000000000000, 0.8660254037844388186, 1.000000000000000000, 0.9330127018922234061, 0.9330127018922194093 ) ) 
 REPRESENTATION_ITEM ( '' )  );
#13653=AXIS2_PLACEMENT_3D ( 'NONE', #18701, #2393, #27714 ) ;
#13654=ORIENTED_EDGE ( 'NONE', *, *, #26369, .F. ) ;
#13656=CARTESIAN_POINT ( 'NONE',  ( 4.763139720814407951, -2.749999999999988454, -96.50000000000002842 ) ) ;
#13657=CARTESIAN_POINT ( 'NONE',  ( 5.412658773652739619, 3.124999999999988898, -104.1830127018922241 ) ) ;
#13660=CARTESIAN_POINT ( 'NONE',  ( 0.4053696738521634368, -11.00000000000001066, -31.00000000000002842 ) ) ;
#13662=CARTESIAN_POINT ( 'NONE',  ( -5.999999999999963585, -1.487416814333745711E-14, -165.8363248654052029 ) ) ;
#13664=FACE_OUTER_BOUND ( 'NONE', #5310, .T. ) ;
#13665=CARTESIAN_POINT ( 'NONE',  ( 4.763139720814407951, -2.749999999999988454, -173.0000000000000568 ) ) ;
#13667=CARTESIAN_POINT ( 'NONE',  ( -6.350852961085760029, -1.281975124255709124E-13, -161.6250000000000284 ) ) ;
#13669=CARTESIAN_POINT ( 'NONE',  ( 3.175426480543072749, 5.499999999999865885, -109.6249999999999716 ) ) ;
#13670=CARTESIAN_POINT ( 'NONE',  ( 6.000000000000000888, -1.607695154586752384, -159.1533121635129646 ) ) ;
#13671=CARTESIAN_POINT ( 'NONE',  ( -3.464101615137757051, -5.999999999999979572, -166.1636751345947687 ) ) ;
#13672=CARTESIAN_POINT ( 'NONE',  ( 3.175426480543072749, -5.500000000000105693, -95.12500000000002842 ) ) ;
#13678=DIRECTION ( 'NONE',  ( 1.000000000000000000, -5.551115123125773458E-17, -1.260129944081490338E-35 ) ) ;
#13684=CARTESIAN_POINT ( 'NONE',  ( -5.412658773652684552, -3.125000000000099920, -86.06698729810780435 ) ) ;
#13686=EDGE_LOOP ( 'NONE', ( #22622, #30310, #11536, #13807 ) ) ;
#13689=SHAPE_REPRESENTATION ( 'Clamp rod', ( #18805 ), #1599 ) ;
#13693=ORIENTED_EDGE ( 'NONE', *, *, #15537, .T. ) ;
#13694=EDGE_CURVE ( 'NONE', #1235, #152, #25243, .T. ) ;
#13695=CARTESIAN_POINT ( 'NONE',  ( 4.763139720814407951, -2.749999999999988454, -122.0000000000000000 ) ) ;
#13697=EDGE_CURVE ( 'NONE', #8975, #856, #12948, .T. ) ;
#13698=CARTESIAN_POINT ( 'NONE',  ( 2.775557561562891351E-14, 6.250000000000033751, -127.9330127018922809 ) ) ;
#13699=ORIENTED_EDGE ( 'NONE', *, *, #22857, .F. ) ;
#13700=DIRECTION ( 'NONE',  ( -7.147005652999508048E-36, 5.642372883946980038E-36, 1.000000000000000000 ) ) ;
#13701=CARTESIAN_POINT ( 'NONE',  ( 2.775557561562891351E-14, -6.250000000000061284, -171.3169872981078470 ) ) ;
#13702=CARTESIAN_POINT ( 'NONE',  ( 7.216878364870455975, -6.409875621278545621E-14, -173.9419872981078470 ) ) ;
#13705=FACE_OUTER_BOUND ( 'NONE', #8494, .T. ) ;
#13706=CARTESIAN_POINT ( 'NONE',  ( 0.000000000000000000, 0.000000000000000000, 0.000000000000000000 ) ) ;
#13710=CARTESIAN_POINT ( 'NONE',  ( 5.412658773652712085, -3.125000000000086153, -76.56698729810784698 ) ) ;
#13711=CARTESIAN_POINT ( 'NONE',  ( 2.775557561562891351E-14, -6.250000000000061284, -60.31698729810780435 ) ) ;
#13712=CARTESIAN_POINT ( 'NONE',  ( -3.608439182435052128, -6.250000000000110134, -181.3080127018922383 ) ) ;
#13714=CARTESIAN_POINT ( 'NONE',  ( 3.464101615137757051, -5.999999999999979572, -153.3363248654051745 ) ) ;
#13716=CARTESIAN_POINT ( 'NONE',  ( 3.175426480543072749, 5.499999999999865885, -118.6250000000000284 ) ) ;
#13717=CARTESIAN_POINT ( 'NONE',  ( -6.350852961085760029, -1.281975124255709124E-13, -155.6249999999999716 ) ) ;
#13718=CARTESIAN_POINT ( 'NONE',  ( -5.999999999999963585, -1.487416814333745711E-14, -137.9136751345947971 ) ) ;
#13722=CARTESIAN_POINT ( 'NONE',  ( 5.999999999999949374, 1.607695154586804565, -123.0193375672974696 ) ) ;
#13727=CARTESIAN_POINT ( 'NONE',  ( -5.196152422706601826, 2.999999999999975131, -121.5386751345948255 ) ) ;
#13729=CARTESIAN_POINT ( 'NONE',  ( 7.216878364870455975, -6.409875621278545621E-14, -113.9419872981078328 ) ) ;
#13733=CARTESIAN_POINT ( 'NONE',  ( -6.000000000000000888, 1.067854986875958443E-15, 7.560779664488942560E-35 ) ) ;
#13735=ADVANCED_FACE ( 'NONE', ( #17697 ), #16019, .T. ) ;
#13736=CARTESIAN_POINT ( 'NONE',  ( 2.775557561562891351E-14, -6.250000000000061284, -49.81698729810779724 ) ) ;
#13737=CARTESIAN_POINT ( 'NONE',  ( 5.412658773652712085, -3.125000000000086153, -147.0669872981078470 ) ) ;
#13741=CARTESIAN_POINT ( 'NONE',  ( -7.216878364870328078, 0.000000000000000000, -69.05801270189226670 ) ) ;
#13742=( BOUNDED_CURVE ( )  B_SPLINE_CURVE ( 2, ( #395, #19163, #704, #2698, #7903, #26484, #21466, #17318, #7320 ),
 .UNSPECIFIED., .F., .T. ) 
 B_SPLINE_CURVE_WITH_KNOTS ( ( 3, 2, 2, 2, 3 ),
 ( 0.9583333333333332593, 0.9592592592592592560, 0.9611111111111111382, 0.9629629629629629095, 0.9638888888888889062 ),
 .UNSPECIFIED. ) 
 CURVE ( )  GEOMETRIC_REPRESENTATION_ITEM ( )  RATIONAL_B_SPLINE_CURVE ( ( 0.9330127018922194093, 0.9330127018922154125, 1.000000000000000000, 0.8660254037844388186, 1.000000000000000000, 0.8660254037844388186, 1.000000000000000000, 0.9330127018922154125, 0.9330127018922194093 ) ) 
 REPRESENTATION_ITEM ( '' )  );
#13744=FACE_OUTER_BOUND ( 'NONE', #25887, .T. ) ;
#13745=CARTESIAN_POINT ( 'NONE',  ( -3.464101615137725076, 5.999999999999979572, -73.66367513459483973 ) ) ;
#13746=CARTESIAN_POINT ( 'NONE',  ( 5.999999999999999112, 2.951592740943527306E-14, -155.1636751345948539 ) ) ;
#13750=CARTESIAN_POINT ( 'NONE',  ( 3.175426480543072749, -5.500000000000105693, -123.6250000000000426 ) ) ;
#13753=CARTESIAN_POINT ( 'NONE',  ( 5.196152422706629359, 3.000000000000002665, -143.0386751345948255 ) ) ;
#13755=CARTESIAN_POINT ( 'NONE',  ( 3.175426480543072749, -5.500000000000105693, -51.62500000000002842 ) ) ;
#13756=CARTESIAN_POINT ( 'NONE',  ( 0.000000000000000000, -5.999999999999991118, -154.9613248654052597 ) ) ;
#13757=CARTESIAN_POINT ( 'NONE',  ( -5.999999999999963585, 1.780251999655701777E-13, -77.33632486540524553 ) ) ;
#13767=CARTESIAN_POINT ( 'NONE',  ( -4.763139720814407951, 2.749999999999946709, -139.2499999999999716 ) ) ;
#13770=ORIENTED_EDGE ( 'NONE', *, *, #2712, .T. ) ;
#13772=ORIENTED_EDGE ( 'NONE', *, *, #27082, .F. ) ;
#13774=CARTESIAN_POINT ( 'NONE',  ( -6.350852961085760029, -1.281975124255709124E-13, -67.12500000000002842 ) ) ;
#13776=CARTESIAN_POINT ( 'NONE',  ( -3.608439182435115633, 6.249999999999965361, -87.30801270189223828 ) ) ;
#13778=EDGE_LOOP ( 'NONE', ( #27227, #11341, #10758, #26515 ) ) ;
#13783=CARTESIAN_POINT ( 'NONE',  ( 4.763139720814407951, 2.750000000000002665, -150.2500000000000000 ) ) ;
#13785=CARTESIAN_POINT ( 'NONE',  ( 0.000000000000000000, 5.499999999999991118, -142.5000000000000284 ) ) ;
#13786=CARTESIAN_POINT ( 'NONE',  ( -3.608439182435052128, -6.250000000000110134, -160.3080127018922383 ) ) ;
#13787=CARTESIAN_POINT ( 'NONE',  ( -5.999999999999963585, -1.487416814333745711E-14, -123.8363248654052171 ) ) ;
#13789=CARTESIAN_POINT ( 'NONE',  ( 3.175426480543072749, -5.500000000000105693, -78.62500000000001421 ) ) ;
#13791=CARTESIAN_POINT ( 'NONE',  ( 3.175426480543072749, 5.499999999999865885, -72.12500000000005684 ) ) ;
#13792=CARTESIAN_POINT ( 'NONE',  ( -5.999999999999963585, 8.134310703387671600E-14, -120.8363248654052171 ) ) ;
#13796=EDGE_CURVE ( 'NONE', #25418, #28105, #13557, .T. ) ;
#13799=EDGE_CURVE ( 'NONE', #19518, #12143, #2317, .T. ) ;
#13800=CARTESIAN_POINT ( 'NONE',  ( 6.000000000000000888, 7.762456499804234384E-14, -119.1636751345948113 ) ) ;
#13801=CARTESIAN_POINT ( 'NONE',  ( 6.000000000000000888, -1.859271017917181981E-14, -170.1636751345948539 ) ) ;
#13802=ORIENTED_EDGE ( 'NONE', *, *, #17887, .F. ) ;
#13806=CARTESIAN_POINT ( 'NONE',  ( 5.999999999999949374, 1.607695154586804565, -157.5193375672974128 ) ) ;
#13807=ORIENTED_EDGE ( 'NONE', *, *, #29482, .F. ) ;
#13811=CARTESIAN_POINT ( 'NONE',  ( -3.175426480542816510, -5.500000000000057732, -90.87500000000001421 ) ) ;
#13813=CARTESIAN_POINT ( 'NONE',  ( -5.412658773652739619, 3.124999999999975131, -108.1830127018922383 ) ) ;
#13817=CARTESIAN_POINT ( 'NONE',  ( -3.175426480542816510, -5.500000000000057732, -164.3750000000000568 ) ) ;
#13818=CARTESIAN_POINT ( 'NONE',  ( 4.758024543289591790, -9.918640242984132271, -28.66037974350899376 ) ) ;
#13819=ORIENTED_EDGE ( 'NONE', *, *, #23392, .T. ) ;
#13820=CARTESIAN_POINT ( 'NONE',  ( 6.000000000000000888, -1.859271017917181981E-14, -47.16367513459483263 ) ) ;
#13822=CARTESIAN_POINT ( 'NONE',  ( 6.350852961086080661, -9.614813431917819062E-14, -172.8750000000000284 ) ) ;
#13823=LINE ( 'NONE', #27888, #7149 ) ;
#13824=CARTESIAN_POINT ( 'NONE',  ( -3.175426480542816510, 5.499999999999865885, -166.3750000000000568 ) ) ;
#13826=CARTESIAN_POINT ( 'NONE',  ( -3.175426480542816066, 5.499999999999865885, -100.3749999999999858 ) ) ;
#13829=CARTESIAN_POINT ( 'NONE',  ( 3.175426480543072749, 5.499999999999865885, -99.12500000000005684 ) ) ;
#13832=ORIENTED_EDGE ( 'NONE', *, *, #13476, .F. ) ;
#13840=( BOUNDED_CURVE ( )  B_SPLINE_CURVE ( 2, ( #28280, #20947, #18504, #7257, #27827, #5383, #28722, #14936, #9725 ),
 .UNSPECIFIED., .F., .T. ) 
 B_SPLINE_CURVE_WITH_KNOTS ( ( 3, 2, 2, 2, 3 ),
 ( 0.8694444444444444642, 0.8703703703703703498, 0.8722222222222222321, 0.8740740740740741144, 0.8750000000000000000 ),
 .UNSPECIFIED. ) 
 CURVE ( )  GEOMETRIC_REPRESENTATION_ITEM ( )  RATIONAL_B_SPLINE_CURVE ( ( 0.9330127018922194093, 0.9330127018922234061, 1.000000000000000000, 0.8660254037844388186, 1.000000000000000000, 0.8660254037844388186, 1.000000000000000000, 0.9330127018922194093, 0.9330127018922194093 ) ) 
 REPRESENTATION_ITEM ( '' )  );
#13842=CARTESIAN_POINT ( 'NONE',  ( 6.000000000000000888, 1.743066579297358182E-13, -112.5863248654052029 ) ) ;
#13849=ORIENTED_EDGE ( 'NONE', *, *, #18882, .F. ) ;
#13852=CARTESIAN_POINT ( 'NONE',  ( -3.175426480542816510, 5.499999999999865885, -113.8750000000000000 ) ) ;
#13854=CARTESIAN_POINT ( 'NONE',  ( -3.608439182435115633, 6.249999999999965361, -127.8080127018922383 ) ) ;
#13855=ORIENTED_EDGE ( 'NONE', *, *, #2331, .T. ) ;
#13856=CARTESIAN_POINT ( 'NONE',  ( 2.775557561562891351E-14, 6.250000000000033751, -170.5669872981078186 ) ) ;
#13857=CARTESIAN_POINT ( 'NONE',  ( 3.608439182435180470, -6.249999999999997335, -175.6919872981078186 ) ) ;
#13863=CARTESIAN_POINT ( 'NONE',  ( -5.999999999999963585, 8.134310703387671600E-14, -136.4136751345948255 ) ) ;
#13864=AXIS2_PLACEMENT_3D ( 'NONE', #16629, #23808, #26244 ) ;
#13865=CARTESIAN_POINT ( 'NONE',  ( 0.000000000000000000, -5.999999999999991118, -150.4613248654052029 ) ) ;
#13867=CARTESIAN_POINT ( 'NONE',  ( -3.608439182435115633, 6.249999999999965361, -77.44198729810777593 ) ) ;
#13868=CARTESIAN_POINT ( 'NONE',  ( -3.608439182435052128, -6.250000000000110134, -61.94198729810783277 ) ) ;
#13869=CARTESIAN_POINT ( 'NONE',  ( 3.175426480543072749, 5.499999999999865885, -48.12500000000000000 ) ) ;
#13870=CARTESIAN_POINT ( 'NONE',  ( 6.000000000000000888, 1.743066579297358182E-13, -111.0863248654051887 ) ) ;
#13871=CARTESIAN_POINT ( 'NONE',  ( 3.464101615137757051, -5.999999999999979572, -47.41367513459483973 ) ) ;
#13873=CARTESIAN_POINT ( 'NONE',  ( -3.175426480542816510, -5.500000000000057732, -125.3749999999999858 ) ) ;
#13875=CARTESIAN_POINT ( 'NONE',  ( -2.910268709469104432E-14, -11.00000000000000000, -14.99152654425661702 ) ) ;
#13878=EDGE_CURVE ( 'NONE', #13234, #26278, #29568, .T. ) ;
#13882=AXIS2_PLACEMENT_3D ( 'NONE', #1918, #29713, #6681 ) ;
#13884=CARTESIAN_POINT ( 'NONE',  ( 0.000000000000000000, 0.000000000000000000, 0.000000000000000000 ) ) ;
#13887=CARTESIAN_POINT ( 'NONE',  ( 2.775557561562891351E-14, -6.250000000000061284, -109.8169872981078470 ) ) ;
#13892=ORIENTED_EDGE ( 'NONE', *, *, #24669, .F. ) ;
#13893=CARTESIAN_POINT ( 'NONE',  ( 5.196152422706629359, 3.000000000000002665, -141.5386751345948255 ) ) ;
#13895=CARTESIAN_POINT ( 'NONE',  ( -7.216878364870328078, 0.000000000000000000, -138.6919872981077901 ) ) ;
#13896=CIRCLE ( 'NONE', #6977, 10.00000000000001421 ) ;
#13901=CARTESIAN_POINT ( 'NONE',  ( 7.216878364870455975, -6.409875621278545621E-14, -66.80801270189228092 ) ) ;
#13904=CARTESIAN_POINT ( 'NONE',  ( -5.196152422706573404, -3.000000000000002665, -70.28867513459479710 ) ) ;
#13905=CARTESIAN_POINT ( 'NONE',  ( 6.000000000000000888, -3.330669073875464691E-16, -7.560779664488942560E-35 ) ) ;
#13907=CARTESIAN_POINT ( 'NONE',  ( 6.000000000000000888, 1.743066579297358182E-13, -66.66367513459481131 ) ) ;
#13909=CARTESIAN_POINT ( 'NONE',  ( 0.000000000000000000, 5.499999999999991118, -121.5000000000000568 ) ) ;
#13910=CARTESIAN_POINT ( 'NONE',  ( -7.216878364870328078, 0.000000000000000000, -145.5580127018922667 ) ) ;
#13912=ORIENTED_EDGE ( 'NONE', *, *, #1538, .F. ) ;
#13914=CARTESIAN_POINT ( 'NONE',  ( -3.175426480542816066, -5.500000000000057732, -56.37500000000004263 ) ) ;
#13915=CARTESIAN_POINT ( 'NONE',  ( -5.999999999999963585, -1.487416814333745711E-14, -133.4136751345948255 ) ) ;
#13916=EDGE_CURVE ( 'NONE', #6411, #22196, #4268, .T. ) ;
#13918=ORIENTED_EDGE ( 'NONE', *, *, #21545, .T. ) ;
#13921=CARTESIAN_POINT ( 'NONE',  ( 2.775557561562891351E-14, -6.250000000000061284, -105.3169872981078470 ) ) ;
#13925=B_SPLINE_CURVE_WITH_KNOTS ( 'NONE', 2,
 ( #13875, #6758, #16027 ),
 .UNSPECIFIED., .F., .F.,
 ( 3, 3 ),
 ( 0.000000000000000000, 1.000000000000000000 ),
 .UNSPECIFIED. ) ;
#13926=CARTESIAN_POINT ( 'NONE',  ( 6.350852961086080661, -9.614813431917819062E-14, -136.8750000000000568 ) ) ;
#13930=ORIENTED_EDGE ( 'NONE', *, *, #24287, .T. ) ;
#13931=CARTESIAN_POINT ( 'NONE',  ( 4.763139720814407951, -2.749999999999988454, -68.00000000000000000 ) ) ;
#13933=CARTESIAN_POINT ( 'NONE',  ( -6.000000000000023093, 1.607695154586625819, -140.4033121635129930 ) ) ;
#13934=CARTESIAN_POINT ( 'NONE',  ( 5.412658773652739619, 3.124999999999988898, -89.18301270189220986 ) ) ;
#13935=AXIS2_PLACEMENT_3D ( 'NONE', #6552, #2108, #20542 ) ;
#13938=DIRECTION ( 'NONE',  ( -7.147005652999508048E-36, 5.642372883946980038E-36, 1.000000000000000000 ) ) ;
#13940=CARTESIAN_POINT ( 'NONE',  ( 3.175426480543072749, 5.499999999999865885, -150.1250000000000284 ) ) ;
#13942=CARTESIAN_POINT ( 'NONE',  ( -4.763139720814407951, -2.750000000000016431, -139.0000000000000000 ) ) ;
#13943=CARTESIAN_POINT ( 'NONE',  ( -3.608439182435052128, -6.250000000000110134, -157.3080127018922383 ) ) ;
#13946=CARTESIAN_POINT ( 'NONE',  ( 4.763139720814407951, -2.749999999999988454, -81.50000000000001421 ) ) ;
#13947=DIRECTION ( 'NONE',  ( -7.147005652999508048E-36, 5.642372883946980038E-36, 1.000000000000000000 ) ) ;
#13948=CARTESIAN_POINT ( 'NONE',  ( -6.350852961085760029, -1.281975124255709124E-13, -71.62500000000005684 ) ) ;
#13953=CARTESIAN_POINT ( 'NONE',  ( 6.000000000000000888, -1.859271017917181981E-14, -114.0863248654052029 ) ) ;
#13954=CARTESIAN_POINT ( 'NONE',  ( -5.999999999999963585, -1.487416814333745711E-14, -124.4136751345948255 ) ) ;
#13956=CARTESIAN_POINT ( 'NONE',  ( 3.464101615137852974, 5.999999999999884537, -133.9136751345947971 ) ) ;
#13958=CARTESIAN_POINT ( 'NONE',  ( -5.999999999999963585, 1.780251999655701777E-13, -94.41367513459482552 ) ) ;
#13961=ORIENTED_EDGE ( 'NONE', *, *, #12845, .T. ) ;
#13965=CARTESIAN_POINT ( 'NONE',  ( 0.000000000000000000, 5.999999999999977796, -179.7113248654052029 ) ) ;
#13967=ORIENTED_EDGE ( 'NONE', *, *, #19213, .F. ) ;
#13970=CARTESIAN_POINT ( 'NONE',  ( 3.175426480543072749, -5.500000000000105693, -92.12500000000001421 ) ) ;
#13971=CARTESIAN_POINT ( 'NONE',  ( 7.216878364870455975, -6.409875621278545621E-14, -104.3080127018922525 ) ) ;
#13974=EDGE_CURVE ( 'NONE', #28542, #20142, #25074, .T. ) ;
#13976=CARTESIAN_POINT ( 'NONE',  ( 4.874391507318805772, -9.861790235658062898, -28.50395189876375213 ) ) ;
#13977=ORIENTED_EDGE ( 'NONE', *, *, #24803, .T. ) ;
#13980=CARTESIAN_POINT ( 'NONE',  ( 4.763139720814407951, 2.750000000000002665, -168.2500000000000000 ) ) ;
#13981=CARTESIAN_POINT ( 'NONE',  ( -5.196152422706573404, -3.000000000000002665, -80.78867513459486815 ) ) ;
#13982=CARTESIAN_POINT ( 'NONE',  ( -4.763139720814407951, -2.750000000000016431, -164.5000000000000284 ) ) ;
#13984=CARTESIAN_POINT ( 'NONE',  ( 6.350852961086080661, -9.614813431917819062E-14, -99.37499999999998579 ) ) ;
#13985=CARTESIAN_POINT ( 'NONE',  ( 0.000000000000000000, 0.000000000000000000, 0.000000000000000000 ) ) ;
#13986=CARTESIAN_POINT ( 'NONE',  ( -5.999999999999963585, -1.487416814333745711E-14, -137.9136751345947971 ) ) ;
#13987=CARTESIAN_POINT ( 'NONE',  ( -3.175426480542816510, -5.500000000000057732, -96.87499999999997158 ) ) ;
#13988=EDGE_CURVE ( 'NONE', #8626, #5164, #16696, .T. ) ;
#13992=EDGE_LOOP ( 'NONE', ( #15890, #3999, #26253, #25813 ) ) ;
#14000=CARTESIAN_POINT ( 'NONE',  ( 6.000000000000052403, -1.607695154586662678, -169.6533121635129646 ) ) ;
#14002=ORIENTED_EDGE ( 'NONE', *, *, #20529, .F. ) ;
#14003=CARTESIAN_POINT ( 'NONE',  ( 6.000000000000000888, -1.859271017917181981E-14, -141.0863248654051745 ) ) ;
#14005=CARTESIAN_POINT ( 'NONE',  ( 4.763139720814407951, 2.750000000000002665, -117.2500000000000142 ) ) ;
#14007=CARTESIAN_POINT ( 'NONE',  ( 3.608439182435180470, 6.249999999999982236, -129.5580127018922383 ) ) ;
#14008=VERTEX_POINT ( 'NONE', #13358 ) ;
#14010=CARTESIAN_POINT ( 'NONE',  ( -5.412658773652739619, 3.124999999999975131, -168.8169872981077901 ) ) ;
#14012=ADVANCED_FACE ( 'NONE', ( #19933 ), #8560, .T. ) ;
#14014=( BOUNDED_CURVE ( )  B_SPLINE_CURVE ( 2, ( #12129, #5447, #7174, #24200, #709, #23768, #5300, #16588, #14567 ),
 .UNSPECIFIED., .F., .T. ) 
 B_SPLINE_CURVE_WITH_KNOTS ( ( 3, 2, 2, 2, 3 ),
 ( 0.3361111111111110827, 0.3370370370370370239, 0.3388888888888889062, 0.3407407407407407329, 0.3416666666666666741 ),
 .UNSPECIFIED. ) 
 CURVE ( )  GEOMETRIC_REPRESENTATION_ITEM ( )  RATIONAL_B_SPLINE_CURVE ( ( 0.9330127018922194093, 0.9330127018922174109, 1.000000000000000000, 0.8660254037844388186, 1.000000000000000000, 0.8660254037844388186, 1.000000000000000000, 0.9330127018922194093, 0.9330127018922194093 ) ) 
 REPRESENTATION_ITEM ( '' )  );
#14016=CARTESIAN_POINT ( 'NONE',  ( -5.999999999999963585, -1.487416814333745711E-14, -134.9136751345948255 ) ) ;
#14020=CARTESIAN_POINT ( 'NONE',  ( 5.412658773652712085, -3.125000000000086153, -177.9330127018922099 ) ) ;
#14021=CYLINDRICAL_SURFACE ( 'NONE', #19986, 6.000000000000000888 ) ;
#14026=CARTESIAN_POINT ( 'NONE',  ( -4.763139720814407951, -2.750000000000016431, -122.5000000000000568 ) ) ;
#14027=( BOUNDED_CURVE ( )  B_SPLINE_CURVE ( 2, ( #15449, #22489, #22329, #12992, #8814, #6030, #25218, #18199, #4186 ),
 .UNSPECIFIED., .F., .T. ) 
 B_SPLINE_CURVE_WITH_KNOTS ( ( 3, 2, 2, 2, 3 ),
 ( 0.9194444444444443976, 0.9203703703703703942, 0.9222222222222222765, 0.9240740740740740478, 0.9250000000000000444 ),
 .UNSPECIFIED. ) 
 CURVE ( )  GEOMETRIC_REPRESENTATION_ITEM ( )  RATIONAL_B_SPLINE_CURVE ( ( 0.9330127018922194093, 0.9330127018922154125, 1.000000000000000000, 0.8660254037844388186, 1.000000000000000000, 0.8660254037844388186, 1.000000000000000000, 0.9330127018922154125, 0.9330127018922194093 ) ) 
 REPRESENTATION_ITEM ( '' )  );
#14029=CARTESIAN_POINT ( 'NONE',  ( 5.999999999999949374, 1.607695154586804565, -166.5193375672974128 ) ) ;
#14034=FACE_BOUND ( 'NONE', #15173, .T. ) ;
#14037=CARTESIAN_POINT ( 'NONE',  ( 0.000000000000000000, -5.999999999999991118, -115.0386751345948682 ) ) ;
#14039=CARTESIAN_POINT ( 'NONE',  ( 3.608439182435180470, -6.249999999999997335, -109.6919872981078186 ) ) ;
#14043=ORIENTED_EDGE ( 'NONE', *, *, #11945, .T. ) ;
#14046=CARTESIAN_POINT ( 'NONE',  ( -5.412658773652684552, -3.125000000000099920, -135.5669872981078470 ) ) ;
#14052=CARTESIAN_POINT ( 'NONE',  ( -6.000000000000000888, 1.067854986875958443E-15, 7.560779664488942560E-35 ) ) ;
#14053=CYLINDRICAL_SURFACE ( 'NONE', #25495, 6.000000000000000888 ) ;
#14057=DIRECTION ( 'NONE',  ( -7.147005652999508048E-36, 5.642372883946980038E-36, 1.000000000000000000 ) ) ;
#14058=AXIS2_PLACEMENT_3D ( 'NONE', #8965, #27366, #27215 ) ;
#14062=LINE ( 'NONE', #11445, #6414 ) ;
#14063=EDGE_CURVE ( 'NONE', #2929, #269, #13742, .T. ) ;
#14065=CARTESIAN_POINT ( 'NONE',  ( 5.412658773652739619, 3.124999999999988898, -143.1830127018922667 ) ) ;
#14066=CARTESIAN_POINT ( 'NONE',  ( -5.999999999999957367, 1.607695154586737507, -148.4806624327026157 ) ) ;
#14068=DIRECTION ( 'NONE',  ( -5.551115123125774074E-17, -1.000000000000000000, -6.394689268473234689E-36 ) ) ;
#14070=CARTESIAN_POINT ( 'NONE',  ( -3.175426480542816066, -5.500000000000057732, -57.87500000000004974 ) ) ;
#14071=CYLINDRICAL_SURFACE ( 'NONE', #25194, 6.000000000000000888 ) ;
#14072=CARTESIAN_POINT ( 'NONE',  ( 5.196152422706629359, -2.999999999999988898, -178.7113248654052029 ) ) ;
#14073=ORIENTED_EDGE ( 'NONE', *, *, #9650, .F. ) ;
#14077=CARTESIAN_POINT ( 'NONE',  ( -3.608439182435052128, -6.250000000000110134, -102.4419872981078328 ) ) ;
#14080=CARTESIAN_POINT ( 'NONE',  ( -5.999999999999963585, -1.487416814333745711E-14, -172.4136751345948255 ) ) ;
#14082=CARTESIAN_POINT ( 'NONE',  ( -4.763139720814407951, 2.749999999999946709, -134.7500000000000284 ) ) ;
#14084=ORIENTED_EDGE ( 'NONE', *, *, #21167, .F. ) ;
#14086=CARTESIAN_POINT ( 'NONE',  ( 4.763139720814407951, 2.750000000000002665, -61.75000000000002842 ) ) ;
#14087=EDGE_CURVE ( 'NONE', #20687, #2600, #14871, .T. ) ;
#14088=CARTESIAN_POINT ( 'NONE',  ( 0.000000000000000000, 5.999999999999977796, -66.28867513459479710 ) ) ;
#14090=CARTESIAN_POINT ( 'NONE',  ( 5.412658773652739619, 3.124999999999988898, -90.68301270189226670 ) ) ;
#14092=VECTOR ( 'NONE', #22233, 1000.000000000000000 ) ;
#14096=AXIS2_PLACEMENT_3D ( 'NONE', #16549, #4820, #212 ) ;
#14097=CARTESIAN_POINT ( 'NONE',  ( -2.775557561562891351E-14, -5.500000000000115463, -149.2500000000000000 ) ) ;
#14099=CARTESIAN_POINT ( 'NONE',  ( 3.175426480543072749, 5.499999999999865885, -138.1250000000000284 ) ) ;
#14100=CARTESIAN_POINT ( 'NONE',  ( 3.608439182435180470, 6.249999999999982236, -162.5580127018921814 ) ) ;
#14101=CARTESIAN_POINT ( 'NONE',  ( -5.196152422706601826, 2.999999999999975131, -89.46132486540525974 ) ) ;
#14102=CARTESIAN_POINT ( 'NONE',  ( 6.350852961086080661, -9.614813431917819062E-14, -75.37500000000002842 ) ) ;
#14104=CARTESIAN_POINT ( 'NONE',  ( -3.175426480542816510, 5.499999999999865885, -62.87500000000001421 ) ) ;
#14106=CARTESIAN_POINT ( 'NONE',  ( 6.000000000000000888, -1.607695154586752384, -114.1533121635129930 ) ) ;
#14107=CARTESIAN_POINT ( 'NONE',  ( -5.196152422706573404, -3.000000000000002665, -175.2886751345948539 ) ) ;
#14110=CYLINDRICAL_SURFACE ( 'NONE', #1318, 6.000000000000000888 ) ;
#14112=CYLINDRICAL_SURFACE ( 'NONE', #24290, 6.000000000000000888 ) ;
#14113=( BOUNDED_CURVE ( )  B_SPLINE_CURVE ( 2, ( #13915, #28426, #9567, #14213, #5230, #16952, #7255, #12503, #2635 ),
 .UNSPECIFIED., .F., .T. ) 
 B_SPLINE_CURVE_WITH_KNOTS ( ( 3, 2, 2, 2, 3 ),
 ( 0.3583333333333333370, 0.3592592592592592782, 0.3611111111111111049, 0.3629629629629629872, 0.3638888888888889284 ),
 .UNSPECIFIED. ) 
 CURVE ( )  GEOMETRIC_REPRESENTATION_ITEM ( )  RATIONAL_B_SPLINE_CURVE ( ( 0.9330127018922194093, 0.9330127018922194093, 1.000000000000000000, 0.8660254037844388186, 1.000000000000000000, 0.8660254037844388186, 1.000000000000000000, 0.9330127018922174109, 0.9330127018922194093 ) ) 
 REPRESENTATION_ITEM ( '' )  );
#14114=ORIENTED_EDGE ( 'NONE', *, *, #17517, .F. ) ;
#14118=CARTESIAN_POINT ( 'NONE',  ( -3.175426480542816510, -5.500000000000057732, -153.8750000000000000 ) ) ;
#14119=CARTESIAN_POINT ( 'NONE',  ( -6.000000000000007105, -1.607695154586655129, -85.34668783648703538 ) ) ;
#14122=VERTEX_POINT ( 'NONE', #10088 ) ;
#14123=CARTESIAN_POINT ( 'NONE',  ( 4.763139720814407951, 2.750000000000002665, -93.25000000000000000 ) ) ;
#14125=CARTESIAN_POINT ( 'NONE',  ( 3.608439182435180470, -6.249999999999997335, -107.5580127018922667 ) ) ;
#14128=AXIS2_PLACEMENT_3D ( 'NONE', #23716, #23569, #28738 ) ;
#14129=CARTESIAN_POINT ( 'NONE',  ( 0.000000000000000000, 5.499999999999991118, -163.5000000000000284 ) ) ;
#14130=CARTESIAN_POINT ( 'NONE',  ( 6.000000000000000888, -1.607695154586752384, -63.15331216351300014 ) ) ;
#14134=CARTESIAN_POINT ( 'NONE',  ( 4.763139720814407951, 2.750000000000002665, -174.2500000000000284 ) ) ;
#14135=DIRECTION ( 'NONE',  ( 1.000000000000000000, -5.551115123125773458E-17, -1.260129944081490338E-35 ) ) ;
#14136=CARTESIAN_POINT ( 'NONE',  ( -3.175426480542816510, -5.500000000000057732, -153.8750000000000000 ) ) ;
#14138=CARTESIAN_POINT ( 'NONE',  ( -3.175426480542816066, 5.499999999999865885, -98.87499999999998579 ) ) ;
#14139=CARTESIAN_POINT ( 'NONE',  ( -5.999999999999956479, -1.607695154586745057, -159.7693375672974412 ) ) ;
#14141=CARTESIAN_POINT ( 'NONE',  ( -3.175426480542816510, -5.500000000000057732, -87.87500000000000000 ) ) ;
#14147=CARTESIAN_POINT ( 'NONE',  ( -6.000000000000000888, 1.067854986875958443E-15, 7.560779664488942560E-35 ) ) ;
#14151=FACE_OUTER_BOUND ( 'NONE', #20241, .T. ) ;
#14153=ADVANCED_FACE ( 'NONE', ( #6643 ), #22938, .T. ) ;
#14155=CARTESIAN_POINT ( 'NONE',  ( -5.196152422706573404, -3.000000000000002665, -141.7113248654052313 ) ) ;
#14157=ORIENTED_EDGE ( 'NONE', *, *, #9261, .T. ) ;
#14158=CARTESIAN_POINT ( 'NONE',  ( -6.350852961085760029, -1.281975124255709124E-13, -110.6249999999999858 ) ) ;
#14161=CARTESIAN_POINT ( 'NONE',  ( 7.216878364870455975, -6.409875621278545621E-14, -132.8080127018922667 ) ) ;
#14164=CARTESIAN_POINT ( 'NONE',  ( 2.775557561562891351E-14, -6.250000000000061284, -165.3169872981078470 ) ) ;
#14168=CARTESIAN_POINT ( 'NONE',  ( -5.999999999999919176, 1.607695154586804565, -95.40331216351297883 ) ) ;
#14170=DIRECTION ( 'NONE',  ( 1.000000000000000000, -5.551115123125773458E-17, -1.260129944081490338E-35 ) ) ;
#14172=CARTESIAN_POINT ( 'NONE',  ( -3.608439182435052128, -6.250000000000110134, -178.3080127018922383 ) ) ;
#14176=CARTESIAN_POINT ( 'NONE',  ( 5.999999999999974243, 1.607695154586759934, -123.5966878364870212 ) ) ;
#14177=CARTESIAN_POINT ( 'NONE',  ( 0.000000000000000000, 5.499999999999991118, -124.5000000000000568 ) ) ;
#14180=VERTEX_POINT ( 'NONE', #9101 ) ;
#14184=CARTESIAN_POINT ( 'NONE',  ( 5.999999999999949374, 1.607695154586804565, -156.0193375672974412 ) ) ;
#14185=ORIENTED_EDGE ( 'NONE', *, *, #22847, .T. ) ;
#14187=ADVANCED_FACE ( 'NONE', ( #5744 ), #4175, .T. ) ;
#14188=CARTESIAN_POINT ( 'NONE',  ( -3.464101615137757051, -5.999999999999979572, -176.6636751345947687 ) ) ;
#14189=CARTESIAN_POINT ( 'NONE',  ( 6.000000000000000888, -1.607695154586752384, -125.2306624327026157 ) ) ;
#14193=CARTESIAN_POINT ( 'NONE',  ( -3.464101615137725076, 5.999999999999979572, -141.1636751345948255 ) ) ;
#14195=EDGE_CURVE ( 'NONE', #15497, #18067, #23137, .T. ) ;
#14196=( BOUNDED_CURVE ( )  B_SPLINE_CURVE ( 2, ( #14397, #9290, #24269, #18990, #3217, #3369, #19685, #9600, #19128 ),
 .UNSPECIFIED., .F., .T. ) 
 B_SPLINE_CURVE_WITH_KNOTS ( ( 3, 2, 2, 2, 3 ),
 ( 0.9416666666666666519, 0.9425925925925926485, 0.9444444444444444198, 0.9462962962962963021, 0.9472222222222221877 ),
 .UNSPECIFIED. ) 
 CURVE ( )  GEOMETRIC_REPRESENTATION_ITEM ( )  RATIONAL_B_SPLINE_CURVE ( ( 0.9330127018922194093, 0.9330127018922154125, 1.000000000000000000, 0.8660254037844388186, 1.000000000000000000, 0.8660254037844388186, 1.000000000000000000, 0.9330127018922234061, 0.9330127018922194093 ) ) 
 REPRESENTATION_ITEM ( '' )  );
#14197=ORIENTED_EDGE ( 'NONE', *, *, #10950, .F. ) ;
#14198=CARTESIAN_POINT ( 'NONE',  ( -3.608439182435052128, -6.250000000000110134, -139.9419872981078470 ) ) ;
#14201=CARTESIAN_POINT ( 'NONE',  ( 5.999999999999949374, -1.607695154586841868, -171.1533121635130215 ) ) ;
#14206=CARTESIAN_POINT ( 'NONE',  ( -5.999999999999963585, -1.487416814333745711E-14, -97.41367513459481131 ) ) ;
#14210=CARTESIAN_POINT ( 'NONE',  ( 5.999999999999999112, 2.951592740943527306E-14, -149.1636751345948824 ) ) ;
#14211=ORIENTED_EDGE ( 'NONE', *, *, #7561, .F. ) ;
#14212=CARTESIAN_POINT ( 'NONE',  ( -3.175426480542816066, 5.499999999999865885, -53.87500000000003553 ) ) ;
#14213=CARTESIAN_POINT ( 'NONE',  ( -3.464101615137757051, -5.999999999999979572, -133.1636751345948539 ) ) ;
#14214=CARTESIAN_POINT ( 'NONE',  ( 3.464101615137852974, 5.999999999999884537, -79.33632486540523132 ) ) ;
#14216=EDGE_LOOP ( 'NONE', ( #2258, #2713, #9502, #6744 ) ) ;
#14221=CARTESIAN_POINT ( 'NONE',  ( 7.216878364870455975, -6.409875621278545621E-14, -100.4419872981078328 ) ) ;
#14227=CARTESIAN_POINT ( 'NONE',  ( 4.763139720814407951, 2.750000000000002665, -133.7500000000000284 ) ) ;
#14229=ORIENTED_EDGE ( 'NONE', *, *, #29117, .F. ) ;
#14230=ORIENTED_EDGE ( 'NONE', *, *, #3096, .T. ) ;
#14231=CARTESIAN_POINT ( 'NONE',  ( -5.196152422706601826, 2.999999999999975131, -162.9613248654052029 ) ) ;
#14232=CARTESIAN_POINT ( 'NONE',  ( 3.175426480543072749, -5.500000000000105693, -68.12500000000002842 ) ) ;
#14233=AXIS2_PLACEMENT_3D ( 'NONE', #9517, #12004, #9051 ) ;
#14235=CARTESIAN_POINT ( 'NONE',  ( 5.196152422706629359, 3.000000000000002665, -66.53867513459482552 ) ) ;
#14236=CARTESIAN_POINT ( 'NONE',  ( -3.608439182435115633, 6.249999999999965361, -79.80801270189226670 ) ) ;
#14237=DIRECTION ( 'NONE',  ( -7.147005652999508048E-36, 5.642372883946980038E-36, 1.000000000000000000 ) ) ;
#14238=CARTESIAN_POINT ( 'NONE',  ( 5.196152422706629359, -2.999999999999988898, -113.2886751345948397 ) ) ;
#14239=( BOUNDED_CURVE ( )  B_SPLINE_CURVE ( 2, ( #10345, #2953, #19706, #28744, #1102, #7863, #17275, #5704, #28592 ),
 .UNSPECIFIED., .F., .F. ) 
 B_SPLINE_CURVE_WITH_KNOTS ( ( 3, 2, 2, 2, 3 ),
 ( 0.9083333333333333259, 0.9092592592592592116, 0.9111111111111110938, 0.9129629629629629761, 0.9138888888888888618 ),
 .UNSPECIFIED. ) 
 CURVE ( )  GEOMETRIC_REPRESENTATION_ITEM ( )  RATIONAL_B_SPLINE_CURVE ( ( 0.9330127018922194093, 0.9330127018922194093, 1.000000000000000000, 0.8660254037844388186, 1.000000000000000000, 0.8660254037844388186, 1.000000000000000000, 0.9330127018922234061, 0.9330127018922194093 ) ) 
 REPRESENTATION_ITEM ( '' )  );
#14242=CARTESIAN_POINT ( 'NONE',  ( 4.763139720814407951, -2.749999999999988454, -147.5000000000000284 ) ) ;
#14243=DIRECTION ( 'NONE',  ( -7.147005652999508048E-36, 5.642372883946980038E-36, 1.000000000000000000 ) ) ;
#14244=CARTESIAN_POINT ( 'NONE',  ( 3.608439182435180470, -6.249999999999997335, -160.0580127018921814 ) ) ;
#14245=CARTESIAN_POINT ( 'NONE',  ( -1.285375204280330350E-15, -10.49588505988223375, 1.184433945098074864E-34 ) ) ;
#14246=CARTESIAN_POINT ( 'NONE',  ( 0.000000000000000000, 5.499999999999991118, -79.50000000000001421 ) ) ;
#14247=CARTESIAN_POINT ( 'NONE',  ( 6.350852961086080661, -9.614813431917819062E-14, -61.87500000000000711 ) ) ;
#14248=CARTESIAN_POINT ( 'NONE',  ( -5.999999999999962697, 3.323446944526963260E-14, -156.8363248654052313 ) ) ;
#14255=AXIS2_PLACEMENT_3D ( 'NONE', #15025, #420, #19339 ) ;
#14256=DIRECTION ( 'NONE',  ( -7.147005652999508048E-36, 5.642372883946980038E-36, 1.000000000000000000 ) ) ;
#14258=CARTESIAN_POINT ( 'NONE',  ( 3.464101615137852974, 5.999999999999884537, -82.33632486540524553 ) ) ;
#14260=AXIS2_PLACEMENT_3D ( 'NONE', #19966, #15864, #10613 ) ;
#14263=ORIENTED_EDGE ( 'NONE', *, *, #22715, .T. ) ;
#14266=CARTESIAN_POINT ( 'NONE',  ( -3.608439182435115633, 6.249999999999965361, -155.4419872981078186 ) ) ;
#14268=CARTESIAN_POINT ( 'NONE',  ( 4.763139720814407951, 2.750000000000002665, -85.75000000000000000 ) ) ;
#14269=CARTESIAN_POINT ( 'NONE',  ( -7.216878364870328078, 0.000000000000000000, -102.0580127018922383 ) ) ;
#14275=CARTESIAN_POINT ( 'NONE',  ( 4.763139720814407951, 2.750000000000002665, -175.7500000000000284 ) ) ;
#14276=CARTESIAN_POINT ( 'NONE',  ( -5.196152422706601826, 2.999999999999975131, -161.4613248654052029 ) ) ;
#14277=CARTESIAN_POINT ( 'NONE',  ( 4.763139720814407951, 2.750000000000002665, -156.2500000000000000 ) ) ;
#14279=CARTESIAN_POINT ( 'NONE',  ( -3.175426480542816066, -5.500000000000057732, -99.87500000000000000 ) ) ;
#14282=CARTESIAN_POINT ( 'NONE',  ( 3.175426480543072749, -5.500000000000105693, -155.1250000000000000 ) ) ;
#14283=CARTESIAN_POINT ( 'NONE',  ( 6.350852961086080661, -9.614813431917819062E-14, -90.37500000000000000 ) ) ;
#14286=FACE_OUTER_BOUND ( 'NONE', #5202, .T. ) ;
#14295=ORIENTED_EDGE ( 'NONE', *, *, #11513, .T. ) ;
#14300=CARTESIAN_POINT ( 'NONE',  ( -5.196152422706573404, -3.000000000000002665, -53.21132486540525264 ) ) ;
#14303=VERTEX_POINT ( 'NONE', #2348 ) ;
#14304=CARTESIAN_POINT ( 'NONE',  ( -4.763139720814407951, -2.750000000000016431, -114.9999999999999858 ) ) ;
#14306=CARTESIAN_POINT ( 'NONE',  ( 2.775557561562891351E-14, -6.250000000000061284, -124.1830127018922525 ) ) ;
#14308=CARTESIAN_POINT ( 'NONE',  ( -7.216878364870328078, 0.000000000000000000, -170.1919872981078186 ) ) ;
#14312=CARTESIAN_POINT ( 'NONE',  ( 2.027308962376910273, 5.280605156494750929, -179.9999999999999716 ) ) ;
#14313=CARTESIAN_POINT ( 'NONE',  ( 0.000000000000000000, 0.000000000000000000, 0.000000000000000000 ) ) ;
#14314=CARTESIAN_POINT ( 'NONE',  ( 4.763139720814407951, -2.749999999999988454, -180.5000000000000000 ) ) ;
#14316=CARTESIAN_POINT ( 'NONE',  ( 3.608439182435180470, -6.249999999999997335, -175.0580127018922383 ) ) ;
#14317=CARTESIAN_POINT ( 'NONE',  ( 6.000000000000000888, 7.762456499804235646E-14, -139.5863248654051745 ) ) ;
#14318=LINE ( 'NONE', #21206, #9882 ) ;
#14322=CARTESIAN_POINT ( 'NONE',  ( 0.000000000000000000, 5.499999999999991118, -115.5000000000000426 ) ) ;
#14324=CARTESIAN_POINT ( 'NONE',  ( 6.000000000000000888, 1.607695154586715303, -146.0966878364870354 ) ) ;
#14325=AXIS2_PLACEMENT_3D ( 'NONE', #855, #10554, #15341 ) ;
#14326=VERTEX_POINT ( 'NONE', #21095 ) ;
#14329=CARTESIAN_POINT ( 'NONE',  ( -5.999999999999919176, 1.607695154586804565, -108.9033121635129930 ) ) ;
#14330=CARTESIAN_POINT ( 'NONE',  ( 5.196152422706629359, 3.000000000000002665, -155.9613248654052597 ) ) ;
#14332=ORIENTED_EDGE ( 'NONE', *, *, #1895, .T. ) ;
#14333=CARTESIAN_POINT ( 'NONE',  ( -3.175426480542816066, 5.499999999999865885, -178.3750000000000568 ) ) ;
#14334=( BOUNDED_CURVE ( )  B_SPLINE_CURVE ( 2, ( #728, #24368, #24512, #1015, #21785, #863, #2875, #29113, #23937 ),
 .UNSPECIFIED., .F., .F. ) 
 B_SPLINE_CURVE_WITH_KNOTS ( ( 3, 2, 2, 2, 3 ),
 ( 0.5194444444444444864, 0.5203703703703703720, 0.5222222222222222543, 0.5240740740740740256, 0.5249999999999999112 ),
 .UNSPECIFIED. ) 
 CURVE ( )  GEOMETRIC_REPRESENTATION_ITEM ( )  RATIONAL_B_SPLINE_CURVE ( ( 0.9330127018922194093, 0.9330127018922234061, 1.000000000000000000, 0.8660254037844388186, 1.000000000000000000, 0.8660254037844388186, 1.000000000000000000, 0.9330127018922234061, 0.9330127018922194093 ) ) 
 REPRESENTATION_ITEM ( '' )  );
#14335=CYLINDRICAL_SURFACE ( 'NONE', #30305, 6.000000000000000888 ) ;
#14338=ORIENTED_EDGE ( 'NONE', *, *, #27746, .F. ) ;
#14341=VERTEX_POINT ( 'NONE', #22290 ) ;
#14342=CARTESIAN_POINT ( 'NONE',  ( 2.775557561562891351E-14, -6.250000000000061284, -141.3169872981078186 ) ) ;
#14344=VECTOR ( 'NONE', #22167, 1000.000000000000000 ) ;
#14346=CARTESIAN_POINT ( 'NONE',  ( 6.000000000000000888, 7.762456499804234384E-14, -129.6636751345948255 ) ) ;
#14350=CARTESIAN_POINT ( 'NONE',  ( 5.999999999999949374, 1.607695154586804565, -99.59668783648702117 ) ) ;
#14351=CARTESIAN_POINT ( 'NONE',  ( 0.000000000000000000, -5.999999999999991118, -70.03867513459482552 ) ) ;
#14353=ADVANCED_FACE ( 'NONE', ( #21838 ), #5824, .T. ) ;
#14355=FILL_AREA_STYLE_COLOUR ( '', #4318 ) ;
#14357=CARTESIAN_POINT ( 'NONE',  ( -6.000000000000000888, 1.067854986875958443E-15, 7.560779664488942560E-35 ) ) ;
#14362=CARTESIAN_POINT ( 'NONE',  ( -3.464101615137757051, -5.999999999999979572, -107.0863248654051461 ) ) ;
#14363=CARTESIAN_POINT ( 'NONE',  ( -3.464101615137725076, 5.999999999999979572, -52.66367513459479710 ) ) ;
#14364=CARTESIAN_POINT ( 'NONE',  ( -5.999999999999964473, 9.063946212346262433E-15, -173.3363248654052597 ) ) ;
#14365=CARTESIAN_POINT ( 'NONE',  ( -5.196152422706573404, -3.000000000000002665, -179.2113248654052597 ) ) ;
#14369=CARTESIAN_POINT ( 'NONE',  ( 7.216878364870455975, -6.409875621278545621E-14, -103.4419872981078328 ) ) ;
#14374=VECTOR ( 'NONE', #2589, 1000.000000000000000 ) ;
#14375=CARTESIAN_POINT ( 'NONE',  ( 4.763139720814407951, 2.750000000000002665, -127.7500000000000284 ) ) ;
#14378=CARTESIAN_POINT ( 'NONE',  ( 5.999999999999949374, 1.607695154586804565, -81.59668783648703538 ) ) ;
#14379=CARTESIAN_POINT ( 'NONE',  ( 3.175426480543072749, -5.500000000000105693, -60.62500000000000000 ) ) ;
#14382=CARTESIAN_POINT ( 'NONE',  ( 2.775557561562891351E-14, 6.250000000000033751, -79.93301270189223828 ) ) ;
#14386=EDGE_CURVE ( 'NONE', #21660, #5195, #8391, .T. ) ;
#14390=CARTESIAN_POINT ( 'NONE',  ( -2.775557561562891351E-14, -5.500000000000115463, -137.2499999999999716 ) ) ;
#14391=CARTESIAN_POINT ( 'NONE',  ( 6.000000000000000888, 1.743066579297358182E-13, -57.08632486540521001 ) ) ;
#14392=CARTESIAN_POINT ( 'NONE',  ( -3.608439182435052128, -6.250000000000110134, -151.3080127018922099 ) ) ;
#14393=CARTESIAN_POINT ( 'NONE',  ( -3.464101615137725076, 5.999999999999979572, -116.5863248654052171 ) ) ;
#14394=CARTESIAN_POINT ( 'NONE',  ( -5.999999999999963585, 1.780251999655701777E-13, -89.33632486540523132 ) ) ;
#14395=CARTESIAN_POINT ( 'NONE',  ( 3.175426480543072749, -5.500000000000105693, -77.12500000000001421 ) ) ;
#14396=CARTESIAN_POINT ( 'NONE',  ( -5.999999999999971578, 1.607695154586715303, -113.9806624327025872 ) ) ;
#14397=CARTESIAN_POINT ( 'NONE',  ( -5.999999999999964473, 9.063946212346262433E-15, -173.3363248654052597 ) ) ;
#14399=CARTESIAN_POINT ( 'NONE',  ( -3.175426480542816510, 5.499999999999865885, -64.37500000000001421 ) ) ;
#14401=LINE ( 'NONE', #21131, #4507 ) ;
#14406=CARTESIAN_POINT ( 'NONE',  ( -5.196152422706573404, -3.000000000000002665, -50.21132486540524553 ) ) ;
#14407=CARTESIAN_POINT ( 'NONE',  ( 0.000000000000000000, 0.000000000000000000, 0.000000000000000000 ) ) ;
#14409=CARTESIAN_POINT ( 'NONE',  ( -5.999999999999919176, 1.607695154586804565, -81.90331216351300725 ) ) ;
#14413=FACE_OUTER_BOUND ( 'NONE', #19832, .T. ) ;
#14415=ORIENTED_EDGE ( 'NONE', *, *, #22680, .F. ) ;
#14416=CARTESIAN_POINT ( 'NONE',  ( 6.350852961086080661, -9.614813431917819062E-14, -87.37500000000007105 ) ) ;
#14417=CARTESIAN_POINT ( 'NONE',  ( 5.412658773652712085, -3.125000000000086153, -101.4330127018922525 ) ) ;
#14418=CARTESIAN_POINT ( 'NONE',  ( -6.000000000000000888, 1.067854986875958443E-15, 7.560779664488942560E-35 ) ) ;
#14422=CARTESIAN_POINT ( 'NONE',  ( -5.196152422706601826, 2.999999999999975131, -58.53867513459481842 ) ) ;
#14424=SURFACE_STYLE_FILL_AREA ( #25751 ) ;
#14426=CARTESIAN_POINT ( 'NONE',  ( -3.175426480542816066, -5.500000000000057732, -162.8750000000000568 ) ) ;
#14427=CARTESIAN_POINT ( 'NONE',  ( -5.196152422706601826, 2.999999999999975131, -57.96132486540523132 ) ) ;
#14428=CARTESIAN_POINT ( 'NONE',  ( 3.175426480543072749, -5.500000000000105693, -155.1250000000000000 ) ) ;
#14430=CARTESIAN_POINT ( 'NONE',  ( -3.175426480542816066, -5.500000000000057732, -102.8750000000000142 ) ) ;
#14432=CARTESIAN_POINT ( 'NONE',  ( 6.000000000000000888, 7.762456499804235646E-14, -121.5863248654052455 ) ) ;
#14433=ADVANCED_FACE ( 'NONE', ( #3523 ), #28717, .T. ) ;
#14434=CARTESIAN_POINT ( 'NONE',  ( 3.175426480543072749, 5.499999999999865885, -90.12500000000001421 ) ) ;
#14439=CARTESIAN_POINT ( 'NONE',  ( -3.464101615137757051, -5.999999999999979572, -66.58632486540523132 ) ) ;
#14441=CARTESIAN_POINT ( 'NONE',  ( -5.999999999999919176, 1.607695154586804565, -77.98066243270260145 ) ) ;
#14443=DIRECTION ( 'NONE',  ( 1.000000000000000000, -5.551115123125773458E-17, -1.260129944081490338E-35 ) ) ;
#14447=CARTESIAN_POINT ( 'NONE',  ( 4.763139720814407951, -2.749999999999988454, -114.5000000000000426 ) ) ;
#14449=CARTESIAN_POINT ( 'NONE',  ( -7.216878364870328078, 0.000000000000000000, -120.0580127018922525 ) ) ;
#14450=ORIENTED_EDGE ( 'NONE', *, *, #19695, .T. ) ;
#14452=CARTESIAN_POINT ( 'NONE',  ( 2.775557561562891351E-14, -6.250000000000061284, -163.8169872981078470 ) ) ;
#14457=EDGE_CURVE ( 'NONE', #26998, #27478, #18661, .T. ) ;
#14458=( BOUNDED_CURVE ( )  B_SPLINE_CURVE ( 2, ( #19842, #24289, #7709, #24756, #12663, #13126, #29043, #17116, #22464 ),
 .UNSPECIFIED., .F., .T. ) 
 B_SPLINE_CURVE_WITH_KNOTS ( ( 3, 2, 2, 2, 3 ),
 ( 0.6805555555555555802, 0.6814814814814814659, 0.6833333333333333481, 0.6851851851851851194, 0.6861111111111111160 ),
 .UNSPECIFIED. ) 
 CURVE ( )  GEOMETRIC_REPRESENTATION_ITEM ( )  RATIONAL_B_SPLINE_CURVE ( ( 0.9330127018922194093, 0.9330127018922234061, 1.000000000000000000, 0.8660254037844388186, 1.000000000000000000, 0.8660254037844388186, 1.000000000000000000, 0.9330127018922194093, 0.9330127018922194093 ) ) 
 REPRESENTATION_ITEM ( '' )  );
#14459=DIRECTION ( 'NONE',  ( 1.000000000000000000, -5.551115123125773458E-17, -1.260129944081490338E-35 ) ) ;
#14460=CYLINDRICAL_SURFACE ( 'NONE', #12878, 6.000000000000000888 ) ;
#14461=CARTESIAN_POINT ( 'NONE',  ( 0.000000000000000000, 5.499999999999991118, -180.0000000000000568 ) ) ;
#14464=CARTESIAN_POINT ( 'NONE',  ( 7.216878364870455975, -6.409875621278545621E-14, -177.8080127018922667 ) ) ;
#14467=CARTESIAN_POINT ( 'NONE',  ( 6.350852961086080661, -9.614813431917819062E-14, -124.8749999999999858 ) ) ;
#14469=CARTESIAN_POINT ( 'NONE',  ( 0.000000000000000000, 5.499999999999991118, -117.0000000000000000 ) ) ;
#14470=DIRECTION ( 'NONE',  ( -7.147005652999508048E-36, 5.642372883946980038E-36, 1.000000000000000000 ) ) ;
#14473=CARTESIAN_POINT ( 'NONE',  ( 6.000000000000000000, 2.951592740943527306E-14, -150.6636751345948539 ) ) ;
#14474=CARTESIAN_POINT ( 'NONE',  ( 5.196152422706629359, -2.999999999999988898, -136.7113248654052029 ) ) ;
#14475=CARTESIAN_POINT ( 'NONE',  ( -5.196152422706601826, 2.999999999999975131, -155.4613248654052029 ) ) ;
#14476=CARTESIAN_POINT ( 'NONE',  ( 5.999999999999949374, 1.607695154586804565, -87.01933756729741276 ) ) ;
#14478=CARTESIAN_POINT ( 'NONE',  ( 3.464101615137757051, -5.999999999999979572, -126.3363248654051887 ) ) ;
#14479=CARTESIAN_POINT ( 'NONE',  ( -3.175426480542417718, 5.500000000000556000, -179.8750000000000853 ) ) ;
#14480=CARTESIAN_POINT ( 'NONE',  ( 0.000000000000000000, 0.000000000000000000, 0.000000000000000000 ) ) ;
#14482=CARTESIAN_POINT ( 'NONE',  ( 5.196152422706629359, -2.999999999999988898, -125.2886751345948539 ) ) ;
#14484=VERTEX_POINT ( 'NONE', #18157 ) ;
#14488=CARTESIAN_POINT ( 'NONE',  ( 3.608439182435180470, 6.249999999999982236, -139.1919872981078470 ) ) ;
#14490=CARTESIAN_POINT ( 'NONE',  ( -5.196152422706601826, 2.999999999999975131, -174.9613248654052313 ) ) ;
#14491=CARTESIAN_POINT ( 'NONE',  ( -5.999999999999971578, 1.607695154586715303, -128.9806624327026441 ) ) ;
#14492=EDGE_LOOP ( 'NONE', ( #12361, #24782, #8854, #9871 ) ) ;
#14494=LINE ( 'NONE', #28410, #12769 ) ;
#14495=CARTESIAN_POINT ( 'NONE',  ( -5.999999999999963585, -1.487416814333745711E-14, -66.83632486540523132 ) ) ;
#14496=EDGE_CURVE ( 'NONE', #8469, #16412, #1755, .T. ) ;
#14500=CARTESIAN_POINT ( 'NONE',  ( -5.999999999999971578, 1.607695154586715303, -59.98066243270260856 ) ) ;
#14503=VERTEX_POINT ( 'NONE', #13260 ) ;
#14504=CARTESIAN_POINT ( 'NONE',  ( -4.763139720814407951, -2.750000000000016431, -49.00000000000004263 ) ) ;
#14505=CARTESIAN_POINT ( 'NONE',  ( 6.000000000000000888, 1.607695154586715303, -79.51933756729744118 ) ) ;
#14506=ORIENTED_EDGE ( 'NONE', *, *, #16711, .T. ) ;
#14509=CARTESIAN_POINT ( 'NONE',  ( -7.216878364870328078, 0.000000000000000000, -107.1919872981078612 ) ) ;
#14510=CARTESIAN_POINT ( 'NONE',  ( -5.999999999999956479, -1.607695154586745057, -50.84668783648707091 ) ) ;
#14514=CARTESIAN_POINT ( 'NONE',  ( 4.763139720814407951, 2.750000000000002665, -132.2500000000000284 ) ) ;
#14517=VERTEX_POINT ( 'NONE', #29641 ) ;
#14518=CARTESIAN_POINT ( 'NONE',  ( -3.464101615137725076, 5.999999999999979572, -96.16367513459479710 ) ) ;
#14520=CARTESIAN_POINT ( 'NONE',  ( 6.350852961086080661, -9.614813431917819062E-14, -60.37500000000000000 ) ) ;
#14521=CARTESIAN_POINT ( 'NONE',  ( -5.196152422706601826, 2.999999999999975131, -115.5386751345948113 ) ) ;
#14523=CARTESIAN_POINT ( 'NONE',  ( -7.216878364870328078, 0.000000000000000000, -81.05801270189220986 ) ) ;
#14525=CARTESIAN_POINT ( 'NONE',  ( 3.464101615137852974, 5.999999999999884537, -149.8363248654051176 ) ) ;
#14528=CARTESIAN_POINT ( 'NONE',  ( 4.763139720814407951, 2.750000000000002665, -138.2499999999999716 ) ) ;
#14530=CARTESIAN_POINT ( 'NONE',  ( 2.775557561562891351E-14, 6.250000000000033751, -150.4330127018922383 ) ) ;
#14531=CARTESIAN_POINT ( 'NONE',  ( -3.175426480542816066, -5.500000000000057732, -69.87500000000004263 ) ) ;
#14533=CARTESIAN_POINT ( 'NONE',  ( 3.175426480543072749, -5.500000000000105693, -68.12500000000002842 ) ) ;
#14534=( BOUNDED_CURVE ( )  B_SPLINE_CURVE ( 2, ( #5286, #12262, #16012, #385, #16164, #6746, #27769, #14557, #19154 ),
 .UNSPECIFIED., .F., .T. ) 
 B_SPLINE_CURVE_WITH_KNOTS ( ( 3, 2, 2, 2, 3 ),
 ( 0.9416666666666666519, 0.9425925925925925375, 0.9444444444444444198, 0.9462962962962963021, 0.9472222222222221877 ),
 .UNSPECIFIED. ) 
 CURVE ( )  GEOMETRIC_REPRESENTATION_ITEM ( )  RATIONAL_B_SPLINE_CURVE ( ( 0.9330127018922194093, 0.9330127018922194093, 1.000000000000000000, 0.8660254037844388186, 1.000000000000000000, 0.8660254037844388186, 1.000000000000000000, 0.9330127018922234061, 0.9330127018922194093 ) ) 
 REPRESENTATION_ITEM ( '' )  );
#14538=CARTESIAN_POINT ( 'NONE',  ( -5.999999999999963585, -1.487416814333745711E-14, -133.4136751345948255 ) ) ;
#14541=CARTESIAN_POINT ( 'NONE',  ( 5.196152422706629359, -2.999999999999988898, -147.2113248654052313 ) ) ;
#14546=EDGE_CURVE ( 'NONE', #23883, #19083, #15876, .T. ) ;
#14547=CARTESIAN_POINT ( 'NONE',  ( 5.196152422706629359, -2.999999999999988898, -102.2113248654051887 ) ) ;
#14548=CARTESIAN_POINT ( 'NONE',  ( -4.763139720814407951, 2.749999999999946709, -179.7500000000000284 ) ) ;
#14550=CARTESIAN_POINT ( 'NONE',  ( -5.412658773652684552, -3.125000000000099920, -152.0669872981078470 ) ) ;
#14552=CARTESIAN_POINT ( 'NONE',  ( 0.000000000000000000, 5.499999999999991118, -81.00000000000001421 ) ) ;
#14553=EDGE_CURVE ( 'NONE', #1699, #12019, #28085, .T. ) ;
#14554=CARTESIAN_POINT ( 'NONE',  ( -5.412658773652739619, 3.124999999999975131, -99.18301270189222407 ) ) ;
#14557=CARTESIAN_POINT ( 'NONE',  ( -5.999999999999919176, 1.607695154586804565, -53.98066243270259434 ) ) ;
#14558=CARTESIAN_POINT ( 'NONE',  ( 3.464101615137852974, 5.999999999999884537, -58.91367513459482552 ) ) ;
#14561=CARTESIAN_POINT ( 'NONE',  ( -3.175426480542816066, -5.500000000000057732, -167.3750000000000568 ) ) ;
#14562=CARTESIAN_POINT ( 'NONE',  ( -6.350852961085760029, -1.281975124255709124E-13, -155.6249999999999716 ) ) ;
#14564=CARTESIAN_POINT ( 'NONE',  ( -6.350852961085760029, -1.281975124255709124E-13, -97.12500000000004263 ) ) ;
#14565=CARTESIAN_POINT ( 'NONE',  ( 3.175426480543072749, 5.499999999999865885, -91.62500000000001421 ) ) ;
#14567=CARTESIAN_POINT ( 'NONE',  ( 6.000000000000000888, -1.859271017917181981E-14, -135.6636751345948255 ) ) ;
#14570=CARTESIAN_POINT ( 'NONE',  ( 0.000000000000000000, 0.000000000000000000, 0.000000000000000000 ) ) ;
#14573=SURFACE_SIDE_STYLE ('',( #12284 ) ) ;
#14577=ORIENTED_EDGE ( 'NONE', *, *, #9039, .F. ) ;
#14579=CARTESIAN_POINT ( 'NONE',  ( 4.763139720814407951, 2.750000000000002665, -108.2500000000000142 ) ) ;
#14582=EDGE_CURVE ( 'NONE', #26402, #15213, #9037, .T. ) ;
#14583=CARTESIAN_POINT ( 'NONE',  ( 3.608439182435180470, -6.249999999999997335, -122.5580127018922667 ) ) ;
#14585=VERTEX_POINT ( 'NONE', #19069 ) ;
#14586=CARTESIAN_POINT ( 'NONE',  ( 6.000000000000000888, -1.859271017917181981E-14, -68.16367513459481131 ) ) ;
#14587=CARTESIAN_POINT ( 'NONE',  ( 3.608439182435180470, -6.249999999999997335, -162.1919872981078754 ) ) ;
#14591=CARTESIAN_POINT ( 'NONE',  ( 2.775557561562891351E-14, 6.250000000000033751, -63.43301270189222407 ) ) ;
#14595=CARTESIAN_POINT ( 'NONE',  ( 4.763139720814407951, -2.749999999999988454, -179.0000000000000568 ) ) ;
#14597=CARTESIAN_POINT ( 'NONE',  ( 0.000000000000000000, -5.999999999999991118, -169.0386751345947971 ) ) ;
#14598=CARTESIAN_POINT ( 'NONE',  ( 7.216878364870455975, -6.409875621278545621E-14, -179.3080127018922667 ) ) ;
#14600=CARTESIAN_POINT ( 'NONE',  ( 6.000000000000000888, 1.743066579297358182E-13, -48.08632486540521711 ) ) ;
#14601=CARTESIAN_POINT ( 'NONE',  ( 0.000000000000000000, 5.499999999999991118, -115.5000000000000426 ) ) ;
#14602=CARTESIAN_POINT ( 'NONE',  ( 5.196152422706629359, 3.000000000000002665, -84.53867513459483973 ) ) ;
#14603=CARTESIAN_POINT ( 'NONE',  ( 3.175426480543072749, 5.499999999999865885, -109.6249999999999716 ) ) ;
#14605=ORIENTED_EDGE ( 'NONE', *, *, #5819, .F. ) ;
#14607=DIRECTION ( 'NONE',  ( -5.551115123125774074E-17, -1.000000000000000000, -6.394689268473234689E-36 ) ) ;
#14608=FACE_OUTER_BOUND ( 'NONE', #25934, .T. ) ;
#14610=ORIENTED_EDGE ( 'NONE', *, *, #17486, .F. ) ;
#14614=ORIENTED_EDGE ( 'NONE', *, *, #28734, .T. ) ;
#14616=( BOUNDED_CURVE ( )  B_SPLINE_CURVE ( 2, ( #29406, #8377, #22064, #29575, #29097, #10250, #6073, #17787, #26787 ),
 .UNSPECIFIED., .F., .F. ) 
 B_SPLINE_CURVE_WITH_KNOTS ( ( 3, 2, 2, 2, 3 ),
 ( 0.4194444444444444531, 0.4203703703703703942, 0.4222222222222222210, 0.4240740740740740478, 0.4249999999999999889 ),
 .UNSPECIFIED. ) 
 CURVE ( )  GEOMETRIC_REPRESENTATION_ITEM ( )  RATIONAL_B_SPLINE_CURVE ( ( 0.9330127018922194093, 0.9330127018922194093, 1.000000000000000000, 0.8660254037844388186, 1.000000000000000000, 0.8660254037844388186, 1.000000000000000000, 0.9330127018922194093, 0.9330127018922194093 ) ) 
 REPRESENTATION_ITEM ( '' )  );
#14619=ORIENTED_EDGE ( 'NONE', *, *, #26811, .F. ) ;
#14624=CARTESIAN_POINT ( 'NONE',  ( -5.412658773652684552, -3.125000000000099920, -129.5669872981078470 ) ) ;
#14628=EDGE_LOOP ( 'NONE', ( #8756, #28178, #14229, #19180 ) ) ;
#14634=CARTESIAN_POINT ( 'NONE',  ( -6.000000000000007105, -1.607695154586655129, -99.76933756729744118 ) ) ;
#14635=CARTESIAN_POINT ( 'NONE',  ( -6.000000000000000888, 1.067854986875958443E-15, 7.560779664488942560E-35 ) ) ;
#14638=CARTESIAN_POINT ( 'NONE',  ( 6.000000000000000888, 1.743066579297358182E-13, -111.6636751345948255 ) ) ;
#14639=CARTESIAN_POINT ( 'NONE',  ( 4.763139720814407951, 2.750000000000002665, -136.7500000000000284 ) ) ;
#14641=VERTEX_POINT ( 'NONE', #2598 ) ;
#14642=CARTESIAN_POINT ( 'NONE',  ( -2.775557561562891351E-14, -5.500000000000115463, -47.25000000000001421 ) ) ;
#14648=CARTESIAN_POINT ( 'NONE',  ( 5.412658773652712085, -3.125000000000086153, -96.06698729810780435 ) ) ;
#14654=CARTESIAN_POINT ( 'NONE',  ( 3.464101615137852974, 5.999999999999884537, -77.83632486540520290 ) ) ;
#14655=CARTESIAN_POINT ( 'NONE',  ( 6.350852961086080661, -9.614813431917819062E-14, -126.3749999999999858 ) ) ;
#14658=CARTESIAN_POINT ( 'NONE',  ( 3.175426480543072749, -5.500000000000105693, -57.62500000000004974 ) ) ;
#14659=CARTESIAN_POINT ( 'NONE',  ( 0.000000000000000000, -5.999999999999991118, -179.5386751345948255 ) ) ;
#14661=CARTESIAN_POINT ( 'NONE',  ( 6.000000000000000888, 1.607695154586715303, -68.09668783648703538 ) ) ;
#14662=CARTESIAN_POINT ( 'NONE',  ( 5.412658773652712085, -3.125000000000086153, -84.93301270189223828 ) ) ;
#14663=CARTESIAN_POINT ( 'NONE',  ( 2.775557561562891351E-14, 20.00000000000001776, -31.00000000000002487 ) ) ;
#14664=CARTESIAN_POINT ( 'NONE',  ( 6.000000000000000888, 1.743066579297358182E-13, -48.08632486540521711 ) ) ;
#14667=CARTESIAN_POINT ( 'NONE',  ( -4.763139720814407951, 2.749999999999946709, -137.7500000000000284 ) ) ;
#14669=CARTESIAN_POINT ( 'NONE',  ( 2.775557561562891351E-14, 6.250000000000033751, -154.9330127018922383 ) ) ;
#14672=ADVANCED_FACE ( 'NONE', ( #17060 ), #5639, .T. ) ;
#14673=CARTESIAN_POINT ( 'NONE',  ( -2.775557561562891351E-14, -5.500000000000115463, -69.75000000000002842 ) ) ;
#14674=CARTESIAN_POINT ( 'NONE',  ( 0.000000000000000000, 5.499999999999991118, -66.00000000000000000 ) ) ;
#14675=CARTESIAN_POINT ( 'NONE',  ( -4.000000000000000000, 7.119033245839722951E-16, -200.0000000000000000 ) ) ;
#14678=FACE_BOUND ( 'NONE', #16746, .T. ) ;
#14680=CARTESIAN_POINT ( 'NONE',  ( 3.464101615137757051, -5.999999999999979572, -98.41367513459481131 ) ) ;
#14681=CARTESIAN_POINT ( 'NONE',  ( 0.000000000000000000, 5.999999999999977796, -82.21132486540521711 ) ) ;
#14683=VERTEX_POINT ( 'NONE', #18270 ) ;
#14686=CARTESIAN_POINT ( 'NONE',  ( 6.000000000000000888, 1.743066579297358182E-13, -64.58632486540520290 ) ) ;
#14687=CARTESIAN_POINT ( 'NONE',  ( -4.763139720814407951, 2.749999999999946709, -178.2500000000000284 ) ) ;
#14690=CARTESIAN_POINT ( 'NONE',  ( 2.775557561562891351E-14, -6.250000000000061284, -154.8169872981078470 ) ) ;
#14692=CARTESIAN_POINT ( 'NONE',  ( -3.175426480542816510, -5.500000000000057732, -84.87500000000004263 ) ) ;
#14697=( BOUNDED_CURVE ( )  B_SPLINE_CURVE ( 2, ( #3945, #14000, #25290, #23340, #13374, #4414, #22717, #18278, #17029 ),
 .UNSPECIFIED., .F., .T. ) 
 B_SPLINE_CURVE_WITH_KNOTS ( ( 3, 2, 2, 2, 3 ),
 ( 0.9138888888888888618, 0.9148148148148148584, 0.9166666666666666297, 0.9185185185185185119, 0.9194444444444443976 ),
 .UNSPECIFIED. ) 
 CURVE ( )  GEOMETRIC_REPRESENTATION_ITEM ( )  RATIONAL_B_SPLINE_CURVE ( ( 0.9330127018922194093, 0.9330127018922154125, 1.000000000000000000, 0.8660254037844388186, 1.000000000000000000, 0.8660254037844388186, 1.000000000000000000, 0.9330127018922234061, 0.9330127018922194093 ) ) 
 REPRESENTATION_ITEM ( '' )  );
#14698=CARTESIAN_POINT ( 'NONE',  ( 3.175426480543072749, -5.500000000000105693, -161.1250000000000284 ) ) ;
#14700=CARTESIAN_POINT ( 'NONE',  ( -3.175426480542816510, -5.500000000000057732, -147.8750000000000284 ) ) ;
#14701=EDGE_CURVE ( 'NONE', #2318, #15772, #29288, .T. ) ;
#14702=CYLINDRICAL_SURFACE ( 'NONE', #4645, 6.000000000000000888 ) ;
#14704=EDGE_CURVE ( 'NONE', #15998, #341, #2918, .T. ) ;
#14705=VECTOR ( 'NONE', #8228, 1000.000000000000000 ) ;
#14706=CARTESIAN_POINT ( 'NONE',  ( 6.350852961086080661, -9.614813431917819062E-14, -97.87499999999998579 ) ) ;
#14708=CARTESIAN_POINT ( 'NONE',  ( -4.763139720814407951, -2.750000000000016431, -92.50000000000002842 ) ) ;
#14712=CARTESIAN_POINT ( 'NONE',  ( -3.464101615137725076, 5.999999999999979572, -64.66367513459478289 ) ) ;
#14713=DIRECTION ( 'NONE',  ( 1.000000000000000000, -5.551115123125773458E-17, -1.260129944081490338E-35 ) ) ;
#14721=CARTESIAN_POINT ( 'NONE',  ( 5.999999999999993783, 1.607695154586726627, -179.0966878364870638 ) ) ;
#14722=CARTESIAN_POINT ( 'NONE',  ( -6.000000000000000888, 1.067854986875958443E-15, 7.560779664488942560E-35 ) ) ;
#14725=CARTESIAN_POINT ( 'NONE',  ( -3.175426480542816510, 5.499999999999865885, -103.3750000000000142 ) ) ;
#14727=CARTESIAN_POINT ( 'NONE',  ( 7.216878364870455975, -6.409875621278545621E-14, -122.3080127018922099 ) ) ;
#14729=CARTESIAN_POINT ( 'NONE',  ( 6.000000000000000888, -1.859271017917181981E-14, -110.1636751345948397 ) ) ;
#14731=CARTESIAN_POINT ( 'NONE',  ( -7.216878364870328078, 0.000000000000000000, -162.6919872981078754 ) ) ;
#14734=CARTESIAN_POINT ( 'NONE',  ( -3.608439182435052128, -6.250000000000110134, -59.80801270189223118 ) ) ;
#14738=CARTESIAN_POINT ( 'NONE',  ( -5.999999999999962697, 3.323446944526963260E-14, -150.8363248654052029 ) ) ;
#14741=CARTESIAN_POINT ( 'NONE',  ( -3.608439182435115633, 6.249999999999965361, -168.3080127018922383 ) ) ;
#14742=MANIFOLD_SOLID_BREP ( 'Cut-Sweep2', #17882 ) ;
#14745=FACE_OUTER_BOUND ( 'NONE', #6878, .T. ) ;
#14747=CARTESIAN_POINT ( 'NONE',  ( -4.763139720814407951, 2.749999999999946709, -115.2500000000000142 ) ) ;
#14749=CARTESIAN_POINT ( 'NONE',  ( -6.000000000000000888, 1.067854986875958443E-15, 7.560779664488942560E-35 ) ) ;
#14750=VERTEX_POINT ( 'NONE', #24341 ) ;
#14752=CYLINDRICAL_SURFACE ( 'NONE', #27039, 6.000000000000001776 ) ;
#14754=CARTESIAN_POINT ( 'NONE',  ( -6.000000000000007105, -1.607695154586655129, -56.26933756729747671 ) ) ;
#14755=EDGE_CURVE ( 'NONE', #12840, #10564, #13201, .T. ) ;
#14757=ORIENTED_EDGE ( 'NONE', *, *, #9919, .F. ) ;
#14766=CARTESIAN_POINT ( 'NONE',  ( -5.412658773652739619, 3.124999999999975131, -134.3169872981078186 ) ) ;
#14768=CARTESIAN_POINT ( 'NONE',  ( -5.999999999999944933, 1.607695154586759934, -130.4806624327025872 ) ) ;
#14769=CARTESIAN_POINT ( 'NONE',  ( 5.196152422706629359, -2.999999999999988898, -116.2886751345948397 ) ) ;
#14771=ORIENTED_EDGE ( 'NONE', *, *, #2050, .F. ) ;
#14775=VECTOR ( 'NONE', #23075, 1000.000000000000000 ) ;
#14779=CARTESIAN_POINT ( 'NONE',  ( 3.464101615137757051, -5.999999999999979572, -69.33632486540518869 ) ) ;
#14781=EDGE_CURVE ( 'NONE', #28335, #14937, #6060, .T. ) ;
#14782=CARTESIAN_POINT ( 'NONE',  ( -5.999999999999982236, -1.607695154586700426, -115.3466878364870638 ) ) ;
#14783=CARTESIAN_POINT ( 'NONE',  ( 3.175426480543072749, 5.499999999999865885, -135.1250000000000000 ) ) ;
#14784=VECTOR ( 'NONE', #23696, 1000.000000000000000 ) ;
#14786=ORIENTED_EDGE ( 'NONE', *, *, #565, .F. ) ;
#14788=EDGE_CURVE ( 'NONE', #28360, #23232, #5866, .T. ) ;
#14790=( BOUNDED_CURVE ( )  B_SPLINE_CURVE ( 2, ( #22827, #11019, #25249, #6687, #3907, #2088, #1926, #18234, #4222 ),
 .UNSPECIFIED., .F., .F. ) 
 B_SPLINE_CURVE_WITH_KNOTS ( ( 3, 2, 2, 2, 3 ),
 ( 0.06388888888888888395, 0.06481481481481476958, 0.06666666666666665186, 0.06851851851851853414, 0.06944444444444441977 ),
 .UNSPECIFIED. ) 
 CURVE ( )  GEOMETRIC_REPRESENTATION_ITEM ( )  RATIONAL_B_SPLINE_CURVE ( ( 0.9330127018922194093, 0.9330127018922194093, 1.000000000000000000, 0.8660254037844388186, 1.000000000000000000, 0.8660254037844388186, 1.000000000000000000, 0.9330127018922234061, 0.9330127018922194093 ) ) 
 REPRESENTATION_ITEM ( '' )  );
#14795=CARTESIAN_POINT ( 'NONE',  ( -5.412658773652684552, -3.125000000000099920, -92.06698729810780435 ) ) ;
#14798=( BOUNDED_CURVE ( )  B_SPLINE_CURVE ( 2, ( #27343, #6002, #11101, #27191, #15255, #22301, #22459, #29342, #15579 ),
 .UNSPECIFIED., .F., .T. ) 
 B_SPLINE_CURVE_WITH_KNOTS ( ( 3, 2, 2, 2, 3 ),
 ( 0.05833333333333332732, 0.05925925925925926152, 0.06111111111111110911, 0.06296296296296295669, 0.06388888888888888395 ),
 .UNSPECIFIED. ) 
 CURVE ( )  GEOMETRIC_REPRESENTATION_ITEM ( )  RATIONAL_B_SPLINE_CURVE ( ( 0.9330127018922194093, 0.9330127018922189652, 1.000000000000000000, 0.8660254037844388186, 1.000000000000000000, 0.8660254037844388186, 1.000000000000000000, 0.9330127018922194093, 0.9330127018922194093 ) ) 
 REPRESENTATION_ITEM ( '' )  );
#14801=CARTESIAN_POINT ( 'NONE',  ( -4.763139720814407951, 2.749999999999946709, -133.2500000000000284 ) ) ;
#14802=VERTEX_POINT ( 'NONE', #1763 ) ;
#14805=CARTESIAN_POINT ( 'NONE',  ( -3.464101615137757051, -5.999999999999979572, -83.08632486540517448 ) ) ;
#14806=CARTESIAN_POINT ( 'NONE',  ( 0.000000000000000000, 5.499999999999991118, -55.49999999999999289 ) ) ;
#14807=CARTESIAN_POINT ( 'NONE',  ( 0.000000000000000000, -5.999999999999991118, -62.53867513459482552 ) ) ;
#14809=CARTESIAN_POINT ( 'NONE',  ( -3.608439182435052128, -6.250000000000110134, -76.30801270189225249 ) ) ;
#14810=CARTESIAN_POINT ( 'NONE',  ( 0.000000000000000000, 0.000000000000000000, -183.0000000000000000 ) ) ;
#14812=CARTESIAN_POINT ( 'NONE',  ( 0.000000000000000000, -5.999999999999991118, -168.4613248654052029 ) ) ;
#14815=EDGE_CURVE ( 'NONE', #29310, #27213, #29244, .T. ) ;
#14816=DIRECTION ( 'NONE',  ( -7.147005652999508048E-36, 5.642372883946980038E-36, 1.000000000000000000 ) ) ;
#14818=EDGE_CURVE ( 'NONE', #30239, #12335, #28030, .T. ) ;
#14819=CARTESIAN_POINT ( 'NONE',  ( -3.175426480542816066, -5.500000000000057732, -141.8750000000000568 ) ) ;
#14823=CARTESIAN_POINT ( 'NONE',  ( -4.763139720814407951, 2.749999999999946709, -67.25000000000002842 ) ) ;
#14824=CARTESIAN_POINT ( 'NONE',  ( -2.775557561562891351E-14, -5.500000000000115463, -60.75000000000002842 ) ) ;
#14831=CARTESIAN_POINT ( 'NONE',  ( 0.000000000000000000, 0.000000000000000000, 0.000000000000000000 ) ) ;
#14832=ORIENTED_EDGE ( 'NONE', *, *, #24184, .T. ) ;
#14836=CARTESIAN_POINT ( 'NONE',  ( -6.350852961085760029, -1.281975124255709124E-13, -178.1250000000000568 ) ) ;
#14838=CARTESIAN_POINT ( 'NONE',  ( 5.412658773652712085, -3.125000000000086153, -156.0669872981078754 ) ) ;
#14840=CARTESIAN_POINT ( 'NONE',  ( 6.350852961086080661, -9.614813431917819062E-14, -78.37500000000001421 ) ) ;
#14841=CARTESIAN_POINT ( 'NONE',  ( 2.775557561562891351E-14, -6.250000000000061284, -103.1830127018922241 ) ) ;
#14842=ORIENTED_EDGE ( 'NONE', *, *, #14781, .T. ) ;
#14843=CARTESIAN_POINT ( 'NONE',  ( -5.999999999999964473, 1.607695154586726405, -175.4806624327026441 ) ) ;
#14846=CARTESIAN_POINT ( 'NONE',  ( 5.608370619328757023, -9.463293048187454204, -22.85879529262368237 ) ) ;
#14848=CARTESIAN_POINT ( 'NONE',  ( 4.763139720814407951, 2.750000000000002665, -166.7500000000000000 ) ) ;
#14850=CARTESIAN_POINT ( 'NONE',  ( 0.000000000000000000, 5.499999999999991118, -147.0000000000000284 ) ) ;
#14853=CARTESIAN_POINT ( 'NONE',  ( -6.350852961085760029, -1.281975124255709124E-13, -95.62500000000004263 ) ) ;
#14854=CARTESIAN_POINT ( 'NONE',  ( -2.775557561562891351E-14, -5.500000000000115463, -80.25000000000004263 ) ) ;
#14855=CARTESIAN_POINT ( 'NONE',  ( -5.999999999999963585, 1.780251999655701777E-13, -72.83632486540523132 ) ) ;
#14856=CARTESIAN_POINT ( 'NONE',  ( 6.000000000000000888, 1.607695154586715303, -144.0193375672974696 ) ) ;
#14858=CARTESIAN_POINT ( 'NONE',  ( -5.999999999999963585, 8.134310703387671600E-14, -125.9136751345948397 ) ) ;
#14861=EDGE_LOOP ( 'NONE', ( #10882, #29101, #10880, #18779 ) ) ;
#14864=CARTESIAN_POINT ( 'NONE',  ( 3.464101615137852974, 5.999999999999884537, -80.83632486540523132 ) ) ;
#14867=ORIENTED_EDGE ( 'NONE', *, *, #15356, .F. ) ;
#14868=ADVANCED_FACE ( 'NONE', ( #5903 ), #3440, .T. ) ;
#14869=CARTESIAN_POINT ( 'NONE',  ( 6.350852961086080661, -9.614813431917819062E-14, -106.8750000000000142 ) ) ;
#14871=( BOUNDED_CURVE ( )  B_SPLINE_CURVE ( 2, ( #24335, #28789, #12715, #21615, #249, #546, #7602, #9632, #19026 ),
 .UNSPECIFIED., .F., .T. ) 
 B_SPLINE_CURVE_WITH_KNOTS ( ( 3, 2, 2, 2, 3 ),
 ( 0.4249999999999999334, 0.4259259259259259300, 0.4277777777777778123, 0.4296296296296295836, 0.4305555555555555802 ),
 .UNSPECIFIED. ) 
 CURVE ( )  GEOMETRIC_REPRESENTATION_ITEM ( )  RATIONAL_B_SPLINE_CURVE ( ( 0.9330127018922194093, 0.9330127018922154125, 1.000000000000000000, 0.8660254037844388186, 1.000000000000000000, 0.8660254037844388186, 1.000000000000000000, 0.9330127018922154125, 0.9330127018922194093 ) ) 
 REPRESENTATION_ITEM ( '' )  );
#14872=CARTESIAN_POINT ( 'NONE',  ( 5.412658773652739619, 3.124999999999988898, -125.1830127018922525 ) ) ;
#14874=VERTEX_POINT ( 'NONE', #22212 ) ;
#14875=CARTESIAN_POINT ( 'NONE',  ( 0.000000000000000000, -5.999999999999991118, -61.03867513459482552 ) ) ;
#14876=CARTESIAN_POINT ( 'NONE',  ( -3.608439182435052128, -6.250000000000110134, -162.4419872981077901 ) ) ;
#14878=CARTESIAN_POINT ( 'NONE',  ( -3.464101615137725076, 5.999999999999979572, -63.16367513459483973 ) ) ;
#14879=CARTESIAN_POINT ( 'NONE',  ( 3.608439182435180470, 6.249999999999982236, -63.55801270189224539 ) ) ;
#14881=CARTESIAN_POINT ( 'NONE',  ( 0.000000000000000000, 0.000000000000000000, 0.000000000000000000 ) ) ;
#14882=EDGE_CURVE ( 'NONE', #4876, #15344, #18479, .T. ) ;
#14883=CARTESIAN_POINT ( 'NONE',  ( 2.799076333356274106E-14, 11.00000000000000000, -19.00000000000002132 ) ) ;
#14884=CARTESIAN_POINT ( 'NONE',  ( 4.763139720814407951, 2.750000000000002665, -168.2500000000000000 ) ) ;
#14887=CARTESIAN_POINT ( 'NONE',  ( -5.412658773652739619, 3.124999999999975131, -171.1830127018922383 ) ) ;
#14890=CARTESIAN_POINT ( 'NONE',  ( -4.763139720814407951, 2.749999999999946709, -118.2500000000000284 ) ) ;
#14891=CARTESIAN_POINT ( 'NONE',  ( 4.763139720814407951, -2.749999999999988454, -114.5000000000000426 ) ) ;
#14893=DIRECTION ( 'NONE',  ( -7.147005652999508048E-36, 5.642372883946980038E-36, 1.000000000000000000 ) ) ;
#14897=CARTESIAN_POINT ( 'NONE',  ( -5.999999999999962697, 3.323446944526963891E-14, -162.8363248654052313 ) ) ;
#14900=CARTESIAN_POINT ( 'NONE',  ( -5.196152422706573404, -3.000000000000002665, -127.2886751345948539 ) ) ;
#14901=AXIS2_PLACEMENT_3D ( 'NONE', #19861, #29678, #20017 ) ;
#14902=CARTESIAN_POINT ( 'NONE',  ( 5.412658773652712085, -3.125000000000086153, -82.56698729810784698 ) ) ;
#14903=CARTESIAN_POINT ( 'NONE',  ( 5.196152422706629359, 3.000000000000002665, -110.0386751345948682 ) ) ;
#14905=CARTESIAN_POINT ( 'NONE',  ( 6.000000000000000888, 7.762456499804235646E-14, -138.6636751345948255 ) ) ;
#14907=VERTEX_POINT ( 'NONE', #22672 ) ;
#14908=ORIENTED_EDGE ( 'NONE', *, *, #27420, .F. ) ;
#14911=ORIENTED_EDGE ( 'NONE', *, *, #8067, .T. ) ;
#14912=CARTESIAN_POINT ( 'NONE',  ( 2.775557561562891351E-14, -6.250000000000061284, -129.3169872981078186 ) ) ;
#14913=CARTESIAN_POINT ( 'NONE',  ( -6.000000000000060396, -1.607695154586566089, -135.7693375672974412 ) ) ;
#14914=CARTESIAN_POINT ( 'NONE',  ( 0.000000000000000000, 0.000000000000000000, 0.000000000000000000 ) ) ;
#14920=CARTESIAN_POINT ( 'NONE',  ( 0.000000000000000000, -5.999999999999991118, -91.96132486540520290 ) ) ;
#14921=CARTESIAN_POINT ( 'NONE',  ( -5.196152422706601826, 2.999999999999975131, -56.46132486540522422 ) ) ;
#14923=CARTESIAN_POINT ( 'NONE',  ( 5.196152422706629359, -2.999999999999988898, -99.21132486540523132 ) ) ;
#14924=CARTESIAN_POINT ( 'NONE',  ( 6.000000000000000888, -1.859271017917181981E-14, -46.58632486540520290 ) ) ;
#14927=DIRECTION ( 'NONE',  ( 1.000000000000000000, -5.551115123125773458E-17, -1.260129944081490338E-35 ) ) ;
#14929=CARTESIAN_POINT ( 'NONE',  ( -5.999999999999963585, -2.788906526875773208E-15, -176.9136751345948539 ) ) ;
#14930=CARTESIAN_POINT ( 'NONE',  ( 6.350852961086080661, -9.614813431917819062E-14, -136.8750000000000568 ) ) ;
#14933=CARTESIAN_POINT ( 'NONE',  ( 6.350852961086080661, -9.614813431917819062E-14, -46.87500000000000000 ) ) ;
#14936=CARTESIAN_POINT ( 'NONE',  ( -5.999999999999956479, -1.607695154586745057, -164.2693375672974412 ) ) ;
#14937=VERTEX_POINT ( 'NONE', #11327 ) ;
#14941=CARTESIAN_POINT ( 'NONE',  ( -3.608439182435115633, 6.249999999999965361, -96.94198729810781856 ) ) ;
#14947=ORIENTED_EDGE ( 'NONE', *, *, #29597, .F. ) ;
#14949=CARTESIAN_POINT ( 'NONE',  ( 4.763139720814407951, 2.750000000000002665, -57.25000000000002132 ) ) ;
#14951=CARTESIAN_POINT ( 'NONE',  ( 3.464101615137757051, -5.999999999999979572, -62.41367513459483973 ) ) ;
#14953=CARTESIAN_POINT ( 'NONE',  ( -5.196152422706601826, 2.999999999999975131, -67.53867513459482552 ) ) ;
#14954=CARTESIAN_POINT ( 'NONE',  ( -3.608439182435115633, 6.249999999999965361, -72.30801270189222407 ) ) ;
#14957=CARTESIAN_POINT ( 'NONE',  ( -5.196152422706601826, 2.999999999999975131, -149.4613248654052029 ) ) ;
#14958=CARTESIAN_POINT ( 'NONE',  ( -5.196152422706573404, -3.000000000000002665, -168.7113248654051745 ) ) ;
#14960=CARTESIAN_POINT ( 'NONE',  ( 4.763139720814407951, -2.749999999999988454, -141.5000000000000284 ) ) ;
#14961=CARTESIAN_POINT ( 'NONE',  ( -3.608439182435052128, -6.250000000000110134, -154.3080127018922383 ) ) ;
#14964=CARTESIAN_POINT ( 'NONE',  ( -2.775557561562891351E-14, -5.500000000000115463, -72.75000000000004263 ) ) ;
#14965=CARTESIAN_POINT ( 'NONE',  ( 3.175426480543072749, -5.500000000000105693, -56.12500000000004263 ) ) ;
#14966=( BOUNDED_CURVE ( )  B_SPLINE_CURVE ( 2, ( #3306, #22687, #5915, #15496, #24505, #12733, #29259, #22072, #10407 ),
 .UNSPECIFIED., .F., .F. ) 
 B_SPLINE_CURVE_WITH_KNOTS ( ( 3, 2, 2, 2, 3 ),
 ( 0.5138888888888888395, 0.5148148148148148362, 0.5166666666666666075, 0.5185185185185186008, 0.5194444444444444864 ),
 .UNSPECIFIED. ) 
 CURVE ( )  GEOMETRIC_REPRESENTATION_ITEM ( )  RATIONAL_B_SPLINE_CURVE ( ( 0.9330127018922194093, 0.9330127018922154125, 1.000000000000000000, 0.8660254037844388186, 1.000000000000000000, 0.8660254037844388186, 1.000000000000000000, 0.9330127018922194093, 0.9330127018922194093 ) ) 
 REPRESENTATION_ITEM ( '' )  );
#14970=CARTESIAN_POINT ( 'NONE',  ( -5.999999999999971578, 1.607695154586715303, -126.9033121635129930 ) ) ;
#14973=VERTEX_POINT ( 'NONE', #23294 ) ;
#14977=EDGE_CURVE ( 'NONE', #16308, #8939, #4528, .T. ) ;
#14978=EDGE_CURVE ( 'NONE', #26678, #23883, #21776, .T. ) ;
#14979=CARTESIAN_POINT ( 'NONE',  ( -5.999999999999968026, -1.607695154586722186, -158.8466878364870070 ) ) ;
#14981=CARTESIAN_POINT ( 'NONE',  ( -3.608439182435052128, -6.250000000000110134, -148.9419872981078186 ) ) ;
#14982=CARTESIAN_POINT ( 'NONE',  ( -4.763139720814407951, -2.750000000000016431, -85.00000000000001421 ) ) ;
#14983=B_SPLINE_CURVE_WITH_KNOTS ( 'NONE', 3,
 ( #18379, #3895, #25095, #20215, #22357, #1293, #29563, #5895, #1607, #6215, #20051, #15322, #8681, #17776, #13326, #20506 ),
 .UNSPECIFIED., .F., .F.,
 ( 4, 2, 2, 2, 2, 2, 2, 4 ),
 ( 0.000000000000000000, 0.001747794382750394527, 0.002621691574125591898, 0.003495588765500789487, 0.004369485956875987509, 0.005243383148251184664, 0.006117280339626383553, 0.006991177531001582443 ),
 .UNSPECIFIED. ) ;
#14985=CARTESIAN_POINT ( 'NONE',  ( 5.412658773652739619, 3.124999999999988898, -95.18301270189222407 ) ) ;
#14989=FACE_OUTER_BOUND ( 'NONE', #1122, .T. ) ;
#14992=CARTESIAN_POINT ( 'NONE',  ( 6.350852961086080661, -9.614813431917819062E-14, -162.3750000000000284 ) ) ;
#14994=CARTESIAN_POINT ( 'NONE',  ( -4.763139720814407951, 2.749999999999946709, -149.7500000000000568 ) ) ;
#14996=CARTESIAN_POINT ( 'NONE',  ( -4.763139720814407951, 2.749999999999946709, -95.75000000000000000 ) ) ;
#14998=CARTESIAN_POINT ( 'NONE',  ( -5.999999999999904965, -1.607695154586834541, -131.2693375672974412 ) ) ;
#14999=CARTESIAN_POINT ( 'NONE',  ( 6.350852961086080661, -9.614813431917819062E-14, -81.37500000000004263 ) ) ;
#15002=DIRECTION ( 'NONE',  ( 7.147005652999508048E-36, -5.642372883946980038E-36, -1.000000000000000000 ) ) ;
#15003=( BOUNDED_CURVE ( )  B_SPLINE_CURVE ( 2, ( #21592, #22032, #14547, #23888, #7886, #3270, #5278, #29072, #5425 ),
 .UNSPECIFIED., .F., .F. ) 
 B_SPLINE_CURVE_WITH_KNOTS ( ( 3, 2, 2, 2, 3 ),
 ( 0.4138888888888888618, 0.4148148148148148584, 0.4166666666666666297, 0.4185185185185185119, 0.4194444444444445086 ),
 .UNSPECIFIED. ) 
 CURVE ( )  GEOMETRIC_REPRESENTATION_ITEM ( )  RATIONAL_B_SPLINE_CURVE ( ( 0.9330127018922194093, 0.9330127018922154125, 1.000000000000000000, 0.8660254037844388186, 1.000000000000000000, 0.8660254037844388186, 1.000000000000000000, 0.9330127018922154125, 0.9330127018922194093 ) ) 
 REPRESENTATION_ITEM ( '' )  );
#15006=( BOUNDED_CURVE ( )  B_SPLINE_CURVE ( 2, ( #25516, #9559, #16654, #9094, #23245, #13745, #8952, #6935, #30132 ),
 .UNSPECIFIED., .F., .F. ) 
 B_SPLINE_CURVE_WITH_KNOTS ( ( 3, 2, 2, 2, 3 ),
 ( 0.7972222222222222765, 0.7981481481481481621, 0.8000000000000000444, 0.8018518518518518157, 0.8027777777777777013 ),
 .UNSPECIFIED. ) 
 CURVE ( )  GEOMETRIC_REPRESENTATION_ITEM ( )  RATIONAL_B_SPLINE_CURVE ( ( 0.9330127018922194093, 0.9330127018922234061, 1.000000000000000000, 0.8660254037844388186, 1.000000000000000000, 0.8660254037844388186, 1.000000000000000000, 0.9330127018922234061, 0.9330127018922194093 ) ) 
 REPRESENTATION_ITEM ( '' )  );
#15007=CARTESIAN_POINT ( 'NONE',  ( 0.000000000000000000, 5.999999999999977796, -128.7113248654052029 ) ) ;
#15011=AXIS2_PLACEMENT_3D ( 'NONE', #29616, #29916, #22721 ) ;
#15018=EDGE_CURVE ( 'NONE', #15083, #9807, #8197, .T. ) ;
#15022=CARTESIAN_POINT ( 'NONE',  ( 4.763139720814407951, -2.749999999999988454, -105.5000000000000426 ) ) ;
#15023=CARTESIAN_POINT ( 'NONE',  ( 3.608439182435180470, -6.249999999999997335, -115.0580127018922383 ) ) ;
#15025=CARTESIAN_POINT ( 'NONE',  ( 0.000000000000000000, 0.000000000000000000, 0.000000000000000000 ) ) ;
#15026=CARTESIAN_POINT ( 'NONE',  ( -5.412658773652684552, -3.125000000000099920, -161.0669872981078754 ) ) ;
#15028=CARTESIAN_POINT ( 'NONE',  ( 2.775557561562891351E-14, 6.250000000000033751, -58.93301270189221697 ) ) ;
#15031=CARTESIAN_POINT ( 'NONE',  ( -4.754775042825807319, 9.920200456738779593, -21.33539821540184889 ) ) ;
#15033=CARTESIAN_POINT ( 'NONE',  ( -2.775557561562891351E-14, -5.500000000000115463, -174.7500000000000284 ) ) ;
#15036=CARTESIAN_POINT ( 'NONE',  ( 2.775557561562891351E-14, -6.250000000000061284, -167.6830127018922383 ) ) ;
#15038=DIRECTION ( 'NONE',  ( -7.147005652999508048E-36, 5.642372883946980038E-36, 1.000000000000000000 ) ) ;
#15039=CARTESIAN_POINT ( 'NONE',  ( -4.763139720814407951, -2.750000000000016431, -118.0000000000000000 ) ) ;
#15042=CARTESIAN_POINT ( 'NONE',  ( 6.350852961086080661, -9.614813431917819062E-14, -103.8750000000000000 ) ) ;
#15043=CARTESIAN_POINT ( 'NONE',  ( -5.999999999999982236, -1.607695154586700426, -131.8466878364870354 ) ) ;
#15044=ORIENTED_EDGE ( 'NONE', *, *, #2331, .F. ) ;
#15048=CARTESIAN_POINT ( 'NONE',  ( 0.000000000000000000, -5.999999999999991118, -76.03867513459483973 ) ) ;
#15049=ORIENTED_EDGE ( 'NONE', *, *, #6689, .F. ) ;
#15052=CARTESIAN_POINT ( 'NONE',  ( 2.775557561562891351E-14, -6.250000000000061284, -84.31698729810783277 ) ) ;
#15053=DIRECTION ( 'NONE',  ( 1.000000000000000000, -5.551115123125773458E-17, -1.260129944081490338E-35 ) ) ;
#15056=CARTESIAN_POINT ( 'NONE',  ( -6.000000000000000888, 1.067854986875958443E-15, 7.560779664488942560E-35 ) ) ;
#15057=( BOUNDED_CURVE ( )  B_SPLINE_CURVE ( 2, ( #15825, #26810, #13510, #27129, #22701, #15510, #11039, #8401, #15667 ),
 .UNSPECIFIED., .F., .T. ) 
 B_SPLINE_CURVE_WITH_KNOTS ( ( 3, 2, 2, 2, 3 ),
 ( 0.8916666666666666075, 0.8925925925925926041, 0.8944444444444444864, 0.8962962962962962576, 0.8972222222222222543 ),
 .UNSPECIFIED. ) 
 CURVE ( )  GEOMETRIC_REPRESENTATION_ITEM ( )  RATIONAL_B_SPLINE_CURVE ( ( 0.9330127018922194093, 0.9330127018922154125, 1.000000000000000000, 0.8660254037844388186, 1.000000000000000000, 0.8660254037844388186, 1.000000000000000000, 0.9330127018922154125, 0.9330127018922194093 ) ) 
 REPRESENTATION_ITEM ( '' )  );
#15058=EDGE_CURVE ( 'NONE', #22104, #9807, #13634, .T. ) ;
#15062=ORIENTED_EDGE ( 'NONE', *, *, #6087, .T. ) ;
#15063=CARTESIAN_POINT ( 'NONE',  ( 2.775557561562891351E-14, -6.250000000000061284, -135.3169872981078186 ) ) ;
#15065=CARTESIAN_POINT ( 'NONE',  ( 3.464101615137852974, 5.999999999999884537, -83.83632486540517448 ) ) ;
#15066=CARTESIAN_POINT ( 'NONE',  ( 3.464101615137852974, 5.999999999999884537, -47.83632486540520290 ) ) ;
#15067=EDGE_LOOP ( 'NONE', ( #24899, #265, #7041, #16521 ) ) ;
#15071=CARTESIAN_POINT ( 'NONE',  ( -3.464101615137725076, 5.999999999999979572, -56.58632486540519579 ) ) ;
#15075=CARTESIAN_POINT ( 'NONE',  ( -5.412658773652739619, 3.124999999999975131, -66.81698729810780435 ) ) ;
#15076=CARTESIAN_POINT ( 'NONE',  ( 2.775557561562891351E-14, 6.250000000000033751, -52.06698729810782567 ) ) ;
#15077=CARTESIAN_POINT ( 'NONE',  ( 6.000000000000000000, 2.951592740943527306E-14, -152.1636751345948255 ) ) ;
#15078=CARTESIAN_POINT ( 'NONE',  ( -5.999999999999963585, 1.780251999655701777E-13, -102.8363248654052313 ) ) ;
#15080=VECTOR ( 'NONE', #27222, 1000.000000000000000 ) ;
#15081=CARTESIAN_POINT ( 'NONE',  ( 3.175426480543072749, 5.499999999999865885, -130.6250000000000284 ) ) ;
#15083=VERTEX_POINT ( 'NONE', #20829 ) ;
#15086=CARTESIAN_POINT ( 'NONE',  ( 6.000000000000052403, 1.607695154586625819, -120.0193375672974412 ) ) ;
#15087=CARTESIAN_POINT ( 'NONE',  ( 3.464101615137757051, -5.999999999999979572, -159.9136751345947971 ) ) ;
#15094=CARTESIAN_POINT ( 'NONE',  ( 3.608439182435180470, 6.249999999999982236, -95.69198729810780435 ) ) ;
#15096=ADVANCED_FACE ( 'NONE', ( #9296 ), #16401, .T. ) ;
#15101=ORIENTED_EDGE ( 'NONE', *, *, #16372, .T. ) ;
#15104=EDGE_LOOP ( 'NONE', ( #9615, #27350, #7490, #18551 ) ) ;
#15106=CARTESIAN_POINT ( 'NONE',  ( 0.000000000000000000, 5.999999999999977796, -81.28867513459481131 ) ) ;
#15107=CARTESIAN_POINT ( 'NONE',  ( 4.763139720814407951, -2.749999999999988454, -48.49999999999998579 ) ) ;
#15108=( BOUNDED_CURVE ( )  B_SPLINE_CURVE ( 2, ( #621, #29157, #12782, #7821, #21684, #3512, #26563, #22277, #21974 ),
 .UNSPECIFIED., .F., .F. ) 
 B_SPLINE_CURVE_WITH_KNOTS ( ( 3, 2, 2, 2, 3 ),
 ( 0.3416666666666666741, 0.3425925925925926152, 0.3444444444444444420, 0.3462962962962962687, 0.3472222222222222099 ),
 .UNSPECIFIED. ) 
 CURVE ( )  GEOMETRIC_REPRESENTATION_ITEM ( )  RATIONAL_B_SPLINE_CURVE ( ( 0.9330127018922194093, 0.9330127018922194093, 1.000000000000000000, 0.8660254037844388186, 1.000000000000000000, 0.8660254037844388186, 1.000000000000000000, 0.9330127018922194093, 0.9330127018922194093 ) ) 
 REPRESENTATION_ITEM ( '' )  );
#15109=CARTESIAN_POINT ( 'NONE',  ( -5.999999999999963585, 1.780251999655701777E-13, -65.91367513459482552 ) ) ;
#15110=CARTESIAN_POINT ( 'NONE',  ( 2.775557561562891351E-14, 6.250000000000033751, -75.43301270189223828 ) ) ;
#15116=CARTESIAN_POINT ( 'NONE',  ( -4.763139720814407951, -2.750000000000016431, -134.5000000000000000 ) ) ;
#15117=CARTESIAN_POINT ( 'NONE',  ( 3.464101615137757051, -5.999999999999979572, -177.3363248654052313 ) ) ;
#15119=CARTESIAN_POINT ( 'NONE',  ( -5.196152422706601826, 2.999999999999975131, -51.03867513459481131 ) ) ;
#15121=CARTESIAN_POINT ( 'NONE',  ( 6.350852961086080661, -9.614813431917819062E-14, -66.37500000000002842 ) ) ;
#15123=CARTESIAN_POINT ( 'NONE',  ( -6.350852961085760029, -1.281975124255709124E-13, -58.12500000000005684 ) ) ;
#15124=CARTESIAN_POINT ( 'NONE',  ( 6.000000000000000888, -1.859271017917181981E-14, -124.5863248654052171 ) ) ;
#15127=DIRECTION ( 'NONE',  ( -3.885780586188043947E-16, 0.8660254037844514752, 0.4999999999999777955 ) ) ;
#15129=ADVANCED_BREP_SHAPE_REPRESENTATION ( '', ( #14742, #18805 ), #1599 ) ;
#15131=EDGE_CURVE ( 'NONE', #20541, #8489, #29186, .T. ) ;
#15132=EDGE_CURVE ( 'NONE', #3491, #16367, #12217, .T. ) ;
#15137=CARTESIAN_POINT ( 'NONE',  ( 4.763139720814407951, -2.749999999999988454, -149.0000000000000284 ) ) ;
#15139=VERTEX_POINT ( 'NONE', #17724 ) ;
#15140=CARTESIAN_POINT ( 'NONE',  ( 5.412658773652739619, 3.124999999999988898, -146.8169872981078186 ) ) ;
#15141=CARTESIAN_POINT ( 'NONE',  ( 6.350852961086080661, -9.614813431917819062E-14, -82.87500000000004263 ) ) ;
#15142=( BOUNDED_CURVE ( )  B_SPLINE_CURVE ( 2, ( #6869, #3001, #26491, #848, #17022, #3145, #10249, #14856, #19607 ),
 .UNSPECIFIED., .F., .T. ) 
 B_SPLINE_CURVE_WITH_KNOTS ( ( 3, 2, 2, 2, 3 ),
 ( 0.7194444444444444420, 0.7203703703703703276, 0.7222222222222222099, 0.7240740740740740922, 0.7249999999999999778 ),
 .UNSPECIFIED. ) 
 CURVE ( )  GEOMETRIC_REPRESENTATION_ITEM ( )  RATIONAL_B_SPLINE_CURVE ( ( 0.9330127018922194093, 0.9330127018922194093, 1.000000000000000000, 0.8660254037844388186, 1.000000000000000000, 0.8660254037844388186, 1.000000000000000000, 0.9330127018922194093, 0.9330127018922194093 ) ) 
 REPRESENTATION_ITEM ( '' )  );
#15143=CARTESIAN_POINT ( 'NONE',  ( -3.608439182435052128, -6.250000000000110134, -97.30801270189220986 ) ) ;
#15144=VERTEX_POINT ( 'NONE', #20623 ) ;
#15145=CARTESIAN_POINT ( 'NONE',  ( -3.464101615137757051, -5.999999999999979572, -128.0863248654052029 ) ) ;
#15150=CARTESIAN_POINT ( 'NONE',  ( -3.175426480542816066, 5.499999999999865885, -154.3749999999999716 ) ) ;
#15152=CARTESIAN_POINT ( 'NONE',  ( -4.763139720814407951, 2.749999999999946709, -143.7500000000000568 ) ) ;
#15155=CARTESIAN_POINT ( 'NONE',  ( -4.763139720814407951, -2.750000000000016431, -98.50000000000002842 ) ) ;
#15158=CARTESIAN_POINT ( 'NONE',  ( -2.775557561562891351E-14, -5.500000000000115463, -78.74999999999998579 ) ) ;
#15163=CARTESIAN_POINT ( 'NONE',  ( 6.000000000000000888, 7.762456499804234384E-14, -129.0863248654052029 ) ) ;
#15164=CARTESIAN_POINT ( 'NONE',  ( -3.464101615137725076, 5.999999999999979572, -72.16367513459481131 ) ) ;
#15165=ADVANCED_FACE ( 'NONE', ( #8796 ), #18182, .T. ) ;
#15166=CARTESIAN_POINT ( 'NONE',  ( 6.000000000000000888, 1.743066579297358182E-13, -75.66367513459485394 ) ) ;
#15167=ORIENTED_EDGE ( 'NONE', *, *, #24053, .T. ) ;
#15170=CARTESIAN_POINT ( 'NONE',  ( 0.000000000000000000, 5.999999999999977796, -80.71132486540521711 ) ) ;
#15173=EDGE_LOOP ( 'NONE', ( #10690, #23155 ) ) ;
#15174=CARTESIAN_POINT ( 'NONE',  ( 0.000000000000000000, 5.499999999999991118, -103.5000000000000426 ) ) ;
#15175=CARTESIAN_POINT ( 'NONE',  ( 3.608439182435180470, 6.249999999999982236, -113.0580127018922241 ) ) ;
#15177=FACE_OUTER_BOUND ( 'NONE', #633, .T. ) ;
#15178=CARTESIAN_POINT ( 'NONE',  ( -5.412658773652684552, -3.125000000000099920, -156.5669872981078186 ) ) ;
#15181=CARTESIAN_POINT ( 'NONE',  ( 3.608439182435180470, -6.249999999999997335, -55.05801270189220276 ) ) ;
#15183=ORIENTED_EDGE ( 'NONE', *, *, #22620, .T. ) ;
#15184=FACE_OUTER_BOUND ( 'NONE', #21486, .T. ) ;
#15185=CARTESIAN_POINT ( 'NONE',  ( -6.000000000000000888, 1.067854986875958443E-15, 7.560779664488942560E-35 ) ) ;
#15189=CARTESIAN_POINT ( 'NONE',  ( 0.000000000000000000, 5.499999999999991118, -168.0000000000000284 ) ) ;
#15192=CARTESIAN_POINT ( 'NONE',  ( 3.464101615137757051, -5.999999999999979572, -157.8363248654052029 ) ) ;
#15193=CARTESIAN_POINT ( 'NONE',  ( 3.608439182435180470, 6.249999999999982236, -171.5580127018922667 ) ) ;
#15199=CARTESIAN_POINT ( 'NONE',  ( 4.763139720814407951, 2.750000000000002665, -105.2500000000000142 ) ) ;
#15202=CARTESIAN_POINT ( 'NONE',  ( 6.000000000000052403, 1.607695154586625819, -145.5193375672974128 ) ) ;
#15205=CARTESIAN_POINT ( 'NONE',  ( 6.000000000000000888, 1.743066579297358182E-13, -90.08632486540521711 ) ) ;
#15208=CARTESIAN_POINT ( 'NONE',  ( 3.175426480543072749, 5.499999999999865885, -159.1250000000000000 ) ) ;
#15209=CARTESIAN_POINT ( 'NONE',  ( 3.464101615137852974, 5.999999999999884537, -156.4136751345947403 ) ) ;
#15210=CARTESIAN_POINT ( 'NONE',  ( 5.412658773652712085, -3.125000000000086153, -78.06698729810779014 ) ) ;
#15213=VERTEX_POINT ( 'NONE', #3853 ) ;
#15214=VECTOR ( 'NONE', #1919, 1000.000000000000000 ) ;
#15217=ORIENTED_EDGE ( 'NONE', *, *, #26541, .F. ) ;
#15220=CARTESIAN_POINT ( 'NONE',  ( -5.412658773652739619, 3.124999999999975131, -136.6830127018922099 ) ) ;
#15221=CARTESIAN_POINT ( 'NONE',  ( 2.775557561562891351E-14, 6.250000000000033751, -130.0669872981078470 ) ) ;
#15222=CARTESIAN_POINT ( 'NONE',  ( 2.775557561562891351E-14, 6.250000000000033751, -181.0669872981078186 ) ) ;
#15223=CARTESIAN_POINT ( 'NONE',  ( 3.175426480543072749, -5.500000000000105693, -173.1250000000000284 ) ) ;
#15224=FACE_OUTER_BOUND ( 'NONE', #18857, .T. ) ;
#15225=CARTESIAN_POINT ( 'NONE',  ( 0.000000000000000000, 5.999999999999977796, -47.71132486540518869 ) ) ;
#15232=CARTESIAN_POINT ( 'NONE',  ( 6.000000000000052403, -1.607695154586662678, -107.2306624327026157 ) ) ;
#15234=CARTESIAN_POINT ( 'NONE',  ( -5.412658773652739619, 3.124999999999975131, -69.81698729810781856 ) ) ;
#15235=CARTESIAN_POINT ( 'NONE',  ( 5.412658773652739619, 3.124999999999988898, -56.81698729810780435 ) ) ;
#15237=CARTESIAN_POINT ( 'NONE',  ( 3.464101615137852974, 5.999999999999884537, -103.3363248654052171 ) ) ;
#15238=CARTESIAN_POINT ( 'NONE',  ( -3.464101615137725076, 5.999999999999979572, -127.6636751345948113 ) ) ;
#15241=CARTESIAN_POINT ( 'NONE',  ( -3.175426480542816510, 5.499999999999865885, -130.3750000000000284 ) ) ;
#15242=CARTESIAN_POINT ( 'NONE',  ( -5.999999999999971578, 1.607695154586715303, -166.4806624327026157 ) ) ;
#15246=CARTESIAN_POINT ( 'NONE',  ( -5.999999999999963585, -1.487416814333745711E-14, -96.83632486540520290 ) ) ;
#15247=CARTESIAN_POINT ( 'NONE',  ( -5.196152422706573404, -3.000000000000002665, -100.2886751345948255 ) ) ;
#15249=( BOUNDED_CURVE ( )  B_SPLINE_CURVE ( 2, ( #18871, #13670, #4705, #11519, #23173, #20860, #9488, #14139, #11362 ),
 .UNSPECIFIED., .F., .T. ) 
 B_SPLINE_CURVE_WITH_KNOTS ( ( 3, 2, 2, 2, 3 ),
 ( 0.8361111111111111382, 0.8370370370370370239, 0.8388888888888889062, 0.8407407407407407884, 0.8416666666666666741 ),
 .UNSPECIFIED. ) 
 CURVE ( )  GEOMETRIC_REPRESENTATION_ITEM ( )  RATIONAL_B_SPLINE_CURVE ( ( 0.9330127018922194093, 0.9330127018922194093, 1.000000000000000000, 0.8660254037844388186, 1.000000000000000000, 0.8660254037844388186, 1.000000000000000000, 0.9330127018922194093, 0.9330127018922194093 ) ) 
 REPRESENTATION_ITEM ( '' )  );
#15252=CARTESIAN_POINT ( 'NONE',  ( 0.000000000000000000, 5.999999999999977796, -71.71132486540521711 ) ) ;
#15254=CARTESIAN_POINT ( 'NONE',  ( 2.775557561562891351E-14, 6.250000000000033751, -94.06698729810780435 ) ) ;
#15255=CARTESIAN_POINT ( 'NONE',  ( 0.000000000000000000, -5.999999999999991118, -173.5386751345948539 ) ) ;
#15259=CARTESIAN_POINT ( 'NONE',  ( 0.000000000000000000, 0.000000000000000000, 0.000000000000000000 ) ) ;
#15260=AXIS2_PLACEMENT_3D ( 'NONE', #9203, #18142, #16718 ) ;
#15264=CARTESIAN_POINT ( 'NONE',  ( 3.464101615137852974, 5.999999999999884537, -81.41367513459479710 ) ) ;
#15266=LINE ( 'NONE', #11110, #25538 ) ;
#15268=CARTESIAN_POINT ( 'NONE',  ( 5.412658773652739619, 3.124999999999988898, -72.68301270189225249 ) ) ;
#15269=CARTESIAN_POINT ( 'NONE',  ( 5.196152422706629359, -2.999999999999988898, -172.7113248654052029 ) ) ;
#15272=CARTESIAN_POINT ( 'NONE',  ( 6.000000000000000888, -3.330669073875464691E-16, -7.560779664488942560E-35 ) ) ;
#15273=CARTESIAN_POINT ( 'NONE',  ( 0.000000000000000000, 0.000000000000000000, 0.000000000000000000 ) ) ;
#15274=CARTESIAN_POINT ( 'NONE',  ( 6.000000000000014211, -1.607695154586730180, -152.2306624327025588 ) ) ;
#15276=ADVANCED_FACE ( 'NONE', ( #11585 ), #30390, .F. ) ;
#15277=CARTESIAN_POINT ( 'NONE',  ( -2.775557561562891351E-14, -5.500000000000115463, -132.7500000000000284 ) ) ;
#15282=CARTESIAN_POINT ( 'NONE',  ( 6.350852961086080661, -9.614813431917819062E-14, -61.87500000000000711 ) ) ;
#15283=CARTESIAN_POINT ( 'NONE',  ( 4.763139720814407951, -2.749999999999988454, -54.49999999999999289 ) ) ;
#15285=CARTESIAN_POINT ( 'NONE',  ( 3.464101615137757051, -5.999999999999979572, -174.3363248654051461 ) ) ;
#15286=VERTEX_POINT ( 'NONE', #16052 ) ;
#15292=CARTESIAN_POINT ( 'NONE',  ( -5.999999999999963585, 1.780251999655701777E-13, -89.33632486540523132 ) ) ;
#15298=ORIENTED_EDGE ( 'NONE', *, *, #8288, .F. ) ;
#15299=( BOUNDED_CURVE ( )  B_SPLINE_CURVE ( 2, ( #16799, #21081, #16938, #11736, #23831, #9854, #25827, #28559, #23976 ),
 .UNSPECIFIED., .F., .F. ) 
 B_SPLINE_CURVE_WITH_KNOTS ( ( 3, 2, 2, 2, 3 ),
 ( 0.3805555555555555358, 0.3814814814814814770, 0.3833333333333333592, 0.3851851851851851860, 0.3861111111111111271 ),
 .UNSPECIFIED. ) 
 CURVE ( )  GEOMETRIC_REPRESENTATION_ITEM ( )  RATIONAL_B_SPLINE_CURVE ( ( 0.9330127018922194093, 0.9330127018922174109, 1.000000000000000000, 0.8660254037844388186, 1.000000000000000000, 0.8660254037844388186, 1.000000000000000000, 0.9330127018922174109, 0.9330127018922194093 ) ) 
 REPRESENTATION_ITEM ( '' )  );
#15300=CARTESIAN_POINT ( 'NONE',  ( 3.175426480543072749, -5.500000000000105693, -146.1250000000000000 ) ) ;
#15301=CARTESIAN_POINT ( 'NONE',  ( -7.216878364870328078, 0.000000000000000000, -48.69198729810783277 ) ) ;
#15304=CARTESIAN_POINT ( 'NONE',  ( 3.608439182435180470, -6.249999999999997335, -150.1919872981078186 ) ) ;
#15306=CARTESIAN_POINT ( 'NONE',  ( 3.175426480543072749, 5.499999999999865885, -70.62500000000004263 ) ) ;
#15309=CARTESIAN_POINT ( 'NONE',  ( -3.608439182435115633, 6.249999999999965361, -93.30801270189219565 ) ) ;
#15310=CARTESIAN_POINT ( 'NONE',  ( 0.000000000000000000, 5.499999999999991118, -153.0000000000000284 ) ) ;
#15312=CARTESIAN_POINT ( 'NONE',  ( -3.199609099280245506, -10.52573284576702406, -30.07939160056616146 ) ) ;
#15316=EDGE_CURVE ( 'NONE', #16412, #17631, #24722, .T. ) ;
#15317=EDGE_CURVE ( 'NONE', #9511, #24851, #4621, .T. ) ;
#15318=CARTESIAN_POINT ( 'NONE',  ( -4.763139720814407951, -2.750000000000016431, -157.0000000000000284 ) ) ;
#15321=CARTESIAN_POINT ( 'NONE',  ( 3.175426480543072749, -5.500000000000105693, -143.1250000000000000 ) ) ;
#15322=CARTESIAN_POINT ( 'NONE',  ( -4.884531539219052476, 3.330387827114730914, -180.0000000000000284 ) ) ;
#15326=CARTESIAN_POINT ( 'NONE',  ( 0.000000000000000000, 5.499999999999991118, -84.00000000000001421 ) ) ;
#15328=CARTESIAN_POINT ( 'NONE',  ( 3.175426480543072749, -5.500000000000105693, -80.12500000000002842 ) ) ;
#15331=CARTESIAN_POINT ( 'NONE',  ( 3.464101615137852974, 5.999999999999884537, -164.8363248654052029 ) ) ;
#15334=CARTESIAN_POINT ( 'NONE',  ( 6.000000000000001776, 5.345404176511898156E-15, -179.1636751345948539 ) ) ;
#15335=CIRCLE ( 'NONE', #7934, 2.000000000000003109 ) ;
#15336=CARTESIAN_POINT ( 'NONE',  ( -3.464101615137725076, 5.999999999999979572, -134.5863248654051745 ) ) ;
#15337=CARTESIAN_POINT ( 'NONE',  ( 5.196152422706629359, 3.000000000000002665, -174.5386751345948539 ) ) ;
#15338=VERTEX_POINT ( 'NONE', #9399 ) ;
#15341=DIRECTION ( 'NONE',  ( 1.000000000000000000, -5.551115123125774074E-17, -1.260129944081490338E-35 ) ) ;
#15344=VERTEX_POINT ( 'NONE', #21230 ) ;
#15348=EDGE_CURVE ( 'NONE', #6076, #22729, #28706, .T. ) ;
#15349=CARTESIAN_POINT ( 'NONE',  ( 4.763139720814407951, 2.750000000000002665, -94.75000000000000000 ) ) ;
#15351=CARTESIAN_POINT ( 'NONE',  ( 3.608439182435180470, 6.249999999999982236, -116.0580127018922383 ) ) ;
#15354=CARTESIAN_POINT ( 'NONE',  ( 3.608439182435180470, -6.249999999999997335, -49.05801270189224539 ) ) ;
#15355=VERTEX_POINT ( 'NONE', #19670 ) ;
#15356=EDGE_CURVE ( 'NONE', #19518, #18212, #12196, .T. ) ;
#15357=CARTESIAN_POINT ( 'NONE',  ( 0.000000000000000000, -5.999999999999991118, -119.5386751345948255 ) ) ;
#15358=LINE ( 'NONE', #24681, #26741 ) ;
#15360=CARTESIAN_POINT ( 'NONE',  ( 4.763139720814407951, -2.749999999999988454, -170.0000000000000284 ) ) ;
#15362=CARTESIAN_POINT ( 'NONE',  ( -5.412658773652684552, -3.125000000000099920, -172.4330127018922667 ) ) ;
#15363=FACE_OUTER_BOUND ( 'NONE', #9641, .T. ) ;
#15364=CARTESIAN_POINT ( 'NONE',  ( 4.763139720814407951, 2.750000000000002665, -109.7500000000000142 ) ) ;
#15365=FACE_OUTER_BOUND ( 'NONE', #1356, .T. ) ;
#15366=CARTESIAN_POINT ( 'NONE',  ( -3.175426480542816510, 5.499999999999865885, -106.3750000000000284 ) ) ;
#15369=CARTESIAN_POINT ( 'NONE',  ( 0.000000000000000000, 5.999999999999977796, -162.2886751345948824 ) ) ;
#15375=ORIENTED_EDGE ( 'NONE', *, *, #15927, .T. ) ;
#15376=CARTESIAN_POINT ( 'NONE',  ( -7.216878364870328078, 0.000000000000000000, -80.19198729810784698 ) ) ;
#15377=CARTESIAN_POINT ( 'NONE',  ( -5.999999999999963585, 1.780251999655701777E-13, -103.4136751345948255 ) ) ;
#15379=DIRECTION ( 'NONE',  ( -7.147005652999508048E-36, 5.642372883946980038E-36, 1.000000000000000000 ) ) ;
#15380=VECTOR ( 'NONE', #17241, 1000.000000000000000 ) ;
#15381=ORIENTED_EDGE ( 'NONE', *, *, #907, .F. ) ;
#15385=CARTESIAN_POINT ( 'NONE',  ( 3.175426480543072749, -5.500000000000105693, -131.1250000000000000 ) ) ;
#15386=EDGE_CURVE ( 'NONE', #10812, #15497, #23832, .T. ) ;
#15388=CARTESIAN_POINT ( 'NONE',  ( -5.412658773652739619, 3.124999999999975131, -138.1830127018922667 ) ) ;
#15390=CARTESIAN_POINT ( 'NONE',  ( 5.412658773652712085, -3.125000000000086153, -121.5669872981078328 ) ) ;
#15392=CARTESIAN_POINT ( 'NONE',  ( -4.763139720814407951, -2.750000000000016431, -169.0000000000000284 ) ) ;
#15393=CARTESIAN_POINT ( 'NONE',  ( 6.000000000000000888, -1.859271017917181981E-14, -131.1636751345948539 ) ) ;
#15397=CARTESIAN_POINT ( 'NONE',  ( 0.000000000000000000, 0.000000000000000000, 0.000000000000000000 ) ) ;
#15403=CARTESIAN_POINT ( 'NONE',  ( 5.412658773652739619, 3.124999999999988898, -64.31698729810780435 ) ) ;
#15404=CARTESIAN_POINT ( 'NONE',  ( -3.608439182435115633, 6.249999999999965361, -53.44198729810779724 ) ) ;
#15408=CARTESIAN_POINT ( 'NONE',  ( -2.775557561562891351E-14, -5.500000000000115463, -126.7500000000000284 ) ) ;
#15410=ORIENTED_EDGE ( 'NONE', *, *, #8813, .F. ) ;
#15413=CARTESIAN_POINT ( 'NONE',  ( 0.000000000000000000, -5.999999999999991118, -160.0386751345948539 ) ) ;
#15414=CARTESIAN_POINT ( 'NONE',  ( 6.000000000000000888, -3.330669073875464691E-16, -7.560779664488942560E-35 ) ) ;
#15419=CARTESIAN_POINT ( 'NONE',  ( 5.412658773652739619, 3.124999999999988898, -118.3169872981078043 ) ) ;
#15420=CARTESIAN_POINT ( 'NONE',  ( 5.196152422706629359, -2.999999999999988898, -54.21132486540525264 ) ) ;
#15421=CARTESIAN_POINT ( 'NONE',  ( -3.464101615137725076, 5.999999999999979572, -91.08632486540520290 ) ) ;
#15423=VERTEX_POINT ( 'NONE', #14495 ) ;
#15430=CARTESIAN_POINT ( 'NONE',  ( 4.763139720814407951, -2.749999999999988454, -50.00000000000004263 ) ) ;
#15432=CARTESIAN_POINT ( 'NONE',  ( 6.000000000000000888, -1.859271017917181981E-14, -130.5863248654052313 ) ) ;
#15433=CARTESIAN_POINT ( 'NONE',  ( 0.000000000000000000, 0.000000000000000000, 0.000000000000000000 ) ) ;
#15434=CARTESIAN_POINT ( 'NONE',  ( 7.216878364870455975, -6.409875621278545621E-14, -77.30801270189223828 ) ) ;
#15435=CARTESIAN_POINT ( 'NONE',  ( 0.000000000000000000, 0.000000000000000000, 0.000000000000000000 ) ) ;
#15440=( BOUNDED_CURVE ( )  B_SPLINE_CURVE ( 2, ( #28293, #14378, #3387, #15264, #15106, #3541, #27045, #1402, #17568 ),
 .UNSPECIFIED., .F., .T. ) 
 B_SPLINE_CURVE_WITH_KNOTS ( ( 3, 2, 2, 2, 3 ),
 ( 0.7416666666666666963, 0.7425925925925925819, 0.7444444444444444642, 0.7462962962962963465, 0.7472222222222222321 ),
 .UNSPECIFIED. ) 
 CURVE ( )  GEOMETRIC_REPRESENTATION_ITEM ( )  RATIONAL_B_SPLINE_CURVE ( ( 0.9330127018922194093, 0.9330127018922234061, 1.000000000000000000, 0.8660254037844388186, 1.000000000000000000, 0.8660254037844388186, 1.000000000000000000, 0.9330127018922194093, 0.9330127018922194093 ) ) 
 REPRESENTATION_ITEM ( '' )  );
#15441=CARTESIAN_POINT ( 'NONE',  ( 4.763139720814407951, 2.750000000000002665, -130.7500000000000284 ) ) ;
#15442=CARTESIAN_POINT ( 'NONE',  ( 5.196152422706629359, -2.999999999999988898, -177.2113248654052597 ) ) ;
#15444=CARTESIAN_POINT ( 'NONE',  ( 5.999999999999949374, 1.607695154586804565, -178.5193375672974412 ) ) ;
#15446=CARTESIAN_POINT ( 'NONE',  ( 3.175426480543072749, 5.499999999999865885, -63.12500000000001421 ) ) ;
#15448=CARTESIAN_POINT ( 'NONE',  ( 3.175426480543072749, 5.499999999999865885, -60.12499999999999289 ) ) ;
#15449=CARTESIAN_POINT ( 'NONE',  ( -5.999999999999963585, -1.487416814333745711E-14, -170.3363248654052313 ) ) ;
#15455=CARTESIAN_POINT ( 'NONE',  ( -5.196152422706573404, -3.000000000000002665, -49.28867513459483973 ) ) ;
#15456=VERTEX_POINT ( 'NONE', #9856 ) ;
#15460=CARTESIAN_POINT ( 'NONE',  ( 3.175426480543072749, -5.500000000000105693, -144.6250000000000000 ) ) ;
#15461=EDGE_CURVE ( 'NONE', #4790, #15666, #15529, .T. ) ;
#15463=CARTESIAN_POINT ( 'NONE',  ( 7.216878364870455975, -6.409875621278545621E-14, -50.94198729810784698 ) ) ;
#15466=CARTESIAN_POINT ( 'NONE',  ( 4.763139720814407951, 2.750000000000002665, -73.75000000000004263 ) ) ;
#15467=CARTESIAN_POINT ( 'NONE',  ( 3.608439182435180470, 6.249999999999982236, -92.05801270189226670 ) ) ;
#15468=CARTESIAN_POINT ( 'NONE',  ( -6.000000000000000888, 1.067854986875958443E-15, 7.560779664488942560E-35 ) ) ;
#15474=CARTESIAN_POINT ( 'NONE',  ( 0.000000000000000000, 5.499999999999991118, -154.5000000000000284 ) ) ;
#15477=CARTESIAN_POINT ( 'NONE',  ( 4.763139720814407951, -2.749999999999988454, -87.50000000000002842 ) ) ;
#15480=CARTESIAN_POINT ( 'NONE',  ( 0.000000000000000000, 5.499999999999991118, -84.00000000000001421 ) ) ;
#15481=CARTESIAN_POINT ( 'NONE',  ( -6.000000000000000888, 1.067854986875958443E-15, 7.560779664488942560E-35 ) ) ;
#15484=CARTESIAN_POINT ( 'NONE',  ( 5.196152422706629359, -2.999999999999988898, -108.2113248654051887 ) ) ;
#15485=CARTESIAN_POINT ( 'NONE',  ( -3.464101615137725076, 5.999999999999979572, -103.6636751345948255 ) ) ;
#15488=CARTESIAN_POINT ( 'NONE',  ( 3.464101615137757051, -5.999999999999979572, -165.3363248654051745 ) ) ;
#15489=( BOUNDED_CURVE ( )  B_SPLINE_CURVE ( 2, ( #24375, #3466, #24080, #7937, #17046, #26522, #3319, #12901, #22086 ),
 .UNSPECIFIED., .F., .F. ) 
 B_SPLINE_CURVE_WITH_KNOTS ( ( 3, 2, 2, 2, 3 ),
 ( 0.4750000000000000333, 0.4759259259259259189, 0.4777777777777778012, 0.4796296296296296280, 0.4805555555555555136 ),
 .UNSPECIFIED. ) 
 CURVE ( )  GEOMETRIC_REPRESENTATION_ITEM ( )  RATIONAL_B_SPLINE_CURVE ( ( 0.9330127018922194093, 0.9330127018922214077, 1.000000000000000000, 0.8660254037844388186, 1.000000000000000000, 0.8660254037844388186, 1.000000000000000000, 0.9330127018922214077, 0.9330127018922194093 ) ) 
 REPRESENTATION_ITEM ( '' )  );
#15490=CARTESIAN_POINT ( 'NONE',  ( -6.000000000000000888, 1.067854986875958443E-15, 7.560779664488942560E-35 ) ) ;
#15491=VERTEX_POINT ( 'NONE', #10007 ) ;
#15493=FACE_OUTER_BOUND ( 'NONE', #6736, .T. ) ;
#15496=CARTESIAN_POINT ( 'NONE',  ( 3.464101615137757051, -5.999999999999979572, -115.8363248654052171 ) ) ;
#15497=VERTEX_POINT ( 'NONE', #16939 ) ;
#15500=CARTESIAN_POINT ( 'NONE',  ( 3.175426480543072749, 5.499999999999865885, -94.62500000000002842 ) ) ;
#15501=CARTESIAN_POINT ( 'NONE',  ( -3.464101615137757051, -5.999999999999979572, -89.66367513459485394 ) ) ;
#15502=CARTESIAN_POINT ( 'NONE',  ( -3.608439182435115633, 6.249999999999965361, -118.8080127018922525 ) ) ;
#15503=ORIENTED_EDGE ( 'NONE', *, *, #11015, .T. ) ;
#15504=CARTESIAN_POINT ( 'NONE',  ( 6.000000000000000888, 1.743066579297358182E-13, -92.16367513459482552 ) ) ;
#15505=CARTESIAN_POINT ( 'NONE',  ( 3.464101615137852974, 5.999999999999884537, -63.41367513459483973 ) ) ;
#15507=CARTESIAN_POINT ( 'NONE',  ( 2.775557561562891351E-14, 6.250000000000033751, -49.93301270189220986 ) ) ;
#15508=ORIENTED_EDGE ( 'NONE', *, *, #17486, .T. ) ;
#15510=CARTESIAN_POINT ( 'NONE',  ( -3.464101615137757051, -5.999999999999979572, -167.0863248654051461 ) ) ;
#15512=CARTESIAN_POINT ( 'NONE',  ( 4.763139720814407951, -2.749999999999988454, -171.5000000000000000 ) ) ;
#15514=CARTESIAN_POINT ( 'NONE',  ( -5.412658773652684552, -3.125000000000099920, -163.4330127018922667 ) ) ;
#15517=CARTESIAN_POINT ( 'NONE',  ( -3.175426480542816510, -5.500000000000057732, -108.8750000000000426 ) ) ;
#15520=CARTESIAN_POINT ( 'NONE',  ( -5.999999999999956479, -1.607695154586745057, -87.76933756729744118 ) ) ;
#15522=CARTESIAN_POINT ( 'NONE',  ( 2.676951800742168933E-14, -11.00000000000000000, -19.00000000000002132 ) ) ;
#15523=ORIENTED_EDGE ( 'NONE', *, *, #16785, .F. ) ;
#15528=CARTESIAN_POINT ( 'NONE',  ( -3.464101615137757051, -5.999999999999979572, -134.0863248654051745 ) ) ;
#15529=( BOUNDED_CURVE ( )  B_SPLINE_CURVE ( 2, ( #7392, #24258, #21537, #21686, #14920, #7677, #3066, #12491, #26120 ),
 .UNSPECIFIED., .F., .F. ) 
 B_SPLINE_CURVE_WITH_KNOTS ( ( 3, 2, 2, 2, 3 ),
 ( 0.3361111111111110272, 0.3370370370370370239, 0.3388888888888889062, 0.3407407407407407884, 0.3416666666666666741 ),
 .UNSPECIFIED. ) 
 CURVE ( )  GEOMETRIC_REPRESENTATION_ITEM ( )  RATIONAL_B_SPLINE_CURVE ( ( 0.9330127018922194093, 0.9330127018922154125, 1.000000000000000000, 0.8660254037844388186, 1.000000000000000000, 0.8660254037844388186, 1.000000000000000000, 0.9330127018922194093, 0.9330127018922194093 ) ) 
 REPRESENTATION_ITEM ( '' )  );
#15530=ORIENTED_EDGE ( 'NONE', *, *, #25761, .F. ) ;
#15531=CARTESIAN_POINT ( 'NONE',  ( 4.763139720814407951, 2.750000000000002665, -157.7500000000000568 ) ) ;
#15533=AXIS2_PLACEMENT_3D ( 'NONE', #7301, #28469, #518 ) ;
#15534=CARTESIAN_POINT ( 'NONE',  ( 5.412658773652712085, -3.125000000000086153, -79.56698729810784698 ) ) ;
#15537=EDGE_CURVE ( 'NONE', #28127, #8469, #13372, .T. ) ;
#15541=CARTESIAN_POINT ( 'NONE',  ( 3.175426480543072749, -5.500000000000105693, -120.6250000000000284 ) ) ;
#15542=CARTESIAN_POINT ( 'NONE',  ( 5.412658773652739619, 3.124999999999988898, -137.1830127018922667 ) ) ;
#15545=CARTESIAN_POINT ( 'NONE',  ( -3.608439182435115633, 6.249999999999965361, -125.4419872981078043 ) ) ;
#15546=CARTESIAN_POINT ( 'NONE',  ( 3.175426480543072749, 5.499999999999865885, -171.1250000000000000 ) ) ;
#15549=CARTESIAN_POINT ( 'NONE',  ( 6.000000000000000888, 1.743066579297358182E-13, -48.08632486540521711 ) ) ;
#15553=CARTESIAN_POINT ( 'NONE',  ( 5.999999999999999112, 2.951592740943527306E-14, -148.5863248654052313 ) ) ;
#15555=DIRECTION ( 'NONE',  ( -7.147005652999508048E-36, 5.642372883946980038E-36, 1.000000000000000000 ) ) ;
#15558=CARTESIAN_POINT ( 'NONE',  ( -5.412658773652739619, 3.124999999999975131, -71.31698729810781856 ) ) ;
#15560=CARTESIAN_POINT ( 'NONE',  ( 5.412658773652739619, 3.124999999999988898, -52.31698729810785409 ) ) ;
#15561=DIRECTION ( 'NONE',  ( -7.147005652999508048E-36, 5.642372883946980038E-36, 1.000000000000000000 ) ) ;
#15564=CARTESIAN_POINT ( 'NONE',  ( -3.175426480542816510, 5.499999999999865885, -133.3750000000000284 ) ) ;
#15565=CARTESIAN_POINT ( 'NONE',  ( 5.196152422706629359, 3.000000000000002665, -50.96132486540522422 ) ) ;
#15567=ORIENTED_EDGE ( 'NONE', *, *, #22466, .F. ) ;
#15569=CYLINDRICAL_SURFACE ( 'NONE', #2794, 6.000000000000000888 ) ;
#15578=CARTESIAN_POINT ( 'NONE',  ( 7.216878364870455975, -6.409875621278545621E-14, -115.4419872981078328 ) ) ;
#15579=CARTESIAN_POINT ( 'NONE',  ( 6.000000000000000888, -1.859271017917181981E-14, -173.1636751345948539 ) ) ;
#15584=ORIENTED_EDGE ( 'NONE', *, *, #5819, .T. ) ;
#15586=CARTESIAN_POINT ( 'NONE',  ( -3.175426480542816510, -5.500000000000057732, -53.37500000000002842 ) ) ;
#15587=PRODUCT_DEFINITION_SHAPE ( 'NONE', 'NONE',  #6719 ) ;
#15588=CARTESIAN_POINT ( 'NONE',  ( -3.464101615137725076, 5.999999999999979572, -120.1636751345947829 ) ) ;
#15590=CARTESIAN_POINT ( 'NONE',  ( -5.412658773652684552, -3.125000000000099920, -65.93301270189222407 ) ) ;
#15591=DIRECTION ( 'NONE',  ( -7.147005652999508048E-36, 5.642372883946980038E-36, 1.000000000000000000 ) ) ;
#15593=DIRECTION ( 'NONE',  ( 1.000000000000000000, -5.551115123125773458E-17, -1.260129944081490338E-35 ) ) ;
#15597=CARTESIAN_POINT ( 'NONE',  ( -6.350852961085760029, -1.281975124255709124E-13, -133.1250000000000284 ) ) ;
#15598=MECHANICAL_DESIGN_GEOMETRIC_PRESENTATION_REPRESENTATION('',(#10736),#9696);
#15599=CARTESIAN_POINT ( 'NONE',  ( 5.412658773652712085, -3.125000000000086153, -149.4330127018922383 ) ) ;
#15600=DIRECTION ( 'NONE',  ( 1.000000000000000000, -5.551115123125773458E-17, -1.260129944081490338E-35 ) ) ;
#15603=CARTESIAN_POINT ( 'NONE',  ( -4.763139720814407951, -2.750000000000016431, -62.50000000000000000 ) ) ;
#15604=CARTESIAN_POINT ( 'NONE',  ( 5.196152422706629359, 3.000000000000002665, -172.4613248654052313 ) ) ;
#15606=CARTESIAN_POINT ( 'NONE',  ( -5.999999999999963585, 1.780251999655701777E-13, -56.91367513459483973 ) ) ;
#15607=EDGE_LOOP ( 'NONE', ( #5610, #419, #11053, #6111 ) ) ;
#15612=CYLINDRICAL_SURFACE ( 'NONE', #5242, 6.000000000000000888 ) ;
#15614=ORIENTED_EDGE ( 'NONE', *, *, #21949, .T. ) ;
#15617=VERTEX_POINT ( 'NONE', #3513 ) ;
#15618=( BOUNDED_CURVE ( )  B_SPLINE_CURVE ( 2, ( #15760, #27825, #18354, #27670, #24774, #29835, #15604, #13149, #29679 ),
 .UNSPECIFIED., .F., .T. ) 
 B_SPLINE_CURVE_WITH_KNOTS ( ( 3, 2, 2, 2, 3 ),
 ( 0.9305555555555555802, 0.9314814814814814659, 0.9333333333333333481, 0.9351851851851852304, 0.9361111111111111160 ),
 .UNSPECIFIED. ) 
 CURVE ( )  GEOMETRIC_REPRESENTATION_ITEM ( )  RATIONAL_B_SPLINE_CURVE ( ( 0.9330127018922194093, 0.9330127018922234061, 1.000000000000000000, 0.8660254037844388186, 1.000000000000000000, 0.8660254037844388186, 1.000000000000000000, 0.9330127018922194093, 0.9330127018922194093 ) ) 
 REPRESENTATION_ITEM ( '' )  );
#15619=CARTESIAN_POINT ( 'NONE',  ( 3.175426480543072749, 5.499999999999865885, -147.1250000000000284 ) ) ;
#15620=ORIENTED_EDGE ( 'NONE', *, *, #570, .F. ) ;
#15622=ORIENTED_EDGE ( 'NONE', *, *, #29154, .F. ) ;
#15623=CARTESIAN_POINT ( 'NONE',  ( -6.350852961085760029, -1.281975124255709124E-13, -70.12500000000005684 ) ) ;
#15625=CARTESIAN_POINT ( 'NONE',  ( 7.216878364870455975, -6.409875621278545621E-14, -95.30801270189220986 ) ) ;
#15626=( BOUNDED_CURVE ( )  B_SPLINE_CURVE ( 2, ( #25086, #18369, #1900, #23119, #16083, #23423, #18519, #11771, #6811 ),
 .UNSPECIFIED., .F., .T. ) 
 B_SPLINE_CURVE_WITH_KNOTS ( ( 3, 2, 2, 2, 3 ),
 ( 0.1249999999999999861, 0.1259259259259259134, 0.1277777777777777679, 0.1296296296296296224, 0.1305555555555555636 ),
 .UNSPECIFIED. ) 
 CURVE ( )  GEOMETRIC_REPRESENTATION_ITEM ( )  RATIONAL_B_SPLINE_CURVE ( ( 0.9330127018922194093, 0.9330127018922189652, 1.000000000000000000, 0.8660254037844388186, 1.000000000000000000, 0.8660254037844388186, 1.000000000000000000, 0.9330127018922184101, 0.9330127018922194093 ) ) 
 REPRESENTATION_ITEM ( '' )  );
#15627=CARTESIAN_POINT ( 'NONE',  ( -1.971541444415825683, -10.82814027403871471, -30.68027829220104863 ) ) ;
#15628=CARTESIAN_POINT ( 'NONE',  ( 3.464101615137852974, 5.999999999999884537, -106.9136751345947971 ) ) ;
#15631=CARTESIAN_POINT ( 'NONE',  ( 3.175426480543072749, -5.500000000000105693, -153.6250000000000568 ) ) ;
#15633=CARTESIAN_POINT ( 'NONE',  ( -5.999999999999963585, 1.780251999655701777E-13, -48.83632486540521711 ) ) ;
#15634=CARTESIAN_POINT ( 'NONE',  ( -3.175426480542816066, 5.499999999999865885, -86.87500000000007105 ) ) ;
#15637=CARTESIAN_POINT ( 'NONE',  ( -2.775557561562891351E-14, -5.500000000000115463, -75.75000000000004263 ) ) ;
#15638=ADVANCED_FACE ( 'NONE', ( #11234 ), #18001, .T. ) ;
#15640=CARTESIAN_POINT ( 'NONE',  ( -5.999999999999971578, 1.607695154586715303, -164.4033121635129930 ) ) ;
#15641=DIRECTION ( 'NONE',  ( -7.147005652999508048E-36, 5.642372883946980038E-36, 1.000000000000000000 ) ) ;
#15643=CARTESIAN_POINT ( 'NONE',  ( 3.464101615137852974, 5.999999999999884537, -103.9136751345948255 ) ) ;
#15646=CYLINDRICAL_SURFACE ( 'NONE', #12093, 6.000000000000000888 ) ;
#15647=ORIENTED_EDGE ( 'NONE', *, *, #20639, .F. ) ;
#15649=DIRECTION ( 'NONE',  ( 1.000000000000000000, -5.551115123125774690E-17, -1.260129944081490338E-35 ) ) ;
#15650=CARTESIAN_POINT ( 'NONE',  ( -5.196152422706573404, -3.000000000000002665, -172.2886751345948255 ) ) ;
#15653=DIRECTION ( 'NONE',  ( 1.000000000000000000, -5.551115123125773458E-17, -1.260129944081490338E-35 ) ) ;
#15656=CARTESIAN_POINT ( 'NONE',  ( -2.775557561562891351E-14, -5.500000000000115463, -99.75000000000000000 ) ) ;
#15657=DIRECTION ( 'NONE',  ( 1.000000000000000000, -5.551115123125773458E-17, -1.260129944081490338E-35 ) ) ;
#15658=CARTESIAN_POINT ( 'NONE',  ( -7.216878364870328078, 0.000000000000000000, -115.5580127018922383 ) ) ;
#15659=ORIENTED_EDGE ( 'NONE', *, *, #25861, .T. ) ;
#15660=CARTESIAN_POINT ( 'NONE',  ( 5.196152422706629359, 3.000000000000002665, -92.03867513459485394 ) ) ;
#15662=EDGE_CURVE ( 'NONE', #21925, #20404, #11406, .T. ) ;
#15663=CARTESIAN_POINT ( 'NONE',  ( -3.464101615137757051, -5.999999999999979572, -143.6636751345948255 ) ) ;
#15665=CARTESIAN_POINT ( 'NONE',  ( 3.608439182435180470, 6.249999999999982236, -48.55801270189223828 ) ) ;
#15666=VERTEX_POINT ( 'NONE', #10781 ) ;
#15667=CARTESIAN_POINT ( 'NONE',  ( -5.999999999999963585, -1.487416814333745711E-14, -167.3363248654052029 ) ) ;
#15668=CARTESIAN_POINT ( 'NONE',  ( 3.175426480543072749, -5.500000000000105693, -161.1250000000000284 ) ) ;
#15670=CARTESIAN_POINT ( 'NONE',  ( 5.999999999999999112, 2.951592740943527306E-14, -157.5863248654052313 ) ) ;
#15671=CARTESIAN_POINT ( 'NONE',  ( -4.763139720814407951, -2.750000000000016431, -106.0000000000000426 ) ) ;
#15674=CARTESIAN_POINT ( 'NONE',  ( -4.763139720814407951, 2.749999999999946709, -97.25000000000000000 ) ) ;
#15675=ADVANCED_FACE ( 'NONE', ( #29473 ), #4126, .T. ) ;
#15678=CARTESIAN_POINT ( 'NONE',  ( 5.196152422706629359, -2.999999999999988898, -84.21132486540521711 ) ) ;
#15683=ORIENTED_EDGE ( 'NONE', *, *, #1925, .T. ) ;
#15685=CARTESIAN_POINT ( 'NONE',  ( 3.608439182435180470, -6.249999999999997335, -88.69198729810783277 ) ) ;
#15686=CARTESIAN_POINT ( 'NONE',  ( -5.999999999999956479, -1.607695154586745057, -97.34668783648704959 ) ) ;
#15687=ORIENTED_EDGE ( 'NONE', *, *, #21507, .F. ) ;
#15688=CARTESIAN_POINT ( 'NONE',  ( -0.8024951133111937196, 10.97768020916284648, -30.95935331155643411 ) ) ;
#15689=CARTESIAN_POINT ( 'NONE',  ( -4.763139720814407951, -2.750000000000016431, -151.0000000000000284 ) ) ;
#15691=ORIENTED_EDGE ( 'NONE', *, *, #12241, .T. ) ;
#15693=CARTESIAN_POINT ( 'NONE',  ( -3.175426480542816510, -5.500000000000057732, -120.8750000000000284 ) ) ;
#15694=CARTESIAN_POINT ( 'NONE',  ( 3.608439182435180470, 6.249999999999982236, -140.0580127018922383 ) ) ;
#15696=CARTESIAN_POINT ( 'NONE',  ( 6.000000000000000888, -3.330669073875464691E-16, -7.560779664488942560E-35 ) ) ;
#15697=CARTESIAN_POINT ( 'NONE',  ( 3.608439182435180470, -6.249999999999997335, -121.6919872981077901 ) ) ;
#15698=CARTESIAN_POINT ( 'NONE',  ( -7.216878364870328078, 0.000000000000000000, -174.6919872981077901 ) ) ;
#15699=CARTESIAN_POINT ( 'NONE',  ( 0.000000000000000000, 5.499999999999991118, -175.5000000000000000 ) ) ;
#15703=ORIENTED_EDGE ( 'NONE', *, *, #17359, .T. ) ;
#15705=CARTESIAN_POINT ( 'NONE',  ( 0.000000000000000000, 0.000000000000000000, 0.000000000000000000 ) ) ;
#15706=CARTESIAN_POINT ( 'NONE',  ( -3.464101615137757051, -5.999999999999979572, -117.5863248654052171 ) ) ;
#15710=CARTESIAN_POINT ( 'NONE',  ( 2.775557561562891351E-14, 6.250000000000033751, -71.56698729810784698 ) ) ;
#15711=CARTESIAN_POINT ( 'NONE',  ( 2.775557561562891351E-14, -6.250000000000061284, -52.81698729810779724 ) ) ;
#15712=CARTESIAN_POINT ( 'NONE',  ( 0.000000000000000000, -5.999999999999991118, -121.0386751345948824 ) ) ;
#15713=CARTESIAN_POINT ( 'NONE',  ( -4.763139720814407951, 2.749999999999946709, -47.75000000000001421 ) ) ;
#15716=ADVANCED_FACE ( 'NONE', ( #26852 ), #6138, .T. ) ;
#15718=CARTESIAN_POINT ( 'NONE',  ( 0.000000000000000000, 5.499999999999991118, -129.0000000000000000 ) ) ;
#15719=EDGE_CURVE ( 'NONE', #1672, #4112, #3719, .T. ) ;
#15722=CARTESIAN_POINT ( 'NONE',  ( -5.196152422706601826, 2.999999999999975131, -132.0386751345948255 ) ) ;
#15725=VECTOR ( 'NONE', #19812, 1000.000000000000000 ) ;
#15726=ORIENTED_EDGE ( 'NONE', *, *, #1608, .F. ) ;
#15729=CARTESIAN_POINT ( 'NONE',  ( -5.412658773652739619, 3.124999999999975131, -113.3169872981077901 ) ) ;
#15732=LINE ( 'NONE', #22764, #1733 ) ;
#15737=CARTESIAN_POINT ( 'NONE',  ( 6.350852961086080661, -9.614813431917819062E-14, -49.87500000000001421 ) ) ;
#15739=VECTOR ( 'NONE', #17348, 1000.000000000000000 ) ;
#15743=CARTESIAN_POINT ( 'NONE',  ( -7.216878364870328078, 0.000000000000000000, -64.55801270189225249 ) ) ;
#15746=FACE_OUTER_BOUND ( 'NONE', #17045, .T. ) ;
#15747=CARTESIAN_POINT ( 'NONE',  ( 2.775557561562891351E-14, 10.99999999999998224, -14.99152654425661702 ) ) ;
#15753=CARTESIAN_POINT ( 'NONE',  ( 4.763139720814407951, -2.749999999999988454, -135.5000000000000000 ) ) ;
#15754=CARTESIAN_POINT ( 'NONE',  ( 3.608439182435180470, 6.249999999999982236, -149.0580127018922667 ) ) ;
#15755=CARTESIAN_POINT ( 'NONE',  ( 0.000000000000000000, 0.000000000000000000, 0.000000000000000000 ) ) ;
#15757=VERTEX_POINT ( 'NONE', #20891 ) ;
#15758=CARTESIAN_POINT ( 'NONE',  ( 4.763139720814407951, 2.750000000000002665, -64.75000000000002842 ) ) ;
#15759=CARTESIAN_POINT ( 'NONE',  ( 0.000000000000000000, 0.000000000000000000, 0.000000000000000000 ) ) ;
#15760=CARTESIAN_POINT ( 'NONE',  ( -5.999999999999963585, -1.487416814333745711E-14, -171.8363248654052313 ) ) ;
#15761=CARTESIAN_POINT ( 'NONE',  ( 5.196152422706629359, -2.999999999999988898, -162.7886751345948255 ) ) ;
#15766=( BOUNDED_CURVE ( )  B_SPLINE_CURVE ( 2, ( #14346, #16797, #23684, #17083, #2621, #12041, #16936, #14491, #5214 ),
 .UNSPECIFIED., .F., .F. ) 
 B_SPLINE_CURVE_WITH_KNOTS ( ( 3, 2, 2, 2, 3 ),
 ( 0.3861111111111111271, 0.3870370370370370128, 0.3888888888888888951, 0.3907407407407407218, 0.3916666666666666630 ),
 .UNSPECIFIED. ) 
 CURVE ( )  GEOMETRIC_REPRESENTATION_ITEM ( )  RATIONAL_B_SPLINE_CURVE ( ( 0.9330127018922194093, 0.9330127018922214077, 1.000000000000000000, 0.8660254037844388186, 1.000000000000000000, 0.8660254037844388186, 1.000000000000000000, 0.9330127018922194093, 0.9330127018922194093 ) ) 
 REPRESENTATION_ITEM ( '' )  );
#15769=AXIS2_PLACEMENT_3D ( 'NONE', #27687, #6670, #20919 ) ;
#15772=VERTEX_POINT ( 'NONE', #2691 ) ;
#15774=CARTESIAN_POINT ( 'NONE',  ( -3.175426480542816510, -5.500000000000057732, -149.3750000000000284 ) ) ;
#15775=VERTEX_POINT ( 'NONE', #18300 ) ;
#15778=CARTESIAN_POINT ( 'NONE',  ( -4.763139720814407951, -2.750000000000016431, -76.00000000000001421 ) ) ;
#15781=CARTESIAN_POINT ( 'NONE',  ( -3.608439182435052128, -6.250000000000110134, -88.30801270189222407 ) ) ;
#15782=ORIENTED_EDGE ( 'NONE', *, *, #221, .T. ) ;
#15783=CARTESIAN_POINT ( 'NONE',  ( -1.584453406822390775, -10.89233254831498598, -19.19936552286312903 ) ) ;
#15784=CARTESIAN_POINT ( 'NONE',  ( -5.999999999999962697, 3.323446944526963891E-14, -149.9136751345948255 ) ) ;
#15785=FACE_OUTER_BOUND ( 'NONE', #8070, .T. ) ;
#15787=CARTESIAN_POINT ( 'NONE',  ( -5.999999999999963585, 1.780251999655701777E-13, -91.41367513459486815 ) ) ;
#15789=CARTESIAN_POINT ( 'NONE',  ( 3.175426480543072749, -5.500000000000105693, -156.6250000000000000 ) ) ;
#15792=CARTESIAN_POINT ( 'NONE',  ( 3.175426480543072749, -5.500000000000105693, -86.12500000000000000 ) ) ;
#15793=DIRECTION ( 'NONE',  ( 1.000000000000000000, -5.551115123125773458E-17, -1.260129944081490338E-35 ) ) ;
#15794=CARTESIAN_POINT ( 'NONE',  ( 3.175426480543072749, 5.499999999999865885, -73.62500000000005684 ) ) ;
#15795=CARTESIAN_POINT ( 'NONE',  ( 6.000000000000052403, -1.607695154586662678, -74.23066243270258724 ) ) ;
#15797=CARTESIAN_POINT ( 'NONE',  ( 5.196152422706629359, -2.999999999999988898, -174.7886751345948255 ) ) ;
#15798=CARTESIAN_POINT ( 'NONE',  ( -5.196152422706573404, -3.000000000000002665, -76.28867513459481131 ) ) ;
#15799=CARTESIAN_POINT ( 'NONE',  ( 5.999999999999992006, -3.330669073875460254E-16, -44.99152654425658682 ) ) ;
#15801=CYLINDRICAL_SURFACE ( 'NONE', #28219, 6.000000000000000888 ) ;
#15802=( BOUNDED_CURVE ( )  B_SPLINE_CURVE ( 2, ( #403, #7760, #2566, #23919, #9792, #14439, #19469, #17025, #16592 ),
 .UNSPECIFIED., .F., .F. ) 
 B_SPLINE_CURVE_WITH_KNOTS ( ( 3, 2, 2, 2, 3 ),
 ( 0.1472222222222221433, 0.1481481481481481399, 0.1500000000000000222, 0.1518518518518519045, 0.1527777777777777901 ),
 .UNSPECIFIED. ) 
 CURVE ( )  GEOMETRIC_REPRESENTATION_ITEM ( )  RATIONAL_B_SPLINE_CURVE ( ( 0.9330127018922194093, 0.9330127018922154125, 1.000000000000000000, 0.8660254037844388186, 1.000000000000000000, 0.8660254037844388186, 1.000000000000000000, 0.9330127018922194093, 0.9330127018922194093 ) ) 
 REPRESENTATION_ITEM ( '' )  );
#15805=CARTESIAN_POINT ( 'NONE',  ( -3.464101615137757051, -5.999999999999979572, -109.1636751345948113 ) ) ;
#15808=CARTESIAN_POINT ( 'NONE',  ( 3.464101615137852974, 5.999999999999884537, -179.8363248654051745 ) ) ;
#15810=( BOUNDED_CURVE ( )  B_SPLINE_CURVE ( 2, ( #16214, #25368, #13753, #27969, #5488, #28677, #10587, #12608, #19938 ),
 .UNSPECIFIED., .F., .T. ) 
 B_SPLINE_CURVE_WITH_KNOTS ( ( 3, 2, 2, 2, 3 ),
 ( 0.2861111111111111494, 0.2870370370370370350, 0.2888888888888888618, 0.2907407407407407440, 0.2916666666666666297 ),
 .UNSPECIFIED. ) 
 CURVE ( )  GEOMETRIC_REPRESENTATION_ITEM ( )  RATIONAL_B_SPLINE_CURVE ( ( 0.9330127018922194093, 0.9330127018922214077, 1.000000000000000000, 0.8660254037844388186, 1.000000000000000000, 0.8660254037844388186, 1.000000000000000000, 0.9330127018922214077, 0.9330127018922194093 ) ) 
 REPRESENTATION_ITEM ( '' )  );
#15813=CARTESIAN_POINT ( 'NONE',  ( 3.175426480543072749, 5.499999999999865885, -100.6250000000000000 ) ) ;
#15814=DIRECTION ( 'NONE',  ( -7.147005652999508048E-36, 5.642372883946980038E-36, 1.000000000000000000 ) ) ;
#15816=CARTESIAN_POINT ( 'NONE',  ( 2.775557561562891351E-14, -6.250000000000061284, -104.6830127018922241 ) ) ;
#15817=ORIENTED_EDGE ( 'NONE', *, *, #4523, .F. ) ;
#15821=CARTESIAN_POINT ( 'NONE',  ( 3.608439182435180470, -6.249999999999997335, -53.55801270189220276 ) ) ;
#15823=ORIENTED_EDGE ( 'NONE', *, *, #14788, .F. ) ;
#15825=CARTESIAN_POINT ( 'NONE',  ( 6.000000000000000888, -1.859271017917181981E-14, -166.5863248654052029 ) ) ;
#15826=CARTESIAN_POINT ( 'NONE',  ( -2.775557561562891351E-14, -5.500000000000115463, -162.7500000000000000 ) ) ;
#15830=CARTESIAN_POINT ( 'NONE',  ( 3.175426480543072749, 5.499999999999865885, -106.6250000000000284 ) ) ;
#15832=DIRECTION ( 'NONE',  ( -7.147005652999508048E-36, 5.642372883946980038E-36, 1.000000000000000000 ) ) ;
#15833=CARTESIAN_POINT ( 'NONE',  ( -3.175426480542816510, -5.500000000000057732, -101.3750000000000000 ) ) ;
#15842=EDGE_LOOP ( 'NONE', ( #13892, #28889, #11995, #25109 ) ) ;
#15845=EDGE_CURVE ( 'NONE', #9966, #12627, #14534, .T. ) ;
#15846=CARTESIAN_POINT ( 'NONE',  ( -3.608439182435115633, 6.249999999999965361, -90.94198729810784698 ) ) ;
#15847=CARTESIAN_POINT ( 'NONE',  ( 6.000000000000000888, 1.743066579297358182E-13, -102.6636751345948397 ) ) ;
#15853=CARTESIAN_POINT ( 'NONE',  ( -6.350852961085760029, -1.281975124255709124E-13, -118.1250000000000142 ) ) ;
#15854=ADVANCED_FACE ( 'NONE', ( #13705 ), #9928, .T. ) ;
#15855=CARTESIAN_POINT ( 'NONE',  ( 3.608439182435180470, 6.249999999999982236, -137.0580127018922099 ) ) ;
#15857=CARTESIAN_POINT ( 'NONE',  ( -6.000000000000007105, -1.607695154586655129, -57.76933756729741276 ) ) ;
#15858=CARTESIAN_POINT ( 'NONE',  ( -5.412658773652684552, -3.125000000000099920, -125.0669872981078328 ) ) ;
#15859=CARTESIAN_POINT ( 'NONE',  ( 7.216878364870455975, -6.409875621278545621E-14, -176.9419872981078754 ) ) ;
#15862=( BOUNDED_CURVE ( )  B_SPLINE_CURVE ( 2, ( #23399, #25679, #6639, #15910, #2345, #23093, #29673, #11278, #11442 ),
 .UNSPECIFIED., .F., .F. ) 
 B_SPLINE_CURVE_WITH_KNOTS ( ( 3, 2, 2, 2, 3 ),
 ( 0.5083333333333333037, 0.5092592592592593004, 0.5111111111111110716, 0.5129629629629629539, 0.5138888888888888395 ),
 .UNSPECIFIED. ) 
 CURVE ( )  GEOMETRIC_REPRESENTATION_ITEM ( )  RATIONAL_B_SPLINE_CURVE ( ( 0.9330127018922194093, 0.9330127018922154125, 1.000000000000000000, 0.8660254037844388186, 1.000000000000000000, 0.8660254037844388186, 1.000000000000000000, 0.9330127018922234061, 0.9330127018922194093 ) ) 
 REPRESENTATION_ITEM ( '' )  );
#15863=ORIENTED_EDGE ( 'NONE', *, *, #19031, .F. ) ;
#15864=DIRECTION ( 'NONE',  ( -7.147005652999508048E-36, 5.642372883946980038E-36, 1.000000000000000000 ) ) ;
#15865=CARTESIAN_POINT ( 'NONE',  ( 5.999999999999949374, 1.607695154586804565, -90.59668783648706381 ) ) ;
#15869=CARTESIAN_POINT ( 'NONE',  ( -5.412658773652739619, 3.124999999999975131, -72.81698729810781856 ) ) ;
#15870=CARTESIAN_POINT ( 'NONE',  ( -3.608439182435052128, -6.250000000000110134, -58.94198729810782567 ) ) ;
#15871=CARTESIAN_POINT ( 'NONE',  ( -5.196152422706573404, -3.000000000000002665, -121.2886751345948539 ) ) ;
#15872=CARTESIAN_POINT ( 'NONE',  ( 4.763139720814407951, -2.749999999999988454, -51.49999999999999289 ) ) ;
#15873=CARTESIAN_POINT ( 'NONE',  ( 6.000000000000000000, 2.951592740943527306E-14, -149.1636751345948824 ) ) ;
#15875=CARTESIAN_POINT ( 'NONE',  ( -4.763139720814407951, 2.749999999999946709, -122.7500000000000284 ) ) ;
#15876=LINE ( 'NONE', #11245, #6839 ) ;
#15879=CARTESIAN_POINT ( 'NONE',  ( 3.464101615137852974, 5.999999999999884537, -132.4136751345947971 ) ) ;
#15880=CARTESIAN_POINT ( 'NONE',  ( -5.999999999999963585, -1.487416814333745711E-14, -122.3363248654052029 ) ) ;
#15882=ORIENTED_EDGE ( 'NONE', *, *, #16511, .F. ) ;
#15884=LINE ( 'NONE', #22611, #23940 ) ;
#15886=CARTESIAN_POINT ( 'NONE',  ( 7.216878364870455975, -6.409875621278545621E-14, -118.4419872981078470 ) ) ;
#15887=CARTESIAN_POINT ( 'NONE',  ( 3.464101615137757051, -5.999999999999979572, -54.33632486540517448 ) ) ;
#15890=ORIENTED_EDGE ( 'NONE', *, *, #18370, .F. ) ;
#15895=CARTESIAN_POINT ( 'NONE',  ( 5.412658773652739619, 3.124999999999988898, -143.8169872981078186 ) ) ;
#15896=ORIENTED_EDGE ( 'NONE', *, *, #17184, .F. ) ;
#15900=CARTESIAN_POINT ( 'NONE',  ( 5.196152422706629359, 3.000000000000002665, -62.03867513459482552 ) ) ;
#15901=CARTESIAN_POINT ( 'NONE',  ( 2.775557561562891351E-14, 6.250000000000033751, -70.93301270189222407 ) ) ;
#15908=CARTESIAN_POINT ( 'NONE',  ( -5.999999999999963585, 8.134310703387671600E-14, -146.9136751345948255 ) ) ;
#15910=CARTESIAN_POINT ( 'NONE',  ( -3.464101615137725076, 5.999999999999979572, -115.0863248654051887 ) ) ;
#15912=CARTESIAN_POINT ( 'NONE',  ( -3.175426480542816066, 5.499999999999865885, -121.3750000000000284 ) ) ;
#15913=DIRECTION ( 'NONE',  ( 1.000000000000000000, -5.551115123125773458E-17, -1.260129944081490338E-35 ) ) ;
#15914=CARTESIAN_POINT ( 'NONE',  ( 7.216878364870455975, -6.409875621278545621E-14, -144.8080127018922667 ) ) ;
#15915=DIRECTION ( 'NONE',  ( -7.147005652999508048E-36, 5.642372883946980038E-36, 1.000000000000000000 ) ) ;
#15917=CARTESIAN_POINT ( 'NONE',  ( 0.000000000000000000, 5.499999999999991118, -54.00000000000004974 ) ) ;
#15927=EDGE_CURVE ( 'NONE', #25700, #11104, #20615, .T. ) ;
#15928=CARTESIAN_POINT ( 'NONE',  ( 0.000000000000000000, 5.499999999999991118, -138.0000000000000000 ) ) ;
#15932=CARTESIAN_POINT ( 'NONE',  ( 3.175426480543072749, -5.500000000000105693, -72.62500000000005684 ) ) ;
#15934=CARTESIAN_POINT ( 'NONE',  ( -5.381246803625084674, -9.595437032880933970, -22.31808132294487734 ) ) ;
#15935=CARTESIAN_POINT ( 'NONE',  ( -5.999999999999971578, 1.607695154586715303, -106.4806624327025872 ) ) ;
#15937=CARTESIAN_POINT ( 'NONE',  ( -6.000000000000000888, 1.067854986875958443E-15, 7.560779664488942560E-35 ) ) ;
#15939=CARTESIAN_POINT ( 'NONE',  ( -3.175426480542816066, -5.500000000000057732, -149.3750000000000284 ) ) ;
#15941=CARTESIAN_POINT ( 'NONE',  ( 6.000000000000000888, 1.743066579297358182E-13, -95.16367513459482552 ) ) ;
#15942=CARTESIAN_POINT ( 'NONE',  ( 4.763139720814407951, 2.750000000000002665, -84.25000000000004263 ) ) ;
#15944=CARTESIAN_POINT ( 'NONE',  ( 4.763139720814407951, -2.749999999999988454, -77.00000000000001421 ) ) ;
#15946=CARTESIAN_POINT ( 'NONE',  ( -5.999999999999963585, 8.134310703387671600E-14, -114.8363248654052171 ) ) ;
#15947=FACE_OUTER_BOUND ( 'NONE', #13992, .T. ) ;
#15951=EDGE_CURVE ( 'NONE', #26678, #23968, #8357, .T. ) ;
#15953=CARTESIAN_POINT ( 'NONE',  ( 6.000000000000052403, -1.607695154586662678, -97.65331216351302146 ) ) ;
#15954=ADVANCED_FACE ( 'NONE', ( #19453 ), #20044, .T. ) ;
#15958=DIRECTION ( 'NONE',  ( -7.147005652999508048E-36, 5.642372883946980038E-36, 1.000000000000000000 ) ) ;
#15962=CARTESIAN_POINT ( 'NONE',  ( 3.175426480543072749, 5.499999999999865885, -99.12500000000005684 ) ) ;
#15964=CARTESIAN_POINT ( 'NONE',  ( -7.216878364870328078, 0.000000000000000000, -108.0580127018922667 ) ) ;
#15965=ORIENTED_EDGE ( 'NONE', *, *, #15018, .T. ) ;
#15967=CARTESIAN_POINT ( 'NONE',  ( -6.350852961085760029, -1.281975124255709124E-13, -149.6250000000000568 ) ) ;
#15968=CARTESIAN_POINT ( 'NONE',  ( -4.763139720814407951, -2.750000000000016431, -163.0000000000000284 ) ) ;
#15969=CARTESIAN_POINT ( 'NONE',  ( 3.464101615137757051, -5.999999999999979572, -105.9136751345947829 ) ) ;
#15971=CARTESIAN_POINT ( 'NONE',  ( 6.000000000000000888, 1.607695154586715303, -160.5193375672974128 ) ) ;
#15974=CARTESIAN_POINT ( 'NONE',  ( 0.000000000000000000, 5.499999999999991118, -163.5000000000000284 ) ) ;
#15976=CARTESIAN_POINT ( 'NONE',  ( 4.763139720814407951, -2.749999999999988454, -111.5000000000000426 ) ) ;
#15977=CARTESIAN_POINT ( 'NONE',  ( -3.464101615137725076, 5.999999999999979572, -87.16367513459483973 ) ) ;
#15978=( BOUNDED_CURVE ( )  B_SPLINE_CURVE ( 2, ( #12018, #21355, #293, #9681, #594, #19070, #28679, #3043, #749 ),
 .UNSPECIFIED., .F., .T. ) 
 B_SPLINE_CURVE_WITH_KNOTS ( ( 3, 2, 2, 2, 3 ),
 ( 0.6861111111111111160, 0.6870370370370370017, 0.6888888888888888840, 0.6907407407407407662, 0.6916666666666666519 ),
 .UNSPECIFIED. ) 
 CURVE ( )  GEOMETRIC_REPRESENTATION_ITEM ( )  RATIONAL_B_SPLINE_CURVE ( ( 0.9330127018922194093, 0.9330127018922194093, 1.000000000000000000, 0.8660254037844388186, 1.000000000000000000, 0.8660254037844388186, 1.000000000000000000, 0.9330127018922194093, 0.9330127018922194093 ) ) 
 REPRESENTATION_ITEM ( '' )  );
#15979=CARTESIAN_POINT ( 'NONE',  ( -3.175426480542816510, 5.499999999999865885, -95.87500000000002842 ) ) ;
#15981=( LENGTH_UNIT ( ) NAMED_UNIT ( * ) SI_UNIT ( .MILLI., .METRE. ) );
#15983=ORIENTED_EDGE ( 'NONE', *, *, #25503, .T. ) ;
#15986=CARTESIAN_POINT ( 'NONE',  ( 0.000000000000000000, 5.999999999999977796, -130.2113248654052029 ) ) ;
#15987=VECTOR ( 'NONE', #20151, 1000.000000000000000 ) ;
#15991=( BOUNDED_CURVE ( )  B_SPLINE_CURVE ( 2, ( #22798, #27072, #15455, #13157, #20190, #29542, #8498, #24925, #13304 ),
 .UNSPECIFIED., .F., .T. ) 
 B_SPLINE_CURVE_WITH_KNOTS ( ( 3, 2, 2, 2, 3 ),
 ( 0.9805555555555555136, 0.9814814814814815103, 0.9833333333333332815, 0.9851851851851851638, 0.9861111111111111605 ),
 .UNSPECIFIED. ) 
 CURVE ( )  GEOMETRIC_REPRESENTATION_ITEM ( )  RATIONAL_B_SPLINE_CURVE ( ( 0.9330127018922194093, 0.9330127018922154125, 1.000000000000000000, 0.8660254037844388186, 1.000000000000000000, 0.8660254037844388186, 1.000000000000000000, 0.9330127018922154125, 0.9330127018922194093 ) ) 
 REPRESENTATION_ITEM ( '' )  );
#15992=EDGE_LOOP ( 'NONE', ( #19799, #18320, #9014, #15647 ) ) ;
#15995=CARTESIAN_POINT ( 'NONE',  ( -5.412658773652739619, 3.124999999999975131, -87.81698729810783277 ) ) ;
#15997=CARTESIAN_POINT ( 'NONE',  ( -5.380679364423349043, 9.595766763449166348, -27.68326114948589733 ) ) ;
#15998=VERTEX_POINT ( 'NONE', #5434 ) ;
#15999=ORIENTED_EDGE ( 'NONE', *, *, #25458, .T. ) ;
#16002=CARTESIAN_POINT ( 'NONE',  ( -3.175426480542816510, -5.500000000000057732, -123.8749999999999716 ) ) ;
#16004=CARTESIAN_POINT ( 'NONE',  ( -7.216878364870328078, 0.000000000000000000, -132.0580127018922383 ) ) ;
#16006=CARTESIAN_POINT ( 'NONE',  ( 3.608439182435180470, -6.249999999999997335, -169.6919872981078470 ) ) ;
#16007=CARTESIAN_POINT ( 'NONE',  ( 2.775557561562891351E-14, 6.250000000000033751, -178.0669872981078186 ) ) ;
#16012=CARTESIAN_POINT ( 'NONE',  ( 5.196152422706629359, 3.000000000000002665, -54.53867513459481842 ) ) ;
#16013=CARTESIAN_POINT ( 'NONE',  ( 5.630955349231442142, 2.071796769705314123, -180.0000000000000568 ) ) ;
#16016=CARTESIAN_POINT ( 'NONE',  ( -5.412658773652684552, -3.125000000000099920, -74.06698729810784698 ) ) ;
#16017=CARTESIAN_POINT ( 'NONE',  ( 2.775557561562891351E-14, 6.250000000000033751, -58.06698729810783277 ) ) ;
#16019=CYLINDRICAL_SURFACE ( 'NONE', #9328, 6.000000000000000888 ) ;
#16020=CARTESIAN_POINT ( 'NONE',  ( -5.412658773652684552, -3.125000000000099920, -181.4330127018922667 ) ) ;
#16021=CARTESIAN_POINT ( 'NONE',  ( 6.000000000000052403, -1.607695154586662678, -111.1533121635129504 ) ) ;
#16022=CARTESIAN_POINT ( 'NONE',  ( -5.999999999999963585, -1.487416814333745711E-14, -123.8363248654052171 ) ) ;
#16023=CARTESIAN_POINT ( 'NONE',  ( -3.464101615137757051, -5.999999999999979572, -177.5863248654051745 ) ) ;
#16024=CARTESIAN_POINT ( 'NONE',  ( 6.350852961086080661, -9.614813431917819062E-14, -124.8749999999999858 ) ) ;
#16025=CARTESIAN_POINT ( 'NONE',  ( -3.175426480542816510, 5.499999999999865885, -157.3750000000000000 ) ) ;
#16026=CARTESIAN_POINT ( 'NONE',  ( 0.000000000000000000, 5.999999999999977796, -138.2886751345947971 ) ) ;
#16027=CARTESIAN_POINT ( 'NONE',  ( 0.000000000000000000, 0.000000000000000000, 0.000000000000000000 ) ) ;
#16030=CARTESIAN_POINT ( 'NONE',  ( 6.000000000000000888, -1.859271017917181981E-14, -105.6636751345948397 ) ) ;
#16034=ORIENTED_EDGE ( 'NONE', *, *, #6509, .T. ) ;
#16038=CARTESIAN_POINT ( 'NONE',  ( 5.412658773652739619, 3.124999999999988898, -115.3169872981078043 ) ) ;
#16039=CARTESIAN_POINT ( 'NONE',  ( 0.000000000000000000, 5.999999999999977796, -108.2886751345948397 ) ) ;
#16045=CARTESIAN_POINT ( 'NONE',  ( -3.608439182435052128, -6.250000000000110134, -144.4419872981078470 ) ) ;
#16052=CARTESIAN_POINT ( 'NONE',  ( 6.000000000000000000, 2.951592740943527306E-14, -151.5863248654052029 ) ) ;
#16053=CARTESIAN_POINT ( 'NONE',  ( 5.412658773652739619, 3.124999999999988898, -69.68301270189225249 ) ) ;
#16059=EDGE_CURVE ( 'NONE', #12915, #3959, #23753, .T. ) ;
#16063=CARTESIAN_POINT ( 'NONE',  ( -4.763139720814407951, 2.749999999999946709, -122.7500000000000284 ) ) ;
#16064=CARTESIAN_POINT ( 'NONE',  ( 2.775557561562891351E-14, -6.250000000000061284, -143.6830127018922099 ) ) ;
#16065=CARTESIAN_POINT ( 'NONE',  ( -5.999999999999963585, 1.780251999655701777E-13, -112.4136751345948255 ) ) ;
#16066=ORIENTED_EDGE ( 'NONE', *, *, #23620, .F. ) ;
#16067=CARTESIAN_POINT ( 'NONE',  ( -3.175426480542816066, -5.500000000000057732, -51.87500000000002132 ) ) ;
#16068=DIRECTION ( 'NONE',  ( 1.000000000000000000, -5.551115123125774074E-17, -1.260129944081490338E-35 ) ) ;
#16070=CARTESIAN_POINT ( 'NONE',  ( -5.999999999999919176, 1.607695154586804565, -69.90331216351299304 ) ) ;
#16072=ORIENTED_EDGE ( 'NONE', *, *, #22885, .F. ) ;
#16075=CARTESIAN_POINT ( 'NONE',  ( -6.000000000000000888, 1.067854986875958443E-15, 7.560779664488942560E-35 ) ) ;
#16077=FACE_OUTER_BOUND ( 'NONE', #30222, .T. ) ;
#16078=CARTESIAN_POINT ( 'NONE',  ( 6.350852961086080661, -9.614813431917819062E-14, -138.3750000000000568 ) ) ;
#16079=( BOUNDED_CURVE ( )  B_SPLINE_CURVE ( 2, ( #24104, #7377, #606, #11725, #9540, #18933, #14482, #14189, #9992 ),
 .UNSPECIFIED., .F., .T. ) 
 B_SPLINE_CURVE_WITH_KNOTS ( ( 3, 2, 2, 2, 3 ),
 ( 0.4138888888888888618, 0.4148148148148148029, 0.4166666666666666852, 0.4185185185185185119, 0.4194444444444444531 ),
 .UNSPECIFIED. ) 
 CURVE ( )  GEOMETRIC_REPRESENTATION_ITEM ( )  RATIONAL_B_SPLINE_CURVE ( ( 0.9330127018922194093, 0.9330127018922174109, 1.000000000000000000, 0.8660254037844388186, 1.000000000000000000, 0.8660254037844388186, 1.000000000000000000, 0.9330127018922194093, 0.9330127018922194093 ) ) 
 REPRESENTATION_ITEM ( '' )  );
#16082=CARTESIAN_POINT ( 'NONE',  ( -4.763139720814407951, -2.750000000000016431, -64.00000000000000000 ) ) ;
#16083=CARTESIAN_POINT ( 'NONE',  ( 0.000000000000000000, -5.999999999999991118, -164.5386751345948539 ) ) ;
#16086=AXIS2_PLACEMENT_3D ( 'NONE', #25880, #681, #28767 ) ;
#16087=CARTESIAN_POINT ( 'NONE',  ( -5.999999999999963585, -1.487416814333745711E-14, -113.9136751345948255 ) ) ;
#16088=ADVANCED_FACE ( 'NONE', ( #27386 ), #23121, .T. ) ;
#16091=CARTESIAN_POINT ( 'NONE',  ( 3.175426480543072749, -5.500000000000105693, -146.1250000000000284 ) ) ;
#16093=CARTESIAN_POINT ( 'NONE',  ( -5.412658773652684552, -3.125000000000099920, -158.9330127018922383 ) ) ;
#16096=CARTESIAN_POINT ( 'NONE',  ( -3.175426480542816066, 5.499999999999865885, -76.37500000000001421 ) ) ;
#16099=EDGE_CURVE ( 'NONE', #21329, #11022, #776, .T. ) ;
#16100=CARTESIAN_POINT ( 'NONE',  ( -2.775557561562891351E-14, -5.500000000000115463, -72.75000000000004263 ) ) ;
#16101=EDGE_CURVE ( 'NONE', #27374, #27987, #16526, .T. ) ;
#16102=CARTESIAN_POINT ( 'NONE',  ( 3.464101615137852974, 5.999999999999884537, -154.9136751345947971 ) ) ;
#16110=CARTESIAN_POINT ( 'NONE',  ( 6.000000000000000888, -1.859271017917181981E-14, -116.1636751345948255 ) ) ;
#16111=ORIENTED_EDGE ( 'NONE', *, *, #25462, .F. ) ;
#16114=CARTESIAN_POINT ( 'NONE',  ( -5.999999999999962697, 3.323446944526963260E-14, -156.8363248654052313 ) ) ;
#16117=VERTEX_POINT ( 'NONE', #13618 ) ;
#16118=CARTESIAN_POINT ( 'NONE',  ( -3.175426480542816510, -5.500000000000057732, -92.37500000000002842 ) ) ;
#16119=CARTESIAN_POINT ( 'NONE',  ( 5.412658773652712085, -3.125000000000086153, -107.4330127018922667 ) ) ;
#16120=VERTEX_POINT ( 'NONE', #18373 ) ;
#16121=FACE_BOUND ( 'NONE', #23105, .T. ) ;
#16123=ADVANCED_FACE ( 'NONE', ( #20660 ), #30008, .T. ) ;
#16124=CARTESIAN_POINT ( 'NONE',  ( 0.8024951133112347978, -10.97768020916284648, -30.95935331155644477 ) ) ;
#16125=ORIENTED_EDGE ( 'NONE', *, *, #28205, .F. ) ;
#16126=CYLINDRICAL_SURFACE ( 'NONE', #10314, 6.000000000000000888 ) ;
#16127=CARTESIAN_POINT ( 'NONE',  ( 0.000000000000000000, 5.499999999999991118, -172.5000000000000000 ) ) ;
#16129=CARTESIAN_POINT ( 'NONE',  ( 4.763139720814407951, -2.749999999999988454, -159.5000000000000284 ) ) ;
#16132=CARTESIAN_POINT ( 'NONE',  ( 0.000000000000000000, 0.000000000000000000, -200.0000000000000000 ) ) ;
#16133=EDGE_CURVE ( 'NONE', #29507, #10931, #20768, .T. ) ;
#16134=CARTESIAN_POINT ( 'NONE',  ( -3.175426480542816510, 5.499999999999865885, -100.3750000000000000 ) ) ;
#16137=VECTOR ( 'NONE', #14068, 1000.000000000000000 ) ;
#16138=ORIENTED_EDGE ( 'NONE', *, *, #14701, .F. ) ;
#16144=AXIS2_PLACEMENT_3D ( 'NONE', #19819, #8284, #24730 ) ;
#16145=ORIENTED_EDGE ( 'NONE', *, *, #19257, .T. ) ;
#16146=CARTESIAN_POINT ( 'NONE',  ( 2.775557561562891351E-14, 6.250000000000033751, -86.56698729810786119 ) ) ;
#16148=CARTESIAN_POINT ( 'NONE',  ( -3.464101615137757051, -5.999999999999979572, -65.66367513459478289 ) ) ;
#16152=CARTESIAN_POINT ( 'NONE',  ( -6.350852961085760029, -1.281975124255709124E-13, -124.1250000000000568 ) ) ;
#16154=CARTESIAN_POINT ( 'NONE',  ( -3.608439182435115633, 6.249999999999965361, -133.8080127018922951 ) ) ;
#16155=ORIENTED_EDGE ( 'NONE', *, *, #22745, .F. ) ;
#16157=CARTESIAN_POINT ( 'NONE',  ( 3.608439182435180470, 6.249999999999982236, -166.1919872981078186 ) ) ;
#16158=CARTESIAN_POINT ( 'NONE',  ( 3.608439182435180470, 6.249999999999982236, -176.6919872981077901 ) ) ;
#16160=FACE_OUTER_BOUND ( 'NONE', #4306, .T. ) ;
#16162=ORIENTED_EDGE ( 'NONE', *, *, #2463, .T. ) ;
#16164=CARTESIAN_POINT ( 'NONE',  ( 0.000000000000000000, 5.999999999999977796, -54.28867513459484684 ) ) ;
#16165=( BOUNDED_CURVE ( )  B_SPLINE_CURVE ( 2, ( #1146, #995, #15484, #10396, #8529, #29245, #1615, #11017, #24653 ),
 .UNSPECIFIED., .F., .T. ) 
 B_SPLINE_CURVE_WITH_KNOTS ( ( 3, 2, 2, 2, 3 ),
 ( 0.4583333333333332593, 0.4592592592592592560, 0.4611111111111111382, 0.4629629629629629095, 0.4638888888888889062 ),
 .UNSPECIFIED. ) 
 CURVE ( )  GEOMETRIC_REPRESENTATION_ITEM ( )  RATIONAL_B_SPLINE_CURVE ( ( 0.9330127018922194093, 0.9330127018922154125, 1.000000000000000000, 0.8660254037844388186, 1.000000000000000000, 0.8660254037844388186, 1.000000000000000000, 0.9330127018922154125, 0.9330127018922194093 ) ) 
 REPRESENTATION_ITEM ( '' )  );
#16167=CARTESIAN_POINT ( 'NONE',  ( 6.000000000000000888, 1.743066579297358182E-13, -96.08632486540521711 ) ) ;
#16168=CARTESIAN_POINT ( 'NONE',  ( -5.196152422706601826, 2.999999999999975131, -136.5386751345948255 ) ) ;
#16171=CARTESIAN_POINT ( 'NONE',  ( 3.608439182435180470, 6.249999999999982236, -73.19198729810781856 ) ) ;
#16172=CARTESIAN_POINT ( 'NONE',  ( 3.608439182435180470, 6.249999999999982236, -61.19198729810783277 ) ) ;
#16173=CARTESIAN_POINT ( 'NONE',  ( 0.000000000000000000, 5.499999999999991118, -49.49999999999998579 ) ) ;
#16174=CARTESIAN_POINT ( 'NONE',  ( -5.196152422706573404, -3.000000000000002665, -111.7113248654052455 ) ) ;
#16175=CARTESIAN_POINT ( 'NONE',  ( -5.196152422706573404, -3.000000000000002665, -123.7113248654052597 ) ) ;
#16176=CARTESIAN_POINT ( 'NONE',  ( 4.763139720814407951, 2.750000000000002665, -118.7500000000000284 ) ) ;
#16177=( BOUNDED_CURVE ( )  B_SPLINE_CURVE ( 2, ( #30028, #1765, #15798, #22108, #15048, #8998, #6684, #24238, #21955 ),
 .UNSPECIFIED., .F., .T. ) 
 B_SPLINE_CURVE_WITH_KNOTS ( ( 3, 2, 2, 2, 3 ),
 ( 0.7805555555555555580, 0.7814814814814814437, 0.7833333333333333259, 0.7851851851851852082, 0.7861111111111112049 ),
 .UNSPECIFIED. ) 
 CURVE ( )  GEOMETRIC_REPRESENTATION_ITEM ( )  RATIONAL_B_SPLINE_CURVE ( ( 0.9330127018922194093, 0.9330127018922194093, 1.000000000000000000, 0.8660254037844388186, 1.000000000000000000, 0.8660254037844388186, 1.000000000000000000, 0.9330127018922154125, 0.9330127018922194093 ) ) 
 REPRESENTATION_ITEM ( '' )  );
#16179=CARTESIAN_POINT ( 'NONE',  ( -5.999999999999919176, 1.607695154586804565, -153.9033121635130215 ) ) ;
#16180=ORIENTED_EDGE ( 'NONE', *, *, #28478, .F. ) ;
#16183=CARTESIAN_POINT ( 'NONE',  ( 0.000000000000000000, 0.000000000000000000, -14.99152654425661702 ) ) ;
#16184=ORIENTED_EDGE ( 'NONE', *, *, #4463, .T. ) ;
#16187=CARTESIAN_POINT ( 'NONE',  ( 2.775557561562891351E-14, 6.250000000000033751, -107.5669872981078186 ) ) ;
#16190=VERTEX_POINT ( 'NONE', #29956 ) ;
#16192=CARTESIAN_POINT ( 'NONE',  ( -5.999999999999963585, 8.134310703387671600E-14, -142.4136751345948539 ) ) ;
#16195=CARTESIAN_POINT ( 'NONE',  ( -7.216878364870328078, 0.000000000000000000, -140.1919872981078186 ) ) ;
#16200=CARTESIAN_POINT ( 'NONE',  ( 5.196152422706629359, -2.999999999999988898, -137.2886751345948539 ) ) ;
#16201=CARTESIAN_POINT ( 'NONE',  ( 5.412658773652712085, -3.125000000000086153, -69.93301270189222407 ) ) ;
#16205=CARTESIAN_POINT ( 'NONE',  ( -5.999999999999963585, -1.487416814333745711E-14, -54.83632486540523132 ) ) ;
#16211=CARTESIAN_POINT ( 'NONE',  ( -2.775557561562891351E-14, -5.500000000000115463, -126.7500000000000284 ) ) ;
#16214=CARTESIAN_POINT ( 'NONE',  ( 6.000000000000000888, 7.762456499804234384E-14, -143.1636751345948255 ) ) ;
#16216=CARTESIAN_POINT ( 'NONE',  ( 6.350852961086080661, -9.614813431917819062E-14, -57.37500000000004974 ) ) ;
#16217=CARTESIAN_POINT ( 'NONE',  ( 5.196152422706629359, 3.000000000000002665, -124.4613248654052313 ) ) ;
#16218=CARTESIAN_POINT ( 'NONE',  ( 6.000000000000000888, 1.743066579297358182E-13, -52.58632486540518869 ) ) ;
#16219=CARTESIAN_POINT ( 'NONE',  ( 6.000000000000052403, -1.607695154586662678, -178.6533121635129362 ) ) ;
#16220=ORIENTED_EDGE ( 'NONE', *, *, #26811, .T. ) ;
#16224=CARTESIAN_POINT ( 'NONE',  ( 3.608439182435180470, 6.249999999999982236, -101.6919872981078328 ) ) ;
#16230=CARTESIAN_POINT ( 'NONE',  ( -3.175426480542816510, 5.499999999999865885, -134.8750000000000000 ) ) ;
#16232=ORIENTED_EDGE ( 'NONE', *, *, #27046, .T. ) ;
#16237=CARTESIAN_POINT ( 'NONE',  ( -2.775557561562891351E-14, -5.500000000000115463, -62.25000000000002842 ) ) ;
#16240=CARTESIAN_POINT ( 'NONE',  ( -3.464101615137757051, -5.999999999999979572, -83.66367513459481131 ) ) ;
#16243=CARTESIAN_POINT ( 'NONE',  ( -4.763139720814407951, -2.750000000000016431, -151.0000000000000284 ) ) ;
#16245=CARTESIAN_POINT ( 'NONE',  ( -4.763139720814407951, 2.749999999999946709, -136.2499999999999716 ) ) ;
#16246=CARTESIAN_POINT ( 'NONE',  ( 2.775557561562891351E-14, -6.250000000000061284, -164.6830127018922383 ) ) ;
#16247=FILL_AREA_STYLE ('',( #7288 ) ) ;
#16249=CARTESIAN_POINT ( 'NONE',  ( -3.175426480542816066, -5.500000000000057732, -80.37500000000002842 ) ) ;
#16251=CARTESIAN_POINT ( 'NONE',  ( -4.763139720814407951, -2.750000000000016431, -71.50000000000001421 ) ) ;
#16252=CARTESIAN_POINT ( 'NONE',  ( -3.464101615137725076, 5.999999999999979572, -154.6636751345947971 ) ) ;
#16254=DIRECTION ( 'NONE',  ( -7.147005652999508048E-36, 5.642372883946980038E-36, 1.000000000000000000 ) ) ;
#16257=CARTESIAN_POINT ( 'NONE',  ( 5.999999999999974243, 1.607695154586759934, -134.0966878364870638 ) ) ;
#16258=CARTESIAN_POINT ( 'NONE',  ( 6.000000000000000888, 1.743066579297358182E-13, -95.16367513459482552 ) ) ;
#16259=CARTESIAN_POINT ( 'NONE',  ( -5.999999999999904965, -1.607695154586834541, -147.7693375672974128 ) ) ;
#16261=CARTESIAN_POINT ( 'NONE',  ( -3.464101615137725076, 5.999999999999979572, -169.6636751345948255 ) ) ;
#16262=( BOUNDED_CURVE ( )  B_SPLINE_CURVE ( 2, ( #11453, #20797, #25066, #9258, #13756, #18653, #18803, #4638, #25371 ),
 .UNSPECIFIED., .F., .F. ) 
 B_SPLINE_CURVE_WITH_KNOTS ( ( 3, 2, 2, 2, 3 ),
 ( 0.8027777777777778123, 0.8037037037037036979, 0.8055555555555555802, 0.8074074074074073515, 0.8083333333333333481 ),
 .UNSPECIFIED. ) 
 CURVE ( )  GEOMETRIC_REPRESENTATION_ITEM ( )  RATIONAL_B_SPLINE_CURVE ( ( 0.9330127018922194093, 0.9330127018922234061, 1.000000000000000000, 0.8660254037844388186, 1.000000000000000000, 0.8660254037844388186, 1.000000000000000000, 0.9330127018922154125, 0.9330127018922194093 ) ) 
 REPRESENTATION_ITEM ( '' )  );
#16268=CARTESIAN_POINT ( 'NONE',  ( 5.196152422706629359, -2.999999999999988898, -84.78867513459481131 ) ) ;
#16269=ORIENTED_EDGE ( 'NONE', *, *, #21884, .T. ) ;
#16271=VERTEX_POINT ( 'NONE', #1705 ) ;
#16272=CARTESIAN_POINT ( 'NONE',  ( -3.175426480542816510, 5.499999999999865885, -92.87500000000002842 ) ) ;
#16275=CARTESIAN_POINT ( 'NONE',  ( -3.608439182435115633, 6.249999999999965361, -105.3080127018922525 ) ) ;
#16276=ORIENTED_EDGE ( 'NONE', *, *, #8288, .T. ) ;
#16278=CARTESIAN_POINT ( 'NONE',  ( 5.799430203125144345, 9.347489878302534194, -23.41021253818531989 ) ) ;
#16280=VERTEX_POINT ( 'NONE', #28100 ) ;
#16283=AXIS2_PLACEMENT_3D ( 'NONE', #21092, #6323, #471 ) ;
#16284=CARTESIAN_POINT ( 'NONE',  ( 3.175426480543072749, -5.500000000000105693, -168.6250000000000000 ) ) ;
#16285=CARTESIAN_POINT ( 'NONE',  ( -5.999999999999956479, -1.607695154586745057, -80.84668783648706381 ) ) ;
#16286=CARTESIAN_POINT ( 'NONE',  ( 4.763139720814407951, 2.750000000000002665, -160.7500000000000568 ) ) ;
#16287=CARTESIAN_POINT ( 'NONE',  ( 4.763139720814407951, -2.749999999999988454, -101.0000000000000284 ) ) ;
#16289=CARTESIAN_POINT ( 'NONE',  ( 6.000000000000000888, 5.577813053751546416E-15, -165.6636751345948255 ) ) ;
#16290=CARTESIAN_POINT ( 'NONE',  ( 4.763139720814407951, 2.750000000000002665, -99.25000000000000000 ) ) ;
#16296=FACE_OUTER_BOUND ( 'NONE', #22377, .T. ) ;
#16301=CARTESIAN_POINT ( 'NONE',  ( 5.196152422706629359, 3.000000000000002665, -112.4613248654052171 ) ) ;
#16302=AXIS2_PLACEMENT_3D ( 'NONE', #2431, #11843, #7031 ) ;
#16304=ORIENTED_EDGE ( 'NONE', *, *, #11215, .F. ) ;
#16305=CARTESIAN_POINT ( 'NONE',  ( 0.000000000000000000, -5.999999999999991118, -52.96132486540522422 ) ) ;
#16308=VERTEX_POINT ( 'NONE', #30415 ) ;
#16309=( BOUNDED_CURVE ( )  B_SPLINE_CURVE ( 2, ( #11621, #27992, #30316, #27417, #6963, #8550, #9276, #18672, #22694 ),
 .UNSPECIFIED., .F., .F. ) 
 B_SPLINE_CURVE_WITH_KNOTS ( ( 3, 2, 2, 2, 3 ),
 ( 0.4249999999999999889, 0.4259259259259259300, 0.4277777777777777568, 0.4296296296296296391, 0.4305555555555555802 ),
 .UNSPECIFIED. ) 
 CURVE ( )  GEOMETRIC_REPRESENTATION_ITEM ( )  RATIONAL_B_SPLINE_CURVE ( ( 0.9330127018922194093, 0.9330127018922194093, 1.000000000000000000, 0.8660254037844388186, 1.000000000000000000, 0.8660254037844388186, 1.000000000000000000, 0.9330127018922174109, 0.9330127018922194093 ) ) 
 REPRESENTATION_ITEM ( '' )  );
#16310=CARTESIAN_POINT ( 'NONE',  ( 0.000000000000000000, 5.499999999999991118, -110.9999999999999858 ) ) ;
#16312=CARTESIAN_POINT ( 'NONE',  ( -5.412658773652739619, 3.124999999999975131, -135.1830127018922667 ) ) ;
#16313=ORIENTED_EDGE ( 'NONE', *, *, #17599, .F. ) ;
#16314=CARTESIAN_POINT ( 'NONE',  ( -3.608439182435052128, -6.250000000000110134, -165.4419872981077901 ) ) ;
#16315=CARTESIAN_POINT ( 'NONE',  ( -7.216878364870328078, 0.000000000000000000, -180.6919872981078186 ) ) ;
#16317=EDGE_LOOP ( 'NONE', ( #4651, #27315, #12293, #13405 ) ) ;
#16318=CARTESIAN_POINT ( 'NONE',  ( 5.374111793520025770, 2.595803520882615789, -180.0000000000001705 ) ) ;
#16319=CARTESIAN_POINT ( 'NONE',  ( 0.000000000000000000, 0.000000000000000000, -43.99152654425658682 ) ) ;
#16320=AXIS2_PLACEMENT_3D ( 'NONE', #28988, #1043, #3638 ) ;
#16323=CARTESIAN_POINT ( 'NONE',  ( 2.775557561562891351E-14, 6.250000000000033751, -62.56698729810783277 ) ) ;
#16324=CARTESIAN_POINT ( 'NONE',  ( -5.412658773652684552, -3.125000000000099920, -175.4330127018922667 ) ) ;
#16326=CARTESIAN_POINT ( 'NONE',  ( 6.000000000000000888, -1.607695154586752384, -47.23066243270262277 ) ) ;
#16327=CARTESIAN_POINT ( 'NONE',  ( -6.350852961085760029, -1.281975124255709124E-13, -119.6250000000000142 ) ) ;
#16329=CARTESIAN_POINT ( 'NONE',  ( 5.196152422706629359, 3.000000000000002665, -154.4613248654052029 ) ) ;
#16332=CARTESIAN_POINT ( 'NONE',  ( -3.464101615137725076, 5.999999999999979572, -122.5863248654052313 ) ) ;
#16336=CARTESIAN_POINT ( 'NONE',  ( 3.464101615137852974, 5.999999999999884537, -121.9136751345948682 ) ) ;
#16337=CARTESIAN_POINT ( 'NONE',  ( 2.775557561562891351E-14, 6.250000000000033751, -110.5669872981078186 ) ) ;
#16338=AXIS2_PLACEMENT_3D ( 'NONE', #20784, #18948, #7246 ) ;
#16339=ADVANCED_FACE ( 'NONE', ( #21370 ), #9695, .T. ) ;
#16341=EDGE_CURVE ( 'NONE', #15144, #17475, #4907, .T. ) ;
#16348=CARTESIAN_POINT ( 'NONE',  ( -7.216878364870328078, 0.000000000000000000, -135.6919872981078754 ) ) ;
#16353=CARTESIAN_POINT ( 'NONE',  ( -7.216878364870328078, 0.000000000000000000, -58.55801270189222407 ) ) ;
#16356=CARTESIAN_POINT ( 'NONE',  ( 6.000000000000000888, 1.743066579297358182E-13, -69.66367513459481131 ) ) ;
#16360=CYLINDRICAL_SURFACE ( 'NONE', #16283, 6.000000000000000888 ) ;
#16363=VERTEX_POINT ( 'NONE', #16638 ) ;
#16364=CARTESIAN_POINT ( 'NONE',  ( 4.763139720814407951, -2.749999999999988454, -59.00000000000004974 ) ) ;
#16367=VERTEX_POINT ( 'NONE', #2612 ) ;
#16370=CARTESIAN_POINT ( 'NONE',  ( 5.412658773652712085, -3.125000000000086153, -100.5669872981078186 ) ) ;
#16372=EDGE_CURVE ( 'NONE', #28281, #3967, #2469, .T. ) ;
#16374=CARTESIAN_POINT ( 'NONE',  ( 6.000000000000000888, -3.330669073875464691E-16, -7.560779664488942560E-35 ) ) ;
#16376=CARTESIAN_POINT ( 'NONE',  ( -4.763139720814407951, -2.750000000000016431, -136.0000000000000000 ) ) ;
#16377=VECTOR ( 'NONE', #30133, 1000.000000000000000 ) ;
#16378=VERTEX_POINT ( 'NONE', #12029 ) ;
#16379=ORIENTED_EDGE ( 'NONE', *, *, #9538, .T. ) ;
#16380=CARTESIAN_POINT ( 'NONE',  ( 4.763139720814407951, 2.750000000000002665, -63.25000000000002842 ) ) ;
#16382=CARTESIAN_POINT ( 'NONE',  ( 5.999999999999949374, 1.607695154586804565, -94.51933756729744118 ) ) ;
#16384=VERTEX_POINT ( 'NONE', #4611 ) ;
#16389=CARTESIAN_POINT ( 'NONE',  ( 4.763139720814407951, 2.750000000000002665, -145.7500000000000568 ) ) ;
#16391=CARTESIAN_POINT ( 'NONE',  ( 3.175426480543072749, -5.500000000000105693, -140.1250000000000000 ) ) ;
#16392=CARTESIAN_POINT ( 'NONE',  ( -3.608439182435115633, 6.249999999999965361, -159.3080127018922667 ) ) ;
#16394=ADVANCED_FACE ( 'NONE', ( #23379 ), #2326, .T. ) ;
#16395=CARTESIAN_POINT ( 'NONE',  ( 4.763139720814407951, 2.750000000000002665, -79.74999999999998579 ) ) ;
#16396=CARTESIAN_POINT ( 'NONE',  ( 6.000000000000000888, 7.762456499804234384E-14, -140.1636751345948255 ) ) ;
#16398=CARTESIAN_POINT ( 'NONE',  ( -4.763139720814407951, -2.750000000000016431, -67.00000000000000000 ) ) ;
#16401=CYLINDRICAL_SURFACE ( 'NONE', #7349, 6.000000000000000888 ) ;
#16402=CARTESIAN_POINT ( 'NONE',  ( -5.999999999999964473, 9.063946212346262433E-15, -175.4136751345948824 ) ) ;
#16410=LINE ( 'NONE', #1770, #1240 ) ;
#16411=EDGE_CURVE ( 'NONE', #8626, #24992, #6559, .T. ) ;
#16412=VERTEX_POINT ( 'NONE', #13986 ) ;
#16416=CARTESIAN_POINT ( 'NONE',  ( 4.763139720814407951, -2.749999999999988454, -153.5000000000000284 ) ) ;
#16419=ORIENTED_EDGE ( 'NONE', *, *, #24910, .F. ) ;
#16421=CARTESIAN_POINT ( 'NONE',  ( -2.775557561562891351E-14, -5.500000000000115463, -92.25000000000000000 ) ) ;
#16422=CARTESIAN_POINT ( 'NONE',  ( -5.412658773652684552, -3.125000000000099920, -109.4330127018922099 ) ) ;
#16423=CARTESIAN_POINT ( 'NONE',  ( 1.595708107228637651, 10.89084870836962260, -30.79786109011546102 ) ) ;
#16425=CARTESIAN_POINT ( 'NONE',  ( 6.350852961086080661, -9.614813431917819062E-14, -166.8750000000000568 ) ) ;
#16426=CARTESIAN_POINT ( 'NONE',  ( 0.000000000000000000, -5.999999999999991118, -63.46132486540523132 ) ) ;
#16427=CARTESIAN_POINT ( 'NONE',  ( 6.000000000000000888, 1.607695154586715303, -47.09668783648704249 ) ) ;
#16428=CARTESIAN_POINT ( 'NONE',  ( -3.175426480542816066, -5.500000000000057732, -173.3750000000000284 ) ) ;
#16430=CARTESIAN_POINT ( 'NONE',  ( 6.350852961086080661, -9.614813431917819062E-14, -154.8750000000000000 ) ) ;
#16433=CARTESIAN_POINT ( 'NONE',  ( -3.175426480542816066, -5.500000000000057732, -101.3750000000000000 ) ) ;
#16435=DIRECTION ( 'NONE',  ( -7.147005652999508048E-36, 5.642372883946980038E-36, 1.000000000000000000 ) ) ;
#16436=CARTESIAN_POINT ( 'NONE',  ( -3.175426480542816510, -5.500000000000057732, -89.37500000000001421 ) ) ;
#16439=DIRECTION ( 'NONE',  ( -7.147005652999508048E-36, 5.642372883946980038E-36, 1.000000000000000000 ) ) ;
#16440=ORIENTED_EDGE ( 'NONE', *, *, #4500, .F. ) ;
#16443=CYLINDRICAL_SURFACE ( 'NONE', #17367, 6.000000000000000888 ) ;
#16445=EDGE_CURVE ( 'NONE', #4894, #11998, #6398, .T. ) ;
#16450=DIRECTION ( 'NONE',  ( 1.000000000000000000, -5.551115123125774074E-17, 0.000000000000000000 ) ) ;
#16452=CARTESIAN_POINT ( 'NONE',  ( -3.464101615137757051, -5.999999999999979572, -53.08632486540517448 ) ) ;
#16454=ORIENTED_EDGE ( 'NONE', *, *, #9919, .T. ) ;
#16455=CARTESIAN_POINT ( 'NONE',  ( -3.175426480542816510, 5.499999999999865885, -116.8750000000000142 ) ) ;
#16457=CARTESIAN_POINT ( 'NONE',  ( 5.412658773652712085, -3.125000000000086153, -132.9330127018922383 ) ) ;
#16458=ORIENTED_EDGE ( 'NONE', *, *, #4726, .F. ) ;
#16460=CARTESIAN_POINT ( 'NONE',  ( 2.775557561562891351E-14, -6.250000000000061284, -166.8169872981077901 ) ) ;
#16463=CARTESIAN_POINT ( 'NONE',  ( 4.293779821593954438, 3.976156217459086317, -180.0000000000000284 ) ) ;
#16464=CARTESIAN_POINT ( 'NONE',  ( 5.999999999999897859, 1.607695154586893826, -133.5193375672974128 ) ) ;
#16465=CARTESIAN_POINT ( 'NONE',  ( -4.763139720814407951, 2.749999999999946709, -179.7500000000000284 ) ) ;
#16467=CARTESIAN_POINT ( 'NONE',  ( 3.608439182435180470, 6.249999999999982236, -177.5580127018922667 ) ) ;
#16469=EDGE_CURVE ( 'NONE', #29957, #6341, #8027, .T. ) ;
#16470=CARTESIAN_POINT ( 'NONE',  ( -5.999999999999963585, 1.780251999655701777E-13, -104.9136751345948255 ) ) ;
#16472=CARTESIAN_POINT ( 'NONE',  ( 0.000000000000000000, 5.499999999999991118, -120.0000000000000000 ) ) ;
#16479=CARTESIAN_POINT ( 'NONE',  ( -5.999999999999963585, 8.134310703387671600E-14, -125.3363248654052171 ) ) ;
#16481=EDGE_CURVE ( 'NONE', #4074, #3881, #13323, .T. ) ;
#16482=VERTEX_POINT ( 'NONE', #18112 ) ;
#16485=CIRCLE ( 'NONE', #3678, 10.00000000000001421 ) ;
#16486=CARTESIAN_POINT ( 'NONE',  ( -7.216878364870328078, 0.000000000000000000, -108.6919872981078043 ) ) ;
#16487=( BOUNDED_CURVE ( )  B_SPLINE_CURVE ( 2, ( #10652, #26446, #12818, #27048, #14807, #14951, #24152, #17570, #3095 ),
 .UNSPECIFIED., .F., .F. ) 
 B_SPLINE_CURVE_WITH_KNOTS ( ( 3, 2, 2, 2, 3 ),
 ( 0.8805555555555555358, 0.8814814814814815325, 0.8833333333333333037, 0.8851851851851851860, 0.8861111111111111827 ),
 .UNSPECIFIED. ) 
 CURVE ( )  GEOMETRIC_REPRESENTATION_ITEM ( )  RATIONAL_B_SPLINE_CURVE ( ( 0.9330127018922194093, 0.9330127018922154125, 1.000000000000000000, 0.8660254037844388186, 1.000000000000000000, 0.8660254037844388186, 1.000000000000000000, 0.9330127018922154125, 0.9330127018922194093 ) ) 
 REPRESENTATION_ITEM ( '' )  );
#16488=CARTESIAN_POINT ( 'NONE',  ( -3.464101615137757051, -5.999999999999979572, -77.66367513459483973 ) ) ;
#16495=CARTESIAN_POINT ( 'NONE',  ( -3.608439182435115633, 6.249999999999965361, -141.9419872981078186 ) ) ;
#16501=CARTESIAN_POINT ( 'NONE',  ( 2.775557561562891351E-14, -6.250000000000061284, -58.18301270189224539 ) ) ;
#16504=DIRECTION ( 'NONE',  ( 1.000000000000000000, -5.551115123125773458E-17, -1.260129944081490338E-35 ) ) ;
#16510=EDGE_CURVE ( 'NONE', #9807, #6115, #22590, .T. ) ;
#16511=EDGE_CURVE ( 'NONE', #5195, #899, #3892, .T. ) ;
#16513=CARTESIAN_POINT ( 'NONE',  ( -5.196152422706601826, 2.999999999999975131, -112.5386751345948113 ) ) ;
#16515=CARTESIAN_POINT ( 'NONE',  ( -4.763139720814407951, -2.750000000000016431, -53.49999999999999289 ) ) ;
#16516=EDGE_CURVE ( 'NONE', #3077, #9966, #18722, .T. ) ;
#16517=CARTESIAN_POINT ( 'NONE',  ( 3.464101615137852974, 5.999999999999884537, -121.3363248654051603 ) ) ;
#16518=CARTESIAN_POINT ( 'NONE',  ( 6.000000000000000888, -1.607695154586752384, -151.6533121635129930 ) ) ;
#16520=AXIS2_PLACEMENT_3D ( 'NONE', #10272, #12304, #14459 ) ;
#16521=ORIENTED_EDGE ( 'NONE', *, *, #9891, .F. ) ;
#16524=CARTESIAN_POINT ( 'NONE',  ( 2.775557561562891351E-14, 6.250000000000033751, -103.0669872981078186 ) ) ;
#16525=CYLINDRICAL_SURFACE ( 'NONE', #16622, 6.000000000000000888 ) ;
#16526=( BOUNDED_CURVE ( )  B_SPLINE_CURVE ( 2, ( #1750, #11149, #6208, #15628, #1445, #1904, #24937, #15935, #4203 ),
 .UNSPECIFIED., .F., .T. ) 
 B_SPLINE_CURVE_WITH_KNOTS ( ( 3, 2, 2, 2, 3 ),
 ( 0.5527777777777778123, 0.5537037037037036979, 0.5555555555555555802, 0.5574074074074074625, 0.5583333333333333481 ),
 .UNSPECIFIED. ) 
 CURVE ( )  GEOMETRIC_REPRESENTATION_ITEM ( )  RATIONAL_B_SPLINE_CURVE ( ( 0.9330127018922194093, 0.9330127018922234061, 1.000000000000000000, 0.8660254037844388186, 1.000000000000000000, 0.8660254037844388186, 1.000000000000000000, 0.9330127018922194093, 0.9330127018922194093 ) ) 
 REPRESENTATION_ITEM ( '' )  );
#16529=CARTESIAN_POINT ( 'NONE',  ( 4.763139720814407951, -2.749999999999988454, -137.0000000000000000 ) ) ;
#16532=CARTESIAN_POINT ( 'NONE',  ( 0.000000000000000000, 5.499999999999991118, -64.50000000000000000 ) ) ;
#16533=CARTESIAN_POINT ( 'NONE',  ( 5.196152422706629359, -2.999999999999988898, -179.2886751345948539 ) ) ;
#16535=CARTESIAN_POINT ( 'NONE',  ( -5.412658773652739619, 3.124999999999975131, -84.18301270189220986 ) ) ;
#16539=CARTESIAN_POINT ( 'NONE',  ( -5.999999999999962697, 3.323446944526963891E-14, -160.4136751345948255 ) ) ;
#16541=DIRECTION ( 'NONE',  ( -7.147005652999508048E-36, 5.642372883946980038E-36, 1.000000000000000000 ) ) ;
#16545=CARTESIAN_POINT ( 'NONE',  ( -4.763139720814407951, 2.749999999999946709, -145.2500000000000000 ) ) ;
#16547=CARTESIAN_POINT ( 'NONE',  ( 3.608439182435180470, -6.249999999999997335, -161.5580127018921814 ) ) ;
#16548=CARTESIAN_POINT ( 'NONE',  ( 5.999999999999999112, 2.951592740943527306E-14, -148.5863248654052313 ) ) ;
#16549=CARTESIAN_POINT ( 'NONE',  ( 0.000000000000000000, 0.000000000000000000, -180.0000000000000568 ) ) ;
#16551=CARTESIAN_POINT ( 'NONE',  ( 6.350852961086080661, -9.614813431917819062E-14, -81.37500000000001421 ) ) ;
#16552=CARTESIAN_POINT ( 'NONE',  ( 6.000000000000000888, -1.859271017917181981E-14, -63.08632486540521711 ) ) ;
#16553=CARTESIAN_POINT ( 'NONE',  ( -4.763139720814407951, -2.750000000000016431, -64.00000000000000000 ) ) ;
#16560=EDGE_LOOP ( 'NONE', ( #25449, #11811, #19008, #26573 ) ) ;
#16562=LINE ( 'NONE', #24435, #26359 ) ;
#16565=CARTESIAN_POINT ( 'NONE',  ( -7.216878364870328078, 0.000000000000000000, -152.1919872981077901 ) ) ;
#16567=CARTESIAN_POINT ( 'NONE',  ( -4.763139720814407951, 2.749999999999946709, -88.25000000000005684 ) ) ;
#16568=CARTESIAN_POINT ( 'NONE',  ( 5.412658773652712085, -3.125000000000086153, -102.9330127018922525 ) ) ;
#16569=CARTESIAN_POINT ( 'NONE',  ( 3.677985992802582871, 10.37237449091584374, -20.24368265486284457 ) ) ;
#16571=CARTESIAN_POINT ( 'NONE',  ( -2.775557561562891351E-14, -5.500000000000115463, -167.2500000000000000 ) ) ;
#16573=CARTESIAN_POINT ( 'NONE',  ( 6.000000000000000888, -1.859271017917181981E-14, -93.66367513459481131 ) ) ;
#16575=VECTOR ( 'NONE', #22140, 1000.000000000000000 ) ;
#16578=CARTESIAN_POINT ( 'NONE',  ( -3.175426480542816066, -5.500000000000057732, -174.8750000000000284 ) ) ;
#16580=CARTESIAN_POINT ( 'NONE',  ( -3.175426480542816510, -5.500000000000057732, -152.3750000000000000 ) ) ;
#16583=CARTESIAN_POINT ( 'NONE',  ( 4.763139720814407951, 2.750000000000002665, -103.7500000000000142 ) ) ;
#16584=CARTESIAN_POINT ( 'NONE',  ( -3.464101615137725076, 5.999999999999979572, -59.58632486540520290 ) ) ;
#16585=CARTESIAN_POINT ( 'NONE',  ( 3.175426480543072749, -5.500000000000105693, -156.6250000000000000 ) ) ;
#16586=CARTESIAN_POINT ( 'NONE',  ( 4.763139720814407951, -2.749999999999988454, -92.00000000000002842 ) ) ;
#16588=CARTESIAN_POINT ( 'NONE',  ( 6.000000000000000888, -1.607695154586752384, -135.7306624327025872 ) ) ;
#16590=ORIENTED_EDGE ( 'NONE', *, *, #21028, .F. ) ;
#16592=CARTESIAN_POINT ( 'NONE',  ( -5.999999999999963585, -1.487416814333745711E-14, -66.83632486540523132 ) ) ;
#16594=CARTESIAN_POINT ( 'NONE',  ( 6.000000000000000888, 1.743066579297358182E-13, -85.58632486540523132 ) ) ;
#16599=CARTESIAN_POINT ( 'NONE',  ( -5.999999999999963585, 8.134310703387671600E-14, -141.8363248654052029 ) ) ;
#16602=EDGE_LOOP ( 'NONE', ( #12728, #10674, #27442, #29368 ) ) ;
#16604=CARTESIAN_POINT ( 'NONE',  ( -3.175426480542816510, 5.499999999999865885, -112.3750000000000426 ) ) ;
#16607=CARTESIAN_POINT ( 'NONE',  ( 2.775557561562891351E-14, 6.250000000000033751, -130.9330127018922383 ) ) ;
#16609=FACE_OUTER_BOUND ( 'NONE', #3615, .T. ) ;
#16610=CARTESIAN_POINT ( 'NONE',  ( 2.775557561562891351E-14, -6.250000000000061284, -169.8169872981077901 ) ) ;
#16612=AXIS2_PLACEMENT_3D ( 'NONE', #7946, #27135, #1913 ) ;
#16616=CARTESIAN_POINT ( 'NONE',  ( -6.350852961085760029, -1.281975124255709124E-13, -181.1249999999999716 ) ) ;
#16618=CARTESIAN_POINT ( 'NONE',  ( -5.412658773652739619, 3.124999999999975131, -174.1830127018922383 ) ) ;
#16621=AXIS2_PLACEMENT_3D ( 'NONE', #9281, #4047, #20818 ) ;
#16622=AXIS2_PLACEMENT_3D ( 'NONE', #23109, #20804, #28137 ) ;
#16623=CARTESIAN_POINT ( 'NONE',  ( -3.464101615137757051, -5.999999999999979572, -53.66367513459480421 ) ) ;
#16624=CARTESIAN_POINT ( 'NONE',  ( -3.175426480542816510, 5.499999999999865885, -110.8750000000000426 ) ) ;
#16625=CARTESIAN_POINT ( 'NONE',  ( 3.464101615137852974, 5.999999999999884537, -166.3363248654052029 ) ) ;
#16626=CARTESIAN_POINT ( 'NONE',  ( 0.000000000000000000, 5.999999999999977796, -145.7886751345948255 ) ) ;
#16627=ORIENTED_EDGE ( 'NONE', *, *, #15131, .T. ) ;
#16629=CARTESIAN_POINT ( 'NONE',  ( 0.000000000000000000, 0.000000000000000000, -44.99152654425658682 ) ) ;
#16632=EDGE_LOOP ( 'NONE', ( #9536, #4232, #1845, #4276 ) ) ;
#16635=CARTESIAN_POINT ( 'NONE',  ( 3.175426480543072749, 5.499999999999865885, -178.6250000000000284 ) ) ;
#16637=DIRECTION ( 'NONE',  ( -7.147005652999508048E-36, 5.642372883946980038E-36, 1.000000000000000000 ) ) ;
#16638=CARTESIAN_POINT ( 'NONE',  ( 6.000000000000000000, 2.951592740943527306E-14, -163.5863248654052313 ) ) ;
#16639=ORIENTED_EDGE ( 'NONE', *, *, #27824, .T. ) ;
#16640=EDGE_LOOP ( 'NONE', ( #6606, #2586 ) ) ;
#16641=CARTESIAN_POINT ( 'NONE',  ( -3.464101615137757051, -5.999999999999979572, -142.1636751345948255 ) ) ;
#16644=CARTESIAN_POINT ( 'NONE',  ( -5.412658773652739619, 3.124999999999975131, -141.8169872981078186 ) ) ;
#16647=DIRECTION ( 'NONE',  ( -7.147005652999508048E-36, 5.642372883946980038E-36, 1.000000000000000000 ) ) ;
#16648=CARTESIAN_POINT ( 'NONE',  ( 0.000000000000000000, 0.000000000000000000, 0.000000000000000000 ) ) ;
#16654=CARTESIAN_POINT ( 'NONE',  ( 5.196152422706629359, 3.000000000000002665, -74.03867513459483973 ) ) ;
#16657=CARTESIAN_POINT ( 'NONE',  ( 6.000000000000000888, 1.607695154586715303, -114.0193375672974412 ) ) ;
#16660=CARTESIAN_POINT ( 'NONE',  ( 6.000000000000000888, 1.743066579297358182E-13, -113.1636751345948397 ) ) ;
#16662=( BOUNDED_CURVE ( )  B_SPLINE_CURVE ( 2, ( #19893, #26934, #24334, #29237, #23907, #2850, #12269, #545, #19311 ),
 .UNSPECIFIED., .F., .F. ) 
 B_SPLINE_CURVE_WITH_KNOTS ( ( 3, 2, 2, 2, 3 ),
 ( 0.7750000000000000222, 0.7759259259259259078, 0.7777777777777777901, 0.7796296296296296724, 0.7805555555555555580 ),
 .UNSPECIFIED. ) 
 CURVE ( )  GEOMETRIC_REPRESENTATION_ITEM ( )  RATIONAL_B_SPLINE_CURVE ( ( 0.9330127018922194093, 0.9330127018922234061, 1.000000000000000000, 0.8660254037844388186, 1.000000000000000000, 0.8660254037844388186, 1.000000000000000000, 0.9330127018922194093, 0.9330127018922194093 ) ) 
 REPRESENTATION_ITEM ( '' )  );
#16663=CARTESIAN_POINT ( 'NONE',  ( 3.175426480543072749, -5.500000000000105693, -50.12500000000001421 ) ) ;
#16664=CARTESIAN_POINT ( 'NONE',  ( 5.999999999999949374, 1.607695154586804565, -53.09668783648702117 ) ) ;
#16665=CARTESIAN_POINT ( 'NONE',  ( 6.000000000000000888, -1.859271017917181981E-14, -63.08632486540521711 ) ) ;
#16666=CARTESIAN_POINT ( 'NONE',  ( -5.999999999999956479, -1.607695154586745057, -152.2693375672974412 ) ) ;
#16667=ORIENTED_EDGE ( 'NONE', *, *, #13799, .F. ) ;
#16670=CARTESIAN_POINT ( 'NONE',  ( -5.412658773652739619, 3.124999999999975131, -105.8169872981078470 ) ) ;
#16675=CARTESIAN_POINT ( 'NONE',  ( -2.775557561562891351E-14, -5.500000000000115463, -129.7500000000000284 ) ) ;
#16677=VERTEX_POINT ( 'NONE', #7169 ) ;
#16678=CARTESIAN_POINT ( 'NONE',  ( -3.175426480542816510, 5.499999999999865885, -62.87500000000001421 ) ) ;
#16680=CARTESIAN_POINT ( 'NONE',  ( -5.999999999999959144, -1.607695154586737951, -179.8466878364870354 ) ) ;
#16682=EDGE_CURVE ( 'NONE', #4758, #23459, #26347, .T. ) ;
#16683=CARTESIAN_POINT ( 'NONE',  ( 2.775557561562891351E-14, 6.250000000000033751, -85.93301270189223828 ) ) ;
#16686=CARTESIAN_POINT ( 'NONE',  ( -5.999999999999956479, -1.607695154586745057, -176.2693375672974412 ) ) ;
#16688=CARTESIAN_POINT ( 'NONE',  ( 3.175426480543072749, 5.499999999999865885, -141.1250000000000000 ) ) ;
#16690=CARTESIAN_POINT ( 'NONE',  ( 2.775557561562891351E-14, 6.250000000000033751, -153.4330127018922383 ) ) ;
#16692=CARTESIAN_POINT ( 'NONE',  ( -5.196152422706573404, -3.000000000000002665, -73.28867513459481131 ) ) ;
#16693=CARTESIAN_POINT ( 'NONE',  ( -3.175426480542816066, 5.499999999999865885, -77.87500000000001421 ) ) ;
#16695=CARTESIAN_POINT ( 'NONE',  ( -4.763139720814407951, 2.749999999999946709, -68.75000000000002842 ) ) ;
#16696=( BOUNDED_CURVE ( )  B_SPLINE_CURVE ( 2, ( #15670, #29600, #3627, #15192, #8721, #1334, #6395, #8405, #22243 ),
 .UNSPECIFIED., .F., .T. ) 
 B_SPLINE_CURVE_WITH_KNOTS ( ( 3, 2, 2, 2, 3 ),
 ( 0.8249999999999999556, 0.8259259259259259522, 0.8277777777777777235, 0.8296296296296296058, 0.8305555555555556024 ),
 .UNSPECIFIED. ) 
 CURVE ( )  GEOMETRIC_REPRESENTATION_ITEM ( )  RATIONAL_B_SPLINE_CURVE ( ( 0.9330127018922194093, 0.9330127018922154125, 1.000000000000000000, 0.8660254037844388186, 1.000000000000000000, 0.8660254037844388186, 1.000000000000000000, 0.9330127018922154125, 0.9330127018922194093 ) ) 
 REPRESENTATION_ITEM ( '' )  );
#16700=CARTESIAN_POINT ( 'NONE',  ( 0.000000000000000000, 5.999999999999977796, -127.2113248654052029 ) ) ;
#16703=CARTESIAN_POINT ( 'NONE',  ( -6.000000000000000888, 1.067854986875958443E-15, 7.560779664488942560E-35 ) ) ;
#16705=VERTEX_POINT ( 'NONE', #21762 ) ;
#16706=AXIS2_PLACEMENT_3D ( 'NONE', #25103, #24808, #3903 ) ;
#16711=EDGE_CURVE ( 'NONE', #14122, #14750, #10210, .T. ) ;
#16713=CARTESIAN_POINT ( 'NONE',  ( 2.775557561562891351E-14, -6.250000000000061284, -156.3169872981078470 ) ) ;
#16715=CARTESIAN_POINT ( 'NONE',  ( 0.000000000000000000, 5.499999999999991118, -88.50000000000002842 ) ) ;
#16716=CARTESIAN_POINT ( 'NONE',  ( 2.775557561562891351E-14, 6.250000000000033751, -102.4330127018922525 ) ) ;
#16718=DIRECTION ( 'NONE',  ( 1.000000000000000000, -5.551115123125774074E-17, -1.260129944081490338E-35 ) ) ;
#16720=CARTESIAN_POINT ( 'NONE',  ( -6.350852961085760029, -1.281975124255709124E-13, -167.6249999999999716 ) ) ;
#16722=CARTESIAN_POINT ( 'NONE',  ( 0.000000000000000000, 5.999999999999977796, -58.78867513459484684 ) ) ;
#16726=CARTESIAN_POINT ( 'NONE',  ( 4.763139720814407951, -2.749999999999988454, -171.5000000000000000 ) ) ;
#16727=CARTESIAN_POINT ( 'NONE',  ( -6.000000000000007105, -1.607695154586655129, -60.76933756729742697 ) ) ;
#16728=CARTESIAN_POINT ( 'NONE',  ( -2.775557561562891351E-14, -5.500000000000115463, -153.7500000000000568 ) ) ;
#16730=CARTESIAN_POINT ( 'NONE',  ( 6.350852961086080661, -9.614813431917819062E-14, -102.3750000000000142 ) ) ;
#16732=CARTESIAN_POINT ( 'NONE',  ( 4.763139720814407951, -2.749999999999988454, -87.50000000000002842 ) ) ;
#16735=VERTEX_POINT ( 'NONE', #14432 ) ;
#16740=CARTESIAN_POINT ( 'NONE',  ( -5.999999999999963585, 1.780251999655701777E-13, -112.4136751345948255 ) ) ;
#16742=DIRECTION ( 'NONE',  ( -7.147005652999508048E-36, 5.642372883946980038E-36, 1.000000000000000000 ) ) ;
#16746=EDGE_LOOP ( 'NONE', ( #21669, #30163 ) ) ;
#16749=CARTESIAN_POINT ( 'NONE',  ( 4.763139720814407951, 2.750000000000002665, -115.7500000000000142 ) ) ;
#16751=CARTESIAN_POINT ( 'NONE',  ( -5.412658773652739619, 3.124999999999975131, -120.1830127018922383 ) ) ;
#16753=EDGE_LOOP ( 'NONE', ( #22698, #29695, #18924, #26224 ) ) ;
#16754=CARTESIAN_POINT ( 'NONE',  ( 3.175426480543072749, -5.500000000000105693, -152.1250000000000568 ) ) ;
#16756=CARTESIAN_POINT ( 'NONE',  ( -5.412658773652684552, -3.125000000000099920, -162.5669872981078186 ) ) ;
#16758=VERTEX_POINT ( 'NONE', #20219 ) ;
#16760=FACE_OUTER_BOUND ( 'NONE', #18365, .T. ) ;
#16762=CARTESIAN_POINT ( 'NONE',  ( 6.350852961086080661, -9.614813431917819062E-14, -175.8750000000000284 ) ) ;
#16764=CARTESIAN_POINT ( 'NONE',  ( 3.608439182435180470, -6.249999999999997335, -176.5580127018922667 ) ) ;
#16767=AXIS2_PLACEMENT_3D ( 'NONE', #24908, #11116, #19850 ) ;
#16768=CARTESIAN_POINT ( 'NONE',  ( 3.175426480543072749, 5.499999999999865885, -127.6249999999999858 ) ) ;
#16769=DIRECTION ( 'NONE',  ( -7.147005652999508048E-36, 5.642372883946980038E-36, 1.000000000000000000 ) ) ;
#16771=CARTESIAN_POINT ( 'NONE',  ( 6.350852961086080661, -9.614813431917819062E-14, -114.3750000000000000 ) ) ;
#16772=AXIS2_PLACEMENT_3D ( 'NONE', #11727, #21221, #21071 ) ;
#16773=CARTESIAN_POINT ( 'NONE',  ( -5.999999999999963585, 1.780251999655701777E-13, -100.4136751345948255 ) ) ;
#16774=ORIENTED_EDGE ( 'NONE', *, *, #4182, .F. ) ;
#16777=CARTESIAN_POINT ( 'NONE',  ( -6.000000000000000888, 1.067854986875958443E-15, 7.560779664488942560E-35 ) ) ;
#16778=CARTESIAN_POINT ( 'NONE',  ( 5.196152422706629359, 3.000000000000002665, -86.96132486540520290 ) ) ;
#16779=CARTESIAN_POINT ( 'NONE',  ( 6.000000000000000888, -1.859271017917181981E-14, -126.0863248654052171 ) ) ;
#16780=AXIS2_PLACEMENT_3D ( 'NONE', #29200, #17892, #22631 ) ;
#16781=CARTESIAN_POINT ( 'NONE',  ( -2.775557561562891351E-14, -5.500000000000115463, -179.2500000000000284 ) ) ;
#16785=EDGE_CURVE ( 'NONE', #25773, #12739, #19617, .T. ) ;
#16786=ORIENTED_EDGE ( 'NONE', *, *, #24703, .T. ) ;
#16788=CARTESIAN_POINT ( 'NONE',  ( 6.000000000000000888, -1.859271017917181981E-14, -141.6636751345948255 ) ) ;
#16792=CARTESIAN_POINT ( 'NONE',  ( 5.412658773652739619, 3.124999999999988898, -137.8169872981078186 ) ) ;
#16796=CARTESIAN_POINT ( 'NONE',  ( -5.999999999999919176, 1.607695154586804565, -174.9033121635129930 ) ) ;
#16797=CARTESIAN_POINT ( 'NONE',  ( 5.999999999999974243, 1.607695154586759934, -129.5966878364870354 ) ) ;
#16799=CARTESIAN_POINT ( 'NONE',  ( -5.999999999999963585, 8.134310703387671600E-14, -130.4136751345948539 ) ) ;
#16800=DIRECTION ( 'NONE',  ( -7.147005652999508048E-36, 5.642372883946980038E-36, 1.000000000000000000 ) ) ;
#16803=CARTESIAN_POINT ( 'NONE',  ( 0.000000000000000000, 5.999999999999977796, -99.28867513459482552 ) ) ;
#16804=CARTESIAN_POINT ( 'NONE',  ( -5.999999999999963585, 1.780251999655701777E-13, -108.8363248654052313 ) ) ;
#16811=CARTESIAN_POINT ( 'NONE',  ( -3.175426480542816066, -5.500000000000057732, -48.87500000000000000 ) ) ;
#16812=CARTESIAN_POINT ( 'NONE',  ( -5.999999999999919176, 1.607695154586804565, -52.48066243270259434 ) ) ;
#16813=ORIENTED_EDGE ( 'NONE', *, *, #7157, .F. ) ;
#16816=CARTESIAN_POINT ( 'NONE',  ( -5.412658773652684552, -3.125000000000099920, -102.5669872981078186 ) ) ;
#16817=CARTESIAN_POINT ( 'NONE',  ( -5.196152422706601826, 2.999999999999975131, -176.4613248654052313 ) ) ;
#16821=VECTOR ( 'NONE', #15127, 1000.000000000000114 ) ;
#16822=CARTESIAN_POINT ( 'NONE',  ( 6.350852961086080661, -9.614813431917819062E-14, -130.8750000000000284 ) ) ;
#16825=CARTESIAN_POINT ( 'NONE',  ( -6.350852961085760029, -1.281975124255709124E-13, -55.12500000000003553 ) ) ;
#16826=CARTESIAN_POINT ( 'NONE',  ( 2.775557561562891351E-14, 5.874999999999977796, -46.71650635094615467 ) ) ;
#16828=CARTESIAN_POINT ( 'NONE',  ( 7.216878364870455975, -6.409875621278545621E-14, -86.30801270189222407 ) ) ;
#16830=CARTESIAN_POINT ( 'NONE',  ( -6.000000000000023093, 1.607695154586625819, -149.4033121635129362 ) ) ;
#16834=CARTESIAN_POINT ( 'NONE',  ( 0.000000000000000000, 5.499999999999991118, -138.0000000000000000 ) ) ;
#16835=CARTESIAN_POINT ( 'NONE',  ( -5.999999999999963585, -1.487416814333745711E-14, -105.8363248654052313 ) ) ;
#16836=CARTESIAN_POINT ( 'NONE',  ( 2.775557561562891351E-14, -6.250000000000061284, -154.1830127018922667 ) ) ;
#16837=CARTESIAN_POINT ( 'NONE',  ( 3.464101615137852974, 5.999999999999884537, -116.8363248654052171 ) ) ;
#16838=CARTESIAN_POINT ( 'NONE',  ( 0.000000000000000000, 5.999999999999977796, -51.28867513459483973 ) ) ;
#16839=ADVANCED_FACE ( 'NONE', ( #10710 ), #12567, .T. ) ;
#16840=CARTESIAN_POINT ( 'NONE',  ( -6.350852961085760029, -1.281975124255709124E-13, -74.62500000000000000 ) ) ;
#16841=CARTESIAN_POINT ( 'NONE',  ( -3.175426480542816510, -5.500000000000057732, -68.37500000000002842 ) ) ;
#16847=EDGE_CURVE ( 'NONE', #9068, #9271, #844, .T. ) ;
#16848=FACE_OUTER_BOUND ( 'NONE', #3051, .T. ) ;
#16849=ORIENTED_EDGE ( 'NONE', *, *, #24974, .F. ) ;
#16854=CARTESIAN_POINT ( 'NONE',  ( 5.196152422706629359, 3.000000000000002665, -64.46132486540523132 ) ) ;
#16856=CARTESIAN_POINT ( 'NONE',  ( 3.175426480543072749, 5.499999999999865885, -178.6250000000000284 ) ) ;
#16859=CARTESIAN_POINT ( 'NONE',  ( -3.608439182435052128, -6.250000000000110134, -154.9419872981078470 ) ) ;
#16860=VERTEX_POINT ( 'NONE', #10542 ) ;
#16861=CARTESIAN_POINT ( 'NONE',  ( 4.763139720814407951, 2.750000000000002665, -84.25000000000004263 ) ) ;
#16862=ORIENTED_EDGE ( 'NONE', *, *, #22328, .T. ) ;
#16865=CARTESIAN_POINT ( 'NONE',  ( 0.4007817556720155161, -11.00000000000000355, -19.00000000000000355 ) ) ;
#16868=( BOUNDED_CURVE ( )  B_SPLINE_CURVE ( 2, ( #4287, #14168, #21047, #141, #23506, #25935, #4742, #9362, #16167 ),
 .UNSPECIFIED., .F., .T. ) 
 B_SPLINE_CURVE_WITH_KNOTS ( ( 3, 2, 2, 2, 3 ),
 ( 0.3638888888888889284, 0.3648148148148148140, 0.3666666666666666963, 0.3685185185185184675, 0.3694444444444443532 ),
 .UNSPECIFIED. ) 
 CURVE ( )  GEOMETRIC_REPRESENTATION_ITEM ( )  RATIONAL_B_SPLINE_CURVE ( ( 0.9330127018922194093, 0.9330127018922234061, 1.000000000000000000, 0.8660254037844388186, 1.000000000000000000, 0.8660254037844388186, 1.000000000000000000, 0.9330127018922234061, 0.9330127018922194093 ) ) 
 REPRESENTATION_ITEM ( '' )  );
#16870=CARTESIAN_POINT ( 'NONE',  ( 0.000000000000000000, 5.499999999999991118, -168.0000000000000284 ) ) ;
#16872=CARTESIAN_POINT ( 'NONE',  ( 4.763139720814407951, 2.750000000000002665, -153.2500000000000000 ) ) ;
#16874=EDGE_CURVE ( 'NONE', #9617, #17636, #8203, .T. ) ;
#16875=CARTESIAN_POINT ( 'NONE',  ( 6.350852961086080661, -9.614813431917819062E-14, -93.37500000000001421 ) ) ;
#16878=CARTESIAN_POINT ( 'NONE',  ( -4.763139720814407951, 2.749999999999946709, -92.75000000000000000 ) ) ;
#16881=CARTESIAN_POINT ( 'NONE',  ( -6.000000000000007105, -1.607695154586655129, -72.76933756729744118 ) ) ;
#16882=DIRECTION ( 'NONE',  ( 1.000000000000000000, -5.551115123125773458E-17, -1.260129944081490338E-35 ) ) ;
#16888=CARTESIAN_POINT ( 'NONE',  ( 0.000000000000000000, 0.000000000000000000, 0.000000000000000000 ) ) ;
#16891=ORIENTED_EDGE ( 'NONE', *, *, #10297, .F. ) ;
#16893=CARTESIAN_POINT ( 'NONE',  ( -3.175426480542816510, -5.500000000000057732, -116.3750000000000142 ) ) ;
#16895=CARTESIAN_POINT ( 'NONE',  ( 3.608439182435180470, 6.249999999999982236, -126.5580127018922383 ) ) ;
#16897=CARTESIAN_POINT ( 'NONE',  ( 6.000000000000000888, -1.607695154586752384, -68.23066243270258724 ) ) ;
#16898=CARTESIAN_POINT ( 'NONE',  ( -3.608439182435052128, -6.250000000000110134, -157.9419872981077617 ) ) ;
#16903=CARTESIAN_POINT ( 'NONE',  ( -3.464101615137757051, -5.999999999999979572, -132.5863248654052313 ) ) ;
#16905=CARTESIAN_POINT ( 'NONE',  ( 0.000000000000000000, 5.499999999999991118, -175.5000000000000000 ) ) ;
#16908=CARTESIAN_POINT ( 'NONE',  ( -7.216878364870328078, 0.000000000000000000, -177.0580127018922667 ) ) ;
#16910=CARTESIAN_POINT ( 'NONE',  ( -3.175426480542816066, -5.500000000000057732, -122.3749999999999716 ) ) ;
#16913=CARTESIAN_POINT ( 'NONE',  ( -2.775557561562891351E-14, -5.500000000000115463, -110.2500000000000142 ) ) ;
#16914=DIRECTION ( 'NONE',  ( -7.147005652999508048E-36, 5.642372883946980038E-36, 1.000000000000000000 ) ) ;
#16920=CARTESIAN_POINT ( 'NONE',  ( -5.196152422706573404, -3.000000000000002665, -56.21132486540525264 ) ) ;
#16921=DIRECTION ( 'NONE',  ( -7.147005652999508048E-36, 5.642372883946980038E-36, 1.000000000000000000 ) ) ;
#16922=VERTEX_POINT ( 'NONE', #4525 ) ;
#16925=EDGE_LOOP ( 'NONE', ( #11531, #22567, #11511, #14947 ) ) ;
#16927=ORIENTED_EDGE ( 'NONE', *, *, #9538, .F. ) ;
#16928=ORIENTED_EDGE ( 'NONE', *, *, #18705, .F. ) ;
#16932=CARTESIAN_POINT ( 'NONE',  ( 3.608439182435180470, 6.249999999999982236, -133.1919872981078470 ) ) ;
#16935=ADVANCED_FACE ( 'NONE', ( #23135 ), #27544, .T. ) ;
#16936=CARTESIAN_POINT ( 'NONE',  ( -5.196152422706601826, 2.999999999999975131, -129.0386751345948824 ) ) ;
#16938=CARTESIAN_POINT ( 'NONE',  ( -5.196152422706573404, -3.000000000000002665, -130.2886751345948539 ) ) ;
#16939=CARTESIAN_POINT ( 'NONE',  ( -5.999999999999963585, -1.487416814333745711E-14, -92.91367513459482552 ) ) ;
#16947=CARTESIAN_POINT ( 'NONE',  ( -4.763139720814407951, 2.749999999999946709, -134.7500000000000284 ) ) ;
#16950=VERTEX_POINT ( 'NONE', #2234 ) ;
#16952=CARTESIAN_POINT ( 'NONE',  ( 3.464101615137757051, -5.999999999999979572, -132.9136751345947971 ) ) ;
#16954=( BOUNDED_CURVE ( )  B_SPLINE_CURVE ( 2, ( #17328, #26644, #5603, #24349, #3302, #9648, #5009, #14441, #13034 ),
 .UNSPECIFIED., .F., .T. ) 
 B_SPLINE_CURVE_WITH_KNOTS ( ( 3, 2, 2, 2, 3 ),
 ( 0.7638888888888889506, 0.7648148148148148362, 0.7666666666666667185, 0.7685185185185184897, 0.7694444444444443754 ),
 .UNSPECIFIED. ) 
 CURVE ( )  GEOMETRIC_REPRESENTATION_ITEM ( )  RATIONAL_B_SPLINE_CURVE ( ( 0.9330127018922194093, 0.9330127018922234061, 1.000000000000000000, 0.8660254037844388186, 1.000000000000000000, 0.8660254037844388186, 1.000000000000000000, 0.9330127018922234061, 0.9330127018922194093 ) ) 
 REPRESENTATION_ITEM ( '' )  );
#16958=CARTESIAN_POINT ( 'NONE',  ( 7.216878364870455975, -6.409875621278545621E-14, -92.94198729810784698 ) ) ;
#16959=CARTESIAN_POINT ( 'NONE',  ( 6.000000000000000888, -3.330669073875464691E-16, -7.560779664488942560E-35 ) ) ;
#16964=CARTESIAN_POINT ( 'NONE',  ( -3.175426480542816510, 5.499999999999865885, -128.8750000000000000 ) ) ;
#16965=ORIENTED_EDGE ( 'NONE', *, *, #22013, .T. ) ;
#16972=CARTESIAN_POINT ( 'NONE',  ( 0.000000000000000000, 5.499999999999991118, -58.50000000000000000 ) ) ;
#16973=CARTESIAN_POINT ( 'NONE',  ( -5.999999999999963585, 1.780251999655701777E-13, -81.83632486540521711 ) ) ;
#16974=CARTESIAN_POINT ( 'NONE',  ( 3.608439182435180470, -6.249999999999997335, -85.05801270189222407 ) ) ;
#16975=CYLINDRICAL_SURFACE ( 'NONE', #5914, 6.000000000000000888 ) ;
#16976=CARTESIAN_POINT ( 'NONE',  ( 6.000000000000000888, -3.330669073875464691E-16, -7.560779664488942560E-35 ) ) ;
#16977=CARTESIAN_POINT ( 'NONE',  ( -5.999999999999962697, 3.323446944526963891E-14, -161.3363248654052597 ) ) ;
#16978=CARTESIAN_POINT ( 'NONE',  ( 5.196152422706629359, 3.000000000000002665, -61.46132486540523132 ) ) ;
#16981=CARTESIAN_POINT ( 'NONE',  ( -3.175426480542816066, -5.500000000000057732, -143.3750000000000000 ) ) ;
#16982=AXIS2_PLACEMENT_3D ( 'NONE', #26687, #3344, #12772 ) ;
#16983=CARTESIAN_POINT ( 'NONE',  ( -5.999999999999919176, 1.607695154586804565, -68.40331216351300725 ) ) ;
#16984=CARTESIAN_POINT ( 'NONE',  ( 5.412658773652739619, 3.124999999999988898, -153.6830127018922099 ) ) ;
#16985=CARTESIAN_POINT ( 'NONE',  ( 6.000000000000000888, 1.607695154586715303, -159.0193375672974412 ) ) ;
#16987=CARTESIAN_POINT ( 'NONE',  ( -4.763139720814407951, 2.749999999999946709, -74.75000000000004263 ) ) ;
#16988=CARTESIAN_POINT ( 'NONE',  ( 6.350852961086080661, -9.614813431917819062E-14, -63.37500000000001421 ) ) ;
#16992=LINE ( 'NONE', #19287, #10182 ) ;
#16994=CARTESIAN_POINT ( 'NONE',  ( -5.196152422706601826, 2.999999999999975131, -81.96132486540518869 ) ) ;
#16995=ORIENTED_EDGE ( 'NONE', *, *, #8408, .T. ) ;
#16997=CARTESIAN_POINT ( 'NONE',  ( -5.196152422706573404, -3.000000000000002665, -158.7886751345948255 ) ) ;
#16998=CARTESIAN_POINT ( 'NONE',  ( -4.763139720814407951, -2.750000000000016431, -176.5000000000000000 ) ) ;
#17001=CARTESIAN_POINT ( 'NONE',  ( -5.412658773652684552, -3.125000000000099920, -155.0669872981078470 ) ) ;
#17003=ORIENTED_EDGE ( 'NONE', *, *, #18222, .F. ) ;
#17005=CARTESIAN_POINT ( 'NONE',  ( 3.175426480543072749, -5.500000000000105693, -81.62500000000002842 ) ) ;
#17006=CARTESIAN_POINT ( 'NONE',  ( -5.412658773652684552, -3.125000000000099920, -101.9330127018922525 ) ) ;
#17007=DIRECTION ( 'NONE',  ( -7.147005652999508048E-36, 5.642372883946980038E-36, 1.000000000000000000 ) ) ;
#17008=AXIS2_PLACEMENT_3D ( 'NONE', #13437, #27361, #22483 ) ;
#17010=EDGE_CURVE ( 'NONE', #15344, #1672, #11324, .T. ) ;
#17011=ADVANCED_FACE ( 'NONE', ( #3899 ), #11484, .T. ) ;
#17012=CARTESIAN_POINT ( 'NONE',  ( -4.763139720814407951, 2.749999999999946709, -166.2500000000000000 ) ) ;
#17014=CARTESIAN_POINT ( 'NONE',  ( -4.763139720814407951, 2.749999999999946709, -154.2500000000000000 ) ) ;
#17017=CARTESIAN_POINT ( 'NONE',  ( -2.775557561562891351E-14, -5.500000000000115463, -93.75000000000000000 ) ) ;
#17018=CARTESIAN_POINT ( 'NONE',  ( 6.000000000000000888, 1.607695154586715303, -126.0193375672974412 ) ) ;
#17020=CARTESIAN_POINT ( 'NONE',  ( 3.175426480543072749, -5.500000000000105693, -89.12500000000000000 ) ) ;
#17021=DIRECTION ( 'NONE',  ( -7.147005652999508048E-36, 5.642372883946980038E-36, 1.000000000000000000 ) ) ;
#17022=CARTESIAN_POINT ( 'NONE',  ( 0.000000000000000000, 5.999999999999977796, -143.7113248654052313 ) ) ;
#17025=CARTESIAN_POINT ( 'NONE',  ( -5.999999999999956479, -1.607695154586745057, -66.76933756729744118 ) ) ;
#17028=ORIENTED_EDGE ( 'NONE', *, *, #18895, .T. ) ;
#17029=CARTESIAN_POINT ( 'NONE',  ( -5.999999999999963585, -1.487416814333745711E-14, -170.3363248654052313 ) ) ;
#17030=ORIENTED_EDGE ( 'NONE', *, *, #24347, .T. ) ;
#17032=VERTEX_POINT ( 'NONE', #30022 ) ;
#17034=CARTESIAN_POINT ( 'NONE',  ( 4.763139720814407951, 2.750000000000002665, -105.2500000000000142 ) ) ;
#17038=CARTESIAN_POINT ( 'NONE',  ( -5.412658773652684552, -3.125000000000099920, -121.4330127018922241 ) ) ;
#17039=ORIENTED_EDGE ( 'NONE', *, *, #4660, .T. ) ;
#17040=CARTESIAN_POINT ( 'NONE',  ( 6.000000000000000888, 1.743066579297358182E-13, -60.66367513459481842 ) ) ;
#17041=CARTESIAN_POINT ( 'NONE',  ( 5.412658773652712085, -3.125000000000086153, -163.5669872981078186 ) ) ;
#17044=CARTESIAN_POINT ( 'NONE',  ( 3.608439182435180470, -6.249999999999997335, -62.55801270189225249 ) ) ;
#17045=EDGE_LOOP ( 'NONE', ( #7920, #20718, #15567, #1743 ) ) ;
#17046=CARTESIAN_POINT ( 'NONE',  ( 0.000000000000000000, 5.999999999999977796, -117.2886751345948397 ) ) ;
#17048=CARTESIAN_POINT ( 'NONE',  ( -5.950275682033375979, 9.251745015924212723, -24.20335556275641054 ) ) ;
#17051=CARTESIAN_POINT ( 'NONE',  ( 3.175426480543072749, -5.500000000000105693, -179.1250000000000568 ) ) ;
#17053=CARTESIAN_POINT ( 'NONE',  ( 6.000000000000000888, -1.859271017917181981E-14, -168.6636751345947971 ) ) ;
#17054=CARTESIAN_POINT ( 'NONE',  ( 5.412658773652712085, -3.125000000000086153, -170.4330127018922667 ) ) ;
#17057=CARTESIAN_POINT ( 'NONE',  ( -6.350852961085760029, -1.281975124255709124E-13, -118.1250000000000426 ) ) ;
#17059=CARTESIAN_POINT ( 'NONE',  ( -6.350852961085760029, -1.281975124255709124E-13, -116.6250000000000000 ) ) ;
#17060=FACE_OUTER_BOUND ( 'NONE', #8462, .T. ) ;
#17061=CARTESIAN_POINT ( 'NONE',  ( 6.000000000000000888, -1.859271017917181981E-14, -54.08632486540521001 ) ) ;
#17062=ORIENTED_EDGE ( 'NONE', *, *, #12034, .T. ) ;
#17065=CARTESIAN_POINT ( 'NONE',  ( -5.196152422706601826, 2.999999999999975131, -108.9613248654052171 ) ) ;
#17066=CARTESIAN_POINT ( 'NONE',  ( -3.464101615137757051, -5.999999999999979572, -146.0863248654052029 ) ) ;
#17067=ORIENTED_EDGE ( 'NONE', *, *, #20951, .F. ) ;
#17073=ORIENTED_EDGE ( 'NONE', *, *, #13694, .T. ) ;
#17077=EDGE_CURVE ( 'NONE', #21702, #28373, #14196, .T. ) ;
#17079=ORIENTED_EDGE ( 'NONE', *, *, #16481, .F. ) ;
#17080=CARTESIAN_POINT ( 'NONE',  ( 5.412658773652712085, -3.125000000000086153, -135.0669872981078470 ) ) ;
#17082=CARTESIAN_POINT ( 'NONE',  ( -3.464101615137725076, 5.999999999999979572, -130.6636751345948539 ) ) ;
#17083=CARTESIAN_POINT ( 'NONE',  ( 3.464101615137852974, 5.999999999999884537, -129.4136751345948255 ) ) ;
#17090=FACE_OUTER_BOUND ( 'NONE', #8791, .T. ) ;
#17091=CARTESIAN_POINT ( 'NONE',  ( -3.464101615137757051, -5.999999999999979572, -140.0863248654051745 ) ) ;
#17093=CARTESIAN_POINT ( 'NONE',  ( -5.196152422706573404, -3.000000000000002665, -69.71132486540521711 ) ) ;
#17095=CARTESIAN_POINT ( 'NONE',  ( 0.000000000000000000, 5.499999999999991118, -139.5000000000000000 ) ) ;
#17097=ORIENTED_EDGE ( 'NONE', *, *, #7241, .F. ) ;
#17098=CARTESIAN_POINT ( 'NONE',  ( -4.763139720814407951, -2.750000000000016431, -47.49999999999998579 ) ) ;
#17099=CARTESIAN_POINT ( 'NONE',  ( 0.000000000000000000, 0.000000000000000000, 0.000000000000000000 ) ) ;
#17101=CARTESIAN_POINT ( 'NONE',  ( 5.999999999999949374, 1.607695154586804565, -153.0193375672974412 ) ) ;
#17106=CARTESIAN_POINT ( 'NONE',  ( -5.412658773652739619, 3.124999999999975131, -92.31698729810783277 ) ) ;
#17107=CARTESIAN_POINT ( 'NONE',  ( -5.999999999999963585, -1.487416814333745711E-14, -172.4136751345948255 ) ) ;
#17112=CARTESIAN_POINT ( 'NONE',  ( 3.175426480543072749, -5.500000000000105693, -129.6250000000000284 ) ) ;
#17113=EDGE_CURVE ( 'NONE', #12780, #13246, #26712, .T. ) ;
#17116=CARTESIAN_POINT ( 'NONE',  ( -5.999999999999956479, -1.607695154586745057, -138.7693375672974412 ) ) ;
#17117=CARTESIAN_POINT ( 'NONE',  ( -6.350852961085760029, -1.281975124255709124E-13, -59.62500000000000000 ) ) ;
#17121=CARTESIAN_POINT ( 'NONE',  ( 3.608439182435180470, 6.249999999999982236, -83.05801270189220986 ) ) ;
#17122=CYLINDRICAL_SURFACE ( 'NONE', #20180, 6.000000000000000888 ) ;
#17123=CARTESIAN_POINT ( 'NONE',  ( -3.464101615137757051, -5.999999999999979572, -152.6636751345947971 ) ) ;
#17125=DIRECTION ( 'NONE',  ( 1.000000000000000000, -5.551115123125773458E-17, -1.260129944081490338E-35 ) ) ;
#17127=( BOUNDED_CURVE ( )  B_SPLINE_CURVE ( 2, ( #24500, #19907, #29252, #23302, #18544, #11334, #20521, #27553, #13641 ),
 .UNSPECIFIED., .F., .T. ) 
 B_SPLINE_CURVE_WITH_KNOTS ( ( 3, 2, 2, 2, 3 ),
 ( 0.6861111111111111160, 0.6870370370370371127, 0.6888888888888888840, 0.6907407407407407662, 0.6916666666666666519 ),
 .UNSPECIFIED. ) 
 CURVE ( )  GEOMETRIC_REPRESENTATION_ITEM ( )  RATIONAL_B_SPLINE_CURVE ( ( 0.9330127018922194093, 0.9330127018922194093, 1.000000000000000000, 0.8660254037844388186, 1.000000000000000000, 0.8660254037844388186, 1.000000000000000000, 0.9330127018922234061, 0.9330127018922194093 ) ) 
 REPRESENTATION_ITEM ( '' )  );
#17128=CARTESIAN_POINT ( 'NONE',  ( -4.763139720814407951, -2.750000000000016431, -143.5000000000000284 ) ) ;
#17130=CARTESIAN_POINT ( 'NONE',  ( 2.775557561562891351E-14, -6.250000000000061284, -152.6830127018922099 ) ) ;
#17132=CARTESIAN_POINT ( 'NONE',  ( 0.000000000000000000, 5.499999999999991118, -75.00000000000001421 ) ) ;
#17133=CARTESIAN_POINT ( 'NONE',  ( 6.350852961086080661, -9.614813431917819062E-14, -58.87500000000005684 ) ) ;
#17134=( BOUNDED_CURVE ( )  B_SPLINE_CURVE ( 2, ( #8372, #17782, #27102, #13332, #1613, #27397, #6362, #27859, #13792 ),
 .UNSPECIFIED., .F., .T. ) 
 B_SPLINE_CURVE_WITH_KNOTS ( ( 3, 2, 2, 2, 3 ),
 ( 0.5472222222222222765, 0.5481481481481481621, 0.5500000000000000444, 0.5518518518518518157, 0.5527777777777778123 ),
 .UNSPECIFIED. ) 
 CURVE ( )  GEOMETRIC_REPRESENTATION_ITEM ( )  RATIONAL_B_SPLINE_CURVE ( ( 0.9330127018922194093, 0.9330127018922234061, 1.000000000000000000, 0.8660254037844388186, 1.000000000000000000, 0.8660254037844388186, 1.000000000000000000, 0.9330127018922154125, 0.9330127018922194093 ) ) 
 REPRESENTATION_ITEM ( '' )  );
#17135=CARTESIAN_POINT ( 'NONE',  ( 5.196152422706629359, 3.000000000000002665, -53.96132486540522422 ) ) ;
#17138=B_SPLINE_CURVE_WITH_KNOTS ( 'NONE', 3,
 ( #18284, #6269, #15688, #27596, #24998, #3952, #13378, #6573, #1665, #11059, #20405, #18128, #6412, #25147, #15997, #7940, #3321, #17350, #3174, #26228, #19493, #17048, #5476, #28974, #12749, #28822, #5625, #22089, #26665, #9668, #15031, #5026, #12595, #21500, #21645, #26086, #24377, #26378, #19058, #21937, #3031, #5180, #2882, #2727 ),
 .UNSPECIFIED., .F., .F.,
 ( 4, 2, 2, 2, 2, 2, 2, 2, 2, 2, 2, 2, 2, 2, 2, 2, 2, 2, 2, 2, 2, 4 ),
 ( 0.000000000000000000, 0.001197331758471044914, 0.002394663516942089829, 0.003591995275413134743, 0.004789327033884179657, 0.005387992913119706018, 0.005986658792355230643, 0.007183990550826279894, 0.008381322309297329146, 0.009578654067768378397, 0.01017731994700390302, 0.01077598582623942765, 0.01137465170547495227, 0.01197331758471047516, 0.01317064934318152615, 0.01376931522241705598, 0.01436798110165258408, 0.01556531286012364373, 0.01676264461859470339, 0.01736131049783023322, 0.01795997637706576652, 0.01915730813553682965 ),
 .UNSPECIFIED. ) ;
#17140=CARTESIAN_POINT ( 'NONE',  ( -3.464101615137757051, -5.999999999999979572, -89.08632486540521711 ) ) ;
#17141=CARTESIAN_POINT ( 'NONE',  ( -3.464101615137725076, 5.999999999999979572, -82.08632486540517448 ) ) ;
#17147=CARTESIAN_POINT ( 'NONE',  ( 6.350852961086080661, -9.614813431917819062E-14, -178.8750000000000284 ) ) ;
#17149=CARTESIAN_POINT ( 'NONE',  ( -5.412658773652739619, 3.124999999999975131, -155.3169872981078470 ) ) ;
#17151=CARTESIAN_POINT ( 'NONE',  ( -6.350852961085760029, -1.281975124255709124E-13, -82.12500000000004263 ) ) ;
#17153=CARTESIAN_POINT ( 'NONE',  ( 5.412658773652739619, 3.124999999999988898, -102.6830127018922241 ) ) ;
#17154=ORIENTED_EDGE ( 'NONE', *, *, #4003, .F. ) ;
#17159=CARTESIAN_POINT ( 'NONE',  ( 0.000000000000000000, 5.499999999999991118, -160.5000000000000284 ) ) ;
#17160=CARTESIAN_POINT ( 'NONE',  ( 3.464101615137757051, -5.999999999999979572, -80.41367513459479710 ) ) ;
#17161=CARTESIAN_POINT ( 'NONE',  ( -2.775557561562891351E-14, -5.500000000000115463, -144.7500000000000568 ) ) ;
#17164=CARTESIAN_POINT ( 'NONE',  ( 3.175426480543072749, -5.500000000000105693, -96.62500000000004263 ) ) ;
#17166=CARTESIAN_POINT ( 'NONE',  ( -3.464101615137757051, -5.999999999999979572, -131.0863248654052029 ) ) ;
#17167=CARTESIAN_POINT ( 'NONE',  ( -4.763139720814407951, -2.750000000000016431, -79.00000000000001421 ) ) ;
#17173=CARTESIAN_POINT ( 'NONE',  ( 5.196152422706629359, 3.000000000000002665, -126.5386751345948255 ) ) ;
#17175=CARTESIAN_POINT ( 'NONE',  ( 6.000000000000000888, -3.330669073875464691E-16, -7.560779664488942560E-35 ) ) ;
#17176=ORIENTED_EDGE ( 'NONE', *, *, #19792, .F. ) ;
#17182=VERTEX_POINT ( 'NONE', #16552 ) ;
#17183=EDGE_CURVE ( 'NONE', #25369, #26795, #22766, .T. ) ;
#17184=EDGE_CURVE ( 'NONE', #28549, #20877, #17665, .T. ) ;
#17186=ORIENTED_EDGE ( 'NONE', *, *, #9744, .F. ) ;
#17187=CARTESIAN_POINT ( 'NONE',  ( 4.763139720814407951, 2.750000000000002665, -103.7500000000000142 ) ) ;
#17190=CARTESIAN_POINT ( 'NONE',  ( -3.608439182435115633, 6.249999999999965361, -126.3080127018922383 ) ) ;
#17192=CARTESIAN_POINT ( 'NONE',  ( 5.196152422706629359, -2.999999999999988898, -110.2886751345948397 ) ) ;
#17193=CARTESIAN_POINT ( 'NONE',  ( -5.412658773652739619, 3.124999999999975131, -161.3169872981078470 ) ) ;
#17196=CARTESIAN_POINT ( 'NONE',  ( -7.216878364870328078, 0.000000000000000000, -60.05801270189223118 ) ) ;
#17200=DIRECTION ( 'NONE',  ( -7.147005652999508048E-36, 5.642372883946980038E-36, 1.000000000000000000 ) ) ;
#17201=CARTESIAN_POINT ( 'NONE',  ( -2.775557561562891351E-14, -5.500000000000115463, -170.2500000000000000 ) ) ;
#17203=CARTESIAN_POINT ( 'NONE',  ( 3.464101615137852974, 5.999999999999884537, -100.3363248654052029 ) ) ;
#17204=CARTESIAN_POINT ( 'NONE',  ( 5.412658773652712085, -3.125000000000086153, -171.9330127018922099 ) ) ;
#17205=CARTESIAN_POINT ( 'NONE',  ( 0.000000000000000000, 0.000000000000000000, 0.000000000000000000 ) ) ;
#17206=CARTESIAN_POINT ( 'NONE',  ( -4.763139720814407951, 2.749999999999946709, -113.7500000000000142 ) ) ;
#17207=CARTESIAN_POINT ( 'NONE',  ( 3.175426480543072749, -5.500000000000105693, -113.1250000000000000 ) ) ;
#17208=CARTESIAN_POINT ( 'NONE',  ( 3.464101615137757051, -5.999999999999979572, -131.4136751345947687 ) ) ;
#17209=ORIENTED_EDGE ( 'NONE', *, *, #18843, .F. ) ;
#17212=EDGE_CURVE ( 'NONE', #8939, #1, #25891, .T. ) ;
#17214=CARTESIAN_POINT ( 'NONE',  ( -6.000000000000000888, 1.067854986875958443E-15, 7.560779664488942560E-35 ) ) ;
#17219=CARTESIAN_POINT ( 'NONE',  ( 5.412658773652712085, -3.125000000000086153, -85.56698729810786119 ) ) ;
#17220=CARTESIAN_POINT ( 'NONE',  ( -5.999999999999963585, 1.780251999655701777E-13, -109.4136751345948113 ) ) ;
#17221=EDGE_LOOP ( 'NONE', ( #16125, #24036, #10294, #15530 ) ) ;
#17224=( BOUNDED_CURVE ( )  B_SPLINE_CURVE ( 2, ( #21397, #2491, #11914, #635, #7542, #9722, #330, #28720, #5380 ),
 .UNSPECIFIED., .F., .T. ) 
 B_SPLINE_CURVE_WITH_KNOTS ( ( 3, 2, 2, 2, 3 ),
 ( 0.3083333333333333481, 0.3092592592592592338, 0.3111111111111111160, 0.3129629629629629983, 0.3138888888888888840 ),
 .UNSPECIFIED. ) 
 CURVE ( )  GEOMETRIC_REPRESENTATION_ITEM ( )  RATIONAL_B_SPLINE_CURVE ( ( 0.9330127018922194093, 0.9330127018922194093, 1.000000000000000000, 0.8660254037844388186, 1.000000000000000000, 0.8660254037844388186, 1.000000000000000000, 0.9330127018922194093, 0.9330127018922194093 ) ) 
 REPRESENTATION_ITEM ( '' )  );
#17225=ORIENTED_EDGE ( 'NONE', *, *, #14195, .F. ) ;
#17226=EDGE_LOOP ( 'NONE', ( #16304, #7340, #29448, #13643 ) ) ;
#17230=EDGE_LOOP ( 'NONE', ( #8215, #20491, #8110, #1579 ) ) ;
#17231=CARTESIAN_POINT ( 'NONE',  ( 3.608439182435180470, -6.249999999999997335, -132.1919872981078470 ) ) ;
#17232=CARTESIAN_POINT ( 'NONE',  ( 3.464101615137757051, -5.999999999999979572, -167.4136751345948255 ) ) ;
#17237=CARTESIAN_POINT ( 'NONE',  ( -6.000000000000000888, 1.067854986875958443E-15, 7.560779664488942560E-35 ) ) ;
#17240=CARTESIAN_POINT ( 'NONE',  ( -5.196152422706573404, -3.000000000000002665, -99.71132486540523132 ) ) ;
#17241=DIRECTION ( 'NONE',  ( -7.147005652999508048E-36, 5.642372883946980038E-36, 1.000000000000000000 ) ) ;
#17242=CARTESIAN_POINT ( 'NONE',  ( -5.196152422706573404, -3.000000000000002665, -162.7113248654051745 ) ) ;
#17246=CARTESIAN_POINT ( 'NONE',  ( 4.763139720814407951, 2.750000000000002665, -138.2499999999999716 ) ) ;
#17250=CARTESIAN_POINT ( 'NONE',  ( 0.000000000000000000, 5.499999999999991118, -48.00000000000004263 ) ) ;
#17252=CARTESIAN_POINT ( 'NONE',  ( 6.000000000000000888, 1.743066579297358182E-13, -99.66367513459479710 ) ) ;
#17253=EDGE_CURVE ( 'NONE', #14683, #3959, #8135, .T. ) ;
#17254=ORIENTED_EDGE ( 'NONE', *, *, #5075, .T. ) ;
#17258=CARTESIAN_POINT ( 'NONE',  ( 7.216878364870455975, -6.409875621278545621E-14, -98.94198729810781856 ) ) ;
#17260=CARTESIAN_POINT ( 'NONE',  ( 6.000000000000052403, -1.607695154586662678, -50.23066243270261566 ) ) ;
#17263=DIRECTION ( 'NONE',  ( 1.000000000000000000, -5.551115123125773458E-17, -1.260129944081490338E-35 ) ) ;
#17268=CARTESIAN_POINT ( 'NONE',  ( -4.763139720814407951, 2.749999999999946709, -58.25000000000002132 ) ) ;
#17269=( BOUNDED_CURVE ( )  B_SPLINE_CURVE ( 2, ( #13438, #8167, #24607, #27061, #6026, #10827, #29531, #15444, #3713 ),
 .UNSPECIFIED., .F., .F. ) 
 B_SPLINE_CURVE_WITH_KNOTS ( ( 3, 2, 2, 2, 3 ),
 ( 0.9749999999999999778, 0.9759259259259259744, 0.9777777777777777457, 0.9796296296296296280, 0.9805555555555555136 ),
 .UNSPECIFIED. ) 
 CURVE ( )  GEOMETRIC_REPRESENTATION_ITEM ( )  RATIONAL_B_SPLINE_CURVE ( ( 0.9330127018922194093, 0.9330127018922154125, 1.000000000000000000, 0.8660254037844388186, 1.000000000000000000, 0.8660254037844388186, 1.000000000000000000, 0.9330127018922234061, 0.9330127018922194093 ) ) 
 REPRESENTATION_ITEM ( '' )  );
#17270=CARTESIAN_POINT ( 'NONE',  ( -5.999999999999919176, 1.607695154586804565, -68.98066243270260145 ) ) ;
#17271=CYLINDRICAL_SURFACE ( 'NONE', #28892, 6.000000000000000888 ) ;
#17272=CARTESIAN_POINT ( 'NONE',  ( 3.464101615137852974, 5.999999999999884537, -67.91367513459479710 ) ) ;
#17273=CARTESIAN_POINT ( 'NONE',  ( 3.608439182435180470, 6.249999999999982236, -72.55801270189222407 ) ) ;
#17275=CARTESIAN_POINT ( 'NONE',  ( 5.196152422706629359, 3.000000000000002665, -169.4613248654052029 ) ) ;
#17276=CARTESIAN_POINT ( 'NONE',  ( -3.464101615137757051, -5.999999999999979572, -168.5863248654051745 ) ) ;
#17279=CARTESIAN_POINT ( 'NONE',  ( -3.464101615137757051, -5.999999999999979572, -94.16367513459479710 ) ) ;
#17280=CARTESIAN_POINT ( 'NONE',  ( 0.000000000000000000, 5.499999999999991118, -142.5000000000000284 ) ) ;
#17282=CARTESIAN_POINT ( 'NONE',  ( 3.608439182435180470, 6.249999999999982236, -152.0580127018922383 ) ) ;
#17285=CARTESIAN_POINT ( 'NONE',  ( -4.763139720814407951, 2.749999999999946709, -71.75000000000004263 ) ) ;
#17286=CARTESIAN_POINT ( 'NONE',  ( 3.175426480543072749, -5.500000000000105693, -54.62500000000003553 ) ) ;
#17292=CARTESIAN_POINT ( 'NONE',  ( 5.196152422706629359, 3.000000000000002665, -98.03867513459485394 ) ) ;
#17300=CARTESIAN_POINT ( 'NONE',  ( -7.216878364870328078, 0.000000000000000000, -47.19198729810782567 ) ) ;
#17302=CARTESIAN_POINT ( 'NONE',  ( -5.412658773652684552, -3.125000000000099920, -150.5669872981077901 ) ) ;
#17304=CARTESIAN_POINT ( 'NONE',  ( -3.175426480542816510, -5.500000000000057732, -81.87500000000004263 ) ) ;
#17307=ORIENTED_EDGE ( 'NONE', *, *, #8328, .F. ) ;
#17308=CARTESIAN_POINT ( 'NONE',  ( -6.000000000000007105, -1.607695154586655129, -128.2693375672974128 ) ) ;
#17311=CARTESIAN_POINT ( 'NONE',  ( 0.000000000000000000, 0.000000000000000000, 0.000000000000000000 ) ) ;
#17313=CARTESIAN_POINT ( 'NONE',  ( -5.999999999999963585, -1.487416814333745711E-14, -59.33632486540522422 ) ) ;
#17314=CARTESIAN_POINT ( 'NONE',  ( -3.175426480542816066, -5.500000000000057732, -164.3750000000000568 ) ) ;
#17315=CARTESIAN_POINT ( 'NONE',  ( 5.196152422706629359, -2.999999999999988898, -60.21132486540520290 ) ) ;
#17316=CARTESIAN_POINT ( 'NONE',  ( -6.350852961085760029, -1.281975124255709124E-13, -145.1250000000000284 ) ) ;
#17318=CARTESIAN_POINT ( 'NONE',  ( 6.000000000000052403, -1.607695154586662678, -51.73066243270262277 ) ) ;
#17319=CARTESIAN_POINT ( 'NONE',  ( 3.175426480543072749, -5.500000000000105693, -95.12500000000002842 ) ) ;
#17320=CARTESIAN_POINT ( 'NONE',  ( 6.350852961086080661, -9.614813431917819062E-14, -79.87500000000001421 ) ) ;
#17321=ADVANCED_FACE ( 'NONE', ( #18887 ), #7030, .F. ) ;
#17323=CARTESIAN_POINT ( 'NONE',  ( 0.000000000000000000, -5.999999999999991118, -72.46132486540524553 ) ) ;
#17326=CARTESIAN_POINT ( 'NONE',  ( -5.999999999999963585, -1.487416814333745711E-14, -128.3363248654052029 ) ) ;
#17328=CARTESIAN_POINT ( 'NONE',  ( 6.000000000000000888, 1.743066579297358182E-13, -78.66367513459482552 ) ) ;
#17331=CARTESIAN_POINT ( 'NONE',  ( 0.000000000000000000, 0.000000000000000000, 0.000000000000000000 ) ) ;
#17332=CARTESIAN_POINT ( 'NONE',  ( 5.196152422706629359, -2.999999999999988898, -78.78867513459486815 ) ) ;
#17334=VERTEX_POINT ( 'NONE', #27341 ) ;
#17335=ORIENTED_EDGE ( 'NONE', *, *, #1174, .F. ) ;
#17336=CARTESIAN_POINT ( 'NONE',  ( -6.350852961085760029, -1.281975124255709124E-13, -104.6250000000000142 ) ) ;
#17338=CARTESIAN_POINT ( 'NONE',  ( 5.412658773652739619, 3.124999999999988898, -123.6830127018922525 ) ) ;
#17339=CIRCLE ( 'NONE', #4057, 0.9999999999999991118 ) ;
#17340=EDGE_LOOP ( 'NONE', ( #4381, #17676, #19761, #15298 ) ) ;
#17341=CARTESIAN_POINT ( 'NONE',  ( -5.999999999999963585, 8.134310703387671600E-14, -135.8363248654052597 ) ) ;
#17342=CARTESIAN_POINT ( 'NONE',  ( 2.775557561562891351E-14, 6.250000000000033751, -163.0669872981078186 ) ) ;
#17343=DIRECTION ( 'NONE',  ( -7.147005652999508048E-36, 5.642372883946980038E-36, 1.000000000000000000 ) ) ;
#17346=CARTESIAN_POINT ( 'NONE',  ( 3.608439182435180470, 6.249999999999982236, -60.55801270189223118 ) ) ;
#17348=DIRECTION ( 'NONE',  ( -7.147005652999508048E-36, 5.642372883946980038E-36, 1.000000000000000000 ) ) ;
#17349=CARTESIAN_POINT ( 'NONE',  ( -6.000000000000000888, 1.067854986875958443E-15, 7.560779664488942560E-35 ) ) ;
#17350=CARTESIAN_POINT ( 'NONE',  ( -5.959171229995748220, 9.246457381727791969, -25.80348449789763876 ) ) ;
#17352=CARTESIAN_POINT ( 'NONE',  ( -6.350852961085760029, -1.281975124255709124E-13, -167.6249999999999716 ) ) ;
#17354=CARTESIAN_POINT ( 'NONE',  ( -5.999999999999919176, 1.607695154586804565, -99.90331216351299304 ) ) ;
#17355=CARTESIAN_POINT ( 'NONE',  ( 5.412658773652739619, 3.124999999999988898, -165.6830127018922383 ) ) ;
#17356=CARTESIAN_POINT ( 'NONE',  ( 5.999999999999949374, 1.607695154586804565, -48.59668783648704249 ) ) ;
#17357=DIRECTION ( 'NONE',  ( 1.000000000000000000, -5.551115123125773458E-17, -1.260129944081490338E-35 ) ) ;
#17359=EDGE_CURVE ( 'NONE', #4337, #26795, #8616, .T. ) ;
#17360=CARTESIAN_POINT ( 'NONE',  ( 3.175426480543072749, 5.499999999999865885, -106.6250000000000284 ) ) ;
#17361=CYLINDRICAL_SURFACE ( 'NONE', #20014, 6.000000000000000888 ) ;
#17364=ORIENTED_EDGE ( 'NONE', *, *, #21840, .T. ) ;
#17367=AXIS2_PLACEMENT_3D ( 'NONE', #18579, #2424, #13678 ) ;
#17368=ORIENTED_EDGE ( 'NONE', *, *, #12931, .F. ) ;
#17369=CARTESIAN_POINT ( 'NONE',  ( 3.608439182435180470, -6.249999999999997335, -82.69198729810781856 ) ) ;
#17371=CYLINDRICAL_SURFACE ( 'NONE', #16982, 6.000000000000000888 ) ;
#17373=EDGE_LOOP ( 'NONE', ( #17079, #16927 ) ) ;
#17376=CARTESIAN_POINT ( 'NONE',  ( 7.216878364870455975, -6.409875621278545621E-14, -133.4419872981077901 ) ) ;
#17380=EDGE_CURVE ( 'NONE', #24771, #22382, #20152, .T. ) ;
#17381=ORIENTED_EDGE ( 'NONE', *, *, #23855, .T. ) ;
#17387=CARTESIAN_POINT ( 'NONE',  ( 5.412658773652739619, 3.124999999999988898, -67.31698729810780435 ) ) ;
#17388=CARTESIAN_POINT ( 'NONE',  ( 5.412658773652712085, -3.125000000000086153, -57.06698729810783277 ) ) ;
#17390=CARTESIAN_POINT ( 'NONE',  ( -5.999999999999963585, -1.487416814333745711E-14, -128.9136751345948539 ) ) ;
#17392=CARTESIAN_POINT ( 'NONE',  ( -5.999999999999963585, 1.780251999655701777E-13, -74.33632486540523132 ) ) ;
#17394=CARTESIAN_POINT ( 'NONE',  ( 6.350852961086080661, -9.614813431917819062E-14, -127.8749999999999858 ) ) ;
#17395=EDGE_CURVE ( 'NONE', #25470, #28274, #15884, .T. ) ;
#17397=EDGE_LOOP ( 'NONE', ( #23347, #14185, #2606, #13562 ) ) ;
#17400=CARTESIAN_POINT ( 'NONE',  ( -5.196152422706573404, -3.000000000000002665, -160.2886751345948824 ) ) ;
#17407=CARTESIAN_POINT ( 'NONE',  ( -3.608439182435052128, -6.250000000000110134, -96.44198729810780435 ) ) ;
#17408=CARTESIAN_POINT ( 'NONE',  ( 5.196152422706629359, -2.999999999999988898, -78.21132486540521711 ) ) ;
#17417=CARTESIAN_POINT ( 'NONE',  ( 3.175426480543072749, 5.499999999999865885, -55.62500000000003553 ) ) ;
#17420=CARTESIAN_POINT ( 'NONE',  ( -5.196152422706573404, -3.000000000000002665, -51.71132486540519579 ) ) ;
#17421=CARTESIAN_POINT ( 'NONE',  ( 5.412658773652739619, 3.124999999999988898, -78.68301270189226670 ) ) ;
#17422=DIRECTION ( 'NONE',  ( 1.000000000000000000, -5.551115123125774690E-17, 0.000000000000000000 ) ) ;
#17425=EDGE_CURVE ( 'NONE', #30226, #20441, #19473, .T. ) ;
#17426=CARTESIAN_POINT ( 'NONE',  ( 3.175426480543072749, 5.499999999999865885, -129.1250000000000284 ) ) ;
#17427=CARTESIAN_POINT ( 'NONE',  ( -5.999999999999904965, -1.607695154586834541, -177.7693375672974412 ) ) ;
#17428=CARTESIAN_POINT ( 'NONE',  ( -5.999999999999963585, -1.487416814333745711E-14, -71.33632486540521711 ) ) ;
#17429=CARTESIAN_POINT ( 'NONE',  ( 6.000000000000000888, -1.859271017917181981E-14, -67.58632486540523132 ) ) ;
#17430=CARTESIAN_POINT ( 'NONE',  ( 0.000000000000000000, 5.499999999999991118, -72.00000000000001421 ) ) ;
#17432=CARTESIAN_POINT ( 'NONE',  ( -4.763139720814407951, 2.749999999999946709, -61.25000000000002842 ) ) ;
#17434=ORIENTED_EDGE ( 'NONE', *, *, #17887, .T. ) ;
#17445=CARTESIAN_POINT ( 'NONE',  ( 4.763139720814407951, -2.749999999999988454, -143.0000000000000284 ) ) ;
#17446=CARTESIAN_POINT ( 'NONE',  ( 4.763139720814407951, 2.750000000000002665, -175.7500000000000284 ) ) ;
#17449=CARTESIAN_POINT ( 'NONE',  ( -3.608439182435115633, 6.249999999999965361, -150.9419872981077901 ) ) ;
#17450=CARTESIAN_POINT ( 'NONE',  ( 3.175426480543072749, -5.500000000000105693, -80.12500000000002842 ) ) ;
#17452=ADVANCED_FACE ( 'NONE', ( #12428 ), #19612, .T. ) ;
#17453=CARTESIAN_POINT ( 'NONE',  ( -5.412658773652739619, 3.124999999999975131, -97.68301270189222407 ) ) ;
#17454=ORIENTED_EDGE ( 'NONE', *, *, #271, .T. ) ;
#17456=CARTESIAN_POINT ( 'NONE',  ( 6.000000000000052403, -1.607695154586662678, -96.15331216351300725 ) ) ;
#17457=CARTESIAN_POINT ( 'NONE',  ( 3.464101615137757051, -5.999999999999979572, -150.9136751345947971 ) ) ;
#17460=CARTESIAN_POINT ( 'NONE',  ( 4.763139720814407951, -2.749999999999988454, -164.0000000000000284 ) ) ;
#17461=CARTESIAN_POINT ( 'NONE',  ( -2.775557561562891351E-14, -5.500000000000115463, -146.2500000000000000 ) ) ;
#17462=DIRECTION ( 'NONE',  ( -7.147005652999508048E-36, 5.642372883946980038E-36, 1.000000000000000000 ) ) ;
#17464=CARTESIAN_POINT ( 'NONE',  ( 4.763139720814407951, 2.750000000000002665, -94.75000000000000000 ) ) ;
#17466=DIRECTION ( 'NONE',  ( 1.000000000000000000, -5.551115123125773458E-17, -1.260129944081490338E-35 ) ) ;
#17467=CARTESIAN_POINT ( 'NONE',  ( -3.175426480542816510, -5.500000000000057732, -84.87500000000004263 ) ) ;
#17468=CARTESIAN_POINT ( 'NONE',  ( 5.196152422706629359, -2.999999999999988898, -72.21132486540521711 ) ) ;
#17470=CARTESIAN_POINT ( 'NONE',  ( -5.196152422706601826, 2.999999999999975131, -131.4613248654052313 ) ) ;
#17474=CARTESIAN_POINT ( 'NONE',  ( 0.000000000000000000, 0.000000000000000000, 0.000000000000000000 ) ) ;
#17475=VERTEX_POINT ( 'NONE', #26502 ) ;
#17476=CARTESIAN_POINT ( 'NONE',  ( 4.000000000000003553, -2.220446049250311602E-16, -180.0000000000000568 ) ) ;
#17477=DIRECTION ( 'NONE',  ( -7.147005652999508048E-36, 5.642372883946980038E-36, 1.000000000000000000 ) ) ;
#17478=CARTESIAN_POINT ( 'NONE',  ( -5.999999999999963585, 1.780251999655701777E-13, -82.41367513459481131 ) ) ;
#17483=( BOUNDED_CURVE ( )  B_SPLINE_CURVE ( 2, ( #19175, #14721, #3009, #10102, #28507, #10255, #28802, #7335, #7764 ),
 .UNSPECIFIED., .F., .T. ) 
 B_SPLINE_CURVE_WITH_KNOTS ( ( 3, 2, 2, 2, 3 ),
 ( 0.01944444444444445169, 0.02037037037037037202, 0.02222222222222222307, 0.02407407407407407413, 0.02499999999999999445 ),
 .UNSPECIFIED. ) 
 CURVE ( )  GEOMETRIC_REPRESENTATION_ITEM ( )  RATIONAL_B_SPLINE_CURVE ( ( 0.9330127018922194093, 0.9330127018922198534, 1.000000000000000000, 0.8660254037844388186, 1.000000000000000000, 0.8660254037844388186, 1.000000000000000000, 0.9330127018922198534, 0.9330127018922195203 ) ) 
 REPRESENTATION_ITEM ( '' )  );
#17485=CARTESIAN_POINT ( 'NONE',  ( -4.763139720814407951, 2.749999999999946709, -109.2500000000000142 ) ) ;
#17486=EDGE_CURVE ( 'NONE', #17588, #22916, #20519, .T. ) ;
#17487=CARTESIAN_POINT ( 'NONE',  ( 2.775557561562891351E-14, 6.250000000000033751, -117.4330127018922099 ) ) ;
#17488=( BOUNDED_CURVE ( )  B_SPLINE_CURVE ( 2, ( #13013, #10700, #17770, #22515, #27089, #1447, #27240, #10855, #27999 ),
 .UNSPECIFIED., .F., .T. ) 
 B_SPLINE_CURVE_WITH_KNOTS ( ( 3, 2, 2, 2, 3 ),
 ( 0.7027777777777777235, 0.7037037037037037202, 0.7055555555555556024, 0.7074074074074073737, 0.7083333333333333703 ),
 .UNSPECIFIED. ) 
 CURVE ( )  GEOMETRIC_REPRESENTATION_ITEM ( )  RATIONAL_B_SPLINE_CURVE ( ( 0.9330127018922194093, 0.9330127018922154125, 1.000000000000000000, 0.8660254037844388186, 1.000000000000000000, 0.8660254037844388186, 1.000000000000000000, 0.9330127018922154125, 0.9330127018922194093 ) ) 
 REPRESENTATION_ITEM ( '' )  );
#17489=EDGE_LOOP ( 'NONE', ( #4752, #16786, #26609, #14867 ) ) ;
#17491=CARTESIAN_POINT ( 'NONE',  ( -3.608439182435052128, -6.250000000000110134, -156.4419872981078470 ) ) ;
#17494=EDGE_LOOP ( 'NONE', ( #17368, #19332, #9981, #28102 ) ) ;
#17495=CARTESIAN_POINT ( 'NONE',  ( 3.464101615137852974, 5.999999999999884537, -99.41367513459482552 ) ) ;
#17496=CARTESIAN_POINT ( 'NONE',  ( 0.000000000000000000, -5.999999999999991118, -61.96132486540523132 ) ) ;
#17498=CARTESIAN_POINT ( 'NONE',  ( 4.763139720814407951, 2.750000000000002665, -169.7500000000000000 ) ) ;
#17501=CARTESIAN_POINT ( 'NONE',  ( -5.412658773652739619, 3.124999999999975131, -172.6830127018922383 ) ) ;
#17504=CARTESIAN_POINT ( 'NONE',  ( 4.763139720814407951, -2.749999999999988454, -117.5000000000000426 ) ) ;
#17507=CARTESIAN_POINT ( 'NONE',  ( 4.763139720814407951, 2.750000000000002665, -102.2500000000000142 ) ) ;
#17508=DIRECTION ( 'NONE',  ( -7.147005652999508048E-36, 5.642372883946980038E-36, 1.000000000000000000 ) ) ;
#17510=CARTESIAN_POINT ( 'NONE',  ( -5.999999999999963585, 1.780251999655701777E-13, -82.41367513459481131 ) ) ;
#17515=ORIENTED_EDGE ( 'NONE', *, *, #13622, .T. ) ;
#17516=CARTESIAN_POINT ( 'NONE',  ( 4.763139720814407951, -2.749999999999988454, -159.5000000000000284 ) ) ;
#17517=EDGE_CURVE ( 'NONE', #22382, #7050, #17483, .T. ) ;
#17518=CARTESIAN_POINT ( 'NONE',  ( 5.412658773652739619, 3.124999999999988898, -79.31698729810781856 ) ) ;
#17519=CARTESIAN_POINT ( 'NONE',  ( -5.999999999999963585, -1.487416814333745711E-14, -97.41367513459481131 ) ) ;
#17520=ORIENTED_EDGE ( 'NONE', *, *, #27637, .T. ) ;
#17524=ORIENTED_EDGE ( 'NONE', *, *, #713, .F. ) ;
#17525=VERTEX_POINT ( 'NONE', #21324 ) ;
#17527=ADVANCED_FACE ( 'NONE', ( #5456 ), #9796, .T. ) ;
#17528=CARTESIAN_POINT ( 'NONE',  ( 5.412658773652712085, -3.125000000000086153, -137.4330127018922383 ) ) ;
#17529=ORIENTED_EDGE ( 'NONE', *, *, #5433, .F. ) ;
#17530=CARTESIAN_POINT ( 'NONE',  ( 7.216878364870455975, -6.409875621278545621E-14, -128.9419872981078186 ) ) ;
#17532=CARTESIAN_POINT ( 'NONE',  ( -2.775557561562891351E-14, -5.500000000000115463, -170.2500000000000000 ) ) ;
#17533=CARTESIAN_POINT ( 'NONE',  ( 5.196152422706629359, -2.999999999999988898, -167.2886751345948255 ) ) ;
#17538=CARTESIAN_POINT ( 'NONE',  ( -3.464101615137725076, 5.999999999999979572, -171.1636751345948255 ) ) ;
#17540=CARTESIAN_POINT ( 'NONE',  ( 5.412658773652739619, 3.124999999999988898, -71.81698729810781856 ) ) ;
#17541=CARTESIAN_POINT ( 'NONE',  ( 3.464101615137757051, -5.999999999999979572, -162.3363248654052313 ) ) ;
#17546=CARTESIAN_POINT ( 'NONE',  ( 3.175426480543072749, 5.499999999999865885, -126.1250000000000426 ) ) ;
#17547=CARTESIAN_POINT ( 'NONE',  ( 5.196152422706629359, 3.000000000000002665, -167.0386751345947971 ) ) ;
#17549=VERTEX_POINT ( 'NONE', #9949 ) ;
#17550=CARTESIAN_POINT ( 'NONE',  ( -3.464101615137725076, 5.999999999999979572, -132.1636751345948539 ) ) ;
#17552=CARTESIAN_POINT ( 'NONE',  ( -6.000000000000000888, 1.067854986875958443E-15, 7.560779664488942560E-35 ) ) ;
#17560=CARTESIAN_POINT ( 'NONE',  ( -3.608439182435052128, -6.250000000000110134, -94.94198729810780435 ) ) ;
#17561=CARTESIAN_POINT ( 'NONE',  ( -5.196152422706573404, -3.000000000000002665, -54.71132486540519579 ) ) ;
#17567=ADVANCED_FACE ( 'NONE', ( #267, #21922 ), #28954, .T. ) ;
#17568=CARTESIAN_POINT ( 'NONE',  ( -5.999999999999963585, -1.487416814333745711E-14, -80.91367513459482552 ) ) ;
#17569=CARTESIAN_POINT ( 'NONE',  ( 4.763139720814407951, 2.750000000000002665, -46.75000000000001421 ) ) ;
#17570=CARTESIAN_POINT ( 'NONE',  ( 6.000000000000052403, -1.607695154586662678, -62.23066243270258724 ) ) ;
#17571=CARTESIAN_POINT ( 'NONE',  ( 5.412658773652739619, 3.124999999999988898, -75.68301270189226670 ) ) ;
#17572=CARTESIAN_POINT ( 'NONE',  ( -5.999999999999963585, -1.487416814333745711E-14, -143.3363248654052029 ) ) ;
#17574=LINE ( 'NONE', #15272, #9917 ) ;
#17576=CARTESIAN_POINT ( 'NONE',  ( 0.000000000000000000, 0.000000000000000000, -44.99152654425658682 ) ) ;
#17577=CARTESIAN_POINT ( 'NONE',  ( -5.999999999999963585, 1.780251999655701777E-13, -79.41367513459482552 ) ) ;
#17578=CARTESIAN_POINT ( 'NONE',  ( 6.000000000000000888, 1.743066579297358182E-13, -113.1636751345948397 ) ) ;
#17580=CARTESIAN_POINT ( 'NONE',  ( 6.350852961086080661, -9.614813431917819062E-14, -129.3750000000000284 ) ) ;
#17582=CARTESIAN_POINT ( 'NONE',  ( -3.464101615137757051, -5.999999999999979572, -71.08632486540520290 ) ) ;
#17584=CARTESIAN_POINT ( 'NONE',  ( 6.350852961086080661, -9.614813431917819062E-14, -63.37500000000001421 ) ) ;
#17585=CARTESIAN_POINT ( 'NONE',  ( 4.763139720814407951, 2.750000000000002665, -55.75000000000002132 ) ) ;
#17586=AXIS2_PLACEMENT_3D ( 'NONE', #26273, #9713, #21691 ) ;
#17587=CARTESIAN_POINT ( 'NONE',  ( 5.196152422706629359, -2.999999999999988898, -174.2113248654052597 ) ) ;
#17588=VERTEX_POINT ( 'NONE', #20067 ) ;
#17590=CYLINDRICAL_SURFACE ( 'NONE', #25624, 6.000000000000000888 ) ;
#17593=CARTESIAN_POINT ( 'NONE',  ( -5.196152422706573404, -3.000000000000002665, -89.21132486540523132 ) ) ;
#17595=ORIENTED_EDGE ( 'NONE', *, *, #14496, .F. ) ;
#17599=EDGE_CURVE ( 'NONE', #10564, #5997, #30199, .T. ) ;
#17600=CARTESIAN_POINT ( 'NONE',  ( -4.763139720814407951, 2.749999999999946709, -143.7500000000000568 ) ) ;
#17601=CARTESIAN_POINT ( 'NONE',  ( 2.775557561562891351E-14, 6.250000000000033751, -49.06698729810782567 ) ) ;
#17604=CARTESIAN_POINT ( 'NONE',  ( 7.216878364870455975, -6.409875621278545621E-14, -143.9419872981078470 ) ) ;
#17605=CARTESIAN_POINT ( 'NONE',  ( 6.350852961086080661, -9.614813431917819062E-14, -76.87500000000000000 ) ) ;
#17607=CARTESIAN_POINT ( 'NONE',  ( 5.412658773652739619, 3.124999999999988898, -98.18301270189222407 ) ) ;
#17608=CARTESIAN_POINT ( 'NONE',  ( -4.763139720814407951, 2.749999999999946709, -152.7500000000000568 ) ) ;
#17609=CARTESIAN_POINT ( 'NONE',  ( 0.000000000000000000, 5.999999999999977796, -175.7886751345948539 ) ) ;
#17613=CARTESIAN_POINT ( 'NONE',  ( 3.175426480543072749, 5.499999999999865885, -154.6250000000000853 ) ) ;
#17615=CARTESIAN_POINT ( 'NONE',  ( -3.175426480542816510, -5.500000000000057732, -144.8750000000000853 ) ) ;
#17618=CARTESIAN_POINT ( 'NONE',  ( 3.175426480543072749, 5.499999999999865885, -88.62500000000001421 ) ) ;
#17619=CARTESIAN_POINT ( 'NONE',  ( 6.000000000000000888, -3.330669073875464691E-16, -7.560779664488942560E-35 ) ) ;
#17620=CARTESIAN_POINT ( 'NONE',  ( 4.763139720814407951, 2.750000000000002665, -84.25000000000004263 ) ) ;
#17623=CARTESIAN_POINT ( 'NONE',  ( 0.000000000000000000, 5.999999999999977796, -142.2113248654052313 ) ) ;
#17629=DIRECTION ( 'NONE',  ( -5.551115123125774074E-17, -1.000000000000000000, 5.642372883946979370E-36 ) ) ;
#17631=VERTEX_POINT ( 'NONE', #13340 ) ;
#17636=VERTEX_POINT ( 'NONE', #24661 ) ;
#17637=CARTESIAN_POINT ( 'NONE',  ( 0.000000000000000000, 5.499999999999991118, -109.5000000000000426 ) ) ;
#17639=CARTESIAN_POINT ( 'NONE',  ( 7.216878364870455975, -6.409875621278545621E-14, -117.8080127018922525 ) ) ;
#17641=CARTESIAN_POINT ( 'NONE',  ( 5.999999999999949374, 1.607695154586804565, -92.09668783648706381 ) ) ;
#17643=CARTESIAN_POINT ( 'NONE',  ( -3.608439182435115633, 6.249999999999965361, -49.80801270189224539 ) ) ;
#17646=LINE ( 'NONE', #17349, #28045 ) ;
#17649=CARTESIAN_POINT ( 'NONE',  ( 3.175426480543072749, -5.500000000000105693, -174.6250000000000284 ) ) ;
#17652=CARTESIAN_POINT ( 'NONE',  ( -5.412658773652739619, 3.124999999999975131, -166.6830127018922383 ) ) ;
#17653=CARTESIAN_POINT ( 'NONE',  ( -2.775557561562891351E-14, -5.500000000000115463, -114.7500000000000142 ) ) ;
#17655=CARTESIAN_POINT ( 'NONE',  ( -4.763139720814407951, 2.749999999999946709, -101.7500000000000000 ) ) ;
#17656=FACE_OUTER_BOUND ( 'NONE', #20308, .T. ) ;
#17657=CARTESIAN_POINT ( 'NONE',  ( -3.464101615137757051, -5.999999999999979572, -87.58632486540518869 ) ) ;
#17658=( NAMED_UNIT ( * ) SI_UNIT ( $, .STERADIAN. ) SOLID_ANGLE_UNIT ( ) );
#17660=ORIENTED_EDGE ( 'NONE', *, *, #10809, .F. ) ;
#17665=( BOUNDED_CURVE ( )  B_SPLINE_CURVE ( 2, ( #22754, #6450, #26867, #4141, #17865, #13406, #6152, #1695, #29491 ),
 .UNSPECIFIED., .F., .T. ) 
 B_SPLINE_CURVE_WITH_KNOTS ( ( 3, 2, 2, 2, 3 ),
 ( 0.5361111111111110938, 0.5370370370370369795, 0.5388888888888888618, 0.5407407407407407440, 0.5416666666666667407 ),
 .UNSPECIFIED. ) 
 CURVE ( )  GEOMETRIC_REPRESENTATION_ITEM ( )  RATIONAL_B_SPLINE_CURVE ( ( 0.9330127018922194093, 0.9330127018922194093, 1.000000000000000000, 0.8660254037844388186, 1.000000000000000000, 0.8660254037844388186, 1.000000000000000000, 0.9330127018922114157, 0.9330127018922194093 ) ) 
 REPRESENTATION_ITEM ( '' )  );
#17668=CARTESIAN_POINT ( 'NONE',  ( 4.763139720814407951, 2.750000000000002665, -159.2500000000000000 ) ) ;
#17669=CARTESIAN_POINT ( 'NONE',  ( 3.608439182435180470, 6.249999999999982236, -83.69198729810780435 ) ) ;
#17670=VECTOR ( 'NONE', #5926, 1000.000000000000000 ) ;
#17672=CARTESIAN_POINT ( 'NONE',  ( 0.000000000000000000, 0.000000000000000000, 0.000000000000000000 ) ) ;
#17673=STYLED_ITEM ( 'NONE', ( #20551 ), #14742 ) ;
#17676=ORIENTED_EDGE ( 'NONE', *, *, #12170, .F. ) ;
#17678=CARTESIAN_POINT ( 'NONE',  ( 0.000000000000000000, 5.499999999999991118, -133.5000000000000000 ) ) ;
#17679=CARTESIAN_POINT ( 'NONE',  ( -5.412658773652684552, -3.125000000000099920, -139.4330127018922383 ) ) ;
#17680=VERTEX_POINT ( 'NONE', #8383 ) ;
#17681=LINE ( 'NONE', #18136, #3114 ) ;
#17682=CARTESIAN_POINT ( 'NONE',  ( -5.412658773652739619, 3.124999999999975131, -122.3169872981078043 ) ) ;
#17683=CARTESIAN_POINT ( 'NONE',  ( 5.196152422706629359, -2.999999999999988898, -135.2113248654052029 ) ) ;
#17684=CARTESIAN_POINT ( 'NONE',  ( -6.350852961085760029, -1.281975124255709124E-13, -169.1249999999999716 ) ) ;
#17685=CARTESIAN_POINT ( 'NONE',  ( 5.196152422706629359, 3.000000000000002665, -83.96132486540520290 ) ) ;
#17686=CARTESIAN_POINT ( 'NONE',  ( -5.999999999999963585, 8.134310703387671600E-14, -130.4136751345948539 ) ) ;
#17689=CARTESIAN_POINT ( 'NONE',  ( -5.196152422706601826, 2.999999999999975131, -147.9613248654052597 ) ) ;
#17690=CARTESIAN_POINT ( 'NONE',  ( 6.000000000000000888, -1.859271017917181981E-14, -168.0863248654052313 ) ) ;
#17691=CARTESIAN_POINT ( 'NONE',  ( 6.000000000000000888, -1.859271017917181981E-14, -54.66367513459481842 ) ) ;
#17694=CARTESIAN_POINT ( 'NONE',  ( 3.608439182435180470, -6.249999999999997335, -64.69198729810784698 ) ) ;
#17695=CARTESIAN_POINT ( 'NONE',  ( -3.608439182435052128, -6.250000000000110134, -55.94198729810781145 ) ) ;
#17697=FACE_OUTER_BOUND ( 'NONE', #1353, .T. ) ;
#17700=CARTESIAN_POINT ( 'NONE',  ( 0.000000000000000000, 5.499999999999991118, -130.5000000000000000 ) ) ;
#17701=CARTESIAN_POINT ( 'NONE',  ( 6.000000000000000888, -1.859271017917181981E-14, -167.1636751345948539 ) ) ;
#17702=ORIENTED_EDGE ( 'NONE', *, *, #5061, .F. ) ;
#17705=CARTESIAN_POINT ( 'NONE',  ( 6.000000000000000888, 1.743066579297358182E-13, -49.58632486540520290 ) ) ;
#17708=ORIENTED_EDGE ( 'NONE', *, *, #22363, .F. ) ;
#17712=CARTESIAN_POINT ( 'NONE',  ( -5.412658773652739619, 3.124999999999975131, -114.8169872981078470 ) ) ;
#17713=CARTESIAN_POINT ( 'NONE',  ( -5.999999999999963585, 1.780251999655701777E-13, -110.3363248654052029 ) ) ;
#17716=CARTESIAN_POINT ( 'NONE',  ( -5.999999999999963585, -1.487416814333745711E-14, -55.41367513459483973 ) ) ;
#17718=AXIS2_PLACEMENT_3D ( 'NONE', #28556, #26263, #10153 ) ;
#17721=CARTESIAN_POINT ( 'NONE',  ( 4.763139720814407951, -2.749999999999988454, -51.49999999999999289 ) ) ;
#17723=CARTESIAN_POINT ( 'NONE',  ( -5.999999999999963585, 9.296355089585909904E-15, -164.9136751345948255 ) ) ;
#17724=CARTESIAN_POINT ( 'NONE',  ( 6.000000000000000888, 1.743066579297358182E-13, -60.66367513459481842 ) ) ;
#17725=CARTESIAN_POINT ( 'NONE',  ( 2.775557561562891351E-14, 6.250000000000033751, -78.43301270189223828 ) ) ;
#17726=CARTESIAN_POINT ( 'NONE',  ( 3.464101615137757051, -5.999999999999979572, -172.8363248654052029 ) ) ;
#17727=AXIS2_PLACEMENT_3D ( 'NONE', #19422, #24159, #21419 ) ;
#17729=CARTESIAN_POINT ( 'NONE',  ( 6.000000000000000888, 5.577813053751546416E-15, -177.6636751345948255 ) ) ;
#17730=DIRECTION ( 'NONE',  ( 1.000000000000000000, -5.551115123125773458E-17, -1.260129944081490338E-35 ) ) ;
#17731=ADVANCED_FACE ( 'NONE', ( #15493 ), #10404, .T. ) ;
#17732=CARTESIAN_POINT ( 'NONE',  ( 5.196152422706629359, 3.000000000000002665, -104.9613248654052171 ) ) ;
#17733=CARTESIAN_POINT ( 'NONE',  ( 0.000000000000000000, 5.499999999999991118, -133.5000000000000000 ) ) ;
#17735=DIRECTION ( 'NONE',  ( -7.147005652999508048E-36, 5.642372883946980038E-36, 1.000000000000000000 ) ) ;
#17736=ORIENTED_EDGE ( 'NONE', *, *, #19742, .F. ) ;
#17737=VECTOR ( 'NONE', #6348, 1000.000000000000000 ) ;
#17738=CARTESIAN_POINT ( 'NONE',  ( 4.763139720814407951, -2.749999999999988454, -63.50000000000000000 ) ) ;
#17739=CARTESIAN_POINT ( 'NONE',  ( -5.999999999999963585, 1.780251999655701777E-13, -72.83632486540523132 ) ) ;
#17740=EDGE_CURVE ( 'NONE', #1, #24992, #9218, .T. ) ;
#17741=CARTESIAN_POINT ( 'NONE',  ( -2.775557561562891351E-14, -5.500000000000115463, -54.75000000000002132 ) ) ;
#17745=DIRECTION ( 'NONE',  ( -7.147005652999508048E-36, 5.642372883946980038E-36, 1.000000000000000000 ) ) ;
#17747=DIRECTION ( 'NONE',  ( 1.000000000000000000, -5.551115123125773458E-17, -1.260129944081490338E-35 ) ) ;
#17752=ORIENTED_EDGE ( 'NONE', *, *, #29771, .F. ) ;
#17753=( BOUNDED_CURVE ( )  B_SPLINE_CURVE ( 2, ( #13800, #1768, #20365, #29716, #8851, #20834, #22984, #11332, #4371 ),
 .UNSPECIFIED., .F., .F. ) 
 B_SPLINE_CURVE_WITH_KNOTS ( ( 3, 2, 2, 2, 3 ),
 ( 0.4638888888888889062, 0.4648148148148147918, 0.4666666666666666741, 0.4685185185185185008, 0.4694444444444444420 ),
 .UNSPECIFIED. ) 
 CURVE ( )  GEOMETRIC_REPRESENTATION_ITEM ( )  RATIONAL_B_SPLINE_CURVE ( ( 0.9330127018922194093, 0.9330127018922214077, 1.000000000000000000, 0.8660254037844388186, 1.000000000000000000, 0.8660254037844388186, 1.000000000000000000, 0.9330127018922194093, 0.9330127018922194093 ) ) 
 REPRESENTATION_ITEM ( '' )  );
#17754=CARTESIAN_POINT ( 'NONE',  ( 4.763139720814407951, 2.750000000000002665, -142.7500000000000568 ) ) ;
#17757=CARTESIAN_POINT ( 'NONE',  ( -3.608439182435052128, -6.250000000000110134, -150.4419872981077901 ) ) ;
#17758=CARTESIAN_POINT ( 'NONE',  ( 6.350852961086080661, -9.614813431917819062E-14, -72.37499999999998579 ) ) ;
#17759=AXIS2_PLACEMENT_3D ( 'NONE', #16319, #23359, #2303 ) ;
#17761=CARTESIAN_POINT ( 'NONE',  ( -5.412658773652684552, -3.125000000000099920, -95.93301270189225249 ) ) ;
#17762=( BOUNDED_CURVE ( )  B_SPLINE_CURVE ( 2, ( #8115, #19376, #10607, #19961, #21969, #15065, #17685, #5659, #770 ),
 .UNSPECIFIED., .F., .F. ) 
 B_SPLINE_CURVE_WITH_KNOTS ( ( 3, 2, 2, 2, 3 ),
 ( 0.2750000000000000222, 0.2759259259259259078, 0.2777777777777777901, 0.2796296296296296724, 0.2805555555555555580 ),
 .UNSPECIFIED. ) 
 CURVE ( )  GEOMETRIC_REPRESENTATION_ITEM ( )  RATIONAL_B_SPLINE_CURVE ( ( 0.9330127018922194093, 0.9330127018922234061, 1.000000000000000000, 0.8660254037844388186, 1.000000000000000000, 0.8660254037844388186, 1.000000000000000000, 0.9330127018922194093, 0.9330127018922194093 ) ) 
 REPRESENTATION_ITEM ( '' )  );
#17763=CARTESIAN_POINT ( 'NONE',  ( -2.775557561562891351E-14, -5.500000000000115463, -152.2500000000000000 ) ) ;
#17764=CIRCLE ( 'NONE', #13864, 5.999999999999992006 ) ;
#17766=AXIS2_PLACEMENT_3D ( 'NONE', #17205, #15038, #17357 ) ;
#17767=EDGE_CURVE ( 'NONE', #18127, #8549, #12385, .T. ) ;
#17770=CARTESIAN_POINT ( 'NONE',  ( -5.196152422706573404, -3.000000000000002665, -86.78867513459486815 ) ) ;
#17771=FACE_OUTER_BOUND ( 'NONE', #15842, .T. ) ;
#17773=CARTESIAN_POINT ( 'NONE',  ( 6.350852961086080661, -9.614813431917819062E-14, -154.8749999999999716 ) ) ;
#17775=CARTESIAN_POINT ( 'NONE',  ( 3.175426480543072749, -5.500000000000105693, -149.1250000000000284 ) ) ;
#17776=CARTESIAN_POINT ( 'NONE',  ( -5.374111793511253232, 2.595803520898224637, -180.0000000000000284 ) ) ;
#17778=CARTESIAN_POINT ( 'NONE',  ( 3.175426480543072749, -5.500000000000105693, -89.12500000000001421 ) ) ;
#17781=CARTESIAN_POINT ( 'NONE',  ( 4.763139720814407951, -2.749999999999988454, -84.50000000000001421 ) ) ;
#17782=CARTESIAN_POINT ( 'NONE',  ( 5.999999999999949374, -1.607695154586841868, -120.1533121635130072 ) ) ;
#17784=CARTESIAN_POINT ( 'NONE',  ( -5.999999999999963585, 1.780251999655701777E-13, -64.41367513459483973 ) ) ;
#17787=CARTESIAN_POINT ( 'NONE',  ( -5.999999999999971578, 1.607695154586715303, -124.4806624327026014 ) ) ;
#17790=DIRECTION ( 'NONE',  ( -7.147005652999508048E-36, 5.642372883946980038E-36, 1.000000000000000000 ) ) ;
#17796=CARTESIAN_POINT ( 'NONE',  ( 3.175426480543072749, 5.499999999999865885, -96.12500000000004263 ) ) ;
#17798=CARTESIAN_POINT ( 'NONE',  ( 0.000000000000000000, 5.999999999999977796, -70.78867513459485394 ) ) ;
#17799=CARTESIAN_POINT ( 'NONE',  ( 3.608439182435180470, 6.249999999999982236, -111.5580127018922099 ) ) ;
#17800=ORIENTED_EDGE ( 'NONE', *, *, #22612, .T. ) ;
#17801=CARTESIAN_POINT ( 'NONE',  ( -3.464101615137725076, 5.999999999999979572, -94.08632486540524553 ) ) ;
#17803=CARTESIAN_POINT ( 'NONE',  ( 5.196152422706629359, 3.000000000000002665, -63.53867513459482552 ) ) ;
#17804=EDGE_CURVE ( 'NONE', #17588, #28274, #9179, .T. ) ;
#17805=CARTESIAN_POINT ( 'NONE',  ( 5.412658773652739619, 3.124999999999988898, -50.18301270189223828 ) ) ;
#17806=ORIENTED_EDGE ( 'NONE', *, *, #17010, .T. ) ;
#17808=CARTESIAN_POINT ( 'NONE',  ( -3.464101615137725076, 5.999999999999979572, -99.16367513459481131 ) ) ;
#17811=CARTESIAN_POINT ( 'NONE',  ( -6.350852961085760029, -1.281975124255709124E-13, -172.1250000000000284 ) ) ;
#17814=CARTESIAN_POINT ( 'NONE',  ( 3.608439182435180470, 6.249999999999982236, -158.0580127018922667 ) ) ;
#17816=CARTESIAN_POINT ( 'NONE',  ( -6.350852961085760029, -1.281975124255709124E-13, -106.1250000000000426 ) ) ;
#17817=DIRECTION ( 'NONE',  ( -7.147005652999508048E-36, 5.642372883946980038E-36, 1.000000000000000000 ) ) ;
#17818=CARTESIAN_POINT ( 'NONE',  ( -4.763139720814407951, 2.749999999999946709, -109.2500000000000142 ) ) ;
#17819=CARTESIAN_POINT ( 'NONE',  ( 0.000000000000000000, 5.999999999999977796, -151.7886751345948255 ) ) ;
#17820=CARTESIAN_POINT ( 'NONE',  ( 5.999999999999988454, 1.607695154586737729, -162.5966878364870638 ) ) ;
#17826=CARTESIAN_POINT ( 'NONE',  ( 3.464101615137757051, -5.999999999999979572, -133.8363248654052313 ) ) ;
#17827=ORIENTED_EDGE ( 'NONE', *, *, #4605, .T. ) ;
#17828=CARTESIAN_POINT ( 'NONE',  ( -4.763139720814407951, -2.750000000000016431, -160.0000000000000284 ) ) ;
#17829=CARTESIAN_POINT ( 'NONE',  ( -5.196152422706601826, 2.999999999999975131, -65.46132486540523132 ) ) ;
#17831=CARTESIAN_POINT ( 'NONE',  ( -3.608439182435052128, -6.250000000000110134, -81.44198729810780435 ) ) ;
#17834=CARTESIAN_POINT ( 'NONE',  ( 5.999999999999974243, 1.607695154586759934, -144.5966878364870354 ) ) ;
#17835=VECTOR ( 'NONE', #14057, 1000.000000000000000 ) ;
#17839=CARTESIAN_POINT ( 'NONE',  ( 3.175426480543072749, 5.499999999999865885, -120.1250000000000284 ) ) ;
#17840=CARTESIAN_POINT ( 'NONE',  ( -3.608439182435052128, -6.250000000000110134, -140.8080127018922383 ) ) ;
#17841=CARTESIAN_POINT ( 'NONE',  ( 5.999999999999988454, 1.607695154586737729, -161.0966878364870922 ) ) ;
#17842=CARTESIAN_POINT ( 'NONE',  ( 3.608439182435180470, -6.249999999999997335, -126.1919872981078328 ) ) ;
#17843=CARTESIAN_POINT ( 'NONE',  ( 6.350852961086080661, -9.614813431917819062E-14, -172.8750000000000284 ) ) ;
#17846=EDGE_CURVE ( 'NONE', #10564, #226, #11804, .T. ) ;
#17855=CARTESIAN_POINT ( 'NONE',  ( -3.608439182435052128, -6.250000000000110134, -64.94198729810784698 ) ) ;
#17856=CARTESIAN_POINT ( 'NONE',  ( 3.608439182435180470, 6.249999999999982236, -56.69198729810781145 ) ) ;
#17857=CARTESIAN_POINT ( 'NONE',  ( -5.999999999999963585, -1.487416814333745711E-14, -170.9136751345948255 ) ) ;
#17859=CARTESIAN_POINT ( 'NONE',  ( -3.464101615137725076, 5.999999999999979572, -74.58632486540520290 ) ) ;
#17861=CARTESIAN_POINT ( 'NONE',  ( -4.763139720814407951, -2.750000000000016431, -127.0000000000000000 ) ) ;
#17862=VECTOR ( 'NONE', #5381, 1000.000000000000000 ) ;
#17863=CARTESIAN_POINT ( 'NONE',  ( 6.000000000000000888, 1.743066579297358182E-13, -51.08632486540523132 ) ) ;
#17865=CARTESIAN_POINT ( 'NONE',  ( 0.000000000000000000, -5.999999999999991118, -118.9613248654052313 ) ) ;
#17866=CARTESIAN_POINT ( 'NONE',  ( 6.000000000000000888, -3.330669073875464691E-16, -7.560779664488942560E-35 ) ) ;
#17867=CARTESIAN_POINT ( 'NONE',  ( 0.000000000000000000, 0.000000000000000000, 0.000000000000000000 ) ) ;
#17871=CARTESIAN_POINT ( 'NONE',  ( -5.999999999999971578, 1.607695154586715303, -71.40331216351300725 ) ) ;
#17873=CARTESIAN_POINT ( 'NONE',  ( 2.775557561562891351E-14, 6.250000000000033751, -115.0669872981078186 ) ) ;
#17882=CLOSED_SHELL ( 'NONE', ( #28673, #2826, #12784, #306, #17321, #12648, #24241, #24624, #23966, #28405, #4213, #23456, #9321, #15854, #23251, #6418, #25826, #1186, #15165, #16088, #25148, #18992, #10238, #27563, #14353, #23623, #24214, #11075, #4963, #23762, #1644, #5208, #814, #21478, #26268, #28537, #7807, #19222, #29979, #17731, #11003, #19096, #11034, #12998, #26485, #10626, #6467, #25387, #30155, #29861, #25954, #2014, #3086, #11658, #28750, #19853, #25112, #29566, #3682, #869, #20252, #14433, #27057, #15096, #11186, #29447, #10663, #14012, #23418, #26757, #14153, #24242, #19928, #20564, #3265, #30365, #18814, #16839, #29908, #12470, #25223, #21130, #16123, #22181, #97, #495, #1316, #21128, #2790, #15638, #2932, #5932, #26496, #298, #23357, #1585, #24428, #21675, #4535, #27858, #2483, #12472, #6263, #21196, #14187, #28772, #1252, #3565, #21368, #27645, #14672, #16394, #15954, #29760, #26151, #12540, #26432, #25747, #20995, #20846, #13489, #650, #17011, #28068, #18059, #12514, #22047, #968, #9246, #8703, #6162, #29169, #1214, #21912, #14868, #28958, #754, #20141, #17452, #3610, #26033, #15716, #20373, #25080, #15675, #13515, #21088, #16935, #24489, #5106, #19917, #8484, #26728, #4631, #18501, #8291, #3332, #23595, #13735, #18714, #23929, #28601, #8379, #8977, #11976, #10370, #5683, #7744, #28413, #8624, #7704, #10837, #21464, #3124, #22263, #17527, #10228, #10544, #11799, #16339, #11322, #7904, #975, #4798, #11259, #20915, #21519, #20531, #17567, #18784, #11533, #10731, #26979, #27855, #15276, #231, #6041, #24597, #23253, #27344 ) ) ;
#17883=CARTESIAN_POINT ( 'NONE',  ( -4.763139720814407951, 2.749999999999946709, -149.7500000000000568 ) ) ;
#17884=CARTESIAN_POINT ( 'NONE',  ( 3.175426480543072749, 5.499999999999865885, -46.62500000000006395 ) ) ;
#17886=CARTESIAN_POINT ( 'NONE',  ( 7.216878364870455975, -6.409875621278545621E-14, -75.80801270189223828 ) ) ;
#17887=EDGE_CURVE ( 'NONE', #8975, #9651, #26325, .T. ) ;
#17888=CYLINDRICAL_SURFACE ( 'NONE', #4513, 6.000000000000000888 ) ;
#17890=DIRECTION ( 'NONE',  ( -7.147005652999508048E-36, 5.642372883946980038E-36, 1.000000000000000000 ) ) ;
#17891=FILL_AREA_STYLE_COLOUR ( '', #4954 ) ;
#17892=DIRECTION ( 'NONE',  ( -7.147005652999508048E-36, 5.642372883946980038E-36, 1.000000000000000000 ) ) ;
#17893=CARTESIAN_POINT ( 'NONE',  ( 4.763139720814407951, 2.750000000000002665, -129.2500000000000284 ) ) ;
#17894=CARTESIAN_POINT ( 'NONE',  ( 3.608439182435180470, -6.249999999999997335, -146.5580127018922383 ) ) ;
#17897=CARTESIAN_POINT ( 'NONE',  ( 3.175426480543072749, -5.500000000000105693, -66.62500000000002842 ) ) ;
#17900=VERTEX_POINT ( 'NONE', #21888 ) ;
#17903=CARTESIAN_POINT ( 'NONE',  ( -3.464101615137757051, -5.999999999999979572, -118.1636751345948397 ) ) ;
#17910=ORIENTED_EDGE ( 'NONE', *, *, #16445, .T. ) ;
#17912=CARTESIAN_POINT ( 'NONE',  ( -3.175426480542816510, 5.499999999999865885, -148.3750000000000568 ) ) ;
#17914=VERTEX_POINT ( 'NONE', #2536 ) ;
#17916=ORIENTED_EDGE ( 'NONE', *, *, #27844, .F. ) ;
#17917=CARTESIAN_POINT ( 'NONE',  ( -4.763139720814407951, 2.749999999999946709, -71.75000000000004263 ) ) ;
#17919=CARTESIAN_POINT ( 'NONE',  ( 3.608439182435180470, 6.249999999999982236, -96.55801270189228092 ) ) ;
#17920=CARTESIAN_POINT ( 'NONE',  ( -4.520452470708151260, -10.03252783106556123, -21.03609891486514627 ) ) ;
#17921=CARTESIAN_POINT ( 'NONE',  ( 5.196152422706629359, -2.999999999999988898, -83.28867513459481131 ) ) ;
#17923=VECTOR ( 'NONE', #6064, 1000.000000000000000 ) ;
#17926=CARTESIAN_POINT ( 'NONE',  ( 4.763139720814407951, 2.750000000000002665, -157.7500000000000568 ) ) ;
#17928=PLANE ( 'NONE',  #13014 ) ;
#17929=CARTESIAN_POINT ( 'NONE',  ( 4.763139720814407951, -2.749999999999988454, -89.00000000000002842 ) ) ;
#17930=CARTESIAN_POINT ( 'NONE',  ( 6.000000000000000888, -3.330669073875464691E-16, -7.560779664488942560E-35 ) ) ;
#17931=CARTESIAN_POINT ( 'NONE',  ( -4.763139720814407951, 2.749999999999946709, -73.25000000000004263 ) ) ;
#17937=DIRECTION ( 'NONE',  ( -7.147005652999508048E-36, 5.642372883946980038E-36, 1.000000000000000000 ) ) ;
#17939=CARTESIAN_POINT ( 'NONE',  ( 10.00000000000001421, -5.551115123125781716E-16, -43.99152654425658682 ) ) ;
#17941=ORIENTED_EDGE ( 'NONE', *, *, #23781, .T. ) ;
#17943=CARTESIAN_POINT ( 'NONE',  ( 0.000000000000000000, 5.999999999999977796, -73.21132486540521711 ) ) ;
#17948=( BOUNDED_CURVE ( )  B_SPLINE_CURVE ( 2, ( #9685, #155, #28839, #7369, #7798, #2744, #5492, #9985, #19361 ),
 .UNSPECIFIED., .F., .F. ) 
 B_SPLINE_CURVE_WITH_KNOTS ( ( 3, 2, 2, 2, 3 ),
 ( 0.09722222222222222376, 0.09814814814814815103, 0.1000000000000000056, 0.1018518518518518462, 0.1027777777777777735 ),
 .UNSPECIFIED. ) 
 CURVE ( )  GEOMETRIC_REPRESENTATION_ITEM ( )  RATIONAL_B_SPLINE_CURVE ( ( 0.9330127018922194093, 0.9330127018922194093, 1.000000000000000000, 0.8660254037844388186, 1.000000000000000000, 0.8660254037844388186, 1.000000000000000000, 0.9330127018922194093, 0.9330127018922194093 ) ) 
 REPRESENTATION_ITEM ( '' )  );
#17950=ORIENTED_EDGE ( 'NONE', *, *, #27676, .T. ) ;
#17951=CARTESIAN_POINT ( 'NONE',  ( -6.350852961085760029, -1.281975124255709124E-13, -98.62500000000005684 ) ) ;
#17952=CARTESIAN_POINT ( 'NONE',  ( -5.999999999999963585, 9.296355089585909904E-15, -169.4136751345948539 ) ) ;
#17953=EDGE_CURVE ( 'NONE', #21789, #15083, #28919, .T. ) ;
#17954=CARTESIAN_POINT ( 'NONE',  ( 3.608439182435180470, 6.249999999999982236, -117.5580127018922383 ) ) ;
#17958=CARTESIAN_POINT ( 'NONE',  ( -5.999999999999956479, -1.607695154586745057, -143.8466878364870354 ) ) ;
#17960=CARTESIAN_POINT ( 'NONE',  ( 7.216878364870455975, -6.409875621278545621E-14, -50.30801270189225249 ) ) ;
#17961=ORIENTED_EDGE ( 'NONE', *, *, #24664, .T. ) ;
#17962=CARTESIAN_POINT ( 'NONE',  ( 6.000000000000000888, 1.743066579297358182E-13, -61.58632486540521001 ) ) ;
#17963=CARTESIAN_POINT ( 'NONE',  ( 6.350852961086080661, -9.614813431917819062E-14, -160.8750000000000284 ) ) ;
#17966=CARTESIAN_POINT ( 'NONE',  ( 6.350852961086080661, -9.614813431917819062E-14, -106.8750000000000426 ) ) ;
#17968=CARTESIAN_POINT ( 'NONE',  ( -3.175426480542816510, 5.499999999999865885, -103.3750000000000142 ) ) ;
#17971=CARTESIAN_POINT ( 'NONE',  ( -5.999999999999866773, 1.607695154586893826, -144.9033121635130215 ) ) ;
#17972=ORIENTED_EDGE ( 'NONE', *, *, #22431, .T. ) ;
#17977=ORIENTED_EDGE ( 'NONE', *, *, #5976, .T. ) ;
#17979=CARTESIAN_POINT ( 'NONE',  ( -5.412658773652739619, 3.124999999999975131, -90.81698729810783277 ) ) ;
#17981=CARTESIAN_POINT ( 'NONE',  ( -6.000000000000007105, -1.607695154586655129, -129.7693375672974128 ) ) ;
#17982=ORIENTED_EDGE ( 'NONE', *, *, #28511, .F. ) ;
#17983=CARTESIAN_POINT ( 'NONE',  ( 6.000000000000000000, 2.951592740943527306E-14, -157.5863248654052313 ) ) ;
#17984=CARTESIAN_POINT ( 'NONE',  ( -3.175426480542816510, 5.499999999999865885, -151.3749999999999716 ) ) ;
#17985=VERTEX_POINT ( 'NONE', #13162 ) ;
#17986=ORIENTED_EDGE ( 'NONE', *, *, #8741, .F. ) ;
#17988=CARTESIAN_POINT ( 'NONE',  ( -3.175426480542816510, 5.499999999999865885, -124.3749999999999858 ) ) ;
#17989=EDGE_CURVE ( 'NONE', #16735, #91, #30013, .T. ) ;
#17990=CARTESIAN_POINT ( 'NONE',  ( -5.412658773652739619, 3.124999999999975131, -141.1830127018922667 ) ) ;
#17991=ORIENTED_EDGE ( 'NONE', *, *, #15316, .F. ) ;
#17992=CARTESIAN_POINT ( 'NONE',  ( 6.000000000000000888, 1.743066579297358182E-13, -57.08632486540521001 ) ) ;
#17993=CARTESIAN_POINT ( 'NONE',  ( 7.216878364870455975, -6.409875621278545621E-14, -127.4419872981078328 ) ) ;
#17994=CARTESIAN_POINT ( 'NONE',  ( 3.608439182435180470, 6.249999999999982236, -175.1919872981077901 ) ) ;
#17995=CARTESIAN_POINT ( 'NONE',  ( 4.763139720814407951, 2.750000000000002665, -174.2500000000000284 ) ) ;
#17996=CARTESIAN_POINT ( 'NONE',  ( 6.000000000000000888, 7.762456499804235646E-14, -122.1636751345948397 ) ) ;
#17997=LINE ( 'NONE', #8116, #1496 ) ;
#17998=( BOUNDED_CURVE ( )  B_SPLINE_CURVE ( 2, ( #11604, #9724, #6947, #7098, #28279, #14214, #28574, #14505, #7405 ),
 .UNSPECIFIED., .F., .T. ) 
 B_SPLINE_CURVE_WITH_KNOTS ( ( 3, 2, 2, 2, 3 ),
 ( 0.2416666666666666963, 0.2425925925925925819, 0.2444444444444444642, 0.2462962962962963465, 0.2472222222222222321 ),
 .UNSPECIFIED. ) 
 CURVE ( )  GEOMETRIC_REPRESENTATION_ITEM ( )  RATIONAL_B_SPLINE_CURVE ( ( 0.9330127018922194093, 0.9330127018922234061, 1.000000000000000000, 0.8660254037844388186, 1.000000000000000000, 0.8660254037844388186, 1.000000000000000000, 0.9330127018922194093, 0.9330127018922194093 ) ) 
 REPRESENTATION_ITEM ( '' )  );
#18001=CYLINDRICAL_SURFACE ( 'NONE', #14260, 6.000000000000000888 ) ;
#18004=CARTESIAN_POINT ( 'NONE',  ( 5.196152422706629359, 3.000000000000002665, -46.46132486540521711 ) ) ;
#18006=CARTESIAN_POINT ( 'NONE',  ( 3.608439182435180470, 6.249999999999982236, -70.19198729810780435 ) ) ;
#18007=VECTOR ( 'NONE', #16439, 1000.000000000000000 ) ;
#18008=CARTESIAN_POINT ( 'NONE',  ( -3.608439182435052128, -6.250000000000110134, -54.44198729810779724 ) ) ;
#18010=CARTESIAN_POINT ( 'NONE',  ( -4.763139720814407951, -2.750000000000016431, -50.49999999999998579 ) ) ;
#18012=DIRECTION ( 'NONE',  ( -7.147005652999508048E-36, 5.642372883946980038E-36, 1.000000000000000000 ) ) ;
#18013=CARTESIAN_POINT ( 'NONE',  ( 6.350852961086080661, -9.614813431917819062E-14, -130.8750000000000284 ) ) ;
#18017=VERTEX_POINT ( 'NONE', #10367 ) ;
#18025=CARTESIAN_POINT ( 'NONE',  ( 7.216878364870455975, -6.409875621278545621E-14, -112.4419872981078186 ) ) ;
#18028=EDGE_CURVE ( 'NONE', #15617, #29147, #20650, .T. ) ;
#18030=ORIENTED_EDGE ( 'NONE', *, *, #24347, .F. ) ;
#18035=CARTESIAN_POINT ( 'NONE',  ( -4.763139720814407951, -2.750000000000016431, -49.00000000000004263 ) ) ;
#18038=CARTESIAN_POINT ( 'NONE',  ( -3.608439182435052128, -6.250000000000110134, -67.30801270189226670 ) ) ;
#18041=CARTESIAN_POINT ( 'NONE',  ( 3.464101615137757051, -5.999999999999979572, -177.9136751345948255 ) ) ;
#18043=CARTESIAN_POINT ( 'NONE',  ( -5.999999999999956479, -1.607695154586745057, -67.34668783648702117 ) ) ;
#18045=CARTESIAN_POINT ( 'NONE',  ( 3.175426480543072749, -5.500000000000105693, -135.6250000000000284 ) ) ;
#18046=AXIS2_PLACEMENT_3D ( 'NONE', #4649, #18663, #4502 ) ;
#18047=CARTESIAN_POINT ( 'NONE',  ( 7.216878364870455975, -6.409875621278545621E-14, -147.8080127018922667 ) ) ;
#18050=CARTESIAN_POINT ( 'NONE',  ( -6.350852961085760029, -1.281975124255709124E-13, -62.62500000000001421 ) ) ;
#18059=ADVANCED_FACE ( 'NONE', ( #16077 ), #9269, .T. ) ;
#18062=CARTESIAN_POINT ( 'NONE',  ( -5.999999999999963585, 1.780251999655701777E-13, -103.4136751345948255 ) ) ;
#18063=VERTEX_POINT ( 'NONE', #23267 ) ;
#18064=CARTESIAN_POINT ( 'NONE',  ( 4.763139720814407951, 2.750000000000002665, -147.2500000000000000 ) ) ;
#18067=VERTEX_POINT ( 'NONE', #18206 ) ;
#18068=CARTESIAN_POINT ( 'NONE',  ( 3.175426480543072749, -5.500000000000105693, -71.12500000000004263 ) ) ;
#18070=CARTESIAN_POINT ( 'NONE',  ( -3.977757852569110852, -10.25981801084819445, -29.50831862515141424 ) ) ;
#18072=CARTESIAN_POINT ( 'NONE',  ( -5.999999999999919176, 1.607695154586804565, -98.40331216351297883 ) ) ;
#18073=CARTESIAN_POINT ( 'NONE',  ( 6.000000000000052403, -1.607695154586662678, -64.65331216351297883 ) ) ;
#18076=CARTESIAN_POINT ( 'NONE',  ( 6.350852961086080661, -9.614813431917819062E-14, -159.3750000000000284 ) ) ;
#18077=DIRECTION ( 'NONE',  ( -7.147005652999508048E-36, 5.642372883946980038E-36, 1.000000000000000000 ) ) ;
#18078=CARTESIAN_POINT ( 'NONE',  ( -3.464101615137725076, 5.999999999999979572, -49.08632486540521711 ) ) ;
#18080=CARTESIAN_POINT ( 'NONE',  ( -3.175426480542816066, -5.500000000000057732, -89.37500000000001421 ) ) ;
#18082=CARTESIAN_POINT ( 'NONE',  ( -3.175426480542816510, -5.500000000000057732, -77.37500000000001421 ) ) ;
#18084=CARTESIAN_POINT ( 'NONE',  ( 3.464101615137852974, 5.999999999999884537, -142.3363248654052029 ) ) ;
#18087=CARTESIAN_POINT ( 'NONE',  ( 0.000000000000000000, 5.999999999999977796, -103.7886751345948255 ) ) ;
#18089=CARTESIAN_POINT ( 'NONE',  ( 0.000000000000000000, 0.000000000000000000, 0.000000000000000000 ) ) ;
#18091=ORIENTED_EDGE ( 'NONE', *, *, #22997, .T. ) ;
#18095=CARTESIAN_POINT ( 'NONE',  ( -6.000000000000000888, 1.067854986875958443E-15, 7.560779664488942560E-35 ) ) ;
#18097=CARTESIAN_POINT ( 'NONE',  ( 4.763139720814407951, 2.750000000000002665, -96.25000000000000000 ) ) ;
#18099=CARTESIAN_POINT ( 'NONE',  ( -3.608439182435115633, 6.249999999999965361, -112.8080127018922241 ) ) ;
#18100=ORIENTED_EDGE ( 'NONE', *, *, #14087, .T. ) ;
#18103=CARTESIAN_POINT ( 'NONE',  ( 3.608439182435180470, 6.249999999999982236, -53.05801270189219565 ) ) ;
#18104=EDGE_LOOP ( 'NONE', ( #9004, #17529, #24410, #29985 ) ) ;
#18106=CARTESIAN_POINT ( 'NONE',  ( 6.000000000000052403, 1.607695154586625819, -136.5193375672973559 ) ) ;
#18107=CARTESIAN_POINT ( 'NONE',  ( -3.175426480542816510, 5.499999999999865885, -163.3750000000000568 ) ) ;
#18110=CARTESIAN_POINT ( 'NONE',  ( -2.775557561562891351E-14, -5.500000000000115463, -107.2500000000000142 ) ) ;
#18112=CARTESIAN_POINT ( 'NONE',  ( 6.000000000000000888, 7.762456499804235646E-14, -123.6636751345948255 ) ) ;
#18113=( BOUNDED_CURVE ( )  B_SPLINE_CURVE ( 2, ( #15166, #1621, #20063, #19754, #6371, #22530, #26951, #29099, #10872 ),
 .UNSPECIFIED., .F., .T. ) 
 B_SPLINE_CURVE_WITH_KNOTS ( ( 3, 2, 2, 2, 3 ),
 ( 0.7861111111111112049, 0.7870370370370370905, 0.7888888888888888618, 0.7907407407407407440, 0.7916666666666666297 ),
 .UNSPECIFIED. ) 
 CURVE ( )  GEOMETRIC_REPRESENTATION_ITEM ( )  RATIONAL_B_SPLINE_CURVE ( ( 0.9330127018922194093, 0.9330127018922234061, 1.000000000000000000, 0.8660254037844388186, 1.000000000000000000, 0.8660254037844388186, 1.000000000000000000, 0.9330127018922234061, 0.9330127018922194093 ) ) 
 REPRESENTATION_ITEM ( '' )  );
#18114=CARTESIAN_POINT ( 'NONE',  ( -4.763139720814407951, 2.749999999999946709, -95.75000000000000000 ) ) ;
#18115=CARTESIAN_POINT ( 'NONE',  ( 5.999999999999999112, 2.951592740943527306E-14, -162.6636751345948824 ) ) ;
#18121=DIRECTION ( 'NONE',  ( -7.147005652999508048E-36, 5.642372883946980038E-36, 1.000000000000000000 ) ) ;
#18125=CARTESIAN_POINT ( 'NONE',  ( 2.775557561562891351E-14, 6.250000000000033751, -91.06698729810780435 ) ) ;
#18126=CARTESIAN_POINT ( 'NONE',  ( 3.464101615137757051, -5.999999999999979572, -96.91367513459481131 ) ) ;
#18127=VERTEX_POINT ( 'NONE', #25077 ) ;
#18128=CARTESIAN_POINT ( 'NONE',  ( -4.758024543289570474, 9.918640242984139377, -28.66037974350895112 ) ) ;
#18129=ORIENTED_EDGE ( 'NONE', *, *, #15845, .T. ) ;
#18132=CARTESIAN_POINT ( 'NONE',  ( -4.763139720814407951, 2.749999999999946709, -122.7500000000000284 ) ) ;
#18134=CARTESIAN_POINT ( 'NONE',  ( 5.412658773652739619, 3.124999999999988898, -140.1830127018922667 ) ) ;
#18135=ORIENTED_EDGE ( 'NONE', *, *, #14546, .F. ) ;
#18136=CARTESIAN_POINT ( 'NONE',  ( 6.000000000000000888, -3.330669073875464691E-16, -7.560779664488942560E-35 ) ) ;
#18138=CARTESIAN_POINT ( 'NONE',  ( -5.412658773652684552, -3.125000000000099920, -120.5669872981078328 ) ) ;
#18139=CARTESIAN_POINT ( 'NONE',  ( 5.412658773652712085, -3.125000000000086153, -174.0669872981078186 ) ) ;
#18140=CARTESIAN_POINT ( 'NONE',  ( -3.175426480542816510, -5.500000000000057732, -171.8750000000000284 ) ) ;
#18142=DIRECTION ( 'NONE',  ( -7.147005652999508048E-36, 5.642372883946980038E-36, 1.000000000000000000 ) ) ;
#18143=ORIENTED_EDGE ( 'NONE', *, *, #8844, .F. ) ;
#18146=CARTESIAN_POINT ( 'NONE',  ( 5.196152422706629359, 3.000000000000002665, -171.5386751345948539 ) ) ;
#18149=CARTESIAN_POINT ( 'NONE',  ( -5.412658773652684552, -3.125000000000099920, -75.56698729810784698 ) ) ;
#18150=CARTESIAN_POINT ( 'NONE',  ( -7.216878364870328078, 0.000000000000000000, -62.19198729810784698 ) ) ;
#18151=CARTESIAN_POINT ( 'NONE',  ( -5.999999999999956479, -1.607695154586745057, -170.8466878364870638 ) ) ;
#18152=CARTESIAN_POINT ( 'NONE',  ( -6.350852961085760029, -1.281975124255709124E-13, -50.62500000000001421 ) ) ;
#18154=EDGE_CURVE ( 'NONE', #16860, #28335, #8971, .T. ) ;
#18156=CARTESIAN_POINT ( 'NONE',  ( 3.175426480543072749, -5.500000000000105693, -120.6250000000000284 ) ) ;
#18157=CARTESIAN_POINT ( 'NONE',  ( -5.999999999999963585, -1.487416814333745711E-14, -80.91367513459482552 ) ) ;
#18159=CARTESIAN_POINT ( 'NONE',  ( -5.999999999999957367, 1.607695154586737507, -157.4806624327026157 ) ) ;
#18161=DIRECTION ( 'NONE',  ( 1.000000000000000000, -5.551115123125774690E-17, 0.000000000000000000 ) ) ;
#18164=DIRECTION ( 'NONE',  ( -7.147005652999508048E-36, 5.642372883946980038E-36, 1.000000000000000000 ) ) ;
#18165=VECTOR ( 'NONE', #16254, 1000.000000000000000 ) ;
#18169=DIRECTION ( 'NONE',  ( -7.147005652999508048E-36, 5.642372883946980038E-36, 1.000000000000000000 ) ) ;
#18171=CARTESIAN_POINT ( 'NONE',  ( -3.608439182435115633, 6.249999999999965361, -117.9419872981078470 ) ) ;
#18173=ORIENTED_EDGE ( 'NONE', *, *, #1753, .F. ) ;
#18174=VERTEX_POINT ( 'NONE', #18062 ) ;
#18177=ORIENTED_EDGE ( 'NONE', *, *, #716, .F. ) ;
#18178=VERTEX_POINT ( 'NONE', #14080 ) ;
#18179=CARTESIAN_POINT ( 'NONE',  ( 4.763139720814407951, 2.750000000000002665, -51.25000000000001421 ) ) ;
#18182=CYLINDRICAL_SURFACE ( 'NONE', #474, 6.000000000000000888 ) ;
#18183=CARTESIAN_POINT ( 'NONE',  ( -3.608439182435052128, -6.250000000000110134, -68.80801270189220986 ) ) ;
#18185=CARTESIAN_POINT ( 'NONE',  ( 0.000000000000000000, 5.499999999999991118, -180.0000000000000568 ) ) ;
#18186=FACE_OUTER_BOUND ( 'NONE', #24546, .T. ) ;
#18187=CARTESIAN_POINT ( 'NONE',  ( -5.999999999999962697, 3.323446944526963891E-14, -155.9136751345948255 ) ) ;
#18193=CARTESIAN_POINT ( 'NONE',  ( -2.775557561562891351E-14, -5.500000000000115463, -122.2500000000000284 ) ) ;
#18195=ORIENTED_EDGE ( 'NONE', *, *, #13697, .F. ) ;
#18196=CARTESIAN_POINT ( 'NONE',  ( -4.763139720814407951, 2.749999999999946709, -65.75000000000002842 ) ) ;
#18197=CARTESIAN_POINT ( 'NONE',  ( 0.000000000000000000, -5.999999999999991118, -154.0386751345948539 ) ) ;
#18199=CARTESIAN_POINT ( 'NONE',  ( 6.000000000000052403, 1.607695154586625819, -171.0193375672974128 ) ) ;
#18206=CARTESIAN_POINT ( 'NONE',  ( 6.000000000000000888, 1.743066579297358182E-13, -92.16367513459482552 ) ) ;
#18207=ORIENTED_EDGE ( 'NONE', *, *, #4726, .T. ) ;
#18208=CARTESIAN_POINT ( 'NONE',  ( 4.763139720814407951, 2.750000000000002665, -138.2499999999999716 ) ) ;
#18212=VERTEX_POINT ( 'NONE', #14638 ) ;
#18213=CARTESIAN_POINT ( 'NONE',  ( 0.000000000000000000, 5.499999999999991118, -75.00000000000001421 ) ) ;
#18217=CARTESIAN_POINT ( 'NONE',  ( -5.999999999999963585, 1.780251999655701777E-13, -83.91367513459482552 ) ) ;
#18222=EDGE_CURVE ( 'NONE', #17636, #7780, #9667, .T. ) ;
#18223=CARTESIAN_POINT ( 'NONE',  ( -2.775557561562891351E-14, -5.500000000000115463, -144.7500000000000568 ) ) ;
#18226=CARTESIAN_POINT ( 'NONE',  ( 0.000000000000000000, 5.499999999999991118, -87.00000000000002842 ) ) ;
#18227=CARTESIAN_POINT ( 'NONE',  ( 0.000000000000000000, 0.000000000000000000, 0.000000000000000000 ) ) ;
#18228=CARTESIAN_POINT ( 'NONE',  ( -3.175426480542816510, -5.500000000000057732, -69.87500000000005684 ) ) ;
#18229=DIRECTION ( 'NONE',  ( -7.147005652999508048E-36, 5.642372883946980038E-36, 1.000000000000000000 ) ) ;
#18231=CARTESIAN_POINT ( 'NONE',  ( -5.999999999999962697, 3.323446944526963891E-14, -149.3363248654052313 ) ) ;
#18234=CARTESIAN_POINT ( 'NONE',  ( 5.999999999999949374, 1.607695154586804565, -55.51933756729742697 ) ) ;
#18236=CARTESIAN_POINT ( 'NONE',  ( -5.999999999999963585, 1.607695154586726627, -169.4806624327026157 ) ) ;
#18237=EDGE_LOOP ( 'NONE', ( #5576, #21631, #27028, #28723 ) ) ;
#18241=CARTESIAN_POINT ( 'NONE',  ( 5.999999999999999112, 2.951592740943527306E-14, -157.5863248654052313 ) ) ;
#18242=ORIENTED_EDGE ( 'NONE', *, *, #2958, .T. ) ;
#18243=ORIENTED_EDGE ( 'NONE', *, *, #25965, .T. ) ;
#18244=VECTOR ( 'NONE', #27144, 1000.000000000000000 ) ;
#18245=EDGE_LOOP ( 'NONE', ( #27715, #17039, #17003, #11841 ) ) ;
#18247=CARTESIAN_POINT ( 'NONE',  ( 6.350852961086080661, -9.614813431917819062E-14, -100.8750000000000000 ) ) ;
#18248=DIRECTION ( 'NONE',  ( -7.147005652999508048E-36, 5.642372883946980038E-36, 1.000000000000000000 ) ) ;
#18249=CARTESIAN_POINT ( 'NONE',  ( 2.775557561562891351E-14, 6.250000000000033751, -106.9330127018922667 ) ) ;
#18250=VERTEX_POINT ( 'NONE', #8604 ) ;
#18252=AXIS2_PLACEMENT_3D ( 'NONE', #11094, #29947, #6762 ) ;
#18254=CARTESIAN_POINT ( 'NONE',  ( -6.350852961085760029, -1.281975124255709124E-13, -164.6249999999999716 ) ) ;
#18255=( BOUNDED_CURVE ( )  B_SPLINE_CURVE ( 2, ( #9482, #6708, #2693, #4554, #9626, #2549, #21456, #4697, #243 ),
 .UNSPECIFIED., .F., .F. ) 
 B_SPLINE_CURVE_WITH_KNOTS ( ( 3, 2, 2, 2, 3 ),
 ( 0.1583333333333333259, 0.1592592592592592116, 0.1611111111111110938, 0.1629629629629629761, 0.1638888888888889728 ),
 .UNSPECIFIED. ) 
 CURVE ( )  GEOMETRIC_REPRESENTATION_ITEM ( )  RATIONAL_B_SPLINE_CURVE ( ( 0.9330127018922194093, 0.9330127018922194093, 1.000000000000000000, 0.8660254037844388186, 1.000000000000000000, 0.8660254037844388186, 1.000000000000000000, 0.9330127018922154125, 0.9330127018922194093 ) ) 
 REPRESENTATION_ITEM ( '' )  );
#18258=CARTESIAN_POINT ( 'NONE',  ( 6.000000000000000888, -1.859271017917181981E-14, -145.5863248654052029 ) ) ;
#18259=DIRECTION ( 'NONE',  ( 1.000000000000000000, 0.000000000000000000, 0.000000000000000000 ) ) ;
#18263=CARTESIAN_POINT ( 'NONE',  ( 6.350852961086080661, -9.614813431917819062E-14, -165.3750000000000284 ) ) ;
#18265=CARTESIAN_POINT ( 'NONE',  ( -2.775557561562891351E-14, -5.500000000000115463, -111.7500000000000142 ) ) ;
#18267=DIRECTION ( 'NONE',  ( -7.147005652999508048E-36, 5.642372883946980038E-36, 1.000000000000000000 ) ) ;
#18268=CARTESIAN_POINT ( 'NONE',  ( 0.000000000000000000, 5.499999999999991118, -96.00000000000002842 ) ) ;
#18270=CARTESIAN_POINT ( 'NONE',  ( -5.999999999999962697, 3.323446944526963891E-14, -150.8363248654052029 ) ) ;
#18272=ORIENTED_EDGE ( 'NONE', *, *, #11513, .F. ) ;
#18277=ORIENTED_EDGE ( 'NONE', *, *, #26186, .T. ) ;
#18278=CARTESIAN_POINT ( 'NONE',  ( -5.999999999999904965, -1.607695154586834541, -170.2693375672974128 ) ) ;
#18281=CARTESIAN_POINT ( 'NONE',  ( -3.608439182435115633, 6.249999999999965361, -87.94198729810783277 ) ) ;
#18283=ORIENTED_EDGE ( 'NONE', *, *, #12685, .T. ) ;
#18284=CARTESIAN_POINT ( 'NONE',  ( 2.775557561562891351E-14, 10.99999999999998224, -31.00000000000002842 ) ) ;
#18285=ORIENTED_EDGE ( 'NONE', *, *, #17740, .F. ) ;
#18286=ORIENTED_EDGE ( 'NONE', *, *, #12812, .F. ) ;
#18289=CARTESIAN_POINT ( 'NONE',  ( 3.175426480543072749, -5.500000000000105693, -117.6250000000000284 ) ) ;
#18290=CARTESIAN_POINT ( 'NONE',  ( 3.608439182435180470, -6.249999999999997335, -134.5580127018922951 ) ) ;
#18292=CARTESIAN_POINT ( 'NONE',  ( -3.464101615137757051, -5.999999999999979572, -57.58632486540518869 ) ) ;
#18293=CARTESIAN_POINT ( 'NONE',  ( -3.608439182435052128, -6.250000000000110134, -120.4419872981077901 ) ) ;
#18294=CARTESIAN_POINT ( 'NONE',  ( 7.216878364870455975, -6.409875621278545621E-14, -175.4419872981078470 ) ) ;
#18297=ORIENTED_EDGE ( 'NONE', *, *, #19829, .T. ) ;
#18300=CARTESIAN_POINT ( 'NONE',  ( -5.999999999999963585, -1.487416814333745711E-14, -75.83632486540521711 ) ) ;
#18301=( BOUNDED_CURVE ( )  B_SPLINE_CURVE ( 2, ( #25562, #7429, #12085, #14393, #2662, #16837, #11784, #19126, #23290 ),
 .UNSPECIFIED., .F., .T. ) 
 B_SPLINE_CURVE_WITH_KNOTS ( ( 3, 2, 2, 2, 3 ),
 ( 0.5194444444444444864, 0.5203703703703703720, 0.5222222222222221433, 0.5240740740740741366, 0.5249999999999999112 ),
 .UNSPECIFIED. ) 
 CURVE ( )  GEOMETRIC_REPRESENTATION_ITEM ( )  RATIONAL_B_SPLINE_CURVE ( ( 0.9330127018922194093, 0.9330127018922194093, 1.000000000000000000, 0.8660254037844388186, 1.000000000000000000, 0.8660254037844388186, 1.000000000000000000, 0.9330127018922274029, 0.9330127018922194093 ) ) 
 REPRESENTATION_ITEM ( '' )  );
#18302=CARTESIAN_POINT ( 'NONE',  ( 4.884531539228700758, 3.330387827102500253, -180.0000000000000568 ) ) ;
#18304=CARTESIAN_POINT ( 'NONE',  ( 5.999999999999999112, 2.951592740943527306E-14, -150.0863248654052313 ) ) ;
#18305=CARTESIAN_POINT ( 'NONE',  ( 3.608439182435180470, -6.249999999999997335, -72.19198729810781856 ) ) ;
#18306=CARTESIAN_POINT ( 'NONE',  ( 5.412658773652712085, -3.125000000000086153, -58.56698729810783277 ) ) ;
#18307=CARTESIAN_POINT ( 'NONE',  ( -5.999999999999982236, -1.607695154586700426, -121.3466878364870070 ) ) ;
#18308=CARTESIAN_POINT ( 'NONE',  ( -3.608439182435115633, 6.249999999999965361, -181.8080127018922383 ) ) ;
#18309=CARTESIAN_POINT ( 'NONE',  ( -5.999999999999963585, 1.780251999655701777E-13, -74.33632486540523132 ) ) ;
#18310=CARTESIAN_POINT ( 'NONE',  ( 6.000000000000052403, -1.607695154586662678, -123.1533121635129788 ) ) ;
#18312=CARTESIAN_POINT ( 'NONE',  ( -2.775557561562891351E-14, -5.500000000000115463, -125.2500000000000284 ) ) ;
#18315=VERTEX_POINT ( 'NONE', #6291 ) ;
#18320=ORIENTED_EDGE ( 'NONE', *, *, #19792, .T. ) ;
#18322=CARTESIAN_POINT ( 'NONE',  ( 6.000000000000000888, -1.859271017917181981E-14, -114.6636751345948255 ) ) ;
#18324=CARTESIAN_POINT ( 'NONE',  ( 5.412658773652712085, -3.125000000000086153, -118.5669872981078328 ) ) ;
#18325=CARTESIAN_POINT ( 'NONE',  ( -5.196152422706601826, 2.999999999999975131, -108.0386751345948682 ) ) ;
#18329=ORIENTED_EDGE ( 'NONE', *, *, #24019, .T. ) ;
#18330=DIRECTION ( 'NONE',  ( -7.147005652999508048E-36, 5.642372883946980038E-36, 1.000000000000000000 ) ) ;
#18333=CARTESIAN_POINT ( 'NONE',  ( 3.608439182435180470, 6.249999999999982236, -151.1919872981078186 ) ) ;
#18339=CARTESIAN_POINT ( 'NONE',  ( 3.608439182435180470, -6.249999999999997335, -70.05801270189228092 ) ) ;
#18348=CARTESIAN_POINT ( 'NONE',  ( 3.464101615137757051, -5.999999999999979572, -94.83632486540517448 ) ) ;
#18349=CARTESIAN_POINT ( 'NONE',  ( 4.763139720814407951, 2.750000000000002665, -124.7500000000000284 ) ) ;
#18350=DIRECTION ( 'NONE',  ( -7.147005652999508048E-36, 5.642372883946980038E-36, 1.000000000000000000 ) ) ;
#18352=CARTESIAN_POINT ( 'NONE',  ( 3.175426480543072749, -5.500000000000105693, -54.62500000000003553 ) ) ;
#18353=CARTESIAN_POINT ( 'NONE',  ( 5.196152422706629359, -2.999999999999988898, -153.7886751345948255 ) ) ;
#18354=CARTESIAN_POINT ( 'NONE',  ( -5.196152422706601826, 2.999999999999975131, -171.9613248654052313 ) ) ;
#18355=CARTESIAN_POINT ( 'NONE',  ( 5.196152422706629359, -2.999999999999988898, -151.7113248654052313 ) ) ;
#18364=CARTESIAN_POINT ( 'NONE',  ( 3.175426480543072749, -5.500000000000105693, -134.1250000000000284 ) ) ;
#18365=EDGE_LOOP ( 'NONE', ( #21843, #17986, #2906, #27904 ) ) ;
#18368=CARTESIAN_POINT ( 'NONE',  ( -6.350852961085760029, -1.281975124255709124E-13, -64.12500000000001421 ) ) ;
#18369=CARTESIAN_POINT ( 'NONE',  ( -5.999999999999962697, -1.607695154586733288, -164.8466878364870354 ) ) ;
#18370=EDGE_CURVE ( 'NONE', #21808, #20687, #20064, .T. ) ;
#18371=CARTESIAN_POINT ( 'NONE',  ( 2.775557561562891351E-14, 6.250000000000033751, -90.43301270189225249 ) ) ;
#18372=LINE ( 'NONE', #10852, #10375 ) ;
#18373=CARTESIAN_POINT ( 'NONE',  ( 6.000000000000000888, 1.743066579297358182E-13, -81.08632486540518869 ) ) ;
#18376=CARTESIAN_POINT ( 'NONE',  ( -3.175426480542816066, 5.499999999999865885, -148.3750000000000000 ) ) ;
#18377=CARTESIAN_POINT ( 'NONE',  ( 3.608439182435180470, -6.249999999999997335, -164.5580127018922099 ) ) ;
#18379=CARTESIAN_POINT ( 'NONE',  ( 0.000000000000000000, 5.499999999999991118, -180.0000000000000568 ) ) ;
#18380=CARTESIAN_POINT ( 'NONE',  ( -4.763139720814407951, -2.750000000000016431, -80.50000000000001421 ) ) ;
#18382=CARTESIAN_POINT ( 'NONE',  ( 3.175426480543072749, -5.500000000000105693, -69.62500000000004263 ) ) ;
#18384=CARTESIAN_POINT ( 'NONE',  ( -5.196152422706573404, -3.000000000000002665, -114.7113248654052455 ) ) ;
#18386=CARTESIAN_POINT ( 'NONE',  ( -5.999999999999956479, -1.607695154586745057, -71.84668783648706381 ) ) ;
#18392=( BOUNDED_CURVE ( )  B_SPLINE_CURVE ( 2, ( #25799, #14176, #23513, #25646, #19066, #9528, #25480, #7057, #28237 ),
 .UNSPECIFIED., .F., .T. ) 
 B_SPLINE_CURVE_WITH_KNOTS ( ( 3, 2, 2, 2, 3 ),
 ( 0.4305555555555555802, 0.4314814814814814659, 0.4333333333333333481, 0.4351851851851851749, 0.4361111111111111160 ),
 .UNSPECIFIED. ) 
 CURVE ( )  GEOMETRIC_REPRESENTATION_ITEM ( )  RATIONAL_B_SPLINE_CURVE ( ( 0.9330127018922194093, 0.9330127018922214077, 1.000000000000000000, 0.8660254037844388186, 1.000000000000000000, 0.8660254037844388186, 1.000000000000000000, 0.9330127018922194093, 0.9330127018922194093 ) ) 
 REPRESENTATION_ITEM ( '' )  );
#18395=CARTESIAN_POINT ( 'NONE',  ( 0.000000000000000000, 0.000000000000000000, -14.99152654425661702 ) ) ;
#18397=EDGE_CURVE ( 'NONE', #28105, #2458, #6510, .T. ) ;
#18400=EDGE_LOOP ( 'NONE', ( #18713, #8980, #14114, #29847, #20065 ) ) ;
#18403=CARTESIAN_POINT ( 'NONE',  ( 0.000000000000000000, 5.499999999999991118, -93.00000000000002842 ) ) ;
#18404=AXIS2_PLACEMENT_3D ( 'NONE', #11321, #1451, #13184 ) ;
#18405=CARTESIAN_POINT ( 'NONE',  ( 3.608439182435180470, 6.249999999999982236, -105.5580127018922667 ) ) ;
#18406=LINE ( 'NONE', #6092, #8840 ) ;
#18407=CARTESIAN_POINT ( 'NONE',  ( 6.000000000000000888, 7.762456499804234384E-14, -143.1636751345948255 ) ) ;
#18408=CARTESIAN_POINT ( 'NONE',  ( 3.033369321062211466, -10.57893614291642059, -30.19141222485919585 ) ) ;
#18411=CARTESIAN_POINT ( 'NONE',  ( -2.775557561562891351E-14, -5.500000000000115463, -170.2500000000000000 ) ) ;
#18413=CARTESIAN_POINT ( 'NONE',  ( -6.350852961085760029, -1.281975124255709124E-13, -164.6249999999999716 ) ) ;
#18416=CARTESIAN_POINT ( 'NONE',  ( 6.000000000000007105, -1.607695154586741060, -165.7306624327025872 ) ) ;
#18417=CARTESIAN_POINT ( 'NONE',  ( 0.000000000000000000, 5.499999999999991118, -97.50000000000002842 ) ) ;
#18422=CARTESIAN_POINT ( 'NONE',  ( -5.196152422706573404, -3.000000000000002665, -161.7886751345948255 ) ) ;
#18427=CARTESIAN_POINT ( 'NONE',  ( 0.000000000000000000, 5.999999999999977796, -112.2113248654051887 ) ) ;
#18428=CARTESIAN_POINT ( 'NONE',  ( 7.216878364870455975, -6.409875621278545621E-14, -88.44198729810783277 ) ) ;
#18430=CARTESIAN_POINT ( 'NONE',  ( 5.196152422706629359, -2.999999999999988898, -75.21132486540521711 ) ) ;
#18433=VERTEX_POINT ( 'NONE', #15873 ) ;
#18435=ORIENTED_EDGE ( 'NONE', *, *, #10984, .F. ) ;
#18437=( BOUNDED_CURVE ( )  B_SPLINE_CURVE ( 2, ( #14394, #356, #14101, #11947, #9288, #30173, #9137, #18529, #6976 ),
 .UNSPECIFIED., .F., .F. ) 
 B_SPLINE_CURVE_WITH_KNOTS ( ( 3, 2, 2, 2, 3 ),
 ( 0.3194444444444445308, 0.3203703703703704164, 0.3222222222222221877, 0.3240740740740740700, 0.3249999999999999556 ),
 .UNSPECIFIED. ) 
 CURVE ( )  GEOMETRIC_REPRESENTATION_ITEM ( )  RATIONAL_B_SPLINE_CURVE ( ( 0.9330127018922194093, 0.9330127018922234061, 1.000000000000000000, 0.8660254037844388186, 1.000000000000000000, 0.8660254037844388186, 1.000000000000000000, 0.9330127018922234061, 0.9330127018922194093 ) ) 
 REPRESENTATION_ITEM ( '' )  );
#18438=CARTESIAN_POINT ( 'NONE',  ( 4.763139720814407951, -2.749999999999988454, -123.5000000000000568 ) ) ;
#18440=CARTESIAN_POINT ( 'NONE',  ( 7.216878364870455975, -6.409875621278545621E-14, -134.3080127018922667 ) ) ;
#18442=DIRECTION ( 'NONE',  ( 1.000000000000000000, -5.551115123125773458E-17, -1.260129944081490338E-35 ) ) ;
#18443=CARTESIAN_POINT ( 'NONE',  ( 5.412658773652712085, -3.125000000000086153, -169.5669872981078186 ) ) ;
#18444=CARTESIAN_POINT ( 'NONE',  ( -7.216878364870328078, 0.000000000000000000, -173.1919872981078754 ) ) ;
#18446=DIRECTION ( 'NONE',  ( -7.147005652999508048E-36, 5.642372883946980038E-36, 1.000000000000000000 ) ) ;
#18450=CARTESIAN_POINT ( 'NONE',  ( -5.999999999999963585, -1.487416814333745711E-14, -132.8363248654052597 ) ) ;
#18453=CARTESIAN_POINT ( 'NONE',  ( -3.608439182435052128, -6.250000000000110134, -75.44198729810784698 ) ) ;
#18454=CARTESIAN_POINT ( 'NONE',  ( -7.216878364870328078, 0.000000000000000000, -63.69198729810785409 ) ) ;
#18455=CARTESIAN_POINT ( 'NONE',  ( -3.175426480542816510, -5.500000000000057732, -51.87500000000002132 ) ) ;
#18456=CARTESIAN_POINT ( 'NONE',  ( 6.000000000000000888, 1.743066579297358182E-13, -103.5863248654052171 ) ) ;
#18457=CARTESIAN_POINT ( 'NONE',  ( 0.000000000000000000, -5.999999999999991118, -123.4613248654052313 ) ) ;
#18458=CARTESIAN_POINT ( 'NONE',  ( 6.000000000000052403, -1.607695154586662678, -53.23066243270259434 ) ) ;
#18459=CARTESIAN_POINT ( 'NONE',  ( 4.763139720814407951, 2.750000000000002665, -121.7500000000000284 ) ) ;
#18464=CARTESIAN_POINT ( 'NONE',  ( 6.000000000000000888, 1.607695154586715303, -105.5966878364870496 ) ) ;
#18465=ORIENTED_EDGE ( 'NONE', *, *, #27676, .F. ) ;
#18467=CARTESIAN_POINT ( 'NONE',  ( -3.464101615137725076, 5.999999999999979572, -121.6636751345947971 ) ) ;
#18469=CARTESIAN_POINT ( 'NONE',  ( -3.608439182435052128, -6.250000000000110134, -109.9419872981078043 ) ) ;
#18474=ORIENTED_EDGE ( 'NONE', *, *, #19591, .T. ) ;
#18475=VERTEX_POINT ( 'NONE', #18309 ) ;
#18479=( BOUNDED_CURVE ( )  B_SPLINE_CURVE ( 2, ( #29865, #15640, #12873, #1145, #13482, #15331, #4059, #24652, #22822 ),
 .UNSPECIFIED., .F., .T. ) 
 B_SPLINE_CURVE_WITH_KNOTS ( ( 3, 2, 2, 2, 3 ),
 ( 0.8750000000000000000, 0.8759259259259258856, 0.8777777777777777679, 0.8796296296296296502, 0.8805555555555555358 ),
 .UNSPECIFIED. ) 
 CURVE ( )  GEOMETRIC_REPRESENTATION_ITEM ( )  RATIONAL_B_SPLINE_CURVE ( ( 0.9330127018922194093, 0.9330127018922194093, 1.000000000000000000, 0.8660254037844388186, 1.000000000000000000, 0.8660254037844388186, 1.000000000000000000, 0.9330127018922234061, 0.9330127018922194093 ) ) 
 REPRESENTATION_ITEM ( '' )  );
#18480=ORIENTED_EDGE ( 'NONE', *, *, #2357, .F. ) ;
#18481=CARTESIAN_POINT ( 'NONE',  ( 5.412658773652712085, -3.125000000000086153, -136.5669872981077901 ) ) ;
#18485=CARTESIAN_POINT ( 'NONE',  ( 6.000000000000000888, -1.859271017917181981E-14, -120.6636751345948255 ) ) ;
#18486=CARTESIAN_POINT ( 'NONE',  ( 3.464101615137757051, -5.999999999999979572, -137.4136751345947971 ) ) ;
#18487=CARTESIAN_POINT ( 'NONE',  ( 3.608439182435180470, -6.249999999999997335, -67.05801270189226670 ) ) ;
#18488=( BOUNDED_CURVE ( )  B_SPLINE_CURVE ( 2, ( #13507, #29159, #14921, #15071, #29318, #12629, #8276, #29011, #20540 ),
 .UNSPECIFIED., .F., .T. ) 
 B_SPLINE_CURVE_WITH_KNOTS ( ( 3, 2, 2, 2, 3 ),
 ( 0.07500000000000006661, 0.07592592592592595224, 0.07777777777777772350, 0.07962962962962960578, 0.08055555555555549141 ),
 .UNSPECIFIED. ) 
 CURVE ( )  GEOMETRIC_REPRESENTATION_ITEM ( )  RATIONAL_B_SPLINE_CURVE ( ( 0.9330127018922194093, 0.9330127018922234061, 1.000000000000000000, 0.8660254037844388186, 1.000000000000000000, 0.8660254037844388186, 1.000000000000000000, 0.9330127018922234061, 0.9330127018922194093 ) ) 
 REPRESENTATION_ITEM ( '' )  );
#18494=CARTESIAN_POINT ( 'NONE',  ( -5.196152422706573404, -3.000000000000002665, -67.28867513459479710 ) ) ;
#18497=CARTESIAN_POINT ( 'NONE',  ( 4.763139720814407951, -2.749999999999988454, -122.0000000000000000 ) ) ;
#18500=ORIENTED_EDGE ( 'NONE', *, *, #28478, .T. ) ;
#18501=ADVANCED_FACE ( 'NONE', ( #23054 ), #14021, .T. ) ;
#18502=CARTESIAN_POINT ( 'NONE',  ( 4.763139720814407951, -2.749999999999988454, -57.49999999999999289 ) ) ;
#18504=CARTESIAN_POINT ( 'NONE',  ( 5.196152422706629359, -2.999999999999988898, -163.7113248654051745 ) ) ;
#18508=CARTESIAN_POINT ( 'NONE',  ( 0.000000000000000000, 5.999999999999977796, -46.21132486540524553 ) ) ;
#18513=CARTESIAN_POINT ( 'NONE',  ( 0.000000000000000000, 5.499999999999991118, -135.0000000000000000 ) ) ;
#18514=ORIENTED_EDGE ( 'NONE', *, *, #22000, .T. ) ;
#18518=CARTESIAN_POINT ( 'NONE',  ( 6.350852961086080661, -9.614813431917819062E-14, -66.37500000000004263 ) ) ;
#18519=CARTESIAN_POINT ( 'NONE',  ( 5.196152422706629359, -2.999999999999988898, -164.2886751345948824 ) ) ;
#18521=CARTESIAN_POINT ( 'NONE',  ( 0.000000000000000000, 5.999999999999977796, -150.2886751345948255 ) ) ;
#18522=CARTESIAN_POINT ( 'NONE',  ( -5.999999999999963585, 0.000000000000000000, -179.9136751345948255 ) ) ;
#18524=CARTESIAN_POINT ( 'NONE',  ( 6.350852961086080661, -9.614813431917819062E-14, -144.3750000000000853 ) ) ;
#18526=CARTESIAN_POINT ( 'NONE',  ( -3.175426480542816510, 5.499999999999865885, -142.3750000000000568 ) ) ;
#18527=CARTESIAN_POINT ( 'NONE',  ( 2.775557561562891351E-14, 6.250000000000033751, -163.9330127018922667 ) ) ;
#18528=CARTESIAN_POINT ( 'NONE',  ( 21.99999999999993605, -11.00000000000004086, -14.99152654425661879 ) ) ;
#18529=CARTESIAN_POINT ( 'NONE',  ( 5.999999999999949374, 1.607695154586804565, -90.01933756729741276 ) ) ;
#18531=CARTESIAN_POINT ( 'NONE',  ( -6.350852961085760029, -1.281975124255709124E-13, -77.62500000000001421 ) ) ;
#18532=VECTOR ( 'NONE', #3985, 1000.000000000000000 ) ;
#18533=CARTESIAN_POINT ( 'NONE',  ( 4.763139720814407951, -2.749999999999988454, -72.50000000000001421 ) ) ;
#18534=CARTESIAN_POINT ( 'NONE',  ( 5.196152422706629359, -2.999999999999988898, -156.2113248654052313 ) ) ;
#18541=CARTESIAN_POINT ( 'NONE',  ( -3.464101615137757051, -5.999999999999979572, -147.5863248654051745 ) ) ;
#18544=CARTESIAN_POINT ( 'NONE',  ( 0.000000000000000000, 5.999999999999977796, -139.2113248654052313 ) ) ;
#18545=ORIENTED_EDGE ( 'NONE', *, *, #13344, .T. ) ;
#18547=CARTESIAN_POINT ( 'NONE',  ( 5.196152422706629359, -2.999999999999988898, -156.7886751345948255 ) ) ;
#18549=CARTESIAN_POINT ( 'NONE',  ( 6.000000000000000888, -3.330669073875464691E-16, -7.560779664488942560E-35 ) ) ;
#18551=ORIENTED_EDGE ( 'NONE', *, *, #6216, .F. ) ;
#18552=VERTEX_POINT ( 'NONE', #7646 ) ;
#18553=CARTESIAN_POINT ( 'NONE',  ( -4.763139720814407951, -2.750000000000016431, -86.50000000000002842 ) ) ;
#18555=CARTESIAN_POINT ( 'NONE',  ( 2.775557561562891351E-14, -6.250000000000061284, -107.6830127018922383 ) ) ;
#18556=CARTESIAN_POINT ( 'NONE',  ( 6.000643140593935776, 9.219125907743233483, -25.38858793365676192 ) ) ;
#18558=CARTESIAN_POINT ( 'NONE',  ( 3.175426480543072749, 5.499999999999865885, -165.1249999999999716 ) ) ;
#18559=CARTESIAN_POINT ( 'NONE',  ( 2.775557561562891351E-14, 6.250000000000033751, -46.93301270189220986 ) ) ;
#18563=CARTESIAN_POINT ( 'NONE',  ( 6.350852961086080661, -9.614813431917819062E-14, -169.8750000000000853 ) ) ;
#18564=DIRECTION ( 'NONE',  ( -7.147005652999508048E-36, 5.642372883946980038E-36, 1.000000000000000000 ) ) ;
#18565=CARTESIAN_POINT ( 'NONE',  ( -4.763139720814407951, 2.749999999999946709, -164.7500000000000000 ) ) ;
#18568=CARTESIAN_POINT ( 'NONE',  ( -2.775557561562891351E-14, -5.500000000000115463, -99.75000000000000000 ) ) ;
#18570=CARTESIAN_POINT ( 'NONE',  ( 3.464101615137852974, 5.999999999999884537, -87.41367513459482552 ) ) ;
#18572=CARTESIAN_POINT ( 'NONE',  ( 3.175426480543072749, 5.499999999999865885, -94.62500000000002842 ) ) ;
#18579=CARTESIAN_POINT ( 'NONE',  ( 0.000000000000000000, 0.000000000000000000, 0.000000000000000000 ) ) ;
#18583=CARTESIAN_POINT ( 'NONE',  ( -5.196152422706601826, 2.999999999999975131, -111.9613248654052171 ) ) ;
#18584=VERTEX_POINT ( 'NONE', #12309 ) ;
#18585=CARTESIAN_POINT ( 'NONE',  ( 0.000000000000000000, -5.999999999999991118, -75.46132486540524553 ) ) ;
#18587=CARTESIAN_POINT ( 'NONE',  ( 4.763139720814407951, -2.749999999999988454, -115.9999999999999858 ) ) ;
#18589=CARTESIAN_POINT ( 'NONE',  ( 2.775557561562891351E-14, 6.250000000000033751, -129.4330127018922383 ) ) ;
#18591=CARTESIAN_POINT ( 'NONE',  ( -5.999999999999919176, 1.607695154586804565, -56.98066243270260145 ) ) ;
#18592=CARTESIAN_POINT ( 'NONE',  ( -5.412658773652684552, -3.125000000000099920, -170.0669872981078186 ) ) ;
#18593=CARTESIAN_POINT ( 'NONE',  ( 2.775557561562891351E-14, 6.250000000000033751, -176.5669872981078186 ) ) ;
#18595=EDGE_LOOP ( 'NONE', ( #9234, #7231, #4154, #6048 ) ) ;
#18599=LINE ( 'NONE', #27921, #1074 ) ;
#18603=CARTESIAN_POINT ( 'NONE',  ( -5.412658773652684552, -3.125000000000099920, -72.56698729810784698 ) ) ;
#18604=CARTESIAN_POINT ( 'NONE',  ( 5.412658773652739619, 3.124999999999988898, -62.81698729810780435 ) ) ;
#18605=CARTESIAN_POINT ( 'NONE',  ( 0.000000000000000000, 5.499999999999991118, -46.49999999999998579 ) ) ;
#18607=FACE_OUTER_BOUND ( 'NONE', #5081, .T. ) ;
#18610=CARTESIAN_POINT ( 'NONE',  ( 4.763139720814407951, 2.750000000000002665, -123.2500000000000284 ) ) ;
#18611=CARTESIAN_POINT ( 'NONE',  ( 6.000000000000000888, -3.330669073875464691E-16, -7.560779664488942560E-35 ) ) ;
#18615=VERTEX_POINT ( 'NONE', #14317 ) ;
#18618=CARTESIAN_POINT ( 'NONE',  ( -3.608439182435052128, -6.250000000000110134, -111.4419872981078186 ) ) ;
#18619=( BOUNDED_CURVE ( )  B_SPLINE_CURVE ( 2, ( #6245, #27423, #6389, #29891, #5931, #8872, #22850, #25269, #25124 ),
 .UNSPECIFIED., .F., .F. ) 
 B_SPLINE_CURVE_WITH_KNOTS ( ( 3, 2, 2, 2, 3 ),
 ( 0.2083333333333333426, 0.2092592592592592560, 0.2111111111111111105, 0.2129629629629629650, 0.2138888888888888784 ),
 .UNSPECIFIED. ) 
 CURVE ( )  GEOMETRIC_REPRESENTATION_ITEM ( )  RATIONAL_B_SPLINE_CURVE ( ( 0.9330127018922194093, 0.9330127018922204085, 1.000000000000000000, 0.8660254037844388186, 1.000000000000000000, 0.8660254037844388186, 1.000000000000000000, 0.9330127018922205195, 0.9330127018922196314 ) ) 
 REPRESENTATION_ITEM ( '' )  );
#18621=AXIS2_PLACEMENT_3D ( 'NONE', #28872, #26424, #5673 ) ;
#18623=ORIENTED_EDGE ( 'NONE', *, *, #22363, .T. ) ;
#18625=DIRECTION ( 'NONE',  ( -7.147005652999508048E-36, 5.642372883946980038E-36, 1.000000000000000000 ) ) ;
#18628=CARTESIAN_POINT ( 'NONE',  ( 7.216878364870455975, -6.409875621278545621E-14, -140.9419872981078470 ) ) ;
#18630=EDGE_CURVE ( 'NONE', #15775, #10765, #27671, .T. ) ;
#18633=LINE ( 'NONE', #28111, #20598 ) ;
#18634=CARTESIAN_POINT ( 'NONE',  ( -3.608439182435115633, 6.249999999999965361, -66.30801270189226670 ) ) ;
#18638=FACE_OUTER_BOUND ( 'NONE', #15104, .T. ) ;
#18639=CARTESIAN_POINT ( 'NONE',  ( 5.196152422706629359, 3.000000000000002665, -165.5386751345948539 ) ) ;
#18646=CARTESIAN_POINT ( 'NONE',  ( -4.763139720814407951, -2.750000000000016431, -122.5000000000000568 ) ) ;
#18650=CARTESIAN_POINT ( 'NONE',  ( 2.849036369511732440E-14, 20.00000000000001776, -19.00000000000002132 ) ) ;
#18652=CARTESIAN_POINT ( 'NONE',  ( -2.775557561562891351E-14, -5.500000000000115463, -53.25000000000002132 ) ) ;
#18653=CARTESIAN_POINT ( 'NONE',  ( -3.464101615137757051, -5.999999999999979572, -155.0863248654052029 ) ) ;
#18654=CARTESIAN_POINT ( 'NONE',  ( 0.000000000000000000, 5.999999999999977796, -121.2113248654052029 ) ) ;
#18655=CARTESIAN_POINT ( 'NONE',  ( 6.000000000000001776, 5.345404176511898156E-15, -178.5863248654052313 ) ) ;
#18656=ORIENTED_EDGE ( 'NONE', *, *, #8411, .T. ) ;
#18659=CARTESIAN_POINT ( 'NONE',  ( -3.608439182435115633, 6.249999999999965361, -104.4419872981078470 ) ) ;
#18661=( BOUNDED_CURVE ( )  B_SPLINE_CURVE ( 2, ( #20593, #24734, #1693, #6604, #3675, #27180, #15565, #8770, #17863 ),
 .UNSPECIFIED., .F., .F. ) 
 B_SPLINE_CURVE_WITH_KNOTS ( ( 3, 2, 2, 2, 3 ),
 ( 0.03055555555555555802, 0.03148148148148144365, 0.03333333333333332593, 0.03518518518518520821, 0.03611111111111109384 ),
 .UNSPECIFIED. ) 
 CURVE ( )  GEOMETRIC_REPRESENTATION_ITEM ( )  RATIONAL_B_SPLINE_CURVE ( ( 0.9330127018922194093, 0.9330127018922194093, 1.000000000000000000, 0.8660254037844388186, 1.000000000000000000, 0.8660254037844388186, 1.000000000000000000, 0.9330127018922234061, 0.9330127018922194093 ) ) 
 REPRESENTATION_ITEM ( '' )  );
#18663=DIRECTION ( 'NONE',  ( -7.147005652999508048E-36, 5.642372883946980038E-36, 1.000000000000000000 ) ) ;
#18664=CARTESIAN_POINT ( 'NONE',  ( 3.175426480543072749, 5.499999999999865885, -136.6250000000000568 ) ) ;
#18669=EDGE_CURVE ( 'NONE', #18250, #23969, #5500, .T. ) ;
#18670=CARTESIAN_POINT ( 'NONE',  ( 6.350852961086080661, -9.614813431917819062E-14, -61.87500000000000711 ) ) ;
#18672=CARTESIAN_POINT ( 'NONE',  ( 6.000000000000026645, -1.607695154586707753, -123.7306624327026014 ) ) ;
#18673=ORIENTED_EDGE ( 'NONE', *, *, #22963, .T. ) ;
#18678=CARTESIAN_POINT ( 'NONE',  ( -3.175426480542816066, -5.500000000000057732, -150.8749999999999716 ) ) ;
#18680=CARTESIAN_POINT ( 'NONE',  ( 3.175426480543072749, -5.500000000000105693, -134.1250000000000284 ) ) ;
#18681=CARTESIAN_POINT ( 'NONE',  ( -3.608439182435052128, -6.250000000000110134, -161.8080127018922667 ) ) ;
#18682=DIRECTION ( 'NONE',  ( -7.147005652999508048E-36, 5.642372883946980038E-36, 1.000000000000000000 ) ) ;
#18683=CARTESIAN_POINT ( 'NONE',  ( -2.775557561562891351E-14, -5.500000000000115463, -81.74999999999998579 ) ) ;
#18684=CARTESIAN_POINT ( 'NONE',  ( 6.000000000000026645, -1.607695154586707753, -140.2306624327026157 ) ) ;
#18686=CARTESIAN_POINT ( 'NONE',  ( 0.000000000000000000, 5.499999999999991118, -63.00000000000000000 ) ) ;
#18687=DIRECTION ( 'NONE',  ( -7.147005652999508048E-36, 5.642372883946980038E-36, 1.000000000000000000 ) ) ;
#18688=CARTESIAN_POINT ( 'NONE',  ( 0.000000000000000000, -5.999999999999991118, -114.4613248654052171 ) ) ;
#18689=LINE ( 'NONE', #13483, #11594 ) ;
#18696=CARTESIAN_POINT ( 'NONE',  ( 5.196152422706629359, -2.999999999999988898, -97.71132486540523132 ) ) ;
#18699=CARTESIAN_POINT ( 'NONE',  ( 6.000000000000000888, 1.743066579297358182E-13, -108.6636751345948255 ) ) ;
#18701=CARTESIAN_POINT ( 'NONE',  ( 0.000000000000000000, 0.000000000000000000, 0.000000000000000000 ) ) ;
#18702=VERTEX_POINT ( 'NONE', #13787 ) ;
#18704=VERTEX_POINT ( 'NONE', #13219 ) ;
#18705=EDGE_CURVE ( 'NONE', #13073, #26551, #12908, .T. ) ;
#18706=CARTESIAN_POINT ( 'NONE',  ( -4.763139720814407951, -2.750000000000016431, -89.50000000000002842 ) ) ;
#18708=CARTESIAN_POINT ( 'NONE',  ( 5.412658773652739619, 3.124999999999988898, -110.1830127018922383 ) ) ;
#18709=VERTEX_POINT ( 'NONE', #8407 ) ;
#18712=CARTESIAN_POINT ( 'NONE',  ( -3.608439182435052128, -6.250000000000110134, -47.80801270189223828 ) ) ;
#18713=ORIENTED_EDGE ( 'NONE', *, *, #3096, .F. ) ;
#18714=ADVANCED_FACE ( 'NONE', ( #15363 ), #12755, .T. ) ;
#18716=VECTOR ( 'NONE', #30262, 1000.000000000000000 ) ;
#18717=CARTESIAN_POINT ( 'NONE',  ( -4.763139720814407951, -2.750000000000016431, -173.5000000000000000 ) ) ;
#18719=CARTESIAN_POINT ( 'NONE',  ( -3.175426480542816510, 5.499999999999865885, -158.8750000000000000 ) ) ;
#18721=CARTESIAN_POINT ( 'NONE',  ( 3.175426480543072749, -5.500000000000105693, -104.1250000000000142 ) ) ;
#18722=LINE ( 'NONE', #23013, #37 ) ;
#18723=CARTESIAN_POINT ( 'NONE',  ( 3.175426480543072749, -5.500000000000105693, -96.62500000000004263 ) ) ;
#18730=CARTESIAN_POINT ( 'NONE',  ( 3.464101615137757051, -5.999999999999979572, -161.4136751345947971 ) ) ;
#18731=CIRCLE ( 'NONE', #5430, 5.999999999999992006 ) ;
#18734=ORIENTED_EDGE ( 'NONE', *, *, #25503, .F. ) ;
#18739=EDGE_LOOP ( 'NONE', ( #17708, #15999, #120, #16849 ) ) ;
#18745=CARTESIAN_POINT ( 'NONE',  ( 3.175426480543072749, -5.500000000000105693, -114.6250000000000000 ) ) ;
#18747=EDGE_CURVE ( 'NONE', #25740, #25500, #18301, .T. ) ;
#18748=CARTESIAN_POINT ( 'NONE',  ( 2.775557561562891351E-14, -6.250000000000061284, -134.6830127018922667 ) ) ;
#18749=EDGE_LOOP ( 'NONE', ( #21839, #27411, #13042, #2470 ) ) ;
#18750=CARTESIAN_POINT ( 'NONE',  ( 5.412658773652739619, 3.124999999999988898, -172.3169872981078470 ) ) ;
#18756=CARTESIAN_POINT ( 'NONE',  ( -4.763139720814407951, -2.750000000000016431, -181.0000000000000568 ) ) ;
#18758=CARTESIAN_POINT ( 'NONE',  ( 5.196152422706629359, 3.000000000000002665, -110.9613248654052171 ) ) ;
#18759=CARTESIAN_POINT ( 'NONE',  ( 3.608439182435180470, -6.249999999999997335, -178.0580127018922383 ) ) ;
#18760=CARTESIAN_POINT ( 'NONE',  ( 5.999999999999949374, 1.607695154586804565, -103.5193375672974412 ) ) ;
#18763=CARTESIAN_POINT ( 'NONE',  ( -6.350852961085760029, -1.281975124255709124E-13, -124.1250000000000568 ) ) ;
#18768=AXIS2_PLACEMENT_3D ( 'NONE', #11630, #8986, #27850 ) ;
#18769=CARTESIAN_POINT ( 'NONE',  ( 6.000000000000000888, -1.859271017917181981E-14, -159.6636751345948539 ) ) ;
#18775=CARTESIAN_POINT ( 'NONE',  ( 6.000000000000000888, -3.330669073875464691E-16, -7.560779664488942560E-35 ) ) ;
#18776=CARTESIAN_POINT ( 'NONE',  ( -5.412658773652684552, -3.125000000000099920, -108.5669872981078186 ) ) ;
#18779=ORIENTED_EDGE ( 'NONE', *, *, #13916, .F. ) ;
#18781=CARTESIAN_POINT ( 'NONE',  ( 0.000000000000000000, -5.999999999999991118, -142.0386751345948255 ) ) ;
#18784=ADVANCED_FACE ( 'NONE', ( #11482 ), #12035, .F. ) ;
#18785=CARTESIAN_POINT ( 'NONE',  ( 5.412658773652712085, -3.125000000000086153, -138.0669872981078470 ) ) ;
#18787=DIRECTION ( 'NONE',  ( -7.147005652999508048E-36, 5.642372883946980038E-36, 1.000000000000000000 ) ) ;
#18788=CARTESIAN_POINT ( 'NONE',  ( 6.000000000000000888, 1.743066579297358182E-13, -51.08632486540523132 ) ) ;
#18791=CARTESIAN_POINT ( 'NONE',  ( 5.412658773652739619, 3.124999999999988898, -59.18301270189224539 ) ) ;
#18793=CARTESIAN_POINT ( 'NONE',  ( -3.464101615137757051, -5.999999999999979572, -125.0863248654052029 ) ) ;
#18794=CARTESIAN_POINT ( 'NONE',  ( 6.000000000000000888, -1.607695154586752384, -160.6533121635129930 ) ) ;
#18800=ORIENTED_EDGE ( 'NONE', *, *, #20218, .F. ) ;
#18801=( BOUNDED_CURVE ( )  B_SPLINE_CURVE ( 2, ( #5371, #19388, #2922, #14779, #25980, #7684, #17093, #9561, #23694 ),
 .UNSPECIFIED., .F., .F. ) 
 B_SPLINE_CURVE_WITH_KNOTS ( ( 3, 2, 2, 2, 3 ),
 ( 0.1694444444444443976, 0.1703703703703703942, 0.1722222222222222765, 0.1740740740740740478, 0.1750000000000000444 ),
 .UNSPECIFIED. ) 
 CURVE ( )  GEOMETRIC_REPRESENTATION_ITEM ( )  RATIONAL_B_SPLINE_CURVE ( ( 0.9330127018922194093, 0.9330127018922154125, 1.000000000000000000, 0.8660254037844388186, 1.000000000000000000, 0.8660254037844388186, 1.000000000000000000, 0.9330127018922154125, 0.9330127018922194093 ) ) 
 REPRESENTATION_ITEM ( '' )  );
#18802=CARTESIAN_POINT ( 'NONE',  ( 4.763139720814407951, -2.749999999999988454, -54.49999999999999289 ) ) ;
#18803=CARTESIAN_POINT ( 'NONE',  ( -5.196152422706573404, -3.000000000000002665, -155.2113248654052313 ) ) ;
#18804=FACE_OUTER_BOUND ( 'NONE', #18595, .T. ) ;
#18805=AXIS2_PLACEMENT_3D ( 'NONE', #20700, #11038, #18259 ) ;
#18806=CARTESIAN_POINT ( 'NONE',  ( -5.999999999999962697, 3.323446944526963260E-14, -152.3363248654052313 ) ) ;
#18810=CARTESIAN_POINT ( 'NONE',  ( 5.412658773652739619, 3.124999999999988898, -106.3169872981078470 ) ) ;
#18811=CARTESIAN_POINT ( 'NONE',  ( 3.464101615137852974, 5.999999999999884537, -176.8363248654051176 ) ) ;
#18813=CARTESIAN_POINT ( 'NONE',  ( 6.350852961086080661, -9.614813431917819062E-14, -133.8750000000000284 ) ) ;
#18814=ADVANCED_FACE ( 'NONE', ( #2232 ), #11633, .T. ) ;
#18816=ORIENTED_EDGE ( 'NONE', *, *, #22117, .F. ) ;
#18818=CARTESIAN_POINT ( 'NONE',  ( -4.763139720814407951, -2.750000000000016431, -65.50000000000000000 ) ) ;
#18819=CARTESIAN_POINT ( 'NONE',  ( -6.000000000000007105, -1.607695154586655129, -81.76933756729744118 ) ) ;
#18821=CARTESIAN_POINT ( 'NONE',  ( 2.775557561562891351E-14, -6.250000000000061284, -86.68301270189226670 ) ) ;
#18822=CARTESIAN_POINT ( 'NONE',  ( -5.196152422706573404, -3.000000000000002665, -101.2113248654052455 ) ) ;
#18827=CARTESIAN_POINT ( 'NONE',  ( -2.775557561562891351E-14, -5.500000000000115463, -147.7500000000000568 ) ) ;
#18829=CARTESIAN_POINT ( 'NONE',  ( -7.216878364870328078, 0.000000000000000000, -162.0580127018922099 ) ) ;
#18830=( LENGTH_UNIT ( ) NAMED_UNIT ( * ) SI_UNIT ( .MILLI., .METRE. ) );
#18832=CARTESIAN_POINT ( 'NONE',  ( -2.775557561562891351E-14, -5.500000000000115463, -80.25000000000004263 ) ) ;
#18834=CARTESIAN_POINT ( 'NONE',  ( 4.763139720814407951, 2.750000000000002665, -67.75000000000002842 ) ) ;
#18835=( BOUNDED_CURVE ( )  B_SPLINE_CURVE ( 2, ( #23668, #2604, #17470, #5749, #12023, #18923, #156, #21360, #21517 ),
 .UNSPECIFIED., .F., .T. ) 
 B_SPLINE_CURVE_WITH_KNOTS ( ( 3, 2, 2, 2, 3 ),
 ( 0.6305555555555555358, 0.6314814814814815325, 0.6333333333333333037, 0.6351851851851851860, 0.6361111111111110716 ),
 .UNSPECIFIED. ) 
 CURVE ( )  GEOMETRIC_REPRESENTATION_ITEM ( )  RATIONAL_B_SPLINE_CURVE ( ( 0.9330127018922194093, 0.9330127018922154125, 1.000000000000000000, 0.8660254037844388186, 1.000000000000000000, 0.8660254037844388186, 1.000000000000000000, 0.9330127018922234061, 0.9330127018922194093 ) ) 
 REPRESENTATION_ITEM ( '' )  );
#18837=CARTESIAN_POINT ( 'NONE',  ( -5.196152422706573404, -3.000000000000002665, -156.7113248654052313 ) ) ;
#18843=EDGE_CURVE ( 'NONE', #20404, #2534, #28477, .T. ) ;
#18844=CARTESIAN_POINT ( 'NONE',  ( -5.999999999999963585, -1.487416814333745711E-14, -50.33632486540523843 ) ) ;
#18845=CARTESIAN_POINT ( 'NONE',  ( 0.000000000000000000, -5.999999999999991118, -147.4613248654052029 ) ) ;
#18847=DIRECTION ( 'NONE',  ( 1.000000000000000000, -5.551115123125773458E-17, -1.260129944081490338E-35 ) ) ;
#18852=CARTESIAN_POINT ( 'NONE',  ( -4.763139720814407951, -2.750000000000016431, -154.0000000000000284 ) ) ;
#18857=EDGE_LOOP ( 'NONE', ( #20918, #18177, #27032, #5868 ) ) ;
#18858=CARTESIAN_POINT ( 'NONE',  ( 4.763139720814407951, -2.749999999999988454, -90.50000000000002842 ) ) ;
#18859=ORIENTED_EDGE ( 'NONE', *, *, #14546, .T. ) ;
#18860=CARTESIAN_POINT ( 'NONE',  ( 1.000434615788146742, 10.95616177385588941, -19.08065934301228594 ) ) ;
#18863=CARTESIAN_POINT ( 'NONE',  ( 4.763139720814407951, -2.749999999999988454, -164.0000000000000284 ) ) ;
#18864=CARTESIAN_POINT ( 'NONE',  ( -3.464101615137757051, -5.999999999999979572, -63.58632486540521711 ) ) ;
#18865=DIRECTION ( 'NONE',  ( -7.147005652999508048E-36, 5.642372883946980038E-36, 1.000000000000000000 ) ) ;
#18866=CARTESIAN_POINT ( 'NONE',  ( 4.763139720814407951, -2.749999999999988454, -176.0000000000000568 ) ) ;
#18868=CARTESIAN_POINT ( 'NONE',  ( -2.775557561562891351E-14, -5.500000000000115463, -156.7500000000000568 ) ) ;
#18870=CARTESIAN_POINT ( 'NONE',  ( 4.763139720814407951, 2.750000000000002665, -100.7500000000000000 ) ) ;
#18871=CARTESIAN_POINT ( 'NONE',  ( 6.000000000000000888, -1.859271017917181981E-14, -159.0863248654052313 ) ) ;
#18873=CARTESIAN_POINT ( 'NONE',  ( -3.175426480542816510, -5.500000000000057732, -155.3750000000000000 ) ) ;
#18874=CARTESIAN_POINT ( 'NONE',  ( 0.000000000000000000, 5.499999999999991118, -90.00000000000002842 ) ) ;
#18878=ORIENTED_EDGE ( 'NONE', *, *, #29228, .F. ) ;
#18882=EDGE_CURVE ( 'NONE', #17680, #9948, #22401, .T. ) ;
#18883=CARTESIAN_POINT ( 'NONE',  ( 6.000000000000000888, -1.859271017917181981E-14, -168.6636751345947971 ) ) ;
#18885=LINE ( 'NONE', #25916, #4169 ) ;
#18887=FACE_OUTER_BOUND ( 'NONE', #27627, .T. ) ;
#18891=VECTOR ( 'NONE', #26987, 1000.000000000000000 ) ;
#18894=CARTESIAN_POINT ( 'NONE',  ( 3.464101615137757051, -5.999999999999979572, -52.83632486540517448 ) ) ;
#18895=EDGE_CURVE ( 'NONE', #3013, #20406, #6697, .T. ) ;
#18899=CARTESIAN_POINT ( 'NONE',  ( 6.350852961086080661, -9.614813431917819062E-14, -109.8750000000000426 ) ) ;
#18901=CARTESIAN_POINT ( 'NONE',  ( -2.775557561562891351E-14, -5.500000000000115463, -150.7500000000000568 ) ) ;
#18902=CARTESIAN_POINT ( 'NONE',  ( -5.412658773652739619, 3.124999999999975131, -130.6830127018922667 ) ) ;
#18905=CARTESIAN_POINT ( 'NONE',  ( -7.216878364870328078, 0.000000000000000000, -171.6919872981078186 ) ) ;
#18911=CARTESIAN_POINT ( 'NONE',  ( -6.350852961085760029, -1.281975124255709124E-13, -179.6250000000000284 ) ) ;
#18913=CARTESIAN_POINT ( 'NONE',  ( -3.608439182435115633, 6.249999999999965361, -175.8080127018922667 ) ) ;
#18914=CARTESIAN_POINT ( 'NONE',  ( 6.000000000000052403, -1.607695154586662678, -48.15331216351300725 ) ) ;
#18915=CARTESIAN_POINT ( 'NONE',  ( -5.196152422706573404, -3.000000000000002665, -53.78867513459483973 ) ) ;
#18917=CARTESIAN_POINT ( 'NONE',  ( 6.350852961086080661, -9.614813431917819062E-14, -111.3750000000000568 ) ) ;
#18923=CARTESIAN_POINT ( 'NONE',  ( 3.464101615137852974, 5.999999999999884537, -131.8363248654052313 ) ) ;
#18924=ORIENTED_EDGE ( 'NONE', *, *, #26226, .F. ) ;
#18925=AXIS2_PLACEMENT_3D ( 'NONE', #18227, #13947, #20826 ) ;
#18929=AXIS2_PLACEMENT_3D ( 'NONE', #22982, #1920, #20830 ) ;
#18930=CARTESIAN_POINT ( 'NONE',  ( 0.000000000000000000, 0.000000000000000000, 0.000000000000000000 ) ) ;
#18931=VERTEX_POINT ( 'NONE', #29057 ) ;
#18932=EDGE_CURVE ( 'NONE', #5324, #5195, #22016, .T. ) ;
#18933=CARTESIAN_POINT ( 'NONE',  ( 3.464101615137757051, -5.999999999999979572, -125.4136751345948113 ) ) ;
#18935=DIRECTION ( 'NONE',  ( 1.000000000000000000, -5.551115123125773458E-17, -1.260129944081490338E-35 ) ) ;
#18937=ORIENTED_EDGE ( 'NONE', *, *, #20218, .T. ) ;
#18942=CARTESIAN_POINT ( 'NONE',  ( 3.608439182435180470, 6.249999999999982236, -142.1919872981078470 ) ) ;
#18948=DIRECTION ( 'NONE',  ( -7.147005652999508048E-36, 5.642372883946980038E-36, 1.000000000000000000 ) ) ;
#18952=CARTESIAN_POINT ( 'NONE',  ( 5.196152422706629359, 3.000000000000002665, -60.53867513459481842 ) ) ;
#18953=CARTESIAN_POINT ( 'NONE',  ( -5.999999999999963585, -1.487416814333745711E-14, -113.3363248654052029 ) ) ;
#18959=CARTESIAN_POINT ( 'NONE',  ( 3.175426480543072749, 5.499999999999865885, -57.12500000000006395 ) ) ;
#18962=CARTESIAN_POINT ( 'NONE',  ( 0.000000000000000000, -5.999999999999991118, -151.9613248654052597 ) ) ;
#18964=EDGE_LOOP ( 'NONE', ( #12223, #22786, #25664, #29615 ) ) ;
#18968=CARTESIAN_POINT ( 'NONE',  ( -5.412658773652684552, -3.125000000000099920, -99.56698729810781856 ) ) ;
#18969=CARTESIAN_POINT ( 'NONE',  ( 6.000000000000000888, 5.577813053751546416E-15, -177.0863248654052597 ) ) ;
#18973=CARTESIAN_POINT ( 'NONE',  ( 6.350852961086080661, -9.614813431917819062E-14, -129.3750000000000284 ) ) ;
#18974=ORIENTED_EDGE ( 'NONE', *, *, #20873, .F. ) ;
#18975=CARTESIAN_POINT ( 'NONE',  ( -2.775557561562891351E-14, -5.500000000000115463, -63.75000000000002842 ) ) ;
#18976=CARTESIAN_POINT ( 'NONE',  ( 0.000000000000000000, 5.999999999999977796, -115.7886751345948397 ) ) ;
#18978=CARTESIAN_POINT ( 'NONE',  ( 5.999999999999974243, 1.607695154586759934, -140.0966878364870354 ) ) ;
#18984=CARTESIAN_POINT ( 'NONE',  ( -4.763139720814407951, 2.749999999999946709, -139.2499999999999716 ) ) ;
#18985=CARTESIAN_POINT ( 'NONE',  ( 0.000000000000000000, -5.999999999999991118, -105.4613248654052171 ) ) ;
#18988=CARTESIAN_POINT ( 'NONE',  ( -2.775557561562891351E-14, -5.500000000000115463, -78.74999999999998579 ) ) ;
#18989=CARTESIAN_POINT ( 'NONE',  ( 6.000000000000000888, -1.859271017917181981E-14, -114.6636751345948255 ) ) ;
#18990=CARTESIAN_POINT ( 'NONE',  ( -3.464101615137725076, 5.999999999999979572, -173.5863248654052313 ) ) ;
#18991=CARTESIAN_POINT ( 'NONE',  ( -4.763139720814407951, 2.749999999999946709, -64.25000000000002842 ) ) ;
#18992=ADVANCED_FACE ( 'NONE', ( #21873 ), #8023, .T. ) ;
#18994=CARTESIAN_POINT ( 'NONE',  ( -5.999999999999968026, -1.607695154586722186, -148.3466878364870354 ) ) ;
#18997=CARTESIAN_POINT ( 'NONE',  ( -5.999999999999963585, 8.134310703387671600E-14, -140.9136751345947971 ) ) ;
#19004=VECTOR ( 'NONE', #19971, 1000.000000000000000 ) ;
#19006=VERTEX_POINT ( 'NONE', #10351 ) ;
#19008=ORIENTED_EDGE ( 'NONE', *, *, #6262, .F. ) ;
#19009=CARTESIAN_POINT ( 'NONE',  ( 3.175426480543072749, -5.500000000000105693, -87.62500000000000000 ) ) ;
#19010=CARTESIAN_POINT ( 'NONE',  ( 2.775557561562891351E-14, -6.250000000000061284, -101.6830127018922241 ) ) ;
#19014=CARTESIAN_POINT ( 'NONE',  ( 4.763139720814407951, -2.749999999999988454, -167.0000000000000284 ) ) ;
#19015=CARTESIAN_POINT ( 'NONE',  ( 2.145494852022844068, -10.79031218954989235, -19.39330237445247462 ) ) ;
#19016=DIRECTION ( 'NONE',  ( -7.147005652999508048E-36, 5.642372883946980038E-36, 1.000000000000000000 ) ) ;
#19020=( BOUNDED_CURVE ( )  B_SPLINE_CURVE ( 2, ( #26450, #26737, #5403, #24297, #14812, #17276, #14958, #3245, #5705 ),
 .UNSPECIFIED., .F., .T. ) 
 B_SPLINE_CURVE_WITH_KNOTS ( ( 3, 2, 2, 2, 3 ),
 ( 0.9027777777777777901, 0.9037037037037036757, 0.9055555555555555580, 0.9074074074074074403, 0.9083333333333333259 ),
 .UNSPECIFIED. ) 
 CURVE ( )  GEOMETRIC_REPRESENTATION_ITEM ( )  RATIONAL_B_SPLINE_CURVE ( ( 0.9330127018922194093, 0.9330127018922194093, 1.000000000000000000, 0.8660254037844388186, 1.000000000000000000, 0.8660254037844388186, 1.000000000000000000, 0.9330127018922194093, 0.9330127018922194093 ) ) 
 REPRESENTATION_ITEM ( '' )  );
#19021=CARTESIAN_POINT ( 'NONE',  ( -6.350852961085760029, -1.281975124255709124E-13, -172.1250000000000284 ) ) ;
#19023=CARTESIAN_POINT ( 'NONE',  ( -3.175426480542816510, -5.500000000000057732, -156.8750000000000284 ) ) ;
#19026=CARTESIAN_POINT ( 'NONE',  ( -5.999999999999963585, 1.780251999655701777E-13, -104.3363248654052313 ) ) ;
#19027=CARTESIAN_POINT ( 'NONE',  ( -2.775557561562891351E-14, -5.500000000000115463, -104.2500000000000142 ) ) ;
#19028=CARTESIAN_POINT ( 'NONE',  ( -5.999999999999963585, -1.487416814333745711E-14, -59.33632486540522422 ) ) ;
#19029=CARTESIAN_POINT ( 'NONE',  ( 4.763139720814407951, 2.750000000000002665, -156.2500000000000000 ) ) ;
#19030=CARTESIAN_POINT ( 'NONE',  ( 3.175426480543072749, -5.500000000000105693, -86.12500000000000000 ) ) ;
#19031=EDGE_CURVE ( 'NONE', #5164, #16308, #21421, .T. ) ;
#19039=LINE ( 'NONE', #3006, #21364 ) ;
#19040=ORIENTED_EDGE ( 'NONE', *, *, #5791, .F. ) ;
#19041=FILL_AREA_STYLE_COLOUR ( '', #2847 ) ;
#19047=ORIENTED_EDGE ( 'NONE', *, *, #23220, .T. ) ;
#19048=CARTESIAN_POINT ( 'NONE',  ( 3.175426480543072749, 5.499999999999865885, -109.6249999999999716 ) ) ;
#19050=CARTESIAN_POINT ( 'NONE',  ( -5.412658773652684552, -3.125000000000099920, -122.9330127018922809 ) ) ;
#19051=VERTEX_POINT ( 'NONE', #22940 ) ;
#19052=CARTESIAN_POINT ( 'NONE',  ( -3.464101615137725076, 5.999999999999979572, -57.16367513459482552 ) ) ;
#19053=CARTESIAN_POINT ( 'NONE',  ( -3.608439182435052128, -6.250000000000110134, -172.9419872981078470 ) ) ;
#19056=EDGE_CURVE ( 'NONE', #14326, #16412, #25211, .T. ) ;
#19058=CARTESIAN_POINT ( 'NONE',  ( -1.960615434941527013, 10.82557180451506973, -19.32589338774631926 ) ) ;
#19060=CARTESIAN_POINT ( 'NONE',  ( 4.763139720814407951, -2.749999999999988454, -176.0000000000000568 ) ) ;
#19062=CARTESIAN_POINT ( 'NONE',  ( 2.775557561562891351E-14, -6.250000000000061284, -173.6830127018922383 ) ) ;
#19063=CARTESIAN_POINT ( 'NONE',  ( -5.196152422706601826, 2.999999999999975131, -75.96132486540518869 ) ) ;
#19064=CIRCLE ( 'NONE', #21971, 11.00000000000001599 ) ;
#19066=CARTESIAN_POINT ( 'NONE',  ( 0.000000000000000000, 5.999999999999977796, -123.2886751345948539 ) ) ;
#19068=CARTESIAN_POINT ( 'NONE',  ( 4.763139720814407951, -2.749999999999988454, -112.9999999999999858 ) ) ;
#19069=CARTESIAN_POINT ( 'NONE',  ( -5.999999999999963585, -1.487416814333745711E-14, -59.91367513459483263 ) ) ;
#19070=CARTESIAN_POINT ( 'NONE',  ( -3.464101615137725076, 5.999999999999979572, -88.66367513459483973 ) ) ;
#19073=DIRECTION ( 'NONE',  ( 0.000000000000000000, 0.000000000000000000, -1.000000000000000000 ) ) ;
#19074=LINE ( 'NONE', #17214, #7221 ) ;
#19075=CARTESIAN_POINT ( 'NONE',  ( 0.000000000000000000, 5.999999999999977796, -155.7113248654052313 ) ) ;
#19076=ORIENTED_EDGE ( 'NONE', *, *, #9744, .T. ) ;
#19077=CARTESIAN_POINT ( 'NONE',  ( -5.999999999999963585, -1.487416814333745711E-14, -113.3363248654052029 ) ) ;
#19078=CARTESIAN_POINT ( 'NONE',  ( 3.464101615137852974, 5.999999999999884537, -109.9136751345947971 ) ) ;
#19080=CARTESIAN_POINT ( 'NONE',  ( 0.000000000000000000, 0.000000000000000000, 0.000000000000000000 ) ) ;
#19081=CARTESIAN_POINT ( 'NONE',  ( -5.196152422706601826, 2.999999999999975131, -141.0386751345948255 ) ) ;
#19083=VERTEX_POINT ( 'NONE', #8807 ) ;
#19084=CARTESIAN_POINT ( 'NONE',  ( 2.775557561562891351E-14, 6.250000000000033751, -139.0669872981078470 ) ) ;
#19087=LINE ( 'NONE', #28408, #22123 ) ;
#19092=CARTESIAN_POINT ( 'NONE',  ( -5.196152422706573404, -3.000000000000002665, -119.7886751345948397 ) ) ;
#19093=CARTESIAN_POINT ( 'NONE',  ( 0.000000000000000000, 5.999999999999977796, -92.71132486540523132 ) ) ;
#19094=CARTESIAN_POINT ( 'NONE',  ( -5.999999999999963585, -1.487416814333745711E-14, -59.91367513459483263 ) ) ;
#19096=ADVANCED_FACE ( 'NONE', ( #8487 ), #24606, .T. ) ;
#19099=ORIENTED_EDGE ( 'NONE', *, *, #14553, .F. ) ;
#19101=CARTESIAN_POINT ( 'NONE',  ( 0.000000000000000000, 5.999999999999977796, -62.71132486540520290 ) ) ;
#19106=CARTESIAN_POINT ( 'NONE',  ( 2.775557561562891351E-14, 6.250000000000033751, -104.5669872981078186 ) ) ;
#19108=( BOUNDED_CURVE ( )  B_SPLINE_CURVE ( 2, ( #25497, #6617, #2467, #14188, #2013, #9539, #4904, #20767, #30113 ),
 .UNSPECIFIED., .F., .F. ) 
 B_SPLINE_CURVE_WITH_KNOTS ( ( 3, 2, 2, 2, 3 ),
 ( 0.03611111111111110772, 0.03703703703703703498, 0.03888888888888888951, 0.04074074074074074403, 0.04166666666666667129 ),
 .UNSPECIFIED. ) 
 CURVE ( )  GEOMETRIC_REPRESENTATION_ITEM ( )  RATIONAL_B_SPLINE_CURVE ( ( 0.9330127018922194093, 0.9330127018922191873, 1.000000000000000000, 0.8660254037844388186, 1.000000000000000000, 0.8660254037844388186, 1.000000000000000000, 0.9330127018922191873, 0.9330127018922194093 ) ) 
 REPRESENTATION_ITEM ( '' )  );
#19110=CARTESIAN_POINT ( 'NONE',  ( -2.775557561562891351E-14, -5.500000000000115463, -131.2500000000000284 ) ) ;
#19111=ORIENTED_EDGE ( 'NONE', *, *, #7417, .F. ) ;
#19112=CARTESIAN_POINT ( 'NONE',  ( -6.350852961085760029, -1.281975124255709124E-13, -56.62500000000004974 ) ) ;
#19114=CARTESIAN_POINT ( 'NONE',  ( 6.000000000000007105, -1.607695154586741060, -179.2306624327026157 ) ) ;
#19117=CARTESIAN_POINT ( 'NONE',  ( 3.608439182435180470, 6.249999999999982236, -81.55801270189219565 ) ) ;
#19119=CARTESIAN_POINT ( 'NONE',  ( -3.464101615137757051, -5.999999999999979572, -176.0863248654052313 ) ) ;
#19123=CARTESIAN_POINT ( 'NONE',  ( 0.000000000000000000, 5.499999999999991118, -144.0000000000000284 ) ) ;
#19124=CARTESIAN_POINT ( 'NONE',  ( -5.196152422706573404, -3.000000000000002665, -105.7113248654052455 ) ) ;
#19125=CARTESIAN_POINT ( 'NONE',  ( -5.412658773652684552, -3.125000000000099920, -155.9330127018922383 ) ) ;
#19126=CARTESIAN_POINT ( 'NONE',  ( 5.999999999999897859, 1.607695154586893826, -117.0193375672974412 ) ) ;
#19127=CARTESIAN_POINT ( 'NONE',  ( -6.350852961085760029, -1.281975124255709124E-13, -68.62500000000002842 ) ) ;
#19128=CARTESIAN_POINT ( 'NONE',  ( 6.000000000000001776, 5.345404176511898156E-15, -174.0863248654052597 ) ) ;
#19129=CARTESIAN_POINT ( 'NONE',  ( 0.000000000000000000, 5.499999999999991118, -69.00000000000000000 ) ) ;
#19136=VECTOR ( 'NONE', #11737, 1000.000000000000000 ) ;
#19143=CARTESIAN_POINT ( 'NONE',  ( -3.175426480542816510, -5.500000000000057732, -180.8750000000000000 ) ) ;
#19145=CARTESIAN_POINT ( 'NONE',  ( 3.608439182435180470, -6.249999999999997335, -156.1919872981078470 ) ) ;
#19147=CARTESIAN_POINT ( 'NONE',  ( -4.763139720814407951, -2.750000000000016431, -82.00000000000001421 ) ) ;
#19150=CARTESIAN_POINT ( 'NONE',  ( -3.608439182435115633, 6.249999999999965361, -100.8080127018922383 ) ) ;
#19152=DIRECTION ( 'NONE',  ( -7.147005652999508048E-36, 5.642372883946980038E-36, 1.000000000000000000 ) ) ;
#19154=CARTESIAN_POINT ( 'NONE',  ( -5.999999999999963585, 1.780251999655701777E-13, -53.91367513459482552 ) ) ;
#19155=FACE_OUTER_BOUND ( 'NONE', #8430, .T. ) ;
#19158=( LENGTH_UNIT ( ) NAMED_UNIT ( * ) SI_UNIT ( .MILLI., .METRE. ) );
#19159=CARTESIAN_POINT ( 'NONE',  ( 6.350852961086080661, -9.614813431917819062E-14, -160.8750000000000284 ) ) ;
#19160=CARTESIAN_POINT ( 'NONE',  ( -5.999999999999963585, 8.134310703387671600E-14, -142.4136751345948539 ) ) ;
#19161=CARTESIAN_POINT ( 'NONE',  ( -3.175426480542816510, 5.499999999999865885, -155.8750000000000000 ) ) ;
#19163=CARTESIAN_POINT ( 'NONE',  ( -6.000000000000007105, -1.607695154586655129, -52.34668783648703538 ) ) ;
#19164=CARTESIAN_POINT ( 'NONE',  ( -4.763139720814407951, -2.750000000000016431, -94.00000000000002842 ) ) ;
#19165=CARTESIAN_POINT ( 'NONE',  ( 5.999999999999949374, 1.607695154586804565, -60.01933756729743408 ) ) ;
#19166=CARTESIAN_POINT ( 'NONE',  ( 6.350852961086080661, -9.614813431917819062E-14, -87.37500000000007105 ) ) ;
#19168=CARTESIAN_POINT ( 'NONE',  ( 0.000000000000000000, 0.000000000000000000, 0.000000000000000000 ) ) ;
#19173=CARTESIAN_POINT ( 'NONE',  ( 0.000000000000000000, 0.000000000000000000, 0.000000000000000000 ) ) ;
#19174=ORIENTED_EDGE ( 'NONE', *, *, #22997, .F. ) ;
#19175=CARTESIAN_POINT ( 'NONE',  ( 6.000000000000001776, 5.345404176511898156E-15, -179.1636751345948255 ) ) ;
#19179=AXIS2_PLACEMENT_3D ( 'NONE', #25469, #18446, #11073 ) ;
#19180=ORIENTED_EDGE ( 'NONE', *, *, #18028, .F. ) ;
#19181=ORIENTED_EDGE ( 'NONE', *, *, #4836, .F. ) ;
#19182=CARTESIAN_POINT ( 'NONE',  ( 3.175426480543072749, 5.499999999999865885, -112.6249999999999858 ) ) ;
#19184=EDGE_CURVE ( 'NONE', #9277, #11496, #10668, .T. ) ;
#19185=CARTESIAN_POINT ( 'NONE',  ( -3.608439182435052128, -6.250000000000110134, -122.8080127018922099 ) ) ;
#19189=CARTESIAN_POINT ( 'NONE',  ( 7.216878364870455975, -6.409875621278545621E-14, -164.9419872981078186 ) ) ;
#19191=ORIENTED_EDGE ( 'NONE', *, *, #28736, .F. ) ;
#19193=CARTESIAN_POINT ( 'NONE',  ( 6.000000000000052403, -1.607695154586662678, -132.1533121635129646 ) ) ;
#19194=CARTESIAN_POINT ( 'NONE',  ( 3.175426480543072749, 5.499999999999865885, -175.6250000000000284 ) ) ;
#19196=CARTESIAN_POINT ( 'NONE',  ( 5.196152422706629359, -2.999999999999988898, -168.7886751345948255 ) ) ;
#19197=CARTESIAN_POINT ( 'NONE',  ( 5.412658773652739619, 3.124999999999988898, -180.6830127018922383 ) ) ;
#19198=CARTESIAN_POINT ( 'NONE',  ( 5.999999999999949374, 1.607695154586804565, -76.51933756729745539 ) ) ;
#19200=CARTESIAN_POINT ( 'NONE',  ( -4.763139720814407951, 2.749999999999946709, -127.2500000000000284 ) ) ;
#19202=CARTESIAN_POINT ( 'NONE',  ( -3.175426480542816510, -5.500000000000057732, -110.3750000000000426 ) ) ;
#19204=ORIENTED_EDGE ( 'NONE', *, *, #24850, .F. ) ;
#19205=CARTESIAN_POINT ( 'NONE',  ( 6.000000000000000888, -3.330669073875464691E-16, -7.560779664488942560E-35 ) ) ;
#19209=EDGE_CURVE ( 'NONE', #5164, #1, #24770, .T. ) ;
#19213=EDGE_CURVE ( 'NONE', #13234, #12154, #6327, .T. ) ;
#19214=CARTESIAN_POINT ( 'NONE',  ( 0.000000000000000000, 5.999999999999977796, -109.7886751345948397 ) ) ;
#19215=ORIENTED_EDGE ( 'NONE', *, *, #1151, .F. ) ;
#19219=CARTESIAN_POINT ( 'NONE',  ( 3.464101615137852974, 5.999999999999884537, -85.33632486540520290 ) ) ;
#19222=ADVANCED_FACE ( 'NONE', ( #6025 ), #13145, .T. ) ;
#19223=EDGE_LOOP ( 'NONE', ( #13967, #7312, #3151, #22330 ) ) ;
#19224=CARTESIAN_POINT ( 'NONE',  ( 7.216878364870455975, -6.409875621278545621E-14, -131.9419872981078470 ) ) ;
#19236=CARTESIAN_POINT ( 'NONE',  ( -5.999999999999904965, -1.607695154586834541, -140.2693375672974412 ) ) ;
#19238=CARTESIAN_POINT ( 'NONE',  ( -5.999999999999962697, 3.323446944526963260E-14, -162.8363248654052313 ) ) ;
#19241=CARTESIAN_POINT ( 'NONE',  ( 6.350852961086080661, -9.614813431917819062E-14, -139.8750000000000568 ) ) ;
#19244=ORIENTED_EDGE ( 'NONE', *, *, #17740, .T. ) ;
#19246=CARTESIAN_POINT ( 'NONE',  ( -3.175426480542816066, 5.499999999999865885, -47.87500000000000000 ) ) ;
#19247=CARTESIAN_POINT ( 'NONE',  ( -5.196152422706601826, 2.999999999999975131, -152.4613248654052029 ) ) ;
#19250=CARTESIAN_POINT ( 'NONE',  ( 6.000000000000000888, -1.859271017917181981E-14, -93.08632486540523132 ) ) ;
#19253=CARTESIAN_POINT ( 'NONE',  ( 7.216878364870455975, -6.409875621278545621E-14, -101.9419872981078328 ) ) ;
#19257=EDGE_CURVE ( 'NONE', #18433, #16280, #21244, .T. ) ;
#19258=CARTESIAN_POINT ( 'NONE',  ( -4.763139720814407951, 2.749999999999946709, -127.2500000000000284 ) ) ;
#19259=EDGE_CURVE ( 'NONE', #23968, #20807, #230, .T. ) ;
#19260=ORIENTED_EDGE ( 'NONE', *, *, #19661, .T. ) ;
#19262=CARTESIAN_POINT ( 'NONE',  ( 0.000000000000000000, 5.499999999999991118, -54.00000000000004974 ) ) ;
#19264=CARTESIAN_POINT ( 'NONE',  ( -6.000000000000000888, 1.067854986875958443E-15, 7.560779664488942560E-35 ) ) ;
#19265=CARTESIAN_POINT ( 'NONE',  ( -3.608439182435052128, -6.250000000000110134, -86.80801270189222407 ) ) ;
#19266=UNCERTAINTY_MEASURE_WITH_UNIT (LENGTH_MEASURE( 1.000000000000000082E-05 ), #19158, 'distance_accuracy_value', 'NONE');
#19267=DIRECTION ( 'NONE',  ( -7.147005652999508048E-36, 5.642372883946980038E-36, 1.000000000000000000 ) ) ;
#19271=CARTESIAN_POINT ( 'NONE',  ( -5.999999999999963585, 8.134310703387671600E-14, -114.8363248654052171 ) ) ;
#19272=CARTESIAN_POINT ( 'NONE',  ( -3.464101615137725076, 5.999999999999979572, -61.08632486540521711 ) ) ;
#19275=CARTESIAN_POINT ( 'NONE',  ( 4.763139720814407951, -2.749999999999988454, -137.0000000000000000 ) ) ;
#19277=CARTESIAN_POINT ( 'NONE',  ( 2.775557561562891351E-14, 6.250000000000033751, -151.9330127018922383 ) ) ;
#19279=CARTESIAN_POINT ( 'NONE',  ( 5.196152422706629359, -2.999999999999988898, -72.78867513459485394 ) ) ;
#19280=CARTESIAN_POINT ( 'NONE',  ( 4.763139720814407951, 2.750000000000002665, -72.25000000000004263 ) ) ;
#19281=CARTESIAN_POINT ( 'NONE',  ( -3.175426480542816510, 5.499999999999865885, -65.87500000000002842 ) ) ;
#19282=( BOUNDED_CURVE ( )  B_SPLINE_CURVE ( 2, ( #6842, #14119, #23153, #82, #22992, #30346, #16268, #23457, #25586 ),
 .UNSPECIFIED., .F., .T. ) 
 B_SPLINE_CURVE_WITH_KNOTS ( ( 3, 2, 2, 2, 3 ),
 ( 0.7138888888888887951, 0.7148148148148147918, 0.7166666666666666741, 0.7185185185185185563, 0.7194444444444444420 ),
 .UNSPECIFIED. ) 
 CURVE ( )  GEOMETRIC_REPRESENTATION_ITEM ( )  RATIONAL_B_SPLINE_CURVE ( ( 0.9330127018922194093, 0.9330127018922154125, 1.000000000000000000, 0.8660254037844388186, 1.000000000000000000, 0.8660254037844388186, 1.000000000000000000, 0.9330127018922194093, 0.9330127018922194093 ) ) 
 REPRESENTATION_ITEM ( '' )  );
#19285=FACE_OUTER_BOUND ( 'NONE', #23353, .T. ) ;
#19287=CARTESIAN_POINT ( 'NONE',  ( -6.000000000000000888, 1.067854986875958443E-15, 7.560779664488942560E-35 ) ) ;
#19295=CARTESIAN_POINT ( 'NONE',  ( 2.775557561562891351E-14, 6.250000000000033751, -46.06698729810781856 ) ) ;
#19298=CARTESIAN_POINT ( 'NONE',  ( 4.763139720814407951, 2.750000000000002665, -78.25000000000004263 ) ) ;
#19299=CARTESIAN_POINT ( 'NONE',  ( -5.412658773652739619, 3.124999999999975131, -100.6830127018922241 ) ) ;
#19302=CARTESIAN_POINT ( 'NONE',  ( 3.175426480543072749, -5.500000000000105693, -168.6250000000000000 ) ) ;
#19304=CARTESIAN_POINT ( 'NONE',  ( 0.000000000000000000, 0.000000000000000000, 0.000000000000000000 ) ) ;
#19305=CARTESIAN_POINT ( 'NONE',  ( -5.196152422706573404, -3.000000000000002665, -59.21132486540525974 ) ) ;
#19307=CARTESIAN_POINT ( 'NONE',  ( 4.763139720814407951, -2.749999999999988454, -162.5000000000000284 ) ) ;
#19309=CARTESIAN_POINT ( 'NONE',  ( -4.763139720814407951, -2.750000000000016431, -154.0000000000000284 ) ) ;
#19310=VECTOR ( 'NONE', #12910, 1000.000000000000000 ) ;
#19311=CARTESIAN_POINT ( 'NONE',  ( -5.999999999999963585, -1.487416814333745711E-14, -76.41367513459481131 ) ) ;
#19313=CARTESIAN_POINT ( 'NONE',  ( 0.000000000000000000, 5.499999999999991118, -93.00000000000002842 ) ) ;
#19314=CARTESIAN_POINT ( 'NONE',  ( 0.000000000000000000, 5.999999999999977796, -125.7113248654052597 ) ) ;
#19316=CARTESIAN_POINT ( 'NONE',  ( 6.350852961086080661, -9.614813431917819062E-14, -93.37500000000001421 ) ) ;
#19319=( BOUNDED_CURVE ( )  B_SPLINE_CURVE ( 2, ( #25977, #14350, #23690, #17495, #16803, #17808, #24680, #23835, #3320 ),
 .UNSPECIFIED., .F., .F. ) 
 B_SPLINE_CURVE_WITH_KNOTS ( ( 3, 2, 2, 2, 3 ),
 ( 0.6083333333333333925, 0.6092592592592592782, 0.6111111111111111605, 0.6129629629629629317, 0.6138888888888888173 ),
 .UNSPECIFIED. ) 
 CURVE ( )  GEOMETRIC_REPRESENTATION_ITEM ( )  RATIONAL_B_SPLINE_CURVE ( ( 0.9330127018922194093, 0.9330127018922234061, 1.000000000000000000, 0.8660254037844388186, 1.000000000000000000, 0.8660254037844388186, 1.000000000000000000, 0.9330127018922234061, 0.9330127018922194093 ) ) 
 REPRESENTATION_ITEM ( '' )  );
#19322=DIRECTION ( 'NONE',  ( -7.147005652999508048E-36, 5.642372883946980038E-36, 1.000000000000000000 ) ) ;
#19328=DIRECTION ( 'NONE',  ( -7.147005652999508048E-36, 5.642372883946980038E-36, 1.000000000000000000 ) ) ;
#19332=ORIENTED_EDGE ( 'NONE', *, *, #24184, .F. ) ;
#19335=CARTESIAN_POINT ( 'NONE',  ( 4.763139720814407951, -2.749999999999988454, -107.0000000000000426 ) ) ;
#19337=CARTESIAN_POINT ( 'NONE',  ( 5.412658773652712085, -3.125000000000086153, -123.9330127018922809 ) ) ;
#19339=DIRECTION ( 'NONE',  ( 1.000000000000000000, -5.551115123125773458E-17, -1.260129944081490338E-35 ) ) ;
#19340=CARTESIAN_POINT ( 'NONE',  ( -5.412658773652739619, 3.124999999999975131, -158.3169872981078470 ) ) ;
#19343=CARTESIAN_POINT ( 'NONE',  ( 2.775557561562891351E-14, 6.250000000000033751, -60.43301270189227381 ) ) ;
#19346=CARTESIAN_POINT ( 'NONE',  ( 3.464101615137757051, -5.999999999999979572, -132.3363248654052313 ) ) ;
#19348=CARTESIAN_POINT ( 'NONE',  ( 6.350852961086080661, -9.614813431917819062E-14, -180.3750000000000284 ) ) ;
#19350=CARTESIAN_POINT ( 'NONE',  ( -5.999999999999963585, 1.780251999655701777E-13, -99.83632486540521711 ) ) ;
#19351=CARTESIAN_POINT ( 'NONE',  ( 3.608439182435180470, 6.249999999999982236, -180.5580127018922383 ) ) ;
#19352=CARTESIAN_POINT ( 'NONE',  ( 5.196152422706629359, -2.999999999999988898, -101.2886751345948255 ) ) ;
#19353=CARTESIAN_POINT ( 'NONE',  ( 4.763139720814407951, 2.750000000000002665, -114.2500000000000142 ) ) ;
#19355=CARTESIAN_POINT ( 'NONE',  ( -4.763139720814407951, 2.749999999999946709, -112.2500000000000142 ) ) ;
#19361=CARTESIAN_POINT ( 'NONE',  ( -5.999999999999963585, -1.487416814333745711E-14, -167.9136751345948255 ) ) ;
#19364=ORIENTED_EDGE ( 'NONE', *, *, #9114, .F. ) ;
#19365=CARTESIAN_POINT ( 'NONE',  ( 3.175426480543072749, -5.500000000000105693, -176.1250000000000284 ) ) ;
#19369=( BOUNDED_CURVE ( )  B_SPLINE_CURVE ( 2, ( #11603, #6794, #22788, #20945, #1730, #2199, #16217, #25216, #8811 ),
 .UNSPECIFIED., .F., .T. ) 
 B_SPLINE_CURVE_WITH_KNOTS ( ( 3, 2, 2, 2, 3 ),
 ( 0.5749999999999999556, 0.5759259259259259522, 0.5777777777777777235, 0.5796296296296296058, 0.5805555555555554914 ),
 .UNSPECIFIED. ) 
 CURVE ( )  GEOMETRIC_REPRESENTATION_ITEM ( )  RATIONAL_B_SPLINE_CURVE ( ( 0.9330127018922194093, 0.9330127018922154125, 1.000000000000000000, 0.8660254037844388186, 1.000000000000000000, 0.8660254037844388186, 1.000000000000000000, 0.9330127018922234061, 0.9330127018922194093 ) ) 
 REPRESENTATION_ITEM ( '' )  );
#19370=ORIENTED_EDGE ( 'NONE', *, *, #23211, .F. ) ;
#19374=CARTESIAN_POINT ( 'NONE',  ( 3.608439182435180470, 6.249999999999982236, -134.6919872981078470 ) ) ;
#19376=CARTESIAN_POINT ( 'NONE',  ( -5.999999999999919176, 1.607695154586804565, -83.40331216351300725 ) ) ;
#19381=CYLINDRICAL_SURFACE ( 'NONE', #20108, 6.000000000000000888 ) ;
#19384=DIRECTION ( 'NONE',  ( -7.147005652999508048E-36, 5.642372883946980038E-36, 1.000000000000000000 ) ) ;
#19385=CARTESIAN_POINT ( 'NONE',  ( 6.000000000000000888, 7.762456499804234384E-14, -139.5863248654051745 ) ) ;
#19387=CARTESIAN_POINT ( 'NONE',  ( -3.464101615137757051, -5.999999999999979572, -162.5863248654052313 ) ) ;
#19388=CARTESIAN_POINT ( 'NONE',  ( 6.000000000000052403, -1.607695154586662678, -69.15331216351300725 ) ) ;
#19390=CARTESIAN_POINT ( 'NONE',  ( -5.999999999999963585, -1.487416814333745711E-14, -143.3363248654052029 ) ) ;
#19391=CARTESIAN_POINT ( 'NONE',  ( -4.763139720814407951, -2.750000000000016431, -136.0000000000000000 ) ) ;
#19395=VECTOR ( 'NONE', #17462, 1000.000000000000000 ) ;
#19399=EDGE_CURVE ( 'NONE', #28019, #87, #19979, .T. ) ;
#19400=ORIENTED_EDGE ( 'NONE', *, *, #11894, .T. ) ;
#19403=CARTESIAN_POINT ( 'NONE',  ( -7.216878364870328078, 0.000000000000000000, -93.69198729810780435 ) ) ;
#19404=CARTESIAN_POINT ( 'NONE',  ( 3.464101615137852974, 5.999999999999884537, -172.9136751345947971 ) ) ;
#19407=DIRECTION ( 'NONE',  ( 1.000000000000000000, -5.551115123125773458E-17, -1.260129944081490338E-35 ) ) ;
#19408=CARTESIAN_POINT ( 'NONE',  ( -6.350852961085760029, -1.281975124255709124E-13, -127.1249999999999858 ) ) ;
#19409=ORIENTED_EDGE ( 'NONE', *, *, #24974, .T. ) ;
#19410=CARTESIAN_POINT ( 'NONE',  ( -5.999999999999963585, 1.780251999655701777E-13, -95.91367513459483973 ) ) ;
#19412=CARTESIAN_POINT ( 'NONE',  ( 0.000000000000000000, 5.499999999999991118, -57.00000000000004974 ) ) ;
#19413=( BOUNDED_CURVE ( )  B_SPLINE_CURVE ( 2, ( #17992, #3656, #24713, #11068, #8588, #18292, #13092, #15857, #4277 ),
 .UNSPECIFIED., .F., .F. ) 
 B_SPLINE_CURVE_WITH_KNOTS ( ( 3, 2, 2, 2, 3 ),
 ( 0.08055555555555549141, 0.08148148148148148806, 0.08333333333333337034, 0.08518518518518514160, 0.08611111111111113825 ),
 .UNSPECIFIED. ) 
 CURVE ( )  GEOMETRIC_REPRESENTATION_ITEM ( )  RATIONAL_B_SPLINE_CURVE ( ( 0.9330127018922194093, 0.9330127018922154125, 1.000000000000000000, 0.8660254037844388186, 1.000000000000000000, 0.8660254037844388186, 1.000000000000000000, 0.9330127018922154125, 0.9330127018922194093 ) ) 
 REPRESENTATION_ITEM ( '' )  );
#19414=CARTESIAN_POINT ( 'NONE',  ( 5.196152422706629359, 3.000000000000002665, -116.0386751345948113 ) ) ;
#19415=CARTESIAN_POINT ( 'NONE',  ( 5.999999999999949374, 1.607695154586804565, -66.59668783648703538 ) ) ;
#19416=CARTESIAN_POINT ( 'NONE',  ( -3.464101615137725076, 5.999999999999979572, -67.66367513459479710 ) ) ;
#19417=CARTESIAN_POINT ( 'NONE',  ( -3.608439182435115633, 6.249999999999965361, -82.80801270189226670 ) ) ;
#19420=CARTESIAN_POINT ( 'NONE',  ( 6.000000000000000000, 2.951592740943527306E-14, -153.6636751345948539 ) ) ;
#19422=CARTESIAN_POINT ( 'NONE',  ( 0.000000000000000000, 0.000000000000000000, -180.0000000000000568 ) ) ;
#19424=CARTESIAN_POINT ( 'NONE',  ( 6.350852961086080661, -9.614813431917819062E-14, -142.8750000000000568 ) ) ;
#19426=CARTESIAN_POINT ( 'NONE',  ( 5.412658773652712085, -3.125000000000086153, -156.9330127018922383 ) ) ;
#19427=CARTESIAN_POINT ( 'NONE',  ( -5.196152422706573404, -3.000000000000002665, -71.21132486540521711 ) ) ;
#19428=CARTESIAN_POINT ( 'NONE',  ( -5.999999999999971578, 1.607695154586715303, -66.90331216351303567 ) ) ;
#19429=CARTESIAN_POINT ( 'NONE',  ( 6.350852961086080661, -9.614813431917819062E-14, -69.37500000000004263 ) ) ;
#19431=CARTESIAN_POINT ( 'NONE',  ( -6.350852961085760029, -1.281975124255709124E-13, -56.62500000000004974 ) ) ;
#19436=CARTESIAN_POINT ( 'NONE',  ( 6.000000000000000888, -1.859271017917181981E-14, -59.16367513459483263 ) ) ;
#19438=VECTOR ( 'NONE', #11958, 1000.000000000000000 ) ;
#19439=CARTESIAN_POINT ( 'NONE',  ( 6.000000000000052403, -1.607695154586662678, -104.2306624327026299 ) ) ;
#19446=ORIENTED_EDGE ( 'NONE', *, *, #13878, .T. ) ;
#19447=CARTESIAN_POINT ( 'NONE',  ( 4.763139720814407951, -2.749999999999988454, -83.00000000000001421 ) ) ;
#19450=CARTESIAN_POINT ( 'NONE',  ( 6.000000000000000888, -1.607695154586752384, -127.6533121635130215 ) ) ;
#19451=VECTOR ( 'NONE', #14893, 1000.000000000000000 ) ;
#19452=EDGE_CURVE ( 'NONE', #4894, #29768, #10850, .T. ) ;
#19453=FACE_OUTER_BOUND ( 'NONE', #10016, .T. ) ;
#19454=CARTESIAN_POINT ( 'NONE',  ( 1.384933631640856255, -10.91424797897491139, -19.15860252534411146 ) ) ;
#19457=CARTESIAN_POINT ( 'NONE',  ( 3.175426480543072749, 5.499999999999865885, -163.6249999999999716 ) ) ;
#19458=CARTESIAN_POINT ( 'NONE',  ( -5.196152422706573404, -3.000000000000002665, -60.71132486540520290 ) ) ;
#19459=CARTESIAN_POINT ( 'NONE',  ( 3.175426480543072749, 5.499999999999865885, -150.1250000000000284 ) ) ;
#19461=CARTESIAN_POINT ( 'NONE',  ( 3.175426480543072749, -5.500000000000105693, -93.62500000000002842 ) ) ;
#19463=EDGE_CURVE ( 'NONE', #3196, #22419, #3347, .T. ) ;
#19464=CARTESIAN_POINT ( 'NONE',  ( 0.000000000000000000, 5.499999999999991118, -91.50000000000002842 ) ) ;
#19466=CYLINDRICAL_SURFACE ( 'NONE', #4722, 6.000000000000000888 ) ;
#19469=CARTESIAN_POINT ( 'NONE',  ( -5.196152422706573404, -3.000000000000002665, -66.71132486540520290 ) ) ;
#19470=CARTESIAN_POINT ( 'NONE',  ( -5.196152422706573404, -3.000000000000002665, -74.21132486540521711 ) ) ;
#19473=LINE ( 'NONE', #718, #10716 ) ;
#19474=CARTESIAN_POINT ( 'NONE',  ( 0.000000000000000000, 5.999999999999977796, -82.78867513459481131 ) ) ;
#19478=CARTESIAN_POINT ( 'NONE',  ( -4.763139720814407951, -2.750000000000016431, -103.0000000000000426 ) ) ;
#19480=CARTESIAN_POINT ( 'NONE',  ( 7.216878364870455975, -6.409875621278545621E-14, -119.3080127018922525 ) ) ;
#19481=ORIENTED_EDGE ( 'NONE', *, *, #9213, .F. ) ;
#19482=CARTESIAN_POINT ( 'NONE',  ( 6.350852961086080661, -9.614813431917819062E-14, -151.8749999999999716 ) ) ;
#19484=CARTESIAN_POINT ( 'NONE',  ( 2.775557561562891351E-14, -6.250000000000061284, -160.8169872981078470 ) ) ;
#19489=CARTESIAN_POINT ( 'NONE',  ( 7.216878364870455975, -6.409875621278545621E-14, -56.30801270189227381 ) ) ;
#19492=EDGE_CURVE ( 'NONE', #9960, #22916, #13925, .T. ) ;
#19493=CARTESIAN_POINT ( 'NONE',  ( -5.990257846049534152, 9.225907948257358271, -24.60347258678507743 ) ) ;
#19494=CARTESIAN_POINT ( 'NONE',  ( 6.350852961086080661, -9.614813431917819062E-14, -168.3750000000000568 ) ) ;
#19496=CARTESIAN_POINT ( 'NONE',  ( 6.000000000000052403, -1.607695154586662678, -112.6533121635129930 ) ) ;
#19497=CARTESIAN_POINT ( 'NONE',  ( 3.608439182435180470, -6.249999999999997335, -167.5580127018922099 ) ) ;
#19500=CARTESIAN_POINT ( 'NONE',  ( 3.175426480543072749, -5.500000000000105693, -119.1250000000000284 ) ) ;
#19501=CARTESIAN_POINT ( 'NONE',  ( 3.175426480543072749, 5.499999999999865885, -115.6250000000000142 ) ) ;
#19503=CIRCLE ( 'NONE', #20975, 6.000000000000009770 ) ;
#19508=CARTESIAN_POINT ( 'NONE',  ( -5.999999999999963585, 1.780251999655701777E-13, -108.8363248654052313 ) ) ;
#19510=CARTESIAN_POINT ( 'NONE',  ( -5.999999999999963585, 1.780251999655701777E-13, -86.33632486540524553 ) ) ;
#19513=CARTESIAN_POINT ( 'NONE',  ( 3.175426480543072749, -5.500000000000105693, -179.1250000000000568 ) ) ;
#19514=CARTESIAN_POINT ( 'NONE',  ( -5.412658773652739619, 3.124999999999975131, -81.81698729810781856 ) ) ;
#19515=ORIENTED_EDGE ( 'NONE', *, *, #25685, .T. ) ;
#19516=CARTESIAN_POINT ( 'NONE',  ( -3.464101615137725076, 5.999999999999979572, -144.1636751345948255 ) ) ;
#19518=VERTEX_POINT ( 'NONE', #5340 ) ;
#19519=VERTEX_POINT ( 'NONE', #17061 ) ;
#19520=CARTESIAN_POINT ( 'NONE',  ( -5.196152422706601826, 2.999999999999975131, -84.96132486540520290 ) ) ;
#19522=ORIENTED_EDGE ( 'NONE', *, *, #6016, .F. ) ;
#19523=CARTESIAN_POINT ( 'NONE',  ( -5.412658773652739619, 3.124999999999975131, -132.8169872981078186 ) ) ;
#19524=CARTESIAN_POINT ( 'NONE',  ( 3.464101615137852974, 5.999999999999884537, -49.91367513459485394 ) ) ;
#19529=CARTESIAN_POINT ( 'NONE',  ( -5.999999999999956479, -1.607695154586745057, -139.3466878364870638 ) ) ;
#19530=EDGE_CURVE ( 'NONE', #22297, #13381, #7952, .T. ) ;
#19537=CARTESIAN_POINT ( 'NONE',  ( -2.775557561562891351E-14, -5.500000000000115463, -138.7500000000000284 ) ) ;
#19538=AXIS2_PLACEMENT_3D ( 'NONE', #16888, #16742, #26067 ) ;
#19539=CARTESIAN_POINT ( 'NONE',  ( 0.000000000000000000, 5.999999999999977796, -166.7886751345948255 ) ) ;
#19540=ORIENTED_EDGE ( 'NONE', *, *, #1712, .F. ) ;
#19541=CARTESIAN_POINT ( 'NONE',  ( -6.350852961085760029, -1.281975124255709124E-13, -49.12500000000000711 ) ) ;
#19545=ORIENTED_EDGE ( 'NONE', *, *, #4663, .F. ) ;
#19549=CARTESIAN_POINT ( 'NONE',  ( -5.412658773652684552, -3.125000000000099920, -93.56698729810780435 ) ) ;
#19552=CARTESIAN_POINT ( 'NONE',  ( 5.999999999999949374, 1.607695154586804565, -78.01933756729742697 ) ) ;
#19554=CARTESIAN_POINT ( 'NONE',  ( 3.175426480543072749, 5.499999999999865885, -127.6249999999999858 ) ) ;
#19555=ORIENTED_EDGE ( 'NONE', *, *, #1551, .T. ) ;
#19556=CARTESIAN_POINT ( 'NONE',  ( 6.000000000000000888, 1.743066579297358182E-13, -82.58632486540520290 ) ) ;
#19557=CARTESIAN_POINT ( 'NONE',  ( -6.350852961085760029, -1.281975124255709124E-13, -53.62500000000002842 ) ) ;
#19558=CARTESIAN_POINT ( 'NONE',  ( 3.464101615137852974, 5.999999999999884537, -69.41367513459479710 ) ) ;
#19559=CARTESIAN_POINT ( 'NONE',  ( -5.196152422706573404, -3.000000000000002665, -134.7886751345947971 ) ) ;
#19560=CARTESIAN_POINT ( 'NONE',  ( 5.803206942314543149, 9.345129262100543954, -26.57517091834634826 ) ) ;
#19561=CARTESIAN_POINT ( 'NONE',  ( 3.608439182435180470, -6.249999999999997335, -74.55801270189223828 ) ) ;
#19566=CARTESIAN_POINT ( 'NONE',  ( 0.000000000000000000, 5.999999999999977796, -61.21132486540520290 ) ) ;
#19567=CARTESIAN_POINT ( 'NONE',  ( 4.763139720814407951, -2.749999999999988454, -140.0000000000000000 ) ) ;
#19569=CARTESIAN_POINT ( 'NONE',  ( 3.608439182435180470, 6.249999999999982236, -153.5580127018922383 ) ) ;
#19570=CARTESIAN_POINT ( 'NONE',  ( 0.000000000000000000, 5.999999999999977796, -101.7113248654052455 ) ) ;
#19571=CARTESIAN_POINT ( 'NONE',  ( 5.999999999999949374, 1.607695154586804565, -51.59668783648704959 ) ) ;
#19572=CARTESIAN_POINT ( 'NONE',  ( -6.350852961085760029, -1.281975124255709124E-13, -73.12500000000007105 ) ) ;
#19573=CARTESIAN_POINT ( 'NONE',  ( -3.175426480542816510, 5.499999999999865885, -56.87500000000004974 ) ) ;
#19577=CARTESIAN_POINT ( 'NONE',  ( -3.464101615137725076, 5.999999999999979572, -133.6636751345948539 ) ) ;
#19578=CARTESIAN_POINT ( 'NONE',  ( 6.000000000000052403, -1.607695154586662678, -57.73066243270260145 ) ) ;
#19583=( BOUNDED_CURVE ( )  B_SPLINE_CURVE ( 2, ( #388, #28935, #7898, #5739, #9931, #12557, #19305, #697, #17313 ),
 .UNSPECIFIED., .F., .F. ) 
 B_SPLINE_CURVE_WITH_KNOTS ( ( 3, 2, 2, 2, 3 ),
 ( 0.09166666666666667407, 0.09259259259259255970, 0.09444444444444444198, 0.09629629629629632426, 0.09722222222222220989 ),
 .UNSPECIFIED. ) 
 CURVE ( )  GEOMETRIC_REPRESENTATION_ITEM ( )  RATIONAL_B_SPLINE_CURVE ( ( 0.9330127018922194093, 0.9330127018922194093, 1.000000000000000000, 0.8660254037844388186, 1.000000000000000000, 0.8660254037844388186, 1.000000000000000000, 0.9330127018922194093, 0.9330127018922194093 ) ) 
 REPRESENTATION_ITEM ( '' )  );
#19585=VECTOR ( 'NONE', #8727, 1000.000000000000000 ) ;
#19586=CARTESIAN_POINT ( 'NONE',  ( -2.775557561562891351E-14, -5.500000000000115463, -176.2500000000000284 ) ) ;
#19588=CARTESIAN_POINT ( 'NONE',  ( 2.775557561562891351E-14, 6.250000000000033751, -149.5669872981077901 ) ) ;
#19590=CARTESIAN_POINT ( 'NONE',  ( 3.175426480543072749, 5.499999999999865885, -81.12500000000002842 ) ) ;
#19591=EDGE_CURVE ( 'NONE', #13461, #23373, #24530, .T. ) ;
#19592=CARTESIAN_POINT ( 'NONE',  ( 3.608439182435180470, 6.249999999999982236, -98.05801270189220986 ) ) ;
#19593=CARTESIAN_POINT ( 'NONE',  ( -5.999999999999963585, -1.487416814333745711E-14, -106.4136751345948113 ) ) ;
#19594=CARTESIAN_POINT ( 'NONE',  ( -5.999999999999956479, -1.607695154586745057, -96.76933756729742697 ) ) ;
#19595=CYLINDRICAL_SURFACE ( 'NONE', #29784, 6.000000000000000888 ) ;
#19598=CARTESIAN_POINT ( 'NONE',  ( -3.175426480542816066, 5.499999999999865885, -167.8750000000000568 ) ) ;
#19600=CARTESIAN_POINT ( 'NONE',  ( 0.000000000000000000, 5.499999999999991118, -144.0000000000000284 ) ) ;
#19602=CARTESIAN_POINT ( 'NONE',  ( -4.763139720814407951, -2.750000000000016431, -91.00000000000002842 ) ) ;
#19605=CARTESIAN_POINT ( 'NONE',  ( 3.175426480543072749, 5.499999999999865885, -84.12499999999997158 ) ) ;
#19607=CARTESIAN_POINT ( 'NONE',  ( 6.000000000000000888, 7.762456499804234384E-14, -144.0863248654052313 ) ) ;
#19609=CARTESIAN_POINT ( 'NONE',  ( 5.196152422706629359, -2.999999999999988898, -73.71132486540521711 ) ) ;
#19612=CYLINDRICAL_SURFACE ( 'NONE', #28817, 6.000000000000000888 ) ;
#19615=EDGE_CURVE ( 'NONE', #26795, #17525, #12825, .T. ) ;
#19616=ORIENTED_EDGE ( 'NONE', *, *, #28247, .F. ) ;
#19617=( BOUNDED_CURVE ( )  B_SPLINE_CURVE ( 2, ( #24197, #24806, #8370, #19744, #10393, #17166, #5595, #14998, #19899 ),
 .UNSPECIFIED., .F., .F. ) 
 B_SPLINE_CURVE_WITH_KNOTS ( ( 3, 2, 2, 2, 3 ),
 ( 0.6250000000000000000, 0.6259259259259259967, 0.6277777777777777679, 0.6296296296296296502, 0.6305555555555555358 ),
 .UNSPECIFIED. ) 
 CURVE ( )  GEOMETRIC_REPRESENTATION_ITEM ( )  RATIONAL_B_SPLINE_CURVE ( ( 0.9330127018922194093, 0.9330127018922194093, 1.000000000000000000, 0.8660254037844388186, 1.000000000000000000, 0.8660254037844388186, 1.000000000000000000, 0.9330127018922234061, 0.9330127018922194093 ) ) 
 REPRESENTATION_ITEM ( '' )  );
#19619=EDGE_LOOP ( 'NONE', ( #14338, #17364, #1198, #1591, #16072, #4787, #15217, #16928 ) ) ;
#19620=CARTESIAN_POINT ( 'NONE',  ( 4.763139720814407951, 2.750000000000002665, -106.7500000000000142 ) ) ;
#19623=CARTESIAN_POINT ( 'NONE',  ( -7.216878364870328078, 0.000000000000000000, -121.5580127018922809 ) ) ;
#19624=( BOUNDED_CURVE ( )  B_SPLINE_CURVE ( 2, ( #9250, #11747, #27964, #18348, #25521, #25361, #4630, #4331, #23252 ),
 .UNSPECIFIED., .F., .F. ) 
 B_SPLINE_CURVE_WITH_KNOTS ( ( 3, 2, 2, 2, 3 ),
 ( 0.3583333333333332815, 0.3592592592592592782, 0.3611111111111111605, 0.3629629629629629317, 0.3638888888888889284 ),
 .UNSPECIFIED. ) 
 CURVE ( )  GEOMETRIC_REPRESENTATION_ITEM ( )  RATIONAL_B_SPLINE_CURVE ( ( 0.9330127018922194093, 0.9330127018922154125, 1.000000000000000000, 0.8660254037844388186, 1.000000000000000000, 0.8660254037844388186, 1.000000000000000000, 0.9330127018922154125, 0.9330127018922194093 ) ) 
 REPRESENTATION_ITEM ( '' )  );
#19625=EDGE_CURVE ( 'NONE', #22729, #15083, #15978, .T. ) ;
#19627=AXIS2_PLACEMENT_3D ( 'NONE', #25311, #23899, #30090 ) ;
#19628=CARTESIAN_POINT ( 'NONE',  ( 5.412658773652712085, -3.125000000000086153, -165.0669872981078186 ) ) ;
#19630=CARTESIAN_POINT ( 'NONE',  ( 6.000000000000000888, -3.330669073875464691E-16, -7.560779664488942560E-35 ) ) ;
#19632=CARTESIAN_POINT ( 'NONE',  ( 7.216878364870455975, -6.409875621278545621E-14, -60.80801270189223118 ) ) ;
#19633=ORIENTED_EDGE ( 'NONE', *, *, #11257, .T. ) ;
#19636=CARTESIAN_POINT ( 'NONE',  ( 6.000000000000000888, 7.762456499804234384E-14, -132.0863248654052313 ) ) ;
#19638=CARTESIAN_POINT ( 'NONE',  ( -3.175426480542816510, 5.499999999999865885, -169.3750000000000853 ) ) ;
#19640=CARTESIAN_POINT ( 'NONE',  ( 7.216878364870455975, -6.409875621278545621E-14, -165.8080127018922951 ) ) ;
#19643=CARTESIAN_POINT ( 'NONE',  ( -3.175426480542816066, 5.499999999999865885, -113.8749999999999858 ) ) ;
#19644=CARTESIAN_POINT ( 'NONE',  ( 6.000000000000000888, 1.607695154586715303, -84.59668783648704959 ) ) ;
#19645=CARTESIAN_POINT ( 'NONE',  ( -3.175426480542816510, -5.500000000000057732, -102.8750000000000142 ) ) ;
#19650=CARTESIAN_POINT ( 'NONE',  ( 3.464101615137757051, -5.999999999999979572, -71.41367513459481131 ) ) ;
#19652=CARTESIAN_POINT ( 'NONE',  ( 6.000000000000000888, -1.607695154586752384, -126.7306624327026157 ) ) ;
#19653=CARTESIAN_POINT ( 'NONE',  ( 3.608439182435180470, 6.249999999999982236, -80.69198729810786119 ) ) ;
#19658=ORIENTED_EDGE ( 'NONE', *, *, #25054, .T. ) ;
#19659=EDGE_LOOP ( 'NONE', ( #1081, #12394, #14415, #25299 ) ) ;
#19661=EDGE_CURVE ( 'NONE', #18063, #26173, #26675, .T. ) ;
#19662=CARTESIAN_POINT ( 'NONE',  ( 2.775557561562891351E-14, 6.250000000000033751, -131.5669872981078470 ) ) ;
#19664=CARTESIAN_POINT ( 'NONE',  ( 0.000000000000000000, 5.999999999999977796, -175.2113248654052597 ) ) ;
#19667=ORIENTED_EDGE ( 'NONE', *, *, #27994, .T. ) ;
#19670=CARTESIAN_POINT ( 'NONE',  ( 6.000000000000000888, 7.762456499804235646E-14, -132.0863248654052313 ) ) ;
#19671=CARTESIAN_POINT ( 'NONE',  ( 0.000000000000000000, 0.000000000000000000, 0.000000000000000000 ) ) ;
#19675=CARTESIAN_POINT ( 'NONE',  ( 5.412658773652739619, 3.124999999999988898, -70.31698729810781856 ) ) ;
#19676=CARTESIAN_POINT ( 'NONE',  ( -5.412658773652684552, -3.125000000000099920, -53.06698729810782567 ) ) ;
#19680=CARTESIAN_POINT ( 'NONE',  ( -6.350852961085760029, -1.281975124255709124E-13, -127.1249999999999858 ) ) ;
#19684=VERTEX_POINT ( 'NONE', #15522 ) ;
#19685=CARTESIAN_POINT ( 'NONE',  ( 5.196152422706629359, 3.000000000000002665, -173.9613248654052313 ) ) ;
#19687=CARTESIAN_POINT ( 'NONE',  ( -5.999999999999968026, -1.607695154586722186, -160.3466878364870638 ) ) ;
#19693=EDGE_CURVE ( 'NONE', #9277, #28549, #4348, .T. ) ;
#19694=CARTESIAN_POINT ( 'NONE',  ( -5.196152422706573404, -3.000000000000002665, -50.78867513459483973 ) ) ;
#19695=EDGE_CURVE ( 'NONE', #9511, #26400, #406, .T. ) ;
#19699=EDGE_LOOP ( 'NONE', ( #11067, #2052, #4606, #19111 ) ) ;
#19700=CARTESIAN_POINT ( 'NONE',  ( 6.000000000000052403, -1.607695154586662678, -82.65331216351297883 ) ) ;
#19701=CARTESIAN_POINT ( 'NONE',  ( 4.763139720814407951, 2.750000000000002665, -55.75000000000002132 ) ) ;
#19702=CARTESIAN_POINT ( 'NONE',  ( -5.999999999999963585, 1.780251999655701777E-13, -86.91367513459485394 ) ) ;
#19703=CARTESIAN_POINT ( 'NONE',  ( -5.999999999999956479, -1.607695154586745057, -134.8466878364870354 ) ) ;
#19704=CARTESIAN_POINT ( 'NONE',  ( 5.412658773652712085, -3.125000000000086153, -74.43301270189223828 ) ) ;
#19706=CARTESIAN_POINT ( 'NONE',  ( -5.196152422706601826, 2.999999999999975131, -168.9613248654052029 ) ) ;
#19707=CARTESIAN_POINT ( 'NONE',  ( 6.000000000000000888, 1.607695154586715303, -80.09668783648703538 ) ) ;
#19710=CARTESIAN_POINT ( 'NONE',  ( 0.000000000000000000, 5.499999999999991118, -135.0000000000000000 ) ) ;
#19712=CARTESIAN_POINT ( 'NONE',  ( -3.608439182435115633, 6.249999999999965361, -147.3080127018922667 ) ) ;
#19714=CARTESIAN_POINT ( 'NONE',  ( -5.999999999999963585, 1.780251999655701777E-13, -81.83632486540521711 ) ) ;
#19715=CARTESIAN_POINT ( 'NONE',  ( 3.175426480543072749, -5.500000000000105693, -74.12500000000007105 ) ) ;
#19716=CARTESIAN_POINT ( 'NONE',  ( -3.175426480542816510, -5.500000000000057732, -57.87500000000004974 ) ) ;
#19717=EDGE_LOOP ( 'NONE', ( #15863, #23499, #13613, #5460 ) ) ;
#19719=CARTESIAN_POINT ( 'NONE',  ( 3.464101615137852974, 5.999999999999884537, -127.3363248654051887 ) ) ;
#19721=CARTESIAN_POINT ( 'NONE',  ( -3.464101615137757051, -5.999999999999979572, -58.16367513459481131 ) ) ;
#19723=ORIENTED_EDGE ( 'NONE', *, *, #1151, .T. ) ;
#19726=CARTESIAN_POINT ( 'NONE',  ( -3.464101615137725076, 5.999999999999979572, -64.08632486540521711 ) ) ;
#19729=CARTESIAN_POINT ( 'NONE',  ( -3.608439182435115633, 6.249999999999965361, -146.4419872981078470 ) ) ;
#19730=CARTESIAN_POINT ( 'NONE',  ( 0.000000000000000000, 5.499999999999991118, -82.50000000000001421 ) ) ;
#19731=CARTESIAN_POINT ( 'NONE',  ( -7.216878364870328078, 0.000000000000000000, -96.05801270189226670 ) ) ;
#19736=CARTESIAN_POINT ( 'NONE',  ( 6.000000000000000888, 1.743066579297358182E-13, -78.08632486540520290 ) ) ;
#19738=CARTESIAN_POINT ( 'NONE',  ( -4.763139720814407951, -2.750000000000016431, -164.5000000000000284 ) ) ;
#19739=CARTESIAN_POINT ( 'NONE',  ( 6.000000000000000888, -3.330669073875464691E-16, -7.560779664488942560E-35 ) ) ;
#19740=CARTESIAN_POINT ( 'NONE',  ( -3.175426480542816510, 5.499999999999865885, -149.8750000000000568 ) ) ;
#19742=EDGE_CURVE ( 'NONE', #24590, #750, #2396, .T. ) ;
#19743=CARTESIAN_POINT ( 'NONE',  ( 4.763139720814407951, 2.750000000000002665, -93.25000000000000000 ) ) ;
#19744=CARTESIAN_POINT ( 'NONE',  ( 3.464101615137757051, -5.999999999999979572, -130.8363248654052029 ) ) ;
#19745=CARTESIAN_POINT ( 'NONE',  ( -4.763139720814407951, 2.749999999999946709, -82.25000000000004263 ) ) ;
#19748=CARTESIAN_POINT ( 'NONE',  ( 3.464101615137757051, -5.999999999999979572, -72.33632486540520290 ) ) ;
#19750=CARTESIAN_POINT ( 'NONE',  ( 5.999999999999999112, 2.951592740943527306E-14, -156.0863248654052597 ) ) ;
#19752=CARTESIAN_POINT ( 'NONE',  ( 6.000000000000052403, 1.607695154586625819, -129.0193375672974128 ) ) ;
#19753=CARTESIAN_POINT ( 'NONE',  ( 6.000000000000000888, -1.859271017917181981E-14, -72.66367513459483973 ) ) ;
#19754=CARTESIAN_POINT ( 'NONE',  ( 3.464101615137852974, 5.999999999999884537, -75.41367513459483973 ) ) ;
#19756=ORIENTED_EDGE ( 'NONE', *, *, #4146, .T. ) ;
#19758=CARTESIAN_POINT ( 'NONE',  ( 0.000000000000000000, 0.000000000000000000, 0.000000000000000000 ) ) ;
#19761=ORIENTED_EDGE ( 'NONE', *, *, #25969, .T. ) ;
#19762=CARTESIAN_POINT ( 'NONE',  ( -4.763139720814407951, -2.750000000000016431, -107.5000000000000426 ) ) ;
#19763=CARTESIAN_POINT ( 'NONE',  ( 4.763139720814407951, 2.750000000000002665, -150.2500000000000000 ) ) ;
#19764=CARTESIAN_POINT ( 'NONE',  ( 2.775557561562891351E-14, -6.250000000000061284, -116.6830127018922383 ) ) ;
#19767=CARTESIAN_POINT ( 'NONE',  ( -3.464101615137757051, -5.999999999999979572, -110.6636751345948113 ) ) ;
#19768=CARTESIAN_POINT ( 'NONE',  ( 2.775557561562891351E-14, 6.250000000000033751, -160.0669872981078754 ) ) ;
#19770=CARTESIAN_POINT ( 'NONE',  ( 5.412658773652739619, 3.124999999999988898, -53.18301270189223828 ) ) ;
#19773=CARTESIAN_POINT ( 'NONE',  ( 6.000000000000000888, 1.743066579297358182E-13, -94.58632486540521711 ) ) ;
#19776=CARTESIAN_POINT ( 'NONE',  ( 3.175426480543072749, 5.499999999999865885, -174.1250000000000284 ) ) ;
#19779=CARTESIAN_POINT ( 'NONE',  ( 2.775557561562891351E-14, -6.250000000000061284, -166.1830127018922383 ) ) ;
#19782=CARTESIAN_POINT ( 'NONE',  ( -4.763139720814407951, -2.750000000000016431, -119.5000000000000568 ) ) ;
#19784=CARTESIAN_POINT ( 'NONE',  ( -4.763139720814407951, 2.749999999999946709, -103.2500000000000142 ) ) ;
#19786=CARTESIAN_POINT ( 'NONE',  ( -5.999999999999963585, 1.780251999655701777E-13, -77.91367513459482552 ) ) ;
#19792=EDGE_CURVE ( 'NONE', #30239, #407, #11523, .T. ) ;
#19793=( BOUNDED_CURVE ( )  B_SPLINE_CURVE ( 2, ( #1304, #22527, #24654, #29248, #1616, #29868, #3600, #8849, #24952 ),
 .UNSPECIFIED., .F., .F. ) 
 B_SPLINE_CURVE_WITH_KNOTS ( ( 3, 2, 2, 2, 3 ),
 ( 0.2361111111111111049, 0.2370370370370370461, 0.2388888888888889006, 0.2407407407407407274, 0.2416666666666666685 ),
 .UNSPECIFIED. ) 
 CURVE ( )  GEOMETRIC_REPRESENTATION_ITEM ( )  RATIONAL_B_SPLINE_CURVE ( ( 0.9330127018922196314, 0.9330127018922185211, 1.000000000000000000, 0.8660254037844388186, 1.000000000000000000, 0.8660254037844388186, 1.000000000000000000, 0.9330127018922184101, 0.9330127018922194093 ) ) 
 REPRESENTATION_ITEM ( '' )  );
#19794=ORIENTED_EDGE ( 'NONE', *, *, #9223, .T. ) ;
#19795=CARTESIAN_POINT ( 'NONE',  ( -6.350852961085760029, -1.281975124255709124E-13, -160.1250000000000284 ) ) ;
#19797=CARTESIAN_POINT ( 'NONE',  ( 3.608439182435180470, -6.249999999999997335, -79.69198729810786119 ) ) ;
#19799=ORIENTED_EDGE ( 'NONE', *, *, #14818, .F. ) ;
#19800=DIRECTION ( 'NONE',  ( -7.147005652999508048E-36, 5.642372883946980038E-36, 1.000000000000000000 ) ) ;
#19804=CARTESIAN_POINT ( 'NONE',  ( 3.608439182435180470, 6.249999999999982236, -138.5580127018922099 ) ) ;
#19806=CARTESIAN_POINT ( 'NONE',  ( 3.608439182435180470, 6.249999999999982236, -130.1919872981078470 ) ) ;
#19807=CARTESIAN_POINT ( 'NONE',  ( -3.175426480542816510, 5.499999999999865885, -170.8750000000000853 ) ) ;
#19809=CARTESIAN_POINT ( 'NONE',  ( 5.999999999999949374, 1.607695154586804565, -48.01933756729744118 ) ) ;
#19812=DIRECTION ( 'NONE',  ( -7.147005652999508048E-36, 5.642372883946980038E-36, 1.000000000000000000 ) ) ;
#19814=CARTESIAN_POINT ( 'NONE',  ( 6.000000000000000888, -1.859271017917181981E-14, -171.6636751345948539 ) ) ;
#19816=CARTESIAN_POINT ( 'NONE',  ( 3.608439182435180470, -6.249999999999997335, -70.69198729810781856 ) ) ;
#19817=CARTESIAN_POINT ( 'NONE',  ( 5.412658773652712085, -3.125000000000086153, -51.06698729810782567 ) ) ;
#19818=CARTESIAN_POINT ( 'NONE',  ( 5.999999999999999112, 2.951592740943527306E-14, -162.0863248654052029 ) ) ;
#19819=CARTESIAN_POINT ( 'NONE',  ( 0.000000000000000000, 0.000000000000000000, 0.000000000000000000 ) ) ;
#19820=CARTESIAN_POINT ( 'NONE',  ( -3.464101615137725076, 5.999999999999979572, -103.0863248654052171 ) ) ;
#19822=CARTESIAN_POINT ( 'NONE',  ( 5.196152422706629359, 3.000000000000002665, -128.0386751345948824 ) ) ;
#19823=CARTESIAN_POINT ( 'NONE',  ( 4.763139720814407951, -2.749999999999988454, -132.5000000000000000 ) ) ;
#19827=CARTESIAN_POINT ( 'NONE',  ( 6.000000000000000888, -3.330669073875464691E-16, -7.560779664488942560E-35 ) ) ;
#19828=DIRECTION ( 'NONE',  ( -7.147005652999508048E-36, 5.642372883946980038E-36, 1.000000000000000000 ) ) ;
#19829=EDGE_CURVE ( 'NONE', #688, #15144, #15142, .T. ) ;
#19831=DIRECTION ( 'NONE',  ( 1.000000000000000000, -5.551115123125773458E-17, -1.260129944081490338E-35 ) ) ;
#19832=EDGE_LOOP ( 'NONE', ( #2614, #9800, #9010, #19925 ) ) ;
#19834=CARTESIAN_POINT ( 'NONE',  ( -3.464101615137725076, 5.999999999999979572, -71.58632486540520290 ) ) ;
#19835=CARTESIAN_POINT ( 'NONE',  ( -7.216878364870328078, 0.000000000000000000, -96.69198729810780435 ) ) ;
#19836=CARTESIAN_POINT ( 'NONE',  ( 0.000000000000000000, 5.999999999999977796, -172.7886751345948255 ) ) ;
#19840=CARTESIAN_POINT ( 'NONE',  ( -5.196152422706601826, 2.999999999999975131, -77.46132486540524553 ) ) ;
#19842=CARTESIAN_POINT ( 'NONE',  ( 6.000000000000000888, 7.762456499804234384E-14, -138.0863248654051745 ) ) ;
#19843=CARTESIAN_POINT ( 'NONE',  ( -3.175426480542816510, 5.499999999999865885, -47.87500000000000000 ) ) ;
#19845=DIRECTION ( 'NONE',  ( -7.147005652999508048E-36, 5.642372883946980038E-36, 1.000000000000000000 ) ) ;
#19846=CARTESIAN_POINT ( 'NONE',  ( -3.608439182435115633, 6.249999999999965361, -76.80801270189225249 ) ) ;
#19847=CARTESIAN_POINT ( 'NONE',  ( 6.000000000000000888, 7.762456499804235646E-14, -129.0863248654052029 ) ) ;
#19849=CARTESIAN_POINT ( 'NONE',  ( -3.464101615137725076, 5.999999999999979572, -177.1636751345947971 ) ) ;
#19850=DIRECTION ( 'NONE',  ( 1.000000000000000000, -5.551115123125773458E-17, -1.260129944081490338E-35 ) ) ;
#19853=ADVANCED_FACE ( 'NONE', ( #14286 ), #26201, .T. ) ;
#19856=CARTESIAN_POINT ( 'NONE',  ( -3.175426480542816066, 5.499999999999865885, -133.3750000000000284 ) ) ;
#19858=CARTESIAN_POINT ( 'NONE',  ( -7.216878364870328078, 0.000000000000000000, -147.0580127018922667 ) ) ;
#19859=CARTESIAN_POINT ( 'NONE',  ( -5.999999999999919176, 1.607695154586804565, -158.4033121635129930 ) ) ;
#19860=CARTESIAN_POINT ( 'NONE',  ( -3.175426480542816066, 5.499999999999865885, -59.87500000000005684 ) ) ;
#19861=CARTESIAN_POINT ( 'NONE',  ( 0.000000000000000000, 0.000000000000000000, 0.000000000000000000 ) ) ;
#19862=CARTESIAN_POINT ( 'NONE',  ( -4.763139720814407951, -2.750000000000016431, -53.49999999999999289 ) ) ;
#19868=CARTESIAN_POINT ( 'NONE',  ( 6.000000000000000888, -1.859271017917181981E-14, -88.58632486540523132 ) ) ;
#19870=ORIENTED_EDGE ( 'NONE', *, *, #1117, .F. ) ;
#19875=CARTESIAN_POINT ( 'NONE',  ( -4.763139720814407951, 2.749999999999946709, -145.2500000000000000 ) ) ;
#19876=CARTESIAN_POINT ( 'NONE',  ( 5.412658773652739619, 3.124999999999988898, -49.31698729810784698 ) ) ;
#19878=ORIENTED_EDGE ( 'NONE', *, *, #13203, .T. ) ;
#19879=CARTESIAN_POINT ( 'NONE',  ( 2.775557561562891351E-14, -6.250000000000061284, -144.3169872981078186 ) ) ;
#19880=CARTESIAN_POINT ( 'NONE',  ( -3.175426480542816510, -5.500000000000057732, -69.87500000000005684 ) ) ;
#19882=CARTESIAN_POINT ( 'NONE',  ( -5.412658773652739619, 3.124999999999975131, -91.68301270189228092 ) ) ;
#19884=CARTESIAN_POINT ( 'NONE',  ( -5.196152422706601826, 2.999999999999975131, -175.5386751345948824 ) ) ;
#19888=DIRECTION ( 'NONE',  ( -7.147005652999508048E-36, 5.642372883946980038E-36, 1.000000000000000000 ) ) ;
#19889=EDGE_CURVE ( 'NONE', #956, #16271, #14014, .T. ) ;
#19890=CARTESIAN_POINT ( 'NONE',  ( -3.175426480542816066, 5.499999999999865885, -157.3750000000000000 ) ) ;
#19892=CARTESIAN_POINT ( 'NONE',  ( -2.775557561562891351E-14, -5.500000000000115463, -143.2500000000000000 ) ) ;
#19893=CARTESIAN_POINT ( 'NONE',  ( 6.000000000000000888, 1.743066579297358182E-13, -77.16367513459482552 ) ) ;
#19897=CARTESIAN_POINT ( 'NONE',  ( 4.763139720814407951, 2.750000000000002665, -88.75000000000000000 ) ) ;
#19899=CARTESIAN_POINT ( 'NONE',  ( -5.999999999999963585, 8.134310703387671600E-14, -131.3363248654052313 ) ) ;
#19900=CARTESIAN_POINT ( 'NONE',  ( -4.763139720814407951, -2.750000000000016431, -77.50000000000001421 ) ) ;
#19901=CARTESIAN_POINT ( 'NONE',  ( 6.000000000000000888, -1.859271017917181981E-14, -79.58632486540520290 ) ) ;
#19905=CARTESIAN_POINT ( 'NONE',  ( -5.999999999999919176, 1.607695154586804565, -128.4033121635129646 ) ) ;
#19907=CARTESIAN_POINT ( 'NONE',  ( -5.999999999999971578, 1.607695154586715303, -138.9033121635130499 ) ) ;
#19908=EDGE_LOOP ( 'NONE', ( #11501, #30116, #23420, #5679 ) ) ;
#19910=( NAMED_UNIT ( * ) SI_UNIT ( $, .STERADIAN. ) SOLID_ANGLE_UNIT ( ) );
#19915=ORIENTED_EDGE ( 'NONE', *, *, #24748, .T. ) ;
#19917=ADVANCED_FACE ( 'NONE', ( #12570 ), #19466, .T. ) ;
#19918=CARTESIAN_POINT ( 'NONE',  ( 4.763139720814407951, -2.749999999999988454, -108.5000000000000426 ) ) ;
#19919=CARTESIAN_POINT ( 'NONE',  ( 6.000000000000000888, -1.859271017917181981E-14, -46.58632486540520290 ) ) ;
#19920=CARTESIAN_POINT ( 'NONE',  ( 5.412658773652739619, 3.124999999999988898, -114.6830127018922383 ) ) ;
#19921=ORIENTED_EDGE ( 'NONE', *, *, #22680, .T. ) ;
#19922=CARTESIAN_POINT ( 'NONE',  ( -3.464101615137725076, 5.999999999999979572, -140.5863248654051745 ) ) ;
#19924=CARTESIAN_POINT ( 'NONE',  ( -3.608439182435115633, 6.249999999999965361, -51.30801270189225249 ) ) ;
#19925=ORIENTED_EDGE ( 'NONE', *, *, #22715, .F. ) ;
#19926=CARTESIAN_POINT ( 'NONE',  ( -3.464101615137725076, 5.999999999999979572, -167.5863248654051745 ) ) ;
#19927=CARTESIAN_POINT ( 'NONE',  ( 3.464101615137757051, -5.999999999999979572, -56.41367513459481131 ) ) ;
#19928=ADVANCED_FACE ( 'NONE', ( #7757 ), #21766, .T. ) ;
#19929=DIRECTION ( 'NONE',  ( -7.147005652999508048E-36, 5.642372883946980038E-36, 1.000000000000000000 ) ) ;
#19931=CARTESIAN_POINT ( 'NONE',  ( -4.763139720814407951, 2.749999999999946709, -170.7500000000000000 ) ) ;
#19933=FACE_OUTER_BOUND ( 'NONE', #8117, .T. ) ;
#19934=CARTESIAN_POINT ( 'NONE',  ( -5.412658773652684552, -3.125000000000099920, -170.9330127018922099 ) ) ;
#19936=CARTESIAN_POINT ( 'NONE',  ( 3.175426480543072749, 5.499999999999865885, -120.1250000000000284 ) ) ;
#19937=CARTESIAN_POINT ( 'NONE',  ( -4.763139720814407951, -2.750000000000016431, -108.9999999999999858 ) ) ;
#19938=CARTESIAN_POINT ( 'NONE',  ( -5.999999999999963585, 8.134310703387671600E-14, -142.4136751345948539 ) ) ;
#19941=VERTEX_POINT ( 'NONE', #24056 ) ;
#19947=CARTESIAN_POINT ( 'NONE',  ( -3.175426480542816510, -5.500000000000057732, -161.3750000000000284 ) ) ;
#19950=CARTESIAN_POINT ( 'NONE',  ( -3.608439182435115633, 6.249999999999965361, -84.94198729810781856 ) ) ;
#19951=CARTESIAN_POINT ( 'NONE',  ( 3.464101615137757051, -5.999999999999979572, -129.3363248654052029 ) ) ;
#19952=ORIENTED_EDGE ( 'NONE', *, *, #4185, .F. ) ;
#19954=EDGE_LOOP ( 'NONE', ( #4723, #9122, #12175, #16066 ) ) ;
#19957=CARTESIAN_POINT ( 'NONE',  ( -5.412658773652684552, -3.125000000000099920, -136.4330127018922383 ) ) ;
#19958=ORIENTED_EDGE ( 'NONE', *, *, #7210, .T. ) ;
#19959=CARTESIAN_POINT ( 'NONE',  ( 2.775557561562891351E-14, 6.250000000000033751, -124.0669872981078328 ) ) ;
#19960=CARTESIAN_POINT ( 'NONE',  ( 4.763139720814407951, 2.750000000000002665, -169.7500000000000000 ) ) ;
#19961=CARTESIAN_POINT ( 'NONE',  ( -3.464101615137725076, 5.999999999999979572, -83.58632486540518869 ) ) ;
#19962=EDGE_LOOP ( 'NONE', ( #27142, #30148, #3339, #21102 ) ) ;
#19966=CARTESIAN_POINT ( 'NONE',  ( 0.000000000000000000, 0.000000000000000000, 0.000000000000000000 ) ) ;
#19967=DIRECTION ( 'NONE',  ( -7.147005652999508048E-36, 5.642372883946980038E-36, 1.000000000000000000 ) ) ;
#19969=VECTOR ( 'NONE', #9275, 1000.000000000000000 ) ;
#19970=CARTESIAN_POINT ( 'NONE',  ( 5.412658773652712085, -3.125000000000086153, -66.06698729810783277 ) ) ;
#19971=DIRECTION ( 'NONE',  ( -7.147005652999508048E-36, 5.642372883946980038E-36, 1.000000000000000000 ) ) ;
#19972=CARTESIAN_POINT ( 'NONE',  ( 5.196152422706629359, -2.999999999999988898, -63.78867513459485394 ) ) ;
#19976=VECTOR ( 'NONE', #26397, 1000.000000000000000 ) ;
#19978=CARTESIAN_POINT ( 'NONE',  ( -4.763139720814407951, -2.750000000000016431, -125.5000000000000568 ) ) ;
#19979=LINE ( 'NONE', #18611, #26290 ) ;
#19980=ORIENTED_EDGE ( 'NONE', *, *, #17184, .T. ) ;
#19982=LINE ( 'NONE', #19827, #16575 ) ;
#19986=AXIS2_PLACEMENT_3D ( 'NONE', #744, #21506, #2732 ) ;
#19989=CARTESIAN_POINT ( 'NONE',  ( -5.412658773652684552, -3.125000000000099920, -117.5669872981078328 ) ) ;
#19996=AXIS2_PLACEMENT_3D ( 'NONE', #14480, #12770, #15053 ) ;
#19999=CARTESIAN_POINT ( 'NONE',  ( -3.175426480542816510, 5.499999999999865885, -50.87500000000001421 ) ) ;
#20000=CARTESIAN_POINT ( 'NONE',  ( -5.196152422706573404, -3.000000000000002665, -59.78867513459484684 ) ) ;
#20003=CARTESIAN_POINT ( 'NONE',  ( 2.775557561562891351E-14, -6.250000000000061284, -71.68301270189225249 ) ) ;
#20008=FACE_OUTER_BOUND ( 'NONE', #16632, .T. ) ;
#20009=CARTESIAN_POINT ( 'NONE',  ( 5.196152422706629359, -2.999999999999988898, -93.78867513459482552 ) ) ;
#20010=CARTESIAN_POINT ( 'NONE',  ( 4.763139720814407951, -2.749999999999988454, -132.5000000000000000 ) ) ;
#20012=CARTESIAN_POINT ( 'NONE',  ( 7.216878364870455975, -6.409875621278545621E-14, -149.3080127018922667 ) ) ;
#20013=CARTESIAN_POINT ( 'NONE',  ( -6.000000000000000888, 1.067854986875958443E-15, 7.560779664488942560E-35 ) ) ;
#20014=AXIS2_PLACEMENT_3D ( 'NONE', #13071, #17508, #22404 ) ;
#20016=CARTESIAN_POINT ( 'NONE',  ( 3.175426480543072749, 5.499999999999865885, -66.12500000000002842 ) ) ;
#20017=DIRECTION ( 'NONE',  ( 1.000000000000000000, -5.551115123125773458E-17, -1.260129944081490338E-35 ) ) ;
#20018=CARTESIAN_POINT ( 'NONE',  ( 4.763139720814407951, 2.750000000000002665, -57.25000000000002132 ) ) ;
#20021=ORIENTED_EDGE ( 'NONE', *, *, #26836, .F. ) ;
#20024=FACE_OUTER_BOUND ( 'NONE', #6027, .T. ) ;
#20030=CARTESIAN_POINT ( 'NONE',  ( 3.464101615137757051, -5.999999999999979572, -121.8363248654051745 ) ) ;
#20034=CARTESIAN_POINT ( 'NONE',  ( -3.175426480542816510, 5.499999999999865885, -145.3750000000000000 ) ) ;
#20035=CARTESIAN_POINT ( 'NONE',  ( 5.412658773652712085, -3.125000000000086153, -49.56698729810782567 ) ) ;
#20038=CARTESIAN_POINT ( 'NONE',  ( 3.608439182435180470, 6.249999999999982236, -145.1919872981078470 ) ) ;
#20039=CARTESIAN_POINT ( 'NONE',  ( 3.175426480543072749, -5.500000000000105693, -77.12500000000001421 ) ) ;
#20041=CARTESIAN_POINT ( 'NONE',  ( 7.216878364870455975, -6.409875621278545621E-14, -96.80801270189220986 ) ) ;
#20042=CARTESIAN_POINT ( 'NONE',  ( -6.350852961085760029, -1.281975124255709124E-13, -152.6250000000000568 ) ) ;
#20043=CARTESIAN_POINT ( 'NONE',  ( -5.382374809129815141, -9.594851770513439959, -27.68068691953151372 ) ) ;
#20044=CYLINDRICAL_SURFACE ( 'NONE', #23564, 6.000000000000000888 ) ;
#20046=CARTESIAN_POINT ( 'NONE',  ( 0.000000000000000000, 5.999999999999977796, -98.71132486540523132 ) ) ;
#20047=CARTESIAN_POINT ( 'NONE',  ( 6.000000000000000888, -1.859271017917181981E-14, -114.0863248654052029 ) ) ;
#20048=CARTESIAN_POINT ( 'NONE',  ( -2.775557561562891351E-14, -5.500000000000115463, -152.2500000000000000 ) ) ;
#20049=DIRECTION ( 'NONE',  ( -7.147005652999508048E-36, 5.642372883946980038E-36, 1.000000000000000000 ) ) ;
#20050=CARTESIAN_POINT ( 'NONE',  ( 3.175426480543072749, 5.499999999999865885, -147.1250000000000284 ) ) ;
#20051=CARTESIAN_POINT ( 'NONE',  ( -4.501142602633604994, 3.771550028943533306, -180.0000000000000568 ) ) ;
#20052=CARTESIAN_POINT ( 'NONE',  ( 3.175426480543072749, -5.500000000000105693, -90.62500000000001421 ) ) ;
#20055=CARTESIAN_POINT ( 'NONE',  ( 4.763139720814407951, -2.749999999999988454, -83.00000000000001421 ) ) ;
#20056=CARTESIAN_POINT ( 'NONE',  ( -5.999999999999963585, 1.780251999655701777E-13, -86.33632486540524553 ) ) ;
#20060=DIRECTION ( 'NONE',  ( -7.147005652999508048E-36, 5.642372883946980038E-36, 1.000000000000000000 ) ) ;
#20062=CARTESIAN_POINT ( 'NONE',  ( 6.000000000000000888, -1.859271017917181981E-14, -135.0863248654052029 ) ) ;
#20063=CARTESIAN_POINT ( 'NONE',  ( 5.196152422706629359, 3.000000000000002665, -75.53867513459483973 ) ) ;
#20064=( BOUNDED_CURVE ( )  B_SPLINE_CURVE ( 2, ( #15078, #8767, #24420, #19820, #29165, #15237, #1994, #18760, #18456 ),
 .UNSPECIFIED., .F., .T. ) 
 B_SPLINE_CURVE_WITH_KNOTS ( ( 3, 2, 2, 2, 3 ),
 ( 0.4194444444444445086, 0.4203703703703703942, 0.4222222222222222765, 0.4240740740740740478, 0.4249999999999999334 ),
 .UNSPECIFIED. ) 
 CURVE ( )  GEOMETRIC_REPRESENTATION_ITEM ( )  RATIONAL_B_SPLINE_CURVE ( ( 0.9330127018922194093, 0.9330127018922234061, 1.000000000000000000, 0.8660254037844388186, 1.000000000000000000, 0.8660254037844388186, 1.000000000000000000, 0.9330127018922234061, 0.9330127018922194093 ) ) 
 REPRESENTATION_ITEM ( '' )  );
#20065=ORIENTED_EDGE ( 'NONE', *, *, #23211, .T. ) ;
#20066=CARTESIAN_POINT ( 'NONE',  ( 3.464101615137852974, 5.999999999999884537, -91.33632486540520290 ) ) ;
#20067=CARTESIAN_POINT ( 'NONE',  ( 2.775557561562895769E-14, 11.00000000000000000, -14.99152654425661702 ) ) ;
#20071=ORIENTED_EDGE ( 'NONE', *, *, #16711, .F. ) ;
#20072=EDGE_CURVE ( 'NONE', #20142, #28820, #16165, .T. ) ;
#20073=( BOUNDED_CURVE ( )  B_SPLINE_CURVE ( 2, ( #5719, #9910, #677, #19721, #10515, #21586, #10364, #19578, #5420 ),
 .UNSPECIFIED., .F., .F. ) 
 B_SPLINE_CURVE_WITH_KNOTS ( ( 3, 2, 2, 2, 3 ),
 ( 0.9138888888888888618, 0.9148148148148148584, 0.9166666666666666297, 0.9185185185185185119, 0.9194444444444445086 ),
 .UNSPECIFIED. ) 
 CURVE ( )  GEOMETRIC_REPRESENTATION_ITEM ( )  RATIONAL_B_SPLINE_CURVE ( ( 0.9330127018922194093, 0.9330127018922154125, 1.000000000000000000, 0.8660254037844388186, 1.000000000000000000, 0.8660254037844388186, 1.000000000000000000, 0.9330127018922154125, 0.9330127018922194093 ) ) 
 REPRESENTATION_ITEM ( '' )  );
#20076=CARTESIAN_POINT ( 'NONE',  ( -6.350852961085760029, -1.281975124255709124E-13, -100.1250000000000568 ) ) ;
#20078=CARTESIAN_POINT ( 'NONE',  ( 7.216878364870455975, -6.409875621278545621E-14, -111.8080127018922241 ) ) ;
#20079=EDGE_LOOP ( 'NONE', ( #6772, #13211, #10141, #11910 ) ) ;
#20083=CARTESIAN_POINT ( 'NONE',  ( -7.216878364870328078, 0.000000000000000000, -54.05801270189220276 ) ) ;
#20089=CARTESIAN_POINT ( 'NONE',  ( 0.000000000000000000, 5.499999999999991118, -169.4999999999999716 ) ) ;
#20091=CARTESIAN_POINT ( 'NONE',  ( 2.775557561562891351E-14, 6.250000000000033751, -171.4330127018922667 ) ) ;
#20093=CARTESIAN_POINT ( 'NONE',  ( -3.175426480542816066, 5.499999999999865885, -106.3750000000000284 ) ) ;
#20095=CARTESIAN_POINT ( 'NONE',  ( 0.000000000000000000, 5.499999999999991118, -107.9999999999999858 ) ) ;
#20098=CARTESIAN_POINT ( 'NONE',  ( 6.000000000000000888, -1.607695154586752384, -84.15331216351299304 ) ) ;
#20099=ORIENTED_EDGE ( 'NONE', *, *, #3850, .F. ) ;
#20101=EDGE_CURVE ( 'NONE', #26392, #3053, #16485, .T. ) ;
#20104=CARTESIAN_POINT ( 'NONE',  ( 6.000000000000000888, 1.743066579297358182E-13, -62.16367513459481131 ) ) ;
#20105=ORIENTED_EDGE ( 'NONE', *, *, #18882, .T. ) ;
#20106=CARTESIAN_POINT ( 'NONE',  ( -5.999999999999963585, 1.780251999655701777E-13, -65.33632486540521711 ) ) ;
#20107=CARTESIAN_POINT ( 'NONE',  ( 5.412658773652739619, 3.124999999999988898, -83.81698729810781856 ) ) ;
#20108=AXIS2_PLACEMENT_3D ( 'NONE', #15397, #5511, #10612 ) ;
#20110=ORIENTED_EDGE ( 'NONE', *, *, #8658, .F. ) ;
#20115=EDGE_LOOP ( 'NONE', ( #12774, #1061, #2106, #14771 ) ) ;
#20117=( BOUNDED_CURVE ( )  B_SPLINE_CURVE ( 2, ( #7396, #3070, #321, #9710, #19093, #28416, #22436, #20130, #12786 ),
 .UNSPECIFIED., .F., .F. ) 
 B_SPLINE_CURVE_WITH_KNOTS ( ( 3, 2, 2, 2, 3 ),
 ( 0.3416666666666666741, 0.3425925925925925597, 0.3444444444444444420, 0.3462962962962963243, 0.3472222222222222099 ),
 .UNSPECIFIED. ) 
 CURVE ( )  GEOMETRIC_REPRESENTATION_ITEM ( )  RATIONAL_B_SPLINE_CURVE ( ( 0.9330127018922194093, 0.9330127018922194093, 1.000000000000000000, 0.8660254037844388186, 1.000000000000000000, 0.8660254037844388186, 1.000000000000000000, 0.9330127018922194093, 0.9330127018922194093 ) ) 
 REPRESENTATION_ITEM ( '' )  );
#20118=CARTESIAN_POINT ( 'NONE',  ( -3.175426480542816510, 5.499999999999865885, -122.8749999999999858 ) ) ;
#20119=CARTESIAN_POINT ( 'NONE',  ( 7.216878364870455975, -6.409875621278545621E-14, -135.8080127018922667 ) ) ;
#20120=EDGE_LOOP ( 'NONE', ( #9158, #22577, #20157, #6588 ) ) ;
#20122=CARTESIAN_POINT ( 'NONE',  ( -3.608439182435052128, -6.250000000000110134, -121.9419872981078043 ) ) ;
#20123=CARTESIAN_POINT ( 'NONE',  ( -5.196152422706573404, -3.000000000000002665, -135.7113248654052029 ) ) ;
#20124=CARTESIAN_POINT ( 'NONE',  ( 0.000000000000000000, 5.499999999999991118, -171.0000000000000284 ) ) ;
#20127=ORIENTED_EDGE ( 'NONE', *, *, #21290, .F. ) ;
#20129=CARTESIAN_POINT ( 'NONE',  ( -5.999999999999956479, -1.607695154586745057, -117.7693375672974696 ) ) ;
#20130=CARTESIAN_POINT ( 'NONE',  ( 6.000000000000000888, 1.607695154586715303, -93.01933756729744118 ) ) ;
#20131=CARTESIAN_POINT ( 'NONE',  ( 6.000000000000000888, -3.330669073875464691E-16, -7.560779664488942560E-35 ) ) ;
#20133=CARTESIAN_POINT ( 'NONE',  ( 7.216878364870455975, -6.409875621278545621E-14, -68.94198729810780435 ) ) ;
#20134=CARTESIAN_POINT ( 'NONE',  ( 2.775557561562891351E-14, -6.250000000000061284, -57.31698729810786119 ) ) ;
#20135=CARTESIAN_POINT ( 'NONE',  ( 3.464101615137757051, -5.999999999999979572, -120.9136751345947971 ) ) ;
#20136=CARTESIAN_POINT ( 'NONE',  ( 3.464101615137757051, -5.999999999999979572, -63.91367513459485394 ) ) ;
#20140=CARTESIAN_POINT ( 'NONE',  ( 3.175426480543072749, -5.500000000000105693, -126.6250000000000000 ) ) ;
#20141=ADVANCED_FACE ( 'NONE', ( #26945 ), #28946, .T. ) ;
#20142=VERTEX_POINT ( 'NONE', #7910 ) ;
#20145=CARTESIAN_POINT ( 'NONE',  ( 5.196152422706629359, 3.000000000000002665, -119.9613248654052313 ) ) ;
#20146=FACE_OUTER_BOUND ( 'NONE', #24176, .T. ) ;
#20147=CARTESIAN_POINT ( 'NONE',  ( 5.999999999999999112, 2.951592740943527306E-14, -161.1636751345949108 ) ) ;
#20149=ORIENTED_EDGE ( 'NONE', *, *, #16510, .T. ) ;
#20151=DIRECTION ( 'NONE',  ( -7.147005652999508048E-36, 5.642372883946980038E-36, 1.000000000000000000 ) ) ;
#20152=LINE ( 'NONE', #28057, #866 ) ;
#20153=CARTESIAN_POINT ( 'NONE',  ( -3.608439182435115633, 6.249999999999965361, -116.4419872981078470 ) ) ;
#20157=ORIENTED_EDGE ( 'NONE', *, *, #15348, .T. ) ;
#20164=CARTESIAN_POINT ( 'NONE',  ( -4.763139720814407951, -2.750000000000016431, -52.00000000000004263 ) ) ;
#20165=CARTESIAN_POINT ( 'NONE',  ( 6.000000000000000888, 1.743066579297358182E-13, -96.08632486540521711 ) ) ;
#20167=CARTESIAN_POINT ( 'NONE',  ( 2.775557561562891351E-14, -6.250000000000061284, -74.68301270189226670 ) ) ;
#20168=( BOUNDED_CURVE ( )  B_SPLINE_CURVE ( 2, ( #5118, #12690, #17292, #22023, #959, #7878, #21881, #26612, #9909 ),
 .UNSPECIFIED., .F., .T. ) 
 B_SPLINE_CURVE_WITH_KNOTS ( ( 3, 2, 2, 2, 3 ),
 ( 0.6194444444444444642, 0.6203703703703703498, 0.6222222222222222321, 0.6240740740740741144, 0.6250000000000000000 ),
 .UNSPECIFIED. ) 
 CURVE ( )  GEOMETRIC_REPRESENTATION_ITEM ( )  RATIONAL_B_SPLINE_CURVE ( ( 0.9330127018922194093, 0.9330127018922234061, 1.000000000000000000, 0.8660254037844388186, 1.000000000000000000, 0.8660254037844388186, 1.000000000000000000, 0.9330127018922194093, 0.9330127018922194093 ) ) 
 REPRESENTATION_ITEM ( '' )  );
#20169=CARTESIAN_POINT ( 'NONE',  ( -5.196152422706573404, -3.000000000000002665, -173.2113248654052597 ) ) ;
#20170=AXIS2_PLACEMENT_3D ( 'NONE', #10199, #14816, #17125 ) ;
#20172=CARTESIAN_POINT ( 'NONE',  ( 6.000000000000000888, 5.577813053751546416E-15, -177.6636751345948255 ) ) ;
#20173=SURFACE_STYLE_USAGE ( .BOTH. , #27054 ) ;
#20174=CARTESIAN_POINT ( 'NONE',  ( -5.999999999999919176, 1.607695154586804565, -104.4033121635129930 ) ) ;
#20175=CARTESIAN_POINT ( 'NONE',  ( -4.763139720814407951, -2.750000000000016431, -131.5000000000000000 ) ) ;
#20177=CARTESIAN_POINT ( 'NONE',  ( -3.608439182435052128, -6.250000000000110134, -146.8080127018922667 ) ) ;
#20180=AXIS2_PLACEMENT_3D ( 'NONE', #12823, #3100, #26150 ) ;
#20181=CARTESIAN_POINT ( 'NONE',  ( -2.775557561562891351E-14, -5.500000000000115463, -65.25000000000002842 ) ) ;
#20182=DIRECTION ( 'NONE',  ( 1.000000000000000000, -5.551115123125773458E-17, -1.260129944081490338E-35 ) ) ;
#20183=CARTESIAN_POINT ( 'NONE',  ( -5.196152422706573404, -3.000000000000002665, -174.7113248654052029 ) ) ;
#20190=CARTESIAN_POINT ( 'NONE',  ( 0.000000000000000000, -5.999999999999991118, -49.03867513459481131 ) ) ;
#20193=EDGE_LOOP ( 'NONE', ( #13294, #19952, #18207, #12552 ) ) ;
#20196=ORIENTED_EDGE ( 'NONE', *, *, #25800, .T. ) ;
#20197=CARTESIAN_POINT ( 'NONE',  ( -2.775557561562891351E-14, -5.500000000000115463, -143.2500000000000000 ) ) ;
#20199=CARTESIAN_POINT ( 'NONE',  ( 3.608439182435180470, -6.249999999999997335, -48.19198729810783277 ) ) ;
#20202=CARTESIAN_POINT ( 'NONE',  ( -3.175426480542816510, -5.500000000000057732, -77.37500000000001421 ) ) ;
#20204=CARTESIAN_POINT ( 'NONE',  ( -5.412658773652739619, 3.124999999999975131, -93.18301270189222407 ) ) ;
#20205=ORIENTED_EDGE ( 'NONE', *, *, #26102, .F. ) ;
#20206=CARTESIAN_POINT ( 'NONE',  ( -0.8029667472979058473, -10.97248951867538302, -19.05056182979571133 ) ) ;
#20212=CARTESIAN_POINT ( 'NONE',  ( 6.350852961086080661, -9.614813431917819062E-14, -153.3749999999999716 ) ) ;
#20213=DIRECTION ( 'NONE',  ( -7.147005652999508048E-36, 5.642372883946980038E-36, 1.000000000000000000 ) ) ;
#20214=AXIS2_PLACEMENT_3D ( 'NONE', #12538, #674, #28912 ) ;
#20215=CARTESIAN_POINT ( 'NONE',  ( -2.027308962371316525, 5.280605156496299024, -179.9999999999999716 ) ) ;
#20218=EDGE_CURVE ( 'NONE', #4196, #18433, #18689, .T. ) ;
#20219=CARTESIAN_POINT ( 'NONE',  ( 0.000000000000000000, 0.000000000000000000, -183.0000000000000000 ) ) ;
#20220=CARTESIAN_POINT ( 'NONE',  ( 3.175426480543072749, -5.500000000000105693, -75.62500000000000000 ) ) ;
#20223=CARTESIAN_POINT ( 'NONE',  ( -3.464101615137725076, 5.999999999999979572, -106.0863248654052313 ) ) ;
#20231=CARTESIAN_POINT ( 'NONE',  ( -5.999999999999964473, 9.063946212346262433E-15, -173.9136751345948255 ) ) ;
#20234=CARTESIAN_POINT ( 'NONE',  ( -5.999999999999919176, 1.607695154586804565, -72.90331216351302146 ) ) ;
#20238=CARTESIAN_POINT ( 'NONE',  ( -4.763139720814407951, -2.750000000000016431, -94.00000000000002842 ) ) ;
#20239=CARTESIAN_POINT ( 'NONE',  ( 0.000000000000000000, 0.000000000000000000, 0.000000000000000000 ) ) ;
#20240=CARTESIAN_POINT ( 'NONE',  ( -5.412658773652739619, 3.124999999999975131, -115.6830127018922383 ) ) ;
#20241=EDGE_LOOP ( 'NONE', ( #7190, #3455, #8381, #9995 ) ) ;
#20242=CARTESIAN_POINT ( 'NONE',  ( 6.000000000000000888, 7.762456499804235646E-14, -132.6636751345948539 ) ) ;
#20243=FACE_OUTER_BOUND ( 'NONE', #9305, .T. ) ;
#20244=CARTESIAN_POINT ( 'NONE',  ( 7.216878364870455975, -6.409875621278545621E-14, -48.80801270189224539 ) ) ;
#20245=VERTEX_POINT ( 'NONE', #13954 ) ;
#20246=CARTESIAN_POINT ( 'NONE',  ( -5.999999999999962697, 3.323446944526963260E-14, -159.8363248654052597 ) ) ;
#20249=CARTESIAN_POINT ( 'NONE',  ( 4.763139720814407951, 2.750000000000002665, -163.7500000000000000 ) ) ;
#20251=CARTESIAN_POINT ( 'NONE',  ( 6.000000000000000888, 1.743066579297358182E-13, -108.0863248654051745 ) ) ;
#20252=ADVANCED_FACE ( 'NONE', ( #15947 ), #25571, .T. ) ;
#20253=CARTESIAN_POINT ( 'NONE',  ( -4.763139720814407951, 2.749999999999946709, -109.2500000000000142 ) ) ;
#20255=( BOUNDED_CURVE ( )  B_SPLINE_CURVE ( 2, ( #21140, #15953, #18696, #6991, #30032, #2388, #28170, #11800, #28018 ),
 .UNSPECIFIED., .F., .T. ) 
 B_SPLINE_CURVE_WITH_KNOTS ( ( 3, 2, 2, 2, 3 ),
 ( 0.3805555555555555358, 0.3814814814814815325, 0.3833333333333333037, 0.3851851851851851860, 0.3861111111111111827 ),
 .UNSPECIFIED. ) 
 CURVE ( )  GEOMETRIC_REPRESENTATION_ITEM ( )  RATIONAL_B_SPLINE_CURVE ( ( 0.9330127018922194093, 0.9330127018922154125, 1.000000000000000000, 0.8660254037844388186, 1.000000000000000000, 0.8660254037844388186, 1.000000000000000000, 0.9330127018922154125, 0.9330127018922194093 ) ) 
 REPRESENTATION_ITEM ( '' )  );
#20257=CARTESIAN_POINT ( 'NONE',  ( 4.763139720814407951, -2.749999999999988454, -107.0000000000000426 ) ) ;
#20259=CARTESIAN_POINT ( 'NONE',  ( 0.000000000000000000, 5.999999999999977796, -118.2113248654052029 ) ) ;
#20265=ORIENTED_EDGE ( 'NONE', *, *, #1620, .F. ) ;
#20266=CARTESIAN_POINT ( 'NONE',  ( -2.775557561562891351E-14, -5.500000000000115463, -161.2500000000000000 ) ) ;
#20267=CARTESIAN_POINT ( 'NONE',  ( -5.412658773652739619, 3.124999999999975131, -89.31698729810783277 ) ) ;
#20270=CARTESIAN_POINT ( 'NONE',  ( -5.999999999999963585, 1.780251999655701777E-13, -65.91367513459482552 ) ) ;
#20273=CARTESIAN_POINT ( 'NONE',  ( 4.763139720814407951, 2.750000000000002665, -123.2500000000000284 ) ) ;
#20275=CARTESIAN_POINT ( 'NONE',  ( -5.412658773652739619, 3.124999999999975131, -125.3169872981078043 ) ) ;
#20276=CARTESIAN_POINT ( 'NONE',  ( 5.412658773652739619, 3.124999999999988898, -178.3169872981078470 ) ) ;
#20277=CARTESIAN_POINT ( 'NONE',  ( -2.775557561562891351E-14, -5.500000000000115463, -174.7500000000000284 ) ) ;
#20279=CARTESIAN_POINT ( 'NONE',  ( -5.999999999999919176, 1.607695154586804565, -47.40331216351300725 ) ) ;
#20280=ORIENTED_EDGE ( 'NONE', *, *, #4605, .F. ) ;
#20282=DIRECTION ( 'NONE',  ( -7.147005652999508048E-36, 5.642372883946980038E-36, 1.000000000000000000 ) ) ;
#20284=CARTESIAN_POINT ( 'NONE',  ( -5.196152422706601826, 2.999999999999975131, -171.0386751345947971 ) ) ;
#20285=CARTESIAN_POINT ( 'NONE',  ( 0.000000000000000000, -5.999999999999991118, -46.96132486540521711 ) ) ;
#20286=CARTESIAN_POINT ( 'NONE',  ( 3.608439182435180470, 6.249999999999982236, -71.69198729810781856 ) ) ;
#20287=CARTESIAN_POINT ( 'NONE',  ( -5.412658773652739619, 3.124999999999975131, -51.81698729810779724 ) ) ;
#20288=CARTESIAN_POINT ( 'NONE',  ( 4.763139720814407951, -2.749999999999988454, -50.00000000000004263 ) ) ;
#20292=CARTESIAN_POINT ( 'NONE',  ( -3.175426480542816510, 5.499999999999865885, -131.8750000000000000 ) ) ;
#20299=LINE ( 'NONE', #11250, #12865 ) ;
#20303=CARTESIAN_POINT ( 'NONE',  ( 5.196152422706629359, 3.000000000000002665, -71.96132486540524553 ) ) ;
#20305=CARTESIAN_POINT ( 'NONE',  ( -5.412658773652684552, -3.125000000000099920, -116.0669872981078328 ) ) ;
#20308=EDGE_LOOP ( 'NONE', ( #27599, #29490, #8171, #19215 ) ) ;
#20314=CARTESIAN_POINT ( 'NONE',  ( 4.763139720814407951, 2.750000000000002665, -52.75000000000002132 ) ) ;
#20316=DIRECTION ( 'NONE',  ( 1.000000000000000000, -5.551115123125773458E-17, -1.260129944081490338E-35 ) ) ;
#20317=CARTESIAN_POINT ( 'NONE',  ( 3.608439182435180470, -6.249999999999997335, -71.55801270189220986 ) ) ;
#20320=CARTESIAN_POINT ( 'NONE',  ( -5.999999999999968026, 1.607695154586720854, -176.9806624327026157 ) ) ;
#20325=CARTESIAN_POINT ( 'NONE',  ( 6.350852961086080661, -9.614813431917819062E-14, -135.3750000000000284 ) ) ;
#20326=DIRECTION ( 'NONE',  ( -7.147005652999508048E-36, 5.642372883946980038E-36, 1.000000000000000000 ) ) ;
#20328=CARTESIAN_POINT ( 'NONE',  ( -4.763139720814407951, -2.750000000000016431, -61.00000000000000000 ) ) ;
#20329=CYLINDRICAL_SURFACE ( 'NONE', #8610, 6.000000000000000888 ) ;
#20334=CARTESIAN_POINT ( 'NONE',  ( 0.000000000000000000, 0.000000000000000000, 0.000000000000000000 ) ) ;
#20335=ORIENTED_EDGE ( 'NONE', *, *, #24803, .F. ) ;
#20338=CARTESIAN_POINT ( 'NONE',  ( -3.175426480542816510, -5.500000000000057732, -146.3750000000000284 ) ) ;
#20339=( BOUNDED_CURVE ( )  B_SPLINE_CURVE ( 2, ( #28277, #16664, #26280, #25987, #4932, #14363, #7404, #16812, #26132 ),
 .UNSPECIFIED., .F., .T. ) 
 B_SPLINE_CURVE_WITH_KNOTS ( ( 3, 2, 2, 2, 3 ),
 ( 0.9527777777777778345, 0.9537037037037037202, 0.9555555555555556024, 0.9574074074074073737, 0.9583333333333332593 ),
 .UNSPECIFIED. ) 
 CURVE ( )  GEOMETRIC_REPRESENTATION_ITEM ( )  RATIONAL_B_SPLINE_CURVE ( ( 0.9330127018922194093, 0.9330127018922234061, 1.000000000000000000, 0.8660254037844388186, 1.000000000000000000, 0.8660254037844388186, 1.000000000000000000, 0.9330127018922234061, 0.9330127018922194093 ) ) 
 REPRESENTATION_ITEM ( '' )  );
#20343=EDGE_CURVE ( 'NONE', #4636, #27213, #7491, .T. ) ;
#20344=CARTESIAN_POINT ( 'NONE',  ( 4.763139720814407951, 2.750000000000002665, -75.25000000000004263 ) ) ;
#20346=ORIENTED_EDGE ( 'NONE', *, *, #25660, .F. ) ;
#20354=CARTESIAN_POINT ( 'NONE',  ( 4.763139720814407951, -2.749999999999988454, -155.0000000000000284 ) ) ;
#20357=CARTESIAN_POINT ( 'NONE',  ( 4.763139720814407951, 2.750000000000002665, -87.25000000000005684 ) ) ;
#20358=CARTESIAN_POINT ( 'NONE',  ( -3.175426480542816510, 5.499999999999865885, -71.87500000000000000 ) ) ;
#20359=AXIS2_PLACEMENT_3D ( 'NONE', #27697, #20668, #15793 ) ;
#20360=CARTESIAN_POINT ( 'NONE',  ( -5.999999999999963585, 8.134310703387671600E-14, -141.8363248654052029 ) ) ;
#20362=CARTESIAN_POINT ( 'NONE',  ( 0.000000000000000000, 0.000000000000000000, 0.000000000000000000 ) ) ;
#20364=AXIS2_PLACEMENT_3D ( 'NONE', #1307, #13193, #22066 ) ;
#20365=CARTESIAN_POINT ( 'NONE',  ( 5.196152422706629359, 3.000000000000002665, -119.0386751345948682 ) ) ;
#20367=DIRECTION ( 'NONE',  ( -7.147005652999508048E-36, 5.642372883946980038E-36, 1.000000000000000000 ) ) ;
#20372=ORIENTED_EDGE ( 'NONE', *, *, #1117, .T. ) ;
#20373=ADVANCED_FACE ( 'NONE', ( #11793 ), #28464, .T. ) ;
#20374=CARTESIAN_POINT ( 'NONE',  ( 6.350852961086080661, -9.614813431917819062E-14, -99.37499999999998579 ) ) ;
#20375=CARTESIAN_POINT ( 'NONE',  ( 5.196152422706629359, -2.999999999999988898, -89.28867513459482552 ) ) ;
#20376=CARTESIAN_POINT ( 'NONE',  ( 5.412658773652739619, 3.124999999999988898, -113.1830127018922383 ) ) ;
#20378=PLANE ( 'NONE',  #1472 ) ;
#20379=CARTESIAN_POINT ( 'NONE',  ( 5.196152422706629359, 3.000000000000002665, -52.46132486540522422 ) ) ;
#20380=CARTESIAN_POINT ( 'NONE',  ( -7.216878364870328078, 0.000000000000000000, -49.55801270189223828 ) ) ;
#20382=CARTESIAN_POINT ( 'NONE',  ( 0.000000000000000000, 5.999999999999977796, -160.2113248654052313 ) ) ;
#20386=CARTESIAN_POINT ( 'NONE',  ( 3.175426480543072749, 5.499999999999865885, -163.6249999999999716 ) ) ;
#20389=CARTESIAN_POINT ( 'NONE',  ( 0.000000000000000000, 5.499999999999991118, -112.5000000000000426 ) ) ;
#20391=CARTESIAN_POINT ( 'NONE',  ( -2.775557561562891351E-14, -5.500000000000115463, -95.25000000000000000 ) ) ;
#20392=VECTOR ( 'NONE', #20543, 1000.000000000000000 ) ;
#20393=CARTESIAN_POINT ( 'NONE',  ( -6.000000000000007105, -1.607695154586655129, -112.3466878364870638 ) ) ;
#20394=CARTESIAN_POINT ( 'NONE',  ( 0.000000000000000000, -5.999999999999991118, -82.03867513459483973 ) ) ;
#20400=CARTESIAN_POINT ( 'NONE',  ( 3.464101615137852974, 5.999999999999884537, -112.3363248654051887 ) ) ;
#20402=CARTESIAN_POINT ( 'NONE',  ( 7.216878364870455975, -6.409875621278545621E-14, -89.94198729810783277 ) ) ;
#20403=CARTESIAN_POINT ( 'NONE',  ( -5.999999999999963585, -1.487416814333745711E-14, -67.41367513459481131 ) ) ;
#20404=VERTEX_POINT ( 'NONE', #23588 ) ;
#20405=CARTESIAN_POINT ( 'NONE',  ( -4.513192036455980549, 10.03241344175770600, -28.95831720094624728 ) ) ;
#20406=VERTEX_POINT ( 'NONE', #29178 ) ;
#20407=ORIENTED_EDGE ( 'NONE', *, *, #8586, .T. ) ;
#20410=CARTESIAN_POINT ( 'NONE',  ( -3.175426480542816510, 5.499999999999865885, -119.8750000000000284 ) ) ;
#20412=CARTESIAN_POINT ( 'NONE',  ( 3.608439182435180470, -6.249999999999997335, -140.5580127018922383 ) ) ;
#20415=CARTESIAN_POINT ( 'NONE',  ( 5.412658773652739619, 3.124999999999988898, -119.8169872981078612 ) ) ;
#20416=CARTESIAN_POINT ( 'NONE',  ( -5.412658773652739619, 3.124999999999975131, -176.3169872981078470 ) ) ;
#20417=CARTESIAN_POINT ( 'NONE',  ( -6.350852961085760029, -1.281975124255709124E-13, -170.6250000000000284 ) ) ;
#20419=CARTESIAN_POINT ( 'NONE',  ( -6.000000000000000888, 1.067854986875958443E-15, 7.560779664488942560E-35 ) ) ;
#20424=AXIS2_PLACEMENT_3D ( 'NONE', #24638, #6056, #982 ) ;
#20426=CARTESIAN_POINT ( 'NONE',  ( -3.464101615137757051, -5.999999999999979572, -55.16367513459481131 ) ) ;
#20427=CARTESIAN_POINT ( 'NONE',  ( 3.608439182435180470, 6.249999999999982236, -76.19198729810784698 ) ) ;
#20429=CARTESIAN_POINT ( 'NONE',  ( 2.775557561562891351E-14, 6.250000000000033751, -61.06698729810783277 ) ) ;
#20430=CARTESIAN_POINT ( 'NONE',  ( -3.464101615137725076, 5.999999999999979572, -110.5863248654051603 ) ) ;
#20431=CARTESIAN_POINT ( 'NONE',  ( -4.763139720814407951, 2.749999999999946709, -50.75000000000001421 ) ) ;
#20433=CARTESIAN_POINT ( 'NONE',  ( -6.000000000000007105, -1.607695154586655129, -47.84668783648706381 ) ) ;
#20434=CARTESIAN_POINT ( 'NONE',  ( 6.350852961086080661, -9.614813431917819062E-14, -121.8750000000000426 ) ) ;
#20439=DIRECTION ( 'NONE',  ( -7.147005652999508048E-36, 5.642372883946980038E-36, 1.000000000000000000 ) ) ;
#20441=VERTEX_POINT ( 'NONE', #26872 ) ;
#20442=VECTOR ( 'NONE', #18248, 1000.000000000000000 ) ;
#20446=CARTESIAN_POINT ( 'NONE',  ( 3.608439182435180470, -6.249999999999997335, -114.1919872981078328 ) ) ;
#20447=CARTESIAN_POINT ( 'NONE',  ( 6.000000000000000888, -1.859271017917181981E-14, -54.08632486540521001 ) ) ;
#20454=ORIENTED_EDGE ( 'NONE', *, *, #6391, .T. ) ;
#20456=CARTESIAN_POINT ( 'NONE',  ( 3.175426480543072749, 5.499999999999865885, -52.62500000000002842 ) ) ;
#20461=CARTESIAN_POINT ( 'NONE',  ( -5.412658773652739619, 3.124999999999975131, -66.18301270189225249 ) ) ;
#20464=CARTESIAN_POINT ( 'NONE',  ( -5.999999999999960032, -1.607695154586736397, -178.3466878364870638 ) ) ;
#20468=CARTESIAN_POINT ( 'NONE',  ( 0.000000000000000000, -5.999999999999991118, -67.03867513459482552 ) ) ;
#20469=CARTESIAN_POINT ( 'NONE',  ( 4.763139720814407951, 2.750000000000002665, -127.7500000000000284 ) ) ;
#20473=CARTESIAN_POINT ( 'NONE',  ( -2.775557561562891351E-14, -5.500000000000115463, -62.25000000000002842 ) ) ;
#20474=CARTESIAN_POINT ( 'NONE',  ( -3.464101615137757051, -5.999999999999979572, -154.1636751345947971 ) ) ;
#20475=CARTESIAN_POINT ( 'NONE',  ( 3.464101615137757051, -5.999999999999979572, -76.83632486540520290 ) ) ;
#20476=ORIENTED_EDGE ( 'NONE', *, *, #19463, .F. ) ;
#20479=CARTESIAN_POINT ( 'NONE',  ( -5.999999999999963585, 1.780251999655701777E-13, -90.83632486540521711 ) ) ;
#20482=LINE ( 'NONE', #16075, #15080 ) ;
#20487=CARTESIAN_POINT ( 'NONE',  ( 6.350852961086080661, -9.614813431917819062E-14, -142.8750000000000568 ) ) ;
#20488=EDGE_CURVE ( 'NONE', #15144, #9511, #28647, .T. ) ;
#20491=ORIENTED_EDGE ( 'NONE', *, *, #8586, .F. ) ;
#20492=CARTESIAN_POINT ( 'NONE',  ( 4.763139720814407951, -2.749999999999988454, -75.50000000000001421 ) ) ;
#20494=CARTESIAN_POINT ( 'NONE',  ( 3.608439182435180470, 6.249999999999982236, -87.55801270189222407 ) ) ;
#20496=CARTESIAN_POINT ( 'NONE',  ( -0.4021627495782659767, -10.99447802115039075, -19.01010557178162941 ) ) ;
#20497=CARTESIAN_POINT ( 'NONE',  ( -3.464101615137725076, 5.999999999999979572, -150.1636751345947971 ) ) ;
#20499=CYLINDRICAL_SURFACE ( 'NONE', #4455, 6.000000000000000888 ) ;
#20504=CARTESIAN_POINT ( 'NONE',  ( -3.175426480542816066, 5.499999999999865885, -152.8749999999999716 ) ) ;
#20506=CARTESIAN_POINT ( 'NONE',  ( -5.630955349224697315, 2.071796769723730058, -179.9999999999999432 ) ) ;
#20507=CARTESIAN_POINT ( 'NONE',  ( -3.175426480542816066, 5.499999999999865885, -85.37500000000004263 ) ) ;
#20509=CARTESIAN_POINT ( 'NONE',  ( 3.175426480543072749, -5.500000000000105693, -74.12500000000007105 ) ) ;
#20515=CARTESIAN_POINT ( 'NONE',  ( -5.999999999999919176, 1.607695154586804565, -103.4806624327025872 ) ) ;
#20517=EDGE_CURVE ( 'NONE', #16280, #3063, #11859, .T. ) ;
#20519=B_SPLINE_CURVE_WITH_KNOTS ( 'NONE', 2,
 ( #561, #5011, #23635 ),
 .UNSPECIFIED., .F., .F.,
 ( 3, 3 ),
 ( 0.000000000000000000, 1.000000000000000000 ),
 .UNSPECIFIED. ) ;
#20521=CARTESIAN_POINT ( 'NONE',  ( 5.196152422706629359, 3.000000000000002665, -139.4613248654052029 ) ) ;
#20522=( BOUNDED_CURVE ( )  B_SPLINE_CURVE ( 2, ( #26237, #19644, #14602, #23954, #2892, #3040, #26534, #12312, #28831 ),
 .UNSPECIFIED., .F., .T. ) 
 B_SPLINE_CURVE_WITH_KNOTS ( ( 3, 2, 2, 2, 3 ),
 ( 0.7194444444444444420, 0.7203703703703703276, 0.7222222222222222099, 0.7240740740740740922, 0.7249999999999999778 ),
 .UNSPECIFIED. ) 
 CURVE ( )  GEOMETRIC_REPRESENTATION_ITEM ( )  RATIONAL_B_SPLINE_CURVE ( ( 0.9330127018922194093, 0.9330127018922194093, 1.000000000000000000, 0.8660254037844388186, 1.000000000000000000, 0.8660254037844388186, 1.000000000000000000, 0.9330127018922234061, 0.9330127018922194093 ) ) 
 REPRESENTATION_ITEM ( '' )  );
#20529=EDGE_CURVE ( 'NONE', #5997, #23417, #8777, .T. ) ;
#20531=ADVANCED_FACE ( 'NONE', ( #14034, #11879 ), #2746, .F. ) ;
#20533=CARTESIAN_POINT ( 'NONE',  ( 4.763139720814407951, -2.749999999999988454, -98.00000000000002842 ) ) ;
#20534=CARTESIAN_POINT ( 'NONE',  ( 3.464101615137852974, 5.999999999999884537, -70.91367513459481131 ) ) ;
#20535=CARTESIAN_POINT ( 'NONE',  ( -5.412658773652684552, -3.125000000000099920, -107.9330127018922667 ) ) ;
#20537=CARTESIAN_POINT ( 'NONE',  ( 0.4021627495783208772, 10.99447802115039075, -19.01010557178162941 ) ) ;
#20539=CARTESIAN_POINT ( 'NONE',  ( -3.175426480542816510, -5.500000000000057732, -165.8750000000000568 ) ) ;
#20540=CARTESIAN_POINT ( 'NONE',  ( 6.000000000000000888, 1.743066579297358182E-13, -57.08632486540521001 ) ) ;
#20541=VERTEX_POINT ( 'NONE', #20104 ) ;
#20542=DIRECTION ( 'NONE',  ( 1.000000000000000000, -5.551115123125773458E-17, -1.260129944081490338E-35 ) ) ;
#20543=DIRECTION ( 'NONE',  ( -7.147005652999508048E-36, 5.642372883946980038E-36, 1.000000000000000000 ) ) ;
#20544=CARTESIAN_POINT ( 'NONE',  ( 3.175426480543072749, 5.499999999999865885, -159.1250000000000000 ) ) ;
#20546=CARTESIAN_POINT ( 'NONE',  ( -6.350852961085760029, -1.281975124255709124E-13, -109.1250000000000426 ) ) ;
#20547=LINE ( 'NONE', #22558, #2164 ) ;
#20548=CARTESIAN_POINT ( 'NONE',  ( -6.000000000000000888, 1.067854986875958443E-15, 7.560779664488942560E-35 ) ) ;
#20549=CARTESIAN_POINT ( 'NONE',  ( 3.175426480543072749, 5.499999999999865885, -100.6250000000000000 ) ) ;
#20551=PRESENTATION_STYLE_ASSIGNMENT (( #24985 ) ) ;
#20558=CYLINDRICAL_SURFACE ( 'NONE', #10569, 6.000000000000000888 ) ;
#20562=CARTESIAN_POINT ( 'NONE',  ( 5.412658773652712085, -3.125000000000086153, -91.56698729810786119 ) ) ;
#20564=ADVANCED_FACE ( 'NONE', ( #6114 ), #20558, .T. ) ;
#20565=CARTESIAN_POINT ( 'NONE',  ( -5.196152422706573404, -3.000000000000002665, -65.78867513459485394 ) ) ;
#20571=( BOUNDED_CURVE ( )  B_SPLINE_CURVE ( 2, ( #6384, #23276, #8394, #17801, #22383, #6091, #29590, #16382, #25117 ),
 .UNSPECIFIED., .F., .F. ) 
 B_SPLINE_CURVE_WITH_KNOTS ( ( 3, 2, 2, 2, 3 ),
 ( 0.3527777777777778567, 0.3537037037037037424, 0.3555555555555555136, 0.3574074074074073959, 0.3583333333333332815 ),
 .UNSPECIFIED. ) 
 CURVE ( )  GEOMETRIC_REPRESENTATION_ITEM ( )  RATIONAL_B_SPLINE_CURVE ( ( 0.9330127018922194093, 0.9330127018922234061, 1.000000000000000000, 0.8660254037844388186, 1.000000000000000000, 0.8660254037844388186, 1.000000000000000000, 0.9330127018922234061, 0.9330127018922194093 ) ) 
 REPRESENTATION_ITEM ( '' )  );
#20572=CARTESIAN_POINT ( 'NONE',  ( 4.763139720814407951, 2.750000000000002665, -120.2500000000000284 ) ) ;
#20573=CARTESIAN_POINT ( 'NONE',  ( 5.412658773652712085, -3.125000000000086153, -131.4330127018922383 ) ) ;
#20574=VERTEX_POINT ( 'NONE', #22410 ) ;
#20575=CARTESIAN_POINT ( 'NONE',  ( -3.464101615137725076, 5.999999999999979572, -160.6636751345948824 ) ) ;
#20576=CARTESIAN_POINT ( 'NONE',  ( 3.608439182435180470, 6.249999999999982236, -119.6919872981077901 ) ) ;
#20577=CARTESIAN_POINT ( 'NONE',  ( -7.216878364870328078, 0.000000000000000000, -179.1919872981078754 ) ) ;
#20587=CARTESIAN_POINT ( 'NONE',  ( 2.775557561562891351E-14, -6.250000000000061284, -72.31698729810781856 ) ) ;
#20588=CARTESIAN_POINT ( 'NONE',  ( -5.412658773652739619, 3.124999999999975131, -60.81698729810780435 ) ) ;
#20589=CARTESIAN_POINT ( 'NONE',  ( 3.175426480543072749, 5.499999999999865885, -46.62500000000006395 ) ) ;
#20591=CARTESIAN_POINT ( 'NONE',  ( -5.196152422706573404, -3.000000000000002665, -47.78867513459483973 ) ) ;
#20592=CARTESIAN_POINT ( 'NONE',  ( 3.175426480543072749, -5.500000000000105693, -123.6250000000000426 ) ) ;
#20593=CARTESIAN_POINT ( 'NONE',  ( -5.999999999999963585, -1.487416814333745711E-14, -50.33632486540523843 ) ) ;
#20597=EDGE_CURVE ( 'NONE', #2765, #16117, #25530, .T. ) ;
#20598=VECTOR ( 'NONE', #25670, 1000.000000000000000 ) ;
#20603=ORIENTED_EDGE ( 'NONE', *, *, #15927, .F. ) ;
#20605=DIRECTION ( 'NONE',  ( -7.147005652999508048E-36, 5.642372883946980038E-36, 1.000000000000000000 ) ) ;
#20608=CARTESIAN_POINT ( 'NONE',  ( -7.216878364870328078, 0.000000000000000000, -119.1919872981078470 ) ) ;
#20611=VERTEX_POINT ( 'NONE', #28055 ) ;
#20613=DIRECTION ( 'NONE',  ( 1.000000000000000000, -5.551115123125773458E-17, -1.260129944081490338E-35 ) ) ;
#20615=( BOUNDED_CURVE ( )  B_SPLINE_CURVE ( 2, ( #26926, #17456, #5888, #3584, #10698, #1131, #26770, #19594, #28777 ),
 .UNSPECIFIED., .F., .T. ) 
 B_SPLINE_CURVE_WITH_KNOTS ( ( 3, 2, 2, 2, 3 ),
 ( 0.3694444444444443532, 0.3703703703703703498, 0.3722222222222222321, 0.3740740740740741144, 0.3750000000000000000 ),
 .UNSPECIFIED. ) 
 CURVE ( )  GEOMETRIC_REPRESENTATION_ITEM ( )  RATIONAL_B_SPLINE_CURVE ( ( 0.9330127018922194093, 0.9330127018922154125, 1.000000000000000000, 0.8660254037844388186, 1.000000000000000000, 0.8660254037844388186, 1.000000000000000000, 0.9330127018922194093, 0.9330127018922194093 ) ) 
 REPRESENTATION_ITEM ( '' )  );
#20616=EDGE_LOOP ( 'NONE', ( #16891, #13770, #132, #1814 ) ) ;
#20617=CARTESIAN_POINT ( 'NONE',  ( -7.216878364870328078, 0.000000000000000000, -149.1919872981077901 ) ) ;
#20623=CARTESIAN_POINT ( 'NONE',  ( 6.000000000000000888, 7.762456499804235646E-14, -144.0863248654052313 ) ) ;
#20624=CARTESIAN_POINT ( 'NONE',  ( 5.412658773652712085, -3.125000000000086153, -63.93301270189222407 ) ) ;
#20626=( BOUNDED_CURVE ( )  B_SPLINE_CURVE ( 2, ( #1133, #18072, #3743, #29232, #20046, #24939, #26928, #22661, #3586 ),
 .UNSPECIFIED., .F., .T. ) 
 B_SPLINE_CURVE_WITH_KNOTS ( ( 3, 2, 2, 2, 3 ),
 ( 0.3861111111111111827, 0.3870370370370370683, 0.3888888888888888395, 0.3907407407407407218, 0.3916666666666666075 ),
 .UNSPECIFIED. ) 
 CURVE ( )  GEOMETRIC_REPRESENTATION_ITEM ( )  RATIONAL_B_SPLINE_CURVE ( ( 0.9330127018922194093, 0.9330127018922234061, 1.000000000000000000, 0.8660254037844388186, 1.000000000000000000, 0.8660254037844388186, 1.000000000000000000, 0.9330127018922234061, 0.9330127018922194093 ) ) 
 REPRESENTATION_ITEM ( '' )  );
#20630=CARTESIAN_POINT ( 'NONE',  ( 6.000000000000014211, -1.607695154586730180, -155.2306624327026441 ) ) ;
#20635=CARTESIAN_POINT ( 'NONE',  ( 3.175426480543072749, 5.499999999999865885, -124.6250000000000426 ) ) ;
#20639=EDGE_CURVE ( 'NONE', #12335, #28056, #4412, .T. ) ;
#20640=CARTESIAN_POINT ( 'NONE',  ( -3.175426480542816066, 5.499999999999865885, -55.37500000000003553 ) ) ;
#20641=DIRECTION ( 'NONE',  ( 1.000000000000000000, -5.551115123125773458E-17, -1.260129944081490338E-35 ) ) ;
#20642=LINE ( 'NONE', #6189, #27228 ) ;
#20645=ORIENTED_EDGE ( 'NONE', *, *, #4170, .F. ) ;
#20650=LINE ( 'NONE', #16374, #7694 ) ;
#20651=CARTESIAN_POINT ( 'NONE',  ( -3.175426480542816510, 5.499999999999865885, -136.3750000000000568 ) ) ;
#20652=VERTEX_POINT ( 'NONE', #9036 ) ;
#20655=CARTESIAN_POINT ( 'NONE',  ( 6.350852961086080661, -9.614813431917819062E-14, -63.37500000000001421 ) ) ;
#20657=CARTESIAN_POINT ( 'NONE',  ( -3.608439182435052128, -6.250000000000110134, -89.80801270189225249 ) ) ;
#20659=CARTESIAN_POINT ( 'NONE',  ( -6.000643140593883373, -9.219125907743269011, -25.38858793365676192 ) ) ;
#20660=FACE_OUTER_BOUND ( 'NONE', #18237, .T. ) ;
#20664=CARTESIAN_POINT ( 'NONE',  ( -4.763139720814407951, 2.749999999999946709, -148.2500000000000000 ) ) ;
#20666=CARTESIAN_POINT ( 'NONE',  ( 2.775557561562891351E-14, -6.250000000000061284, -161.6830127018922383 ) ) ;
#20668=DIRECTION ( 'NONE',  ( -7.147005652999508048E-36, 5.642372883946980038E-36, 1.000000000000000000 ) ) ;
#20669=CARTESIAN_POINT ( 'NONE',  ( -4.763139720814407951, -2.750000000000016431, -73.00000000000001421 ) ) ;
#20671=CARTESIAN_POINT ( 'NONE',  ( -6.000000000000007105, -1.607695154586655129, -74.84668783648703538 ) ) ;
#20676=CARTESIAN_POINT ( 'NONE',  ( -5.999999999999963585, -1.487416814333745711E-14, -71.91367513459482552 ) ) ;
#20685=AXIS2_PLACEMENT_3D ( 'NONE', #28865, #19384, #7978 ) ;
#20687=VERTEX_POINT ( 'NONE', #25448 ) ;
#20690=CARTESIAN_POINT ( 'NONE',  ( 0.000000000000000000, 5.499999999999991118, -99.00000000000002842 ) ) ;
#20691=CARTESIAN_POINT ( 'NONE',  ( -5.412658773652739619, 3.124999999999975131, -103.6830127018922241 ) ) ;
#20696=CARTESIAN_POINT ( 'NONE',  ( 4.763139720814407951, 2.750000000000002665, -163.7500000000000000 ) ) ;
#20697=CARTESIAN_POINT ( 'NONE',  ( 1.966823652257182253, -10.82907957849942981, -30.68208441639942308 ) ) ;
#20699=DIRECTION ( 'NONE',  ( 1.000000000000000000, -5.551115123125773458E-17, -1.260129944081490338E-35 ) ) ;
#20700=CARTESIAN_POINT ( 'NONE',  ( 0.000000000000000000, 0.000000000000000000, 0.000000000000000000 ) ) ;
#20701=CARTESIAN_POINT ( 'NONE',  ( -6.350852961085760029, -1.281975124255709124E-13, -170.6249999999999716 ) ) ;
#20702=CARTESIAN_POINT ( 'NONE',  ( -5.999999999999962697, 3.323446944526963891E-14, -155.9136751345948255 ) ) ;
#20704=CARTESIAN_POINT ( 'NONE',  ( 3.175426480543072749, -5.500000000000105693, -165.6250000000000000 ) ) ;
#20706=CARTESIAN_POINT ( 'NONE',  ( -3.175426480542816066, -5.500000000000057732, -111.8750000000000426 ) ) ;
#20709=CARTESIAN_POINT ( 'NONE',  ( -3.175426480542816510, 5.499999999999865885, -94.37500000000002842 ) ) ;
#20710=( BOUNDED_CURVE ( )  B_SPLINE_CURVE ( 2, ( #15393, #22121, #21681, #616, #28700, #17082, #5360, #14768, #5808 ),
 .UNSPECIFIED., .F., .T. ) 
 B_SPLINE_CURVE_WITH_KNOTS ( ( 3, 2, 2, 2, 3 ),
 ( 0.3750000000000000000, 0.3759259259259259411, 0.3777777777777777679, 0.3796296296296296502, 0.3805555555555555358 ),
 .UNSPECIFIED. ) 
 CURVE ( )  GEOMETRIC_REPRESENTATION_ITEM ( )  RATIONAL_B_SPLINE_CURVE ( ( 0.9330127018922194093, 0.9330127018922194093, 1.000000000000000000, 0.8660254037844388186, 1.000000000000000000, 0.8660254037844388186, 1.000000000000000000, 0.9330127018922214077, 0.9330127018922194093 ) ) 
 REPRESENTATION_ITEM ( '' )  );
#20711=EDGE_CURVE ( 'NONE', #4711, #3683, #1394, .T. ) ;
#20718=ORIENTED_EDGE ( 'NONE', *, *, #6195, .T. ) ;
#20722=CARTESIAN_POINT ( 'NONE',  ( -5.412658773652684552, -3.125000000000099920, -89.06698729810780435 ) ) ;
#20724=CARTESIAN_POINT ( 'NONE',  ( 6.000000000000000888, 1.743066579297358182E-13, -108.6636751345948255 ) ) ;
#20727=CARTESIAN_POINT ( 'NONE',  ( -4.763139720814407951, 2.749999999999946709, -124.2500000000000284 ) ) ;
#20729=CARTESIAN_POINT ( 'NONE',  ( -5.412658773652739619, 3.124999999999975131, -127.6830127018922525 ) ) ;
#20730=ORIENTED_EDGE ( 'NONE', *, *, #20343, .T. ) ;
#20732=CARTESIAN_POINT ( 'NONE',  ( -5.412658773652684552, -3.125000000000099920, -165.5669872981078186 ) ) ;
#20733=CARTESIAN_POINT ( 'NONE',  ( 2.775557561562891351E-14, 6.250000000000033751, -173.5669872981078186 ) ) ;
#20745=CARTESIAN_POINT ( 'NONE',  ( 3.608439182435180470, 6.249999999999982236, -74.69198729810781856 ) ) ;
#20746=CARTESIAN_POINT ( 'NONE',  ( 2.775557561562891351E-14, -6.250000000000061284, -63.31698729810780435 ) ) ;
#20747=CARTESIAN_POINT ( 'NONE',  ( 3.175426480543072749, -5.500000000000105693, -48.62500000000000711 ) ) ;
#20749=CARTESIAN_POINT ( 'NONE',  ( -6.000000000000007105, -1.607695154586655129, -153.7693375672974128 ) ) ;
#20750=CARTESIAN_POINT ( 'NONE',  ( 5.196152422706629359, 3.000000000000002665, -159.5386751345948539 ) ) ;
#20751=EDGE_CURVE ( 'NONE', #17680, #2251, #18885, .T. ) ;
#20752=CARTESIAN_POINT ( 'NONE',  ( 3.175426480543072749, -5.500000000000105693, -119.1250000000000142 ) ) ;
#20754=CARTESIAN_POINT ( 'NONE',  ( 4.763139720814407951, 2.750000000000002665, -154.7500000000000568 ) ) ;
#20759=CARTESIAN_POINT ( 'NONE',  ( 6.000000000000000888, 1.743066579297358182E-13, -55.58632486540519579 ) ) ;
#20764=CARTESIAN_POINT ( 'NONE',  ( 5.999999999999974243, 1.607695154586759934, -122.0966878364870496 ) ) ;
#20766=CARTESIAN_POINT ( 'NONE',  ( 2.775557561562891351E-14, -6.250000000000061284, -111.3169872981077901 ) ) ;
#20767=CARTESIAN_POINT ( 'NONE',  ( 6.000000000000004441, -1.607695154586747055, -176.2306624327026157 ) ) ;
#20768=LINE ( 'NONE', #29653, #14775 ) ;
#20773=CARTESIAN_POINT ( 'NONE',  ( 2.775557561562891351E-14, 6.250000000000033751, -50.56698729810782567 ) ) ;
#20774=CARTESIAN_POINT ( 'NONE',  ( -5.412658773652739619, 3.124999999999975131, -137.3169872981078186 ) ) ;
#20776=CARTESIAN_POINT ( 'NONE',  ( 6.000000000000000888, 1.607695154586715303, -151.5193375672974128 ) ) ;
#20780=CARTESIAN_POINT ( 'NONE',  ( -3.464101615137757051, -5.999999999999979572, -137.6636751345947971 ) ) ;
#20781=CARTESIAN_POINT ( 'NONE',  ( 5.412658773652712085, -3.125000000000086153, -68.43301270189222407 ) ) ;
#20784=CARTESIAN_POINT ( 'NONE',  ( 0.000000000000000000, 0.000000000000000000, 0.000000000000000000 ) ) ;
#20786=LINE ( 'NONE', #13905, #16377 ) ;
#20791=CARTESIAN_POINT ( 'NONE',  ( 3.175426480543072749, -5.500000000000105693, -125.1250000000000426 ) ) ;
#20793=CARTESIAN_POINT ( 'NONE',  ( -5.412658773652739619, 3.124999999999975131, -142.6830127018922099 ) ) ;
#20796=CARTESIAN_POINT ( 'NONE',  ( 4.763139720814407951, 2.750000000000002665, -54.25000000000002132 ) ) ;
#20797=CARTESIAN_POINT ( 'NONE',  ( 5.999999999999949374, -1.607695154586841868, -154.6533121635130215 ) ) ;
#20798=CARTESIAN_POINT ( 'NONE',  ( 5.196152422706629359, -2.999999999999988898, -76.71132486540521711 ) ) ;
#20799=CARTESIAN_POINT ( 'NONE',  ( 5.999999999999999112, 2.951592740943527306E-14, -151.5863248654052029 ) ) ;
#20800=EDGE_LOOP ( 'NONE', ( #16180, #24397, #3198 ) ) ;
#20804=DIRECTION ( 'NONE',  ( -7.147005652999508048E-36, 5.642372883946980038E-36, 1.000000000000000000 ) ) ;
#20807=VERTEX_POINT ( 'NONE', #16740 ) ;
#20808=CARTESIAN_POINT ( 'NONE',  ( 3.175426480543072749, -5.500000000000105693, -135.6250000000000000 ) ) ;
#20812=CARTESIAN_POINT ( 'NONE',  ( 6.350852961086080661, -9.614813431917819062E-14, -69.37500000000004263 ) ) ;
#20814=CARTESIAN_POINT ( 'NONE',  ( -6.000000000000000888, 1.067854986875958443E-15, 7.560779664488942560E-35 ) ) ;
#20818=DIRECTION ( 'NONE',  ( 1.000000000000000000, -5.551115123125773458E-17, -1.260129944081490338E-35 ) ) ;
#20820=CARTESIAN_POINT ( 'NONE',  ( 4.763139720814407951, -2.749999999999988454, -144.5000000000000284 ) ) ;
#20822=CARTESIAN_POINT ( 'NONE',  ( 4.763139720814407951, 2.750000000000002665, -142.7500000000000568 ) ) ;
#20823=CARTESIAN_POINT ( 'NONE',  ( 3.608439182435180470, -6.249999999999997335, -163.0580127018922099 ) ) ;
#20824=CARTESIAN_POINT ( 'NONE',  ( 3.044979857375308677E-14, 10.99999999999998224, -14.99152654425661702 ) ) ;
#20825=CARTESIAN_POINT ( 'NONE',  ( 3.175426480543072749, -5.500000000000105693, -81.62500000000002842 ) ) ;
#20826=DIRECTION ( 'NONE',  ( 1.000000000000000000, -5.551115123125773458E-17, -1.260129944081490338E-35 ) ) ;
#20827=CARTESIAN_POINT ( 'NONE',  ( -4.763139720814407951, -2.750000000000016431, -76.00000000000001421 ) ) ;
#20828=CARTESIAN_POINT ( 'NONE',  ( 6.000000000000052403, -1.607695154586662678, -156.1533121635129930 ) ) ;
#20829=CARTESIAN_POINT ( 'NONE',  ( -5.999999999999963585, -1.487416814333745711E-14, -88.41367513459482552 ) ) ;
#20830=DIRECTION ( 'NONE',  ( 1.000000000000000000, -5.551115123125773458E-17, -1.260129944081490338E-35 ) ) ;
#20834=CARTESIAN_POINT ( 'NONE',  ( -3.464101615137725076, 5.999999999999979572, -118.6636751345947829 ) ) ;
#20836=CARTESIAN_POINT ( 'NONE',  ( 0.000000000000000000, 0.000000000000000000, 0.000000000000000000 ) ) ;
#20837=ORIENTED_EDGE ( 'NONE', *, *, #28246, .F. ) ;
#20841=DIRECTION ( 'NONE',  ( -7.147005652999508048E-36, 5.642372883946980038E-36, 1.000000000000000000 ) ) ;
#20842=ORIENTED_EDGE ( 'NONE', *, *, #27637, .F. ) ;
#20844=EDGE_LOOP ( 'NONE', ( #6575, #9314, #6532 ) ) ;
#20845=CARTESIAN_POINT ( 'NONE',  ( -3.175426480542816510, 5.499999999999865885, -86.87500000000007105 ) ) ;
#20846=ADVANCED_FACE ( 'NONE', ( #559 ), #7617, .T. ) ;
#20847=CARTESIAN_POINT ( 'NONE',  ( -5.412658773652684552, -3.125000000000099920, -104.9330127018922525 ) ) ;
#20848=CARTESIAN_POINT ( 'NONE',  ( 0.000000000000000000, 5.999999999999977796, -52.21132486540525264 ) ) ;
#20849=CARTESIAN_POINT ( 'NONE',  ( 3.175426480543072749, 5.499999999999865885, -166.6249999999999716 ) ) ;
#20850=CARTESIAN_POINT ( 'NONE',  ( 5.801553858104719019, -9.346157964213302805, -26.58091173639827431 ) ) ;
#20852=FACE_OUTER_BOUND ( 'NONE', #1508, .T. ) ;
#20854=CARTESIAN_POINT ( 'NONE',  ( -4.763139720814407951, 2.749999999999946709, -173.7500000000000284 ) ) ;
#20855=DIRECTION ( 'NONE',  ( -7.147005652999508048E-36, 5.642372883946980038E-36, 1.000000000000000000 ) ) ;
#20856=CARTESIAN_POINT ( 'NONE',  ( 3.175426480543072749, 5.499999999999865885, -165.1249999999999716 ) ) ;
#20859=CARTESIAN_POINT ( 'NONE',  ( -4.763139720814407951, 2.749999999999946709, -104.7500000000000142 ) ) ;
#20860=CARTESIAN_POINT ( 'NONE',  ( -3.464101615137757051, -5.999999999999979572, -159.5863248654051176 ) ) ;
#20861=CARTESIAN_POINT ( 'NONE',  ( -5.999999999999963585, -1.487416814333745711E-14, -122.9136751345948255 ) ) ;
#20862=CARTESIAN_POINT ( 'NONE',  ( 4.763139720814407951, 2.750000000000002665, -100.7500000000000000 ) ) ;
#20870=CARTESIAN_POINT ( 'NONE',  ( 0.000000000000000000, -5.999999999999991118, -85.96132486540520290 ) ) ;
#20871=VERTEX_POINT ( 'NONE', #2707 ) ;
#20873=EDGE_CURVE ( 'NONE', #18702, #29957, #19039, .T. ) ;
#20877=VERTEX_POINT ( 'NONE', #28505 ) ;
#20879=CARTESIAN_POINT ( 'NONE',  ( -3.175426480542816510, -5.500000000000057732, -113.3750000000000568 ) ) ;
#20883=CARTESIAN_POINT ( 'NONE',  ( 5.412658773652712085, -3.125000000000086153, -134.4330127018922383 ) ) ;
#20884=ORIENTED_EDGE ( 'NONE', *, *, #17395, .T. ) ;
#20886=CARTESIAN_POINT ( 'NONE',  ( -7.216878364870328078, 0.000000000000000000, -168.6919872981078186 ) ) ;
#20887=CARTESIAN_POINT ( 'NONE',  ( -5.412658773652739619, 3.124999999999975131, -180.8169872981077901 ) ) ;
#20891=CARTESIAN_POINT ( 'NONE',  ( 6.000000000000000888, 7.762456499804235646E-14, -144.6636751345948255 ) ) ;
#20895=VECTOR ( 'NONE', #12926, 1000.000000000000000 ) ;
#20899=CARTESIAN_POINT ( 'NONE',  ( 5.412658773652739619, 3.124999999999988898, -73.31698729810781856 ) ) ;
#20900=CARTESIAN_POINT ( 'NONE',  ( -5.412658773652739619, 3.124999999999975131, -59.31698729810786119 ) ) ;
#20901=CARTESIAN_POINT ( 'NONE',  ( 6.000000000000000888, 1.743066579297358182E-13, -112.5863248654052029 ) ) ;
#20902=CARTESIAN_POINT ( 'NONE',  ( -7.216878364870328078, 0.000000000000000000, -181.5580127018922383 ) ) ;
#20904=CARTESIAN_POINT ( 'NONE',  ( -5.999999999999963585, -1.487416814333745711E-14, -71.91367513459482552 ) ) ;
#20905=CARTESIAN_POINT ( 'NONE',  ( -5.999999999999963585, -1.487416814333745711E-14, -71.33632486540521711 ) ) ;
#20906=CARTESIAN_POINT ( 'NONE',  ( -3.175426480542816510, 5.499999999999865885, -124.3749999999999858 ) ) ;
#20908=ORIENTED_EDGE ( 'NONE', *, *, #15386, .F. ) ;
#20911=LINE ( 'NONE', #9071, #6448 ) ;
#20915=ADVANCED_FACE ( 'NONE', ( #10252 ), #23920, .T. ) ;
#20916=CARTESIAN_POINT ( 'NONE',  ( 3.608439182435180470, 6.249999999999982236, -109.1919872981078043 ) ) ;
#20918=ORIENTED_EDGE ( 'NONE', *, *, #12545, .F. ) ;
#20919=DIRECTION ( 'NONE',  ( 1.000000000000000000, -5.551115123125773458E-17, -1.260129944081490338E-35 ) ) ;
#20920=ORIENTED_EDGE ( 'NONE', *, *, #27090, .T. ) ;
#20924=CARTESIAN_POINT ( 'NONE',  ( 2.775557561562891351E-14, 6.250000000000033751, -140.5669872981077901 ) ) ;
#20930=CARTESIAN_POINT ( 'NONE',  ( 2.775557561562891351E-14, 6.250000000000033751, -66.43301270189222407 ) ) ;
#20933=DIRECTION ( 'NONE',  ( -7.147005652999508048E-36, 5.642372883946980038E-36, 1.000000000000000000 ) ) ;
#20934=CARTESIAN_POINT ( 'NONE',  ( -5.999999999999963585, 1.780251999655701777E-13, -70.41367513459482552 ) ) ;
#20935=CARTESIAN_POINT ( 'NONE',  ( -5.999999999999963585, 1.607695154586726627, -164.9806624327025588 ) ) ;
#20939=DIRECTION ( 'NONE',  ( -7.147005652999508048E-36, 5.642372883946980038E-36, 1.000000000000000000 ) ) ;
#20940=CARTESIAN_POINT ( 'NONE',  ( -6.350852961085760029, -1.281975124255709124E-13, -125.6250000000000426 ) ) ;
#20941=CARTESIAN_POINT ( 'NONE',  ( -5.412658773652684552, -3.125000000000099920, -143.9330127018922383 ) ) ;
#20942=ORIENTED_EDGE ( 'NONE', *, *, #19889, .T. ) ;
#20944=CARTESIAN_POINT ( 'NONE',  ( -4.763139720814407951, -2.750000000000016431, -55.00000000000004974 ) ) ;
#20945=CARTESIAN_POINT ( 'NONE',  ( -3.464101615137725076, 5.999999999999979572, -124.0863248654052455 ) ) ;
#20946=CARTESIAN_POINT ( 'NONE',  ( -5.999999999999963585, 8.134310703387671600E-14, -120.8363248654052171 ) ) ;
#20947=CARTESIAN_POINT ( 'NONE',  ( 5.999999999999949374, -1.607695154586841868, -163.6533121635129646 ) ) ;
#20948=ORIENTED_EDGE ( 'NONE', *, *, #13140, .F. ) ;
#20951=EDGE_CURVE ( 'NONE', #18704, #21171, #264, .T. ) ;
#20952=CARTESIAN_POINT ( 'NONE',  ( 3.608439182435180470, -6.249999999999997335, -103.6919872981078470 ) ) ;
#20957=EDGE_CURVE ( 'NONE', #18615, #8469, #7914, .T. ) ;
#20958=CARTESIAN_POINT ( 'NONE',  ( 4.763139720814407951, 2.750000000000002665, -139.7500000000000284 ) ) ;
#20963=CARTESIAN_POINT ( 'NONE',  ( 4.763139720814407951, -2.749999999999988454, -62.00000000000000000 ) ) ;
#20966=CARTESIAN_POINT ( 'NONE',  ( -3.608439182435115633, 6.249999999999965361, -88.80801270189223828 ) ) ;
#20970=DIRECTION ( 'NONE',  ( -7.147005652999508048E-36, 5.642372883946980038E-36, 1.000000000000000000 ) ) ;
#20973=CARTESIAN_POINT ( 'NONE',  ( 0.000000000000000000, 5.499999999999991118, -150.0000000000000284 ) ) ;
#20975=AXIS2_PLACEMENT_3D ( 'NONE', #22741, #1684, #13551 ) ;
#20976=CARTESIAN_POINT ( 'NONE',  ( -4.763139720814407951, -2.750000000000016431, -134.5000000000000000 ) ) ;
#20977=CARTESIAN_POINT ( 'NONE',  ( 3.608439182435180470, -6.249999999999997335, -157.0580127018922383 ) ) ;
#20978=CARTESIAN_POINT ( 'NONE',  ( 0.000000000000000000, 0.000000000000000000, 0.000000000000000000 ) ) ;
#20979=LINE ( 'NONE', #25716, #7570 ) ;
#20981=CARTESIAN_POINT ( 'NONE',  ( -4.763139720814407951, 2.749999999999946709, -80.74999999999998579 ) ) ;
#20983=CARTESIAN_POINT ( 'NONE',  ( -6.350852961085760029, -1.281975124255709124E-13, -64.12500000000001421 ) ) ;
#20984=( BOUNDED_CURVE ( )  B_SPLINE_CURVE ( 2, ( #6831, #16257, #4531, #13956, #516, #19577, #5567, #2823, #14538 ),
 .UNSPECIFIED., .F., .F. ) 
 B_SPLINE_CURVE_WITH_KNOTS ( ( 3, 2, 2, 2, 3 ),
 ( 0.3527777777777778012, 0.3537037037037036868, 0.3555555555555555691, 0.3574074074074073959, 0.3583333333333333370 ),
 .UNSPECIFIED. ) 
 CURVE ( )  GEOMETRIC_REPRESENTATION_ITEM ( )  RATIONAL_B_SPLINE_CURVE ( ( 0.9330127018922194093, 0.9330127018922214077, 1.000000000000000000, 0.8660254037844388186, 1.000000000000000000, 0.8660254037844388186, 1.000000000000000000, 0.9330127018922194093, 0.9330127018922194093 ) ) 
 REPRESENTATION_ITEM ( '' )  );
#20986=CARTESIAN_POINT ( 'NONE',  ( 0.000000000000000000, -5.999999999999991118, -88.03867513459483973 ) ) ;
#20991=EDGE_CURVE ( 'NONE', #26834, #7517, #16954, .T. ) ;
#20992=CARTESIAN_POINT ( 'NONE',  ( -6.000000000000007105, -1.607695154586655129, -98.84668783648703538 ) ) ;
#20995=ADVANCED_FACE ( 'NONE', ( #12880 ), #8059, .T. ) ;
#21000=LINE ( 'NONE', #18095, #28328 ) ;
#21004=CARTESIAN_POINT ( 'NONE',  ( -4.763139720814407951, 2.749999999999946709, -86.75000000000000000 ) ) ;
#21005=CARTESIAN_POINT ( 'NONE',  ( 3.608439182435180470, -6.249999999999997335, -110.5580127018922241 ) ) ;
#21009=CARTESIAN_POINT ( 'NONE',  ( 6.000000000000000888, -1.859271017917181981E-14, -63.08632486540521711 ) ) ;
#21010=ORIENTED_EDGE ( 'NONE', *, *, #20991, .F. ) ;
#21011=CARTESIAN_POINT ( 'NONE',  ( 3.464101615137852974, 5.999999999999884537, -93.41367513459479710 ) ) ;
#21012=CARTESIAN_POINT ( 'NONE',  ( 4.763139720814407951, -2.749999999999988454, -168.4999999999999716 ) ) ;
#21013=CARTESIAN_POINT ( 'NONE',  ( 0.000000000000000000, 5.499999999999991118, -156.0000000000000284 ) ) ;
#21015=CARTESIAN_POINT ( 'NONE',  ( -4.763139720814407951, 2.749999999999946709, -103.2500000000000142 ) ) ;
#21016=CARTESIAN_POINT ( 'NONE',  ( 5.999999999999949374, 1.607695154586804565, -87.59668783648704959 ) ) ;
#21017=CARTESIAN_POINT ( 'NONE',  ( -6.350852961085760029, -1.281975124255709124E-13, -98.62500000000005684 ) ) ;
#21024=LINE ( 'NONE', #14147, #7036 ) ;
#21025=EDGE_CURVE ( 'NONE', #16384, #20652, #29718, .T. ) ;
#21028=EDGE_CURVE ( 'NONE', #11352, #8549, #22371, .T. ) ;
#21029=ORIENTED_EDGE ( 'NONE', *, *, #10694, .T. ) ;
#21030=DIRECTION ( 'NONE',  ( 1.000000000000000000, -5.551115123125774074E-17, -1.260129944081490338E-35 ) ) ;
#21031=DIRECTION ( 'NONE',  ( -7.147005652999508048E-36, 5.642372883946980038E-36, 1.000000000000000000 ) ) ;
#21033=( BOUNDED_CURVE ( )  B_SPLINE_CURVE ( 2, ( #25507, #11432, #9087, #4159, #4773, #9396, #30124, #20776, #10 ),
 .UNSPECIFIED., .F., .F. ) 
 B_SPLINE_CURVE_WITH_KNOTS ( ( 3, 2, 2, 2, 3 ),
 ( 0.7750000000000000222, 0.7759259259259259078, 0.7777777777777777901, 0.7796296296296296724, 0.7805555555555555580 ),
 .UNSPECIFIED. ) 
 CURVE ( )  GEOMETRIC_REPRESENTATION_ITEM ( )  RATIONAL_B_SPLINE_CURVE ( ( 0.9330127018922194093, 0.9330127018922194093, 1.000000000000000000, 0.8660254037844388186, 1.000000000000000000, 0.8660254037844388186, 1.000000000000000000, 0.9330127018922194093, 0.9330127018922194093 ) ) 
 REPRESENTATION_ITEM ( '' )  );
#21036=CARTESIAN_POINT ( 'NONE',  ( 5.196152422706629359, -2.999999999999988898, -141.2113248654052313 ) ) ;
#21039=CARTESIAN_POINT ( 'NONE',  ( -4.763139720814407951, 2.749999999999946709, -113.7500000000000142 ) ) ;
#21041=CARTESIAN_POINT ( 'NONE',  ( -3.608439182435052128, -6.250000000000110134, -128.8080127018922383 ) ) ;
#21044=CARTESIAN_POINT ( 'NONE',  ( 3.608439182435180470, 6.249999999999982236, -167.6919872981078186 ) ) ;
#21046=ORIENTED_EDGE ( 'NONE', *, *, #17183, .F. ) ;
#21047=CARTESIAN_POINT ( 'NONE',  ( -5.196152422706601826, 2.999999999999975131, -95.46132486540520290 ) ) ;
#21048=CARTESIAN_POINT ( 'NONE',  ( 6.000000000000000888, -6.507448562710137091E-15, -175.5863248654052029 ) ) ;
#21051=CARTESIAN_POINT ( 'NONE',  ( 3.608439182435180470, 6.249999999999982236, -174.5580127018922667 ) ) ;
#21053=CARTESIAN_POINT ( 'NONE',  ( -5.999999999999956479, -1.607695154586745057, -101.8466878364870354 ) ) ;
#21055=CARTESIAN_POINT ( 'NONE',  ( -2.775557561562891351E-14, -5.500000000000115463, -120.7500000000000284 ) ) ;
#21059=CARTESIAN_POINT ( 'NONE',  ( 6.000000000000000888, -3.330669073875464691E-16, -7.560779664488942560E-35 ) ) ;
#21060=CARTESIAN_POINT ( 'NONE',  ( -5.196152422706601826, 2.999999999999975131, -122.4613248654052313 ) ) ;
#21062=EDGE_CURVE ( 'NONE', #3053, #22801, #9117, .T. ) ;
#21063=ORIENTED_EDGE ( 'NONE', *, *, #25275, .F. ) ;
#21066=CARTESIAN_POINT ( 'NONE',  ( 5.412658773652739619, 3.124999999999988898, -107.8169872981078470 ) ) ;
#21071=DIRECTION ( 'NONE',  ( 1.000000000000000000, -5.551115123125773458E-17, -1.260129944081490338E-35 ) ) ;
#21073=VERTEX_POINT ( 'NONE', #12727 ) ;
#21075=( BOUNDED_CURVE ( )  B_SPLINE_CURVE ( 2, ( #16030, #18464, #2316, #29797, #29946, #25488, #27784, #11566, #4453 ),
 .UNSPECIFIED., .F., .T. ) 
 B_SPLINE_CURVE_WITH_KNOTS ( ( 3, 2, 2, 2, 3 ),
 ( 0.5638888888888888840, 0.5648148148148147696, 0.5666666666666666519, 0.5685185185185185341, 0.5694444444444444198 ),
 .UNSPECIFIED. ) 
 CURVE ( )  GEOMETRIC_REPRESENTATION_ITEM ( )  RATIONAL_B_SPLINE_CURVE ( ( 0.9330127018922194093, 0.9330127018922194093, 1.000000000000000000, 0.8660254037844388186, 1.000000000000000000, 0.8660254037844388186, 1.000000000000000000, 0.9330127018922234061, 0.9330127018922194093 ) ) 
 REPRESENTATION_ITEM ( '' )  );
#21076=CARTESIAN_POINT ( 'NONE',  ( 3.608439182435180470, -6.249999999999997335, -142.6919872981078186 ) ) ;
#21079=CARTESIAN_POINT ( 'NONE',  ( -5.196152422706573404, -3.000000000000002665, -93.71132486540523132 ) ) ;
#21081=CARTESIAN_POINT ( 'NONE',  ( -5.999999999999982236, -1.607695154586700426, -130.3466878364870638 ) ) ;
#21087=CARTESIAN_POINT ( 'NONE',  ( 0.000000000000000000, -5.999999999999991118, -146.5386751345948539 ) ) ;
#21088=ADVANCED_FACE ( 'NONE', ( #27405 ), #15801, .T. ) ;
#21089=CARTESIAN_POINT ( 'NONE',  ( 6.000000000000000888, -1.859271017917181981E-14, -101.1636751345948397 ) ) ;
#21090=FACE_OUTER_BOUND ( 'NONE', #28254, .T. ) ;
#21092=CARTESIAN_POINT ( 'NONE',  ( 0.000000000000000000, 0.000000000000000000, 0.000000000000000000 ) ) ;
#21094=COLOUR_RGB ( '', 0.72549020, 0.75294118, 0.79215686) ;
#21095=CARTESIAN_POINT ( 'NONE',  ( -5.999999999999963585, -1.487416814333745711E-14, -138.8363248654052597 ) ) ;
#21097=ORIENTED_EDGE ( 'NONE', *, *, #12685, .F. ) ;
#21098=AXIS2_PLACEMENT_3D ( 'NONE', #19671, #7976, #5663 ) ;
#21099=CARTESIAN_POINT ( 'NONE',  ( -4.763139720814407951, 2.749999999999946709, -56.75000000000002132 ) ) ;
#21100=EDGE_CURVE ( 'NONE', #27213, #20652, #23228, .T. ) ;
#21101=EDGE_CURVE ( 'NONE', #8441, #9719, #18113, .T. ) ;
#21102=ORIENTED_EDGE ( 'NONE', *, *, #16411, .F. ) ;
#21105=CARTESIAN_POINT ( 'NONE',  ( 2.775557561562891351E-14, -6.250000000000061284, -106.8169872981078470 ) ) ;
#21110=CARTESIAN_POINT ( 'NONE',  ( -2.775557561562891351E-14, -5.500000000000115463, -134.2500000000000284 ) ) ;
#21112=CARTESIAN_POINT ( 'NONE',  ( -3.175426480542816510, 5.499999999999865885, -68.87500000000002842 ) ) ;
#21113=CARTESIAN_POINT ( 'NONE',  ( 5.196152422706629359, -2.999999999999988898, -81.21132486540521711 ) ) ;
#21114=LINE ( 'NONE', #28739, #26915 ) ;
#21115=CARTESIAN_POINT ( 'NONE',  ( 3.608439182435180470, -6.249999999999997335, -83.55801270189222407 ) ) ;
#21121=CARTESIAN_POINT ( 'NONE',  ( 0.000000000000000000, 5.499999999999991118, -145.5000000000000284 ) ) ;
#21123=CARTESIAN_POINT ( 'NONE',  ( 4.763139720814407951, -2.749999999999988454, -138.5000000000000000 ) ) ;
#21124=CARTESIAN_POINT ( 'NONE',  ( 7.216878364870455975, -6.409875621278545621E-14, -164.3080127018922951 ) ) ;
#21127=CARTESIAN_POINT ( 'NONE',  ( -4.763139720814407951, -2.750000000000016431, -79.00000000000001421 ) ) ;
#21128=ADVANCED_FACE ( 'NONE', ( #27255 ), #11021, .T. ) ;
#21129=CARTESIAN_POINT ( 'NONE',  ( -3.175426480542816510, 5.499999999999865885, -67.37500000000002842 ) ) ;
#21130=ADVANCED_FACE ( 'NONE', ( #6226 ), #15646, .T. ) ;
#21131=CARTESIAN_POINT ( 'NONE',  ( 6.000000000000000888, -3.330669073875464691E-16, -7.560779664488942560E-35 ) ) ;
#21133=CARTESIAN_POINT ( 'NONE',  ( 5.196152422706629359, -2.999999999999988898, -87.78867513459486815 ) ) ;
#21134=CARTESIAN_POINT ( 'NONE',  ( 0.000000000000000000, -5.999999999999991118, -144.4613248654052029 ) ) ;
#21137=CARTESIAN_POINT ( 'NONE',  ( 5.196152422706629359, -2.999999999999988898, -49.71132486540519579 ) ) ;
#21140=CARTESIAN_POINT ( 'NONE',  ( 6.000000000000000888, 1.743066579297358182E-13, -97.58632486540524553 ) ) ;
#21141=ORIENTED_EDGE ( 'NONE', *, *, #15461, .T. ) ;
#21144=CARTESIAN_POINT ( 'NONE',  ( -3.464101615137725076, 5.999999999999979572, -179.5863248654052029 ) ) ;
#21145=ORIENTED_EDGE ( 'NONE', *, *, #8147, .T. ) ;
#21148=ORIENTED_EDGE ( 'NONE', *, *, #29977, .F. ) ;
#21149=CARTESIAN_POINT ( 'NONE',  ( 4.763139720814407951, -2.749999999999988454, -86.00000000000001421 ) ) ;
#21150=CARTESIAN_POINT ( 'NONE',  ( -5.412658773652684552, -3.125000000000099920, -110.9330127018922667 ) ) ;
#21153=CARTESIAN_POINT ( 'NONE',  ( 0.4044047236351530628, 10.99999999999998224, -31.00000000000002842 ) ) ;
#21155=CARTESIAN_POINT ( 'NONE',  ( 6.350852961086080661, -9.614813431917819062E-14, -165.3750000000000284 ) ) ;
#21156=EDGE_CURVE ( 'NONE', #14326, #18615, #17127, .T. ) ;
#21157=CARTESIAN_POINT ( 'NONE',  ( 2.775557561562891351E-14, -6.250000000000061284, -47.68301270189223828 ) ) ;
#21158=CARTESIAN_POINT ( 'NONE',  ( 5.196152422706629359, 3.000000000000002665, -47.03867513459481131 ) ) ;
#21161=CARTESIAN_POINT ( 'NONE',  ( -4.763139720814407951, -2.750000000000016431, -172.0000000000000284 ) ) ;
#21163=CARTESIAN_POINT ( 'NONE',  ( -3.175426480542816510, 5.499999999999865885, -151.3749999999999716 ) ) ;
#21165=CARTESIAN_POINT ( 'NONE',  ( -6.350852961085760029, -1.281975124255709124E-13, -98.62500000000004263 ) ) ;
#21166=CARTESIAN_POINT ( 'NONE',  ( -5.196152422706601826, 2.999999999999975131, -59.46132486540523132 ) ) ;
#21167=EDGE_CURVE ( 'NONE', #26645, #4859, #16410, .T. ) ;
#21168=CARTESIAN_POINT ( 'NONE',  ( -6.350852961085760029, -1.281975124255709124E-13, -88.12500000000000000 ) ) ;
#21171=VERTEX_POINT ( 'NONE', #2090 ) ;
#21174=DIRECTION ( 'NONE',  ( -7.147005652999508048E-36, 5.642372883946980038E-36, 1.000000000000000000 ) ) ;
#21178=EDGE_LOOP ( 'NONE', ( #25791, #15896, #1962, #3920 ) ) ;
#21180=LINE ( 'NONE', #7477, #24094 ) ;
#21182=ORIENTED_EDGE ( 'NONE', *, *, #12516, .F. ) ;
#21183=DIRECTION ( 'NONE',  ( -7.147005652999508048E-36, 5.642372883946980038E-36, 1.000000000000000000 ) ) ;
#21186=ORIENTED_EDGE ( 'NONE', *, *, #9633, .T. ) ;
#21187=CARTESIAN_POINT ( 'NONE',  ( 6.350852961086080661, -9.614813431917819062E-14, -112.8750000000000568 ) ) ;
#21189=CARTESIAN_POINT ( 'NONE',  ( -3.608439182435052128, -6.250000000000110134, -134.8080127018922667 ) ) ;
#21191=CYLINDRICAL_SURFACE ( 'NONE', #939, 6.000000000000000888 ) ;
#21192=CARTESIAN_POINT ( 'NONE',  ( 2.775557561562891351E-14, 6.250000000000033751, -167.5669872981078186 ) ) ;
#21196=ADVANCED_FACE ( 'NONE', ( #25733 ), #14112, .T. ) ;
#21197=ORIENTED_EDGE ( 'NONE', *, *, #2815, .F. ) ;
#21200=CARTESIAN_POINT ( 'NONE',  ( 4.501142602643242618, 3.771550028933623011, -180.0000000000000853 ) ) ;
#21201=CARTESIAN_POINT ( 'NONE',  ( 0.000000000000000000, 5.999999999999977796, -136.7886751345947971 ) ) ;
#21202=CARTESIAN_POINT ( 'NONE',  ( -2.775557561562891351E-14, -5.500000000000115463, -179.2500000000000284 ) ) ;
#21204=CARTESIAN_POINT ( 'NONE',  ( -3.608439182435052128, -6.250000000000110134, -176.8080127018922099 ) ) ;
#21206=CARTESIAN_POINT ( 'NONE',  ( 6.000000000000000888, -3.330669073875464691E-16, -7.560779664488942560E-35 ) ) ;
#21208=CARTESIAN_POINT ( 'NONE',  ( 4.763139720814407951, -2.749999999999988454, -111.5000000000000426 ) ) ;
#21209=CARTESIAN_POINT ( 'NONE',  ( 5.196152422706629359, 3.000000000000002665, -166.4613248654052029 ) ) ;
#21213=CARTESIAN_POINT ( 'NONE',  ( 0.000000000000000000, -5.999999999999991118, -55.96132486540522422 ) ) ;
#21221=DIRECTION ( 'NONE',  ( -7.147005652999508048E-36, 5.642372883946980038E-36, 1.000000000000000000 ) ) ;
#21222=VERTEX_POINT ( 'NONE', #29873 ) ;
#21223=ORIENTED_EDGE ( 'NONE', *, *, #2389, .T. ) ;
#21226=CARTESIAN_POINT ( 'NONE',  ( 7.216878364870455975, -6.409875621278545621E-14, -139.4419872981078186 ) ) ;
#21227=LINE ( 'NONE', #11733, #27292 ) ;
#21228=CARTESIAN_POINT ( 'NONE',  ( 3.464101615137757051, -5.999999999999979572, -93.33632486540517448 ) ) ;
#21230=CARTESIAN_POINT ( 'NONE',  ( 6.000000000000000888, 5.577813053751546416E-15, -165.0863248654052313 ) ) ;
#21231=EDGE_CURVE ( 'NONE', #3131, #22297, #20255, .T. ) ;
#21238=SURFACE_STYLE_USAGE ( .BOTH. , #2485 ) ;
#21242=CARTESIAN_POINT ( 'NONE',  ( -4.763139720814407951, 2.749999999999946709, -58.25000000000002132 ) ) ;
#21243=CARTESIAN_POINT ( 'NONE',  ( -5.999999999999963585, 1.780251999655701777E-13, -62.33632486540522422 ) ) ;
#21244=( BOUNDED_CURVE ( )  B_SPLINE_CURVE ( 2, ( #14210, #2632, #25838, #9718, #30292, #11909, #9254, #14066, #9564 ),
 .UNSPECIFIED., .F., .T. ) 
 B_SPLINE_CURVE_WITH_KNOTS ( ( 3, 2, 2, 2, 3 ),
 ( 0.2416666666666666685, 0.2425925925925925819, 0.2444444444444444364, 0.2462962962962962910, 0.2472222222222222043 ),
 .UNSPECIFIED. ) 
 CURVE ( )  GEOMETRIC_REPRESENTATION_ITEM ( )  RATIONAL_B_SPLINE_CURVE ( ( 0.9330127018922194093, 0.9330127018922204085, 1.000000000000000000, 0.8660254037844388186, 1.000000000000000000, 0.8660254037844388186, 1.000000000000000000, 0.9330127018922205195, 0.9330127018922196314 ) ) 
 REPRESENTATION_ITEM ( '' )  );
#21245=CARTESIAN_POINT ( 'NONE',  ( 3.464101615137757051, -5.999999999999979572, -151.8363248654051745 ) ) ;
#21246=ORIENTED_EDGE ( 'NONE', *, *, #15537, .F. ) ;
#21249=CARTESIAN_POINT ( 'NONE',  ( -3.608439182435115633, 6.249999999999965361, -99.94198729810783277 ) ) ;
#21250=FACE_OUTER_BOUND ( 'NONE', #6415, .T. ) ;
#21255=CARTESIAN_POINT ( 'NONE',  ( -3.175426480542816510, -5.500000000000057732, -138.8750000000000568 ) ) ;
#21258=CARTESIAN_POINT ( 'NONE',  ( 3.464101615137852974, 5.999999999999884537, -163.3363248654052313 ) ) ;
#21259=CARTESIAN_POINT ( 'NONE',  ( 4.763139720814407951, 2.750000000000002665, -66.25000000000002842 ) ) ;
#21261=CARTESIAN_POINT ( 'NONE',  ( -5.412658773652739619, 3.124999999999975131, -79.68301270189226670 ) ) ;
#21264=CARTESIAN_POINT ( 'NONE',  ( -5.999999999999963585, -1.487416814333745711E-14, -139.4136751345948255 ) ) ;
#21268=CARTESIAN_POINT ( 'NONE',  ( -3.175426480542816066, 5.499999999999865885, -145.3750000000000000 ) ) ;
#21269=CARTESIAN_POINT ( 'NONE',  ( -5.412658773652739619, 3.124999999999975131, -154.6830127018922099 ) ) ;
#21270=CARTESIAN_POINT ( 'NONE',  ( 0.000000000000000000, 0.000000000000000000, 0.000000000000000000 ) ) ;
#21272=CARTESIAN_POINT ( 'NONE',  ( -4.763139720814407951, 2.749999999999946709, -79.25000000000004263 ) ) ;
#21273=CARTESIAN_POINT ( 'NONE',  ( -5.196152422706601826, 2.999999999999975131, -85.53867513459483973 ) ) ;
#21275=CARTESIAN_POINT ( 'NONE',  ( 6.350852961086080661, -9.614813431917819062E-14, -64.87500000000002842 ) ) ;
#21283=LINE ( 'NONE', #4533, #25349 ) ;
#21285=CARTESIAN_POINT ( 'NONE',  ( -3.464101615137757051, -5.999999999999979572, -145.1636751345948255 ) ) ;
#21290=EDGE_CURVE ( 'NONE', #19006, #6411, #24350, .T. ) ;
#21291=DIRECTION ( 'NONE',  ( -7.147005652999508048E-36, 5.642372883946980038E-36, 1.000000000000000000 ) ) ;
#21293=CARTESIAN_POINT ( 'NONE',  ( -3.608439182435052128, -6.250000000000110134, -151.9419872981077901 ) ) ;
#21294=ORIENTED_EDGE ( 'NONE', *, *, #15951, .T. ) ;
#21295=CARTESIAN_POINT ( 'NONE',  ( 4.763139720814407951, 2.750000000000002665, -88.75000000000000000 ) ) ;
#21298=CARTESIAN_POINT ( 'NONE',  ( -5.412658773652739619, 3.124999999999975131, -102.1830127018922241 ) ) ;
#21299=VERTEX_POINT ( 'NONE', #16110 ) ;
#21301=CARTESIAN_POINT ( 'NONE',  ( 5.676437577760689912, -9.422458200488941671, -23.04620489006167716 ) ) ;
#21303=CYLINDRICAL_SURFACE ( 'NONE', #7830, 6.000000000000000888 ) ;
#21305=CARTESIAN_POINT ( 'NONE',  ( 0.000000000000000000, 5.499999999999991118, -174.0000000000000568 ) ) ;
#21306=CARTESIAN_POINT ( 'NONE',  ( 5.999999999999949374, 1.607695154586804565, -162.0193375672974128 ) ) ;
#21307=CARTESIAN_POINT ( 'NONE',  ( 0.000000000000000000, 5.499999999999991118, -153.0000000000000284 ) ) ;
#21309=CARTESIAN_POINT ( 'NONE',  ( 4.763139720814407951, 2.750000000000002665, -99.25000000000000000 ) ) ;
#21312=CARTESIAN_POINT ( 'NONE',  ( 6.350852961086080661, -9.614813431917819062E-14, -156.3750000000000000 ) ) ;
#21313=CARTESIAN_POINT ( 'NONE',  ( -4.763139720814407951, 2.749999999999946709, -89.75000000000000000 ) ) ;
#21324=CARTESIAN_POINT ( 'NONE',  ( 6.000000000000000888, -1.859271017917181981E-14, -131.1636751345948539 ) ) ;
#21328=VECTOR ( 'NONE', #793, 1000.000000000000000 ) ;
#21329=VERTEX_POINT ( 'NONE', #27709 ) ;
#21332=CARTESIAN_POINT ( 'NONE',  ( -4.763139720814407951, -2.750000000000016431, -116.5000000000000426 ) ) ;
#21335=( BOUNDED_CURVE ( )  B_SPLINE_CURVE ( 2, ( #28939, #5143, #17315, #24046, #701, #26631, #19458, #16727, #26192 ),
 .UNSPECIFIED., .F., .T. ) 
 B_SPLINE_CURVE_WITH_KNOTS ( ( 3, 2, 2, 2, 3 ),
 ( 0.1027777777777777457, 0.1037037037037037424, 0.1055555555555555136, 0.1074074074074073959, 0.1083333333333333925 ),
 .UNSPECIFIED. ) 
 CURVE ( )  GEOMETRIC_REPRESENTATION_ITEM ( )  RATIONAL_B_SPLINE_CURVE ( ( 0.9330127018922194093, 0.9330127018922154125, 1.000000000000000000, 0.8660254037844388186, 1.000000000000000000, 0.8660254037844388186, 1.000000000000000000, 0.9330127018922154125, 0.9330127018922194093 ) ) 
 REPRESENTATION_ITEM ( '' )  );
#21336=CARTESIAN_POINT ( 'NONE',  ( 5.412658773652712085, -3.125000000000086153, -126.9330127018922809 ) ) ;
#21339=CARTESIAN_POINT ( 'NONE',  ( 2.775557561562891351E-14, -6.250000000000061284, -172.8169872981077901 ) ) ;
#21342=ORIENTED_EDGE ( 'NONE', *, *, #22189, .T. ) ;
#21345=CARTESIAN_POINT ( 'NONE',  ( -4.763139720814407951, -2.750000000000016431, -176.5000000000000000 ) ) ;
#21347=CARTESIAN_POINT ( 'NONE',  ( 3.608439182435180470, -6.249999999999997335, -173.5580127018922383 ) ) ;
#21348=CARTESIAN_POINT ( 'NONE',  ( -5.999999999999963585, -1.487416814333745711E-14, -75.83632486540521711 ) ) ;
#21349=CARTESIAN_POINT ( 'NONE',  ( 5.196152422706629359, -2.999999999999988898, -48.21132486540524553 ) ) ;
#21350=CARTESIAN_POINT ( 'NONE',  ( 6.000000000000000888, -3.330669073875464691E-16, -7.560779664488942560E-35 ) ) ;
#21352=CARTESIAN_POINT ( 'NONE',  ( -4.763139720814407951, -2.750000000000016431, -110.5000000000000426 ) ) ;
#21353=AXIS2_PLACEMENT_3D ( 'NONE', #15259, #7852, #17263 ) ;
#21355=CARTESIAN_POINT ( 'NONE',  ( 6.000000000000000888, 1.607695154586715303, -89.09668783648706381 ) ) ;
#21359=CARTESIAN_POINT ( 'NONE',  ( -5.999999999999963585, 1.780251999655701777E-13, -111.8363248654052313 ) ) ;
#21360=CARTESIAN_POINT ( 'NONE',  ( 5.999999999999949374, 1.607695154586804565, -132.0193375672974412 ) ) ;
#21361=ORIENTED_EDGE ( 'NONE', *, *, #18932, .F. ) ;
#21362=CARTESIAN_POINT ( 'NONE',  ( -6.350852961085760029, -1.281975124255709124E-13, -179.6249999999999716 ) ) ;
#21364=VECTOR ( 'NONE', #7473, 1000.000000000000000 ) ;
#21365=EDGE_CURVE ( 'NONE', #22419, #15757, #3173, .T. ) ;
#21366=CARTESIAN_POINT ( 'NONE',  ( -3.464101615137725076, 5.999999999999979572, -108.1636751345948397 ) ) ;
#21367=CARTESIAN_POINT ( 'NONE',  ( -5.196152422706573404, -3.000000000000002665, -77.78867513459481131 ) ) ;
#21368=ADVANCED_FACE ( 'NONE', ( #5274 ), #24026, .T. ) ;
#21370=FACE_OUTER_BOUND ( 'NONE', #1126, .T. ) ;
#21372=ORIENTED_EDGE ( 'NONE', *, *, #3884, .T. ) ;
#21375=ORIENTED_EDGE ( 'NONE', *, *, #22466, .T. ) ;
#21377=CARTESIAN_POINT ( 'NONE',  ( 3.608439182435180470, 6.249999999999982236, -137.6919872981078186 ) ) ;
#21379=CARTESIAN_POINT ( 'NONE',  ( -5.999999999999964473, 9.063946212346262433E-15, -174.8363248654052313 ) ) ;
#21380=CARTESIAN_POINT ( 'NONE',  ( -5.999999999999982236, -1.607695154586700426, -116.8466878364870638 ) ) ;
#21383=CARTESIAN_POINT ( 'NONE',  ( 7.147005652999508048E-33, -5.642372883946980038E-33, -1183.000000000000000 ) ) ;
#21390=CARTESIAN_POINT ( 'NONE',  ( 6.000000000000000888, 1.743066579297358182E-13, -60.66367513459481842 ) ) ;
#21393=( BOUNDED_CURVE ( )  B_SPLINE_CURVE ( 2, ( #30206, #16427, #21158, #25750, #4393 ),
 .UNSPECIFIED., .F., .F. ) 
 B_SPLINE_CURVE_WITH_KNOTS ( ( 3, 2, 3 ),
 ( 0.9972222222222222321, 0.9981481481481481177, 1.000000000000000000 ),
 .UNSPECIFIED. ) 
 CURVE ( )  GEOMETRIC_REPRESENTATION_ITEM ( )  RATIONAL_B_SPLINE_CURVE ( ( 0.9330127018922194093, 0.9330127018922194093, 1.000000000000000000, 0.8660254037844388186, 1.000000000000000000 ) ) 
 REPRESENTATION_ITEM ( '' )  );
#21394=CARTESIAN_POINT ( 'NONE',  ( 6.000000000000000888, 7.762456499804234384E-14, -142.5863248654051745 ) ) ;
#21396=CARTESIAN_POINT ( 'NONE',  ( 6.000000000000052403, -1.607695154586662678, -106.6533121635130072 ) ) ;
#21397=CARTESIAN_POINT ( 'NONE',  ( -5.999999999999963585, -1.487416814333745711E-14, -87.83632486540521711 ) ) ;
#21403=CARTESIAN_POINT ( 'NONE',  ( -7.216878364870328078, 0.000000000000000000, -102.6919872981078328 ) ) ;
#21408=CARTESIAN_POINT ( 'NONE',  ( -3.175426480542816510, -5.500000000000057732, -129.8750000000000284 ) ) ;
#21410=CARTESIAN_POINT ( 'NONE',  ( -5.999999999999962697, 3.323446944526963260E-14, -162.8363248654052313 ) ) ;
#21411=CARTESIAN_POINT ( 'NONE',  ( -3.175426480542816510, 5.499999999999865885, -59.87500000000005684 ) ) ;
#21412=CARTESIAN_POINT ( 'NONE',  ( -3.464101615137757051, -5.999999999999979572, -81.58632486540517448 ) ) ;
#21414=CARTESIAN_POINT ( 'NONE',  ( 3.608439182435180470, -6.249999999999997335, -86.55801270189223828 ) ) ;
#21418=CARTESIAN_POINT ( 'NONE',  ( 0.000000000000000000, -5.999999999999991118, -175.9613248654052313 ) ) ;
#21419=DIRECTION ( 'NONE',  ( 1.000000000000000000, -5.551115123125773458E-17, 0.000000000000000000 ) ) ;
#21421=( BOUNDED_CURVE ( )  B_SPLINE_CURVE ( 2, ( #10505, #19859, #28599, #8166, #26899, #7567, #26308, #16985, #11123 ),
 .UNSPECIFIED., .F., .T. ) 
 B_SPLINE_CURVE_WITH_KNOTS ( ( 3, 2, 2, 2, 3 ),
 ( 0.8305555555555556024, 0.8314814814814814881, 0.8333333333333333703, 0.8351851851851852526, 0.8361111111111111382 ),
 .UNSPECIFIED. ) 
 CURVE ( )  GEOMETRIC_REPRESENTATION_ITEM ( )  RATIONAL_B_SPLINE_CURVE ( ( 0.9330127018922194093, 0.9330127018922234061, 1.000000000000000000, 0.8660254037844388186, 1.000000000000000000, 0.8660254037844388186, 1.000000000000000000, 0.9330127018922194093, 0.9330127018922194093 ) ) 
 REPRESENTATION_ITEM ( '' )  );
#21422=CARTESIAN_POINT ( 'NONE',  ( 6.350852961086080661, -9.614813431917819062E-14, -141.3750000000000568 ) ) ;
#21424=CARTESIAN_POINT ( 'NONE',  ( -3.608439182435115633, 6.249999999999965361, -153.3080127018922383 ) ) ;
#21425=CARTESIAN_POINT ( 'NONE',  ( 3.464101615137757051, -5.999999999999979572, -72.91367513459482552 ) ) ;
#21426=EDGE_CURVE ( 'NONE', #24823, #18709, #23036, .T. ) ;
#21427=CARTESIAN_POINT ( 'NONE',  ( 4.763139720814407951, 2.750000000000002665, -70.75000000000002842 ) ) ;
#21429=DIRECTION ( 'NONE',  ( -7.147005652999508048E-36, 5.642372883946980038E-36, 1.000000000000000000 ) ) ;
#21430=CARTESIAN_POINT ( 'NONE',  ( 4.763139720814407951, 2.750000000000002665, -66.25000000000002842 ) ) ;
#21431=( BOUNDED_CURVE ( )  B_SPLINE_CURVE ( 2, ( #27329, #18310, #9064, #8920, #18457, #2157, #16175, #11404, #16022 ),
 .UNSPECIFIED., .F., .T. ) 
 B_SPLINE_CURVE_WITH_KNOTS ( ( 3, 2, 2, 2, 3 ),
 ( 0.5694444444444444198, 0.5703703703703704164, 0.5722222222222221877, 0.5740740740740740700, 0.5749999999999999556 ),
 .UNSPECIFIED. ) 
 CURVE ( )  GEOMETRIC_REPRESENTATION_ITEM ( )  RATIONAL_B_SPLINE_CURVE ( ( 0.9330127018922194093, 0.9330127018922154125, 1.000000000000000000, 0.8660254037844388186, 1.000000000000000000, 0.8660254037844388186, 1.000000000000000000, 0.9330127018922234061, 0.9330127018922194093 ) ) 
 REPRESENTATION_ITEM ( '' )  );
#21437=CARTESIAN_POINT ( 'NONE',  ( 6.000000000000000888, 1.743066579297358182E-13, -82.58632486540520290 ) ) ;
#21438=EDGE_CURVE ( 'NONE', #20404, #3063, #23596, .T. ) ;
#21439=ORIENTED_EDGE ( 'NONE', *, *, #24446, .F. ) ;
#21441=CARTESIAN_POINT ( 'NONE',  ( -2.775557561562891351E-14, -5.500000000000115463, -153.7500000000000568 ) ) ;
#21442=CARTESIAN_POINT ( 'NONE',  ( 3.464101615137757051, -5.999999999999979572, -158.4136751345948255 ) ) ;
#21443=CARTESIAN_POINT ( 'NONE',  ( -5.412658773652739619, 3.124999999999975131, -47.31698729810784698 ) ) ;
#21444=AXIS2_PLACEMENT_3D ( 'NONE', #19758, #29580, #8062 ) ;
#21446=CARTESIAN_POINT ( 'NONE',  ( -7.216878364870328078, 0.000000000000000000, -155.1919872981078186 ) ) ;
#21447=ORIENTED_EDGE ( 'NONE', *, *, #3884, .F. ) ;
#21448=CARTESIAN_POINT ( 'NONE',  ( 6.350852961086080661, -9.614813431917819062E-14, -91.87500000000001421 ) ) ;
#21449=CARTESIAN_POINT ( 'NONE',  ( 7.216878364870455975, -6.409875621278545621E-14, -102.8080127018922383 ) ) ;
#21450=ORIENTED_EDGE ( 'NONE', *, *, #28374, .T. ) ;
#21451=CARTESIAN_POINT ( 'NONE',  ( 3.464101615137852974, 5.999999999999884537, -147.4136751345947687 ) ) ;
#21453=VECTOR ( 'NONE', #10002, 1000.000000000000000 ) ;
#21456=CARTESIAN_POINT ( 'NONE',  ( -5.196152422706573404, -3.000000000000002665, -68.21132486540520290 ) ) ;
#21459=( NAMED_UNIT ( * ) SI_UNIT ( $, .STERADIAN. ) SOLID_ANGLE_UNIT ( ) );
#21460=CARTESIAN_POINT ( 'NONE',  ( -3.175426480542816066, 5.499999999999865885, -164.8750000000000568 ) ) ;
#21461=CARTESIAN_POINT ( 'NONE',  ( 0.000000000000000000, 5.999999999999977796, -58.21132486540525974 ) ) ;
#21462=CARTESIAN_POINT ( 'NONE',  ( 3.175426480543072749, 5.499999999999865885, -151.6250000000000284 ) ) ;
#21464=ADVANCED_FACE ( 'NONE', ( #16848 ), #21587, .T. ) ;
#21466=CARTESIAN_POINT ( 'NONE',  ( 5.196152422706629359, -2.999999999999988898, -51.78867513459483973 ) ) ;
#21468=CARTESIAN_POINT ( 'NONE',  ( 0.000000000000000000, 5.499999999999991118, -100.5000000000000284 ) ) ;
#21470=CARTESIAN_POINT ( 'NONE',  ( 4.763139720814407951, -2.749999999999988454, -90.50000000000002842 ) ) ;
#21473=DIRECTION ( 'NONE',  ( -7.147005652999508048E-36, 5.642372883946980038E-36, 1.000000000000000000 ) ) ;
#21476=CYLINDRICAL_SURFACE ( 'NONE', #3076, 6.000000000000000888 ) ;
#21477=CARTESIAN_POINT ( 'NONE',  ( -5.999999999999963585, -1.487416814333745711E-14, -71.91367513459482552 ) ) ;
#21478=ADVANCED_FACE ( 'NONE', ( #6795 ), #1731, .T. ) ;
#21480=ORIENTED_EDGE ( 'NONE', *, *, #11929, .T. ) ;
#21486=EDGE_LOOP ( 'NONE', ( #15823, #17062, #30229, #22262 ) ) ;
#21489=CARTESIAN_POINT ( 'NONE',  ( 6.350852961086080661, -9.614813431917819062E-14, -117.3750000000000142 ) ) ;
#21491=CARTESIAN_POINT ( 'NONE',  ( -5.412658773652739619, 3.124999999999975131, -123.1830127018922525 ) ) ;
#21493=CARTESIAN_POINT ( 'NONE',  ( -6.000000000000007105, -1.607695154586655129, -68.84668783648704959 ) ) ;
#21494=CARTESIAN_POINT ( 'NONE',  ( -7.216878364870328078, 0.000000000000000000, -164.1919872981078754 ) ) ;
#21498=ORIENTED_EDGE ( 'NONE', *, *, #25462, .T. ) ;
#21500=CARTESIAN_POINT ( 'NONE',  ( -3.973952007372655526, 10.26128916632344357, -20.48836482813350912 ) ) ;
#21501=CARTESIAN_POINT ( 'NONE',  ( 3.464101615137852974, 5.999999999999884537, -137.8363248654052313 ) ) ;
#21502=CARTESIAN_POINT ( 'NONE',  ( -3.175426480542816510, -5.500000000000057732, -179.3750000000000568 ) ) ;
#21504=CARTESIAN_POINT ( 'NONE',  ( 6.000000000000000888, 1.607695154586715303, -100.5193375672974270 ) ) ;
#21505=CARTESIAN_POINT ( 'NONE',  ( -5.412658773652684552, -3.125000000000099920, -176.9330127018922099 ) ) ;
#21506=DIRECTION ( 'NONE',  ( -7.147005652999508048E-36, 5.642372883946980038E-36, 1.000000000000000000 ) ) ;
#21507=EDGE_CURVE ( 'NONE', #14008, #7517, #20642, .T. ) ;
#21508=CARTESIAN_POINT ( 'NONE',  ( -5.196152422706573404, -3.000000000000002665, -48.71132486540518869 ) ) ;
#21509=CARTESIAN_POINT ( 'NONE',  ( 6.350852961086080661, -9.614813431917819062E-14, -121.8750000000000426 ) ) ;
#21510=CARTESIAN_POINT ( 'NONE',  ( -4.763139720814407951, -2.750000000000016431, -116.5000000000000426 ) ) ;
#21511=DIRECTION ( 'NONE',  ( -7.147005652999508048E-36, 5.642372883946980038E-36, 1.000000000000000000 ) ) ;
#21512=CARTESIAN_POINT ( 'NONE',  ( -3.464101615137757051, -5.999999999999979572, -131.6636751345948539 ) ) ;
#21515=CARTESIAN_POINT ( 'NONE',  ( -5.999999999999963585, -1.487416814333745711E-14, -126.8363248654052171 ) ) ;
#21516=CARTESIAN_POINT ( 'NONE',  ( -5.196152422706573404, -3.000000000000002665, -137.2113248654052029 ) ) ;
#21517=CARTESIAN_POINT ( 'NONE',  ( 6.000000000000000888, 7.762456499804234384E-14, -132.0863248654052313 ) ) ;
#21518=EDGE_CURVE ( 'NONE', #16922, #17680, #5388, .T. ) ;
#21519=ADVANCED_FACE ( 'NONE', ( #13600 ), #20329, .T. ) ;
#21522=CARTESIAN_POINT ( 'NONE',  ( -4.763139720814407951, -2.750000000000016431, -176.5000000000000000 ) ) ;
#21524=CARTESIAN_POINT ( 'NONE',  ( 6.000000000000052403, -1.607695154586662678, -77.23066243270261566 ) ) ;
#21525=( BOUNDED_CURVE ( )  B_SPLINE_CURVE ( 2, ( #3469, #29742, #27274, #24521, #6247, #8082, #1640, #18106, #29430 ),
 .UNSPECIFIED., .F., .T. ) 
 B_SPLINE_CURVE_WITH_KNOTS ( ( 3, 2, 2, 2, 3 ),
 ( 0.6638888888888889728, 0.6648148148148147474, 0.6666666666666667407, 0.6685185185185185119, 0.6694444444444445086 ),
 .UNSPECIFIED. ) 
 CURVE ( )  GEOMETRIC_REPRESENTATION_ITEM ( )  RATIONAL_B_SPLINE_CURVE ( ( 0.9330127018922194093, 0.9330127018922274029, 1.000000000000000000, 0.8660254037844388186, 1.000000000000000000, 0.8660254037844388186, 1.000000000000000000, 0.9330127018922154125, 0.9330127018922194093 ) ) 
 REPRESENTATION_ITEM ( '' )  );
#21531=CARTESIAN_POINT ( 'NONE',  ( -3.608439182435115633, 6.249999999999965361, -128.4419872981078186 ) ) ;
#21536=DIRECTION ( 'NONE',  ( -7.147005652999508048E-36, 5.642372883946980038E-36, 1.000000000000000000 ) ) ;
#21537=CARTESIAN_POINT ( 'NONE',  ( 5.196152422706629359, -2.999999999999988898, -91.71132486540523132 ) ) ;
#21542=CYLINDRICAL_SURFACE ( 'NONE', #7665, 6.000000000000000888 ) ;
#21545=EDGE_CURVE ( 'NONE', #10765, #29837, #23281, .T. ) ;
#21548=CARTESIAN_POINT ( 'NONE',  ( -4.763139720814407951, 2.749999999999946709, -49.25000000000001421 ) ) ;
#21551=CARTESIAN_POINT ( 'NONE',  ( -5.999999999999971578, 1.607695154586715303, -152.4033121635129930 ) ) ;
#21556=CARTESIAN_POINT ( 'NONE',  ( -3.608439182435115633, 6.249999999999965361, -102.9419872981078470 ) ) ;
#21559=CARTESIAN_POINT ( 'NONE',  ( -4.763139720814407951, 2.749999999999946709, -130.2500000000000284 ) ) ;
#21561=CARTESIAN_POINT ( 'NONE',  ( 6.000000000000000888, 1.743066579297358182E-13, -61.58632486540521001 ) ) ;
#21562=CARTESIAN_POINT ( 'NONE',  ( -2.775557561562891351E-14, -5.500000000000115463, -57.75000000000002132 ) ) ;
#21564=CARTESIAN_POINT ( 'NONE',  ( -5.196152422706573404, -3.000000000000002665, -81.71132486540521711 ) ) ;
#21566=CARTESIAN_POINT ( 'NONE',  ( 5.412658773652712085, -3.125000000000086153, -80.43301270189223828 ) ) ;
#21574=CARTESIAN_POINT ( 'NONE',  ( 3.175426480543072749, -5.500000000000105693, -138.6250000000000568 ) ) ;
#21575=LINE ( 'NONE', #28597, #24591 ) ;
#21576=CARTESIAN_POINT ( 'NONE',  ( -3.608439182435052128, -6.250000000000110134, -149.8080127018922667 ) ) ;
#21578=CARTESIAN_POINT ( 'NONE',  ( 3.175426480543072749, -5.500000000000105693, -71.12500000000004263 ) ) ;
#21579=CARTESIAN_POINT ( 'NONE',  ( -3.175426480542816510, -5.500000000000057732, -63.87500000000001421 ) ) ;
#21580=DIRECTION ( 'NONE',  ( -7.147005652999508048E-36, 5.642372883946980038E-36, 1.000000000000000000 ) ) ;
#21585=AXIS2_PLACEMENT_3D ( 'NONE', #26119, #5217, #7527 ) ;
#21586=CARTESIAN_POINT ( 'NONE',  ( 3.464101615137757051, -5.999999999999979572, -57.91367513459482552 ) ) ;
#21587=CYLINDRICAL_SURFACE ( 'NONE', #6173, 6.000000000000000888 ) ;
#21592=CARTESIAN_POINT ( 'NONE',  ( 6.000000000000000888, 1.743066579297358182E-13, -102.0863248654051887 ) ) ;
#21593=CARTESIAN_POINT ( 'NONE',  ( -3.175426480542816510, 5.499999999999865885, -176.8750000000000568 ) ) ;
#21596=CARTESIAN_POINT ( 'NONE',  ( 3.608439182435180470, -6.249999999999997335, -151.6919872981078186 ) ) ;
#21598=CARTESIAN_POINT ( 'NONE',  ( 6.350852961086080661, -9.614813431917819062E-14, -84.37500000000005684 ) ) ;
#21602=CARTESIAN_POINT ( 'NONE',  ( 6.000000000000000888, -6.507448562710137091E-15, -176.1636751345947971 ) ) ;
#21604=CARTESIAN_POINT ( 'NONE',  ( -3.464101615137725076, 5.999999999999979572, -58.66367513459482552 ) ) ;
#21609=EDGE_CURVE ( 'NONE', #21672, #15617, #15618, .T. ) ;
#21610=( BOUNDED_CURVE ( )  B_SPLINE_CURVE ( 2, ( #5033, #21053, #28381, #9675, #12310, #11708, #19352, #7361, #434 ),
 .UNSPECIFIED., .F., .T. ) 
 B_SPLINE_CURVE_WITH_KNOTS ( ( 3, 2, 2, 2, 3 ),
 ( 0.5916666666666666741, 0.5925925925925925597, 0.5944444444444444420, 0.5962962962962963243, 0.5972222222222222099 ),
 .UNSPECIFIED. ) 
 CURVE ( )  GEOMETRIC_REPRESENTATION_ITEM ( )  RATIONAL_B_SPLINE_CURVE ( ( 0.9330127018922194093, 0.9330127018922194093, 1.000000000000000000, 0.8660254037844388186, 1.000000000000000000, 0.8660254037844388186, 1.000000000000000000, 0.9330127018922194093, 0.9330127018922194093 ) ) 
 REPRESENTATION_ITEM ( '' )  );
#21611=CARTESIAN_POINT ( 'NONE',  ( 6.350852961086080661, -9.614813431917819062E-14, -166.8750000000000568 ) ) ;
#21613=CARTESIAN_POINT ( 'NONE',  ( 6.350852961086080661, -9.614813431917819062E-14, -153.3750000000000000 ) ) ;
#21615=CARTESIAN_POINT ( 'NONE',  ( 3.464101615137757051, -5.999999999999979572, -103.8363248654052171 ) ) ;
#21616=CARTESIAN_POINT ( 'NONE',  ( 4.763139720814407951, -2.749999999999988454, -93.50000000000002842 ) ) ;
#21618=CARTESIAN_POINT ( 'NONE',  ( 3.175426480543072749, 5.499999999999865885, -85.62500000000000000 ) ) ;
#21626=CARTESIAN_POINT ( 'NONE',  ( 0.000000000000000000, 0.000000000000000000, 0.000000000000000000 ) ) ;
#21631=ORIENTED_EDGE ( 'NONE', *, *, #12931, .T. ) ;
#21632=ORIENTED_EDGE ( 'NONE', *, *, #13594, .T. ) ;
#21635=CARTESIAN_POINT ( 'NONE',  ( -3.175426480542816510, -5.500000000000057732, -108.8750000000000426 ) ) ;
#21636=CARTESIAN_POINT ( 'NONE',  ( 3.608439182435180470, -6.249999999999997335, -124.0580127018922099 ) ) ;
#21637=EDGE_LOOP ( 'NONE', ( #24222, #20205, #14911, #9837 ) ) ;
#21639=CARTESIAN_POINT ( 'NONE',  ( -5.412658773652684552, -3.125000000000099920, -159.5669872981078186 ) ) ;
#21642=CARTESIAN_POINT ( 'NONE',  ( -3.608439182435115633, 6.249999999999965361, -63.30801270189224539 ) ) ;
#21643=ORIENTED_EDGE ( 'NONE', *, *, #26320, .F. ) ;
#21645=CARTESIAN_POINT ( 'NONE',  ( -3.675482141847861151, 10.37335300580275188, -20.24150316489821932 ) ) ;
#21647=CARTESIAN_POINT ( 'NONE',  ( -6.350852961085760029, -1.281975124255709124E-13, -175.1250000000000284 ) ) ;
#21650=CARTESIAN_POINT ( 'NONE',  ( -5.196152422706601826, 2.999999999999975131, -99.96132486540520290 ) ) ;
#21651=CARTESIAN_POINT ( 'NONE',  ( -5.412658773652684552, -3.125000000000099920, -178.4330127018922667 ) ) ;
#21654=CARTESIAN_POINT ( 'NONE',  ( -3.175426480542816066, -5.500000000000057732, -113.3750000000000568 ) ) ;
#21655=CARTESIAN_POINT ( 'NONE',  ( 11.00000000000001599, -6.106226635438360972E-16, -14.99152654425661702 ) ) ;
#21656=CARTESIAN_POINT ( 'NONE',  ( 6.350852961086080661, -9.614813431917819062E-14, -115.8750000000000000 ) ) ;
#21660=VERTEX_POINT ( 'NONE', #29 ) ;
#21664=VERTEX_POINT ( 'NONE', #16218 ) ;
#21665=CARTESIAN_POINT ( 'NONE',  ( -5.999999999999963585, -1.487416814333745711E-14, -126.8363248654052171 ) ) ;
#21669=ORIENTED_EDGE ( 'NONE', *, *, #12923, .T. ) ;
#21672=VERTEX_POINT ( 'NONE', #4639 ) ;
#21673=CARTESIAN_POINT ( 'NONE',  ( 5.999999999999949374, 1.607695154586804565, -85.51933756729742697 ) ) ;
#21675=ADVANCED_FACE ( 'NONE', ( #18804 ), #186, .T. ) ;
#21677=CARTESIAN_POINT ( 'NONE',  ( -3.608439182435115633, 6.249999999999965361, -134.4419872981077901 ) ) ;
#21681=CARTESIAN_POINT ( 'NONE',  ( 5.196152422706629359, 3.000000000000002665, -131.0386751345948824 ) ) ;
#21684=CARTESIAN_POINT ( 'NONE',  ( 0.000000000000000000, 5.999999999999977796, -135.2886751345948539 ) ) ;
#21686=CARTESIAN_POINT ( 'NONE',  ( 3.464101615137757051, -5.999999999999979572, -91.83632486540516027 ) ) ;
#21687=EDGE_CURVE ( 'NONE', #14008, #3491, #17998, .T. ) ;
#21690=CARTESIAN_POINT ( 'NONE',  ( 0.000000000000000000, 5.999999999999977796, -146.7113248654052313 ) ) ;
#21691=DIRECTION ( 'NONE',  ( 1.000000000000000000, -5.551115123125773458E-17, -1.260129944081490338E-35 ) ) ;
#21693=CARTESIAN_POINT ( 'NONE',  ( 0.000000000000000000, 5.499999999999991118, -141.0000000000000000 ) ) ;
#21694=AXIS2_PLACEMENT_3D ( 'NONE', #1299, #10712, #8526 ) ;
#21697=CARTESIAN_POINT ( 'NONE',  ( 0.000000000000000000, 5.499999999999991118, -51.00000000000004263 ) ) ;
#21698=DIRECTION ( 'NONE',  ( -7.147005652999508048E-36, 5.642372883946980038E-36, 1.000000000000000000 ) ) ;
#21700=( BOUNDED_CURVE ( )  B_SPLINE_CURVE ( 2, ( #1037, #20393, #22405, #29750, #6400, #8726, #6108, #24389, #24533 ),
 .UNSPECIFIED., .F., .T. ) 
 B_SPLINE_CURVE_WITH_KNOTS ( ( 3, 2, 2, 2, 3 ),
 ( 0.5138888888888888395, 0.5148148148148148362, 0.5166666666666667185, 0.5185185185185184897, 0.5194444444444444864 ),
 .UNSPECIFIED. ) 
 CURVE ( )  GEOMETRIC_REPRESENTATION_ITEM ( )  RATIONAL_B_SPLINE_CURVE ( ( 0.9330127018922194093, 0.9330127018922154125, 1.000000000000000000, 0.8660254037844388186, 1.000000000000000000, 0.8660254037844388186, 1.000000000000000000, 0.9330127018922154125, 0.9330127018922194093 ) ) 
 REPRESENTATION_ITEM ( '' )  );
#21701=CARTESIAN_POINT ( 'NONE',  ( 5.196152422706629359, 3.000000000000002665, -152.9613248654052597 ) ) ;
#21702=VERTEX_POINT ( 'NONE', #14364 ) ;
#21704=CARTESIAN_POINT ( 'NONE',  ( 5.412658773652712085, -3.125000000000086153, -99.06698729810781856 ) ) ;
#21705=DIRECTION ( 'NONE',  ( -7.147005652999508048E-36, 5.642372883946980038E-36, 1.000000000000000000 ) ) ;
#21708=CYLINDRICAL_SURFACE ( 'NONE', #9085, 6.000000000000000888 ) ;
#21710=CARTESIAN_POINT ( 'NONE',  ( 4.763139720814407951, -2.749999999999988454, -129.5000000000000000 ) ) ;
#21711=ORIENTED_EDGE ( 'NONE', *, *, #26401, .F. ) ;
#21713=CARTESIAN_POINT ( 'NONE',  ( -2.775557561562891351E-14, -5.500000000000115463, -60.75000000000002842 ) ) ;
#21714=FACE_OUTER_BOUND ( 'NONE', #18245, .T. ) ;
#21716=EDGE_CURVE ( 'NONE', #25854, #17182, #8296, .T. ) ;
#21717=CARTESIAN_POINT ( 'NONE',  ( 3.977757852569170804, 10.25981801084817135, -29.50831862515141069 ) ) ;
#21718=CARTESIAN_POINT ( 'NONE',  ( -5.412658773652684552, -3.125000000000099920, -86.93301270189223828 ) ) ;
#21719=CARTESIAN_POINT ( 'NONE',  ( 6.000000000000000888, -1.607695154586752384, -100.6533121635130072 ) ) ;
#21720=DIRECTION ( 'NONE',  ( -5.551115123125774074E-17, -1.000000000000000000, -6.394689268473234689E-36 ) ) ;
#21724=CARTESIAN_POINT ( 'NONE',  ( -3.175426480542816066, 5.499999999999865885, -136.3750000000000568 ) ) ;
#21726=CARTESIAN_POINT ( 'NONE',  ( 7.216878364870455975, -6.409875621278545621E-14, -150.8080127018922099 ) ) ;
#21727=CARTESIAN_POINT ( 'NONE',  ( 6.000000000000052403, -1.607695154586662678, -70.65331216351297883 ) ) ;
#21729=CARTESIAN_POINT ( 'NONE',  ( -3.175426480542816066, 5.499999999999865885, -67.37500000000002842 ) ) ;
#21730=CARTESIAN_POINT ( 'NONE',  ( 5.196152422706629359, 3.000000000000002665, -114.5386751345948113 ) ) ;
#21731=CARTESIAN_POINT ( 'NONE',  ( 6.350852961086080661, -9.614813431917819062E-14, -54.37500000000002842 ) ) ;
#21735=CARTESIAN_POINT ( 'NONE',  ( 0.000000000000000000, 0.000000000000000000, -44.99152654425658682 ) ) ;
#21737=CARTESIAN_POINT ( 'NONE',  ( 0.000000000000000000, -5.999999999999991118, -98.53867513459479710 ) ) ;
#21738=VECTOR ( 'NONE', #25677, 1000.000000000000000 ) ;
#21741=( BOUNDED_CURVE ( )  B_SPLINE_CURVE ( 2, ( #20246, #11037, #4241, #22548, #20382, #27571, #1482, #15971, #6551 ),
 .UNSPECIFIED., .F., .F. ) 
 B_SPLINE_CURVE_WITH_KNOTS ( ( 3, 2, 2, 2, 3 ),
 ( 0.8416666666666666741, 0.8425925925925925597, 0.8444444444444444420, 0.8462962962962963243, 0.8472222222222222099 ),
 .UNSPECIFIED. ) 
 CURVE ( )  GEOMETRIC_REPRESENTATION_ITEM ( )  RATIONAL_B_SPLINE_CURVE ( ( 0.9330127018922194093, 0.9330127018922194093, 1.000000000000000000, 0.8660254037844388186, 1.000000000000000000, 0.8660254037844388186, 1.000000000000000000, 0.9330127018922194093, 0.9330127018922194093 ) ) 
 REPRESENTATION_ITEM ( '' )  );
#21742=EDGE_CURVE ( 'NONE', #15338, #16735, #11494, .T. ) ;
#21745=CARTESIAN_POINT ( 'NONE',  ( 6.000000000000014211, -1.607695154586730180, -158.2306624327026441 ) ) ;
#21746=CARTESIAN_POINT ( 'NONE',  ( -6.350852961085760029, -1.281975124255709124E-13, -176.6250000000000568 ) ) ;
#21748=CARTESIAN_POINT ( 'NONE',  ( 5.412658773652739619, 3.124999999999988898, -152.8169872981078186 ) ) ;
#21749=ORIENTED_EDGE ( 'NONE', *, *, #15132, .T. ) ;
#21750=CARTESIAN_POINT ( 'NONE',  ( -2.775557561562891351E-14, -5.500000000000115463, -84.74999999999998579 ) ) ;
#21751=CARTESIAN_POINT ( 'NONE',  ( 3.608439182435180470, -6.249999999999997335, -103.0580127018922383 ) ) ;
#21753=CARTESIAN_POINT ( 'NONE',  ( -3.175426480542816510, 5.499999999999865885, -167.8750000000000568 ) ) ;
#21757=CARTESIAN_POINT ( 'NONE',  ( -6.350852961085760029, -1.281975124255709124E-13, -164.6249999999999716 ) ) ;
#21759=CARTESIAN_POINT ( 'NONE',  ( -4.763139720814407951, -2.750000000000016431, -146.5000000000000284 ) ) ;
#21761=CARTESIAN_POINT ( 'NONE',  ( -4.763139720814407951, 2.749999999999946709, -92.75000000000000000 ) ) ;
#21762=CARTESIAN_POINT ( 'NONE',  ( -5.999999999999963585, 9.296355089585909904E-15, -168.8363248654052029 ) ) ;
#21763=CARTESIAN_POINT ( 'NONE',  ( -2.775557561562891351E-14, -5.500000000000115463, -87.75000000000000000 ) ) ;
#21766=CYLINDRICAL_SURFACE ( 'NONE', #12611, 6.000000000000000888 ) ;
#21769=CARTESIAN_POINT ( 'NONE',  ( 3.464101615137757051, -5.999999999999979572, -73.83632486540521711 ) ) ;
#21772=CARTESIAN_POINT ( 'NONE',  ( 6.000000000000000888, 1.743066579297358182E-13, -83.16367513459481131 ) ) ;
#21776=( BOUNDED_CURVE ( )  B_SPLINE_CURVE ( 2, ( #13953, #14106, #6983, #70, #18688, #11640, #18384, #30026, #15946 ),
 .UNSPECIFIED., .F., .T. ) 
 B_SPLINE_CURVE_WITH_KNOTS ( ( 3, 2, 2, 2, 3 ),
 ( 0.5027777777777777679, 0.5037037037037037646, 0.5055555555555555358, 0.5074074074074074181, 0.5083333333333333037 ),
 .UNSPECIFIED. ) 
 CURVE ( )  GEOMETRIC_REPRESENTATION_ITEM ( )  RATIONAL_B_SPLINE_CURVE ( ( 0.9330127018922194093, 0.9330127018922194093, 1.000000000000000000, 0.8660254037844388186, 1.000000000000000000, 0.8660254037844388186, 1.000000000000000000, 0.9330127018922234061, 0.9330127018922194093 ) ) 
 REPRESENTATION_ITEM ( '' )  );
#21778=EDGE_LOOP ( 'NONE', ( #28960, #17977, #11845, #30197, #7953, #27988, #19667, #20730, #28428, #26395, #28837, #7253, #1822, #21632, #23004, #12326, #23409, #29543, #7883, #1041, #19921, #29179, #11528, #4541, #7438, #10811, #23076, #24358, #16454, #9231, #1519, #19244, #15691, #14263, #29140, #21029, #26071, #27611, #29506, #8034, #6695, #8289, #16145, #26883, #16639, #15183, #26747, #22804, #29253, #23897, #29762, #3008, #28065, #2754, #27186, #13693, #7235, #5415, #30348, #20942, #12250, #20196, #14295, #2097, #4739, #27346, #30121, #13421, #23815, #3839, #7875, #27896, #21342, #16276, #4231, #15983, #22768, #29187, #1383, #17073, #15659, #24751, #21375, #28176, #5761, #17520, #3275, #26179, #11835, #451, #23653, #9795, #7334, #1543, #9204, #12112, #13343, #27224, #30384, #28622, #28207, #13523, #13169, #6463, #10792, #27113, #18474, #16269, #22993, #10107, #23184, #1816, #6449, #9516, #10365, #4456, #11874, #11383, #21498, #19723, #19400, #20454, #7762, #15965, #20149, #29642, #4616, #4110, #7451, #3048, #12167, #30159, #24507, #6203, #859, #18283, #23272, #10510, #23309, #11286, #23029, #24548, #8704, #19915, #6244, #10985, #16034, #14614, #15062, #301, #20920, #15167, #19515, #2173, #14842, #13930, #19958, #27217, #16627, #2471, #18545, #6275, #13819, #16184, #19658, #26241, #10287, #13491, #18129, #11886, #5509, #1880, #26097, #7814, #4314, #25649, #22872, #15782, #1420, #6169, #13056, #24932 ) ) ;
#21781=CARTESIAN_POINT ( 'NONE',  ( 3.175426480543072749, -5.500000000000105693, -102.6250000000000000 ) ) ;
#21783=CARTESIAN_POINT ( 'NONE',  ( 2.775557561562891351E-14, 6.250000000000033751, -124.9330127018922809 ) ) ;
#21784=ORIENTED_EDGE ( 'NONE', *, *, #20711, .T. ) ;
#21785=CARTESIAN_POINT ( 'NONE',  ( 0.000000000000000000, 5.999999999999977796, -111.2886751345948397 ) ) ;
#21786=CARTESIAN_POINT ( 'NONE',  ( 5.412658773652712085, -3.125000000000086153, -159.0669872981078754 ) ) ;
#21788=CARTESIAN_POINT ( 'NONE',  ( 3.608439182435180470, -6.249999999999997335, -58.05801270189221697 ) ) ;
#21789=VERTEX_POINT ( 'NONE', #26716 ) ;
#21790=LINE ( 'NONE', #28972, #15739 ) ;
#21793=CARTESIAN_POINT ( 'NONE',  ( 3.175426480543072749, -5.500000000000105693, -180.6250000000000284 ) ) ;
#21795=CARTESIAN_POINT ( 'NONE',  ( 2.775557561562891351E-14, 6.250000000000033751, -166.9330127018922099 ) ) ;
#21799=CARTESIAN_POINT ( 'NONE',  ( 0.000000000000000000, 5.499999999999991118, -113.9999999999999858 ) ) ;
#21801=CARTESIAN_POINT ( 'NONE',  ( 3.175426480543072749, -5.500000000000105693, -116.1250000000000000 ) ) ;
#21804=ORIENTED_EDGE ( 'NONE', *, *, #8869, .F. ) ;
#21808=VERTEX_POINT ( 'NONE', #12350 ) ;
#21811=CARTESIAN_POINT ( 'NONE',  ( 6.000000000000000888, 1.607695154586715303, -110.0966878364870638 ) ) ;
#21812=VERTEX_POINT ( 'NONE', #1085 ) ;
#21820=ORIENTED_EDGE ( 'NONE', *, *, #27221, .T. ) ;
#21822=CARTESIAN_POINT ( 'NONE',  ( -7.216878364870328078, 0.000000000000000000, -134.1919872981078754 ) ) ;
#21824=CARTESIAN_POINT ( 'NONE',  ( -3.464101615137725076, 5.999999999999979572, -49.66367513459484684 ) ) ;
#21828=CARTESIAN_POINT ( 'NONE',  ( -6.000000000000000888, 1.067854986875958443E-15, 7.560779664488942560E-35 ) ) ;
#21836=CARTESIAN_POINT ( 'NONE',  ( -5.999999999999963585, -1.487416814333745711E-14, -122.3363248654052029 ) ) ;
#21837=CARTESIAN_POINT ( 'NONE',  ( 4.763139720814407951, -2.749999999999988454, -135.5000000000000000 ) ) ;
#21838=FACE_OUTER_BOUND ( 'NONE', #19962, .T. ) ;
#21839=ORIENTED_EDGE ( 'NONE', *, *, #22013, .F. ) ;
#21840=EDGE_CURVE ( 'NONE', #25123, #10004, #5530, .T. ) ;
#21841=CARTESIAN_POINT ( 'NONE',  ( 4.763139720814407951, -2.749999999999988454, -47.00000000000004263 ) ) ;
#21843=ORIENTED_EDGE ( 'NONE', *, *, #17359, .F. ) ;
#21846=CARTESIAN_POINT ( 'NONE',  ( 3.608439182435180470, -6.249999999999997335, -97.69198729810781856 ) ) ;
#21848=CARTESIAN_POINT ( 'NONE',  ( 6.000000000000052403, -1.607695154586662678, -78.15331216351297883 ) ) ;
#21853=CARTESIAN_POINT ( 'NONE',  ( 3.175426480543072749, 5.499999999999865885, -130.6250000000000284 ) ) ;
#21854=ORIENTED_EDGE ( 'NONE', *, *, #7678, .F. ) ;
#21857=CARTESIAN_POINT ( 'NONE',  ( 4.763139720814407951, 2.750000000000002665, -54.25000000000002132 ) ) ;
#21858=CARTESIAN_POINT ( 'NONE',  ( 6.000000000000000888, 1.743066579297358182E-13, -69.66367513459481131 ) ) ;
#21859=DIRECTION ( 'NONE',  ( 1.000000000000000000, -5.551115123125773458E-17, -1.260129944081490338E-35 ) ) ;
#21860=CARTESIAN_POINT ( 'NONE',  ( 2.693961096941849487, 10.67153403684353385, -19.62422301979503203 ) ) ;
#21862=CARTESIAN_POINT ( 'NONE',  ( 3.608439182435180470, -6.249999999999997335, -79.05801270189225249 ) ) ;
#21867=CARTESIAN_POINT ( 'NONE',  ( -5.196152422706601826, 2.999999999999975131, -60.96132486540523132 ) ) ;
#21870=CARTESIAN_POINT ( 'NONE',  ( -4.763139720814407951, -2.750000000000016431, -139.0000000000000000 ) ) ;
#21872=CARTESIAN_POINT ( 'NONE',  ( 3.608439182435180470, -6.249999999999997335, -154.0580127018922099 ) ) ;
#21873=FACE_OUTER_BOUND ( 'NONE', #1885, .T. ) ;
#21874=EDGE_CURVE ( 'NONE', #21808, #5958, #28721, .T. ) ;
#21875=CARTESIAN_POINT ( 'NONE',  ( 3.175426480543072749, 5.499999999999865885, -70.62500000000004263 ) ) ;
#21876=CARTESIAN_POINT ( 'NONE',  ( -3.175426480542816510, 5.499999999999865885, -61.37500000000000000 ) ) ;
#21881=CARTESIAN_POINT ( 'NONE',  ( -5.196152422706601826, 2.999999999999975131, -97.53867513459479710 ) ) ;
#21884=EDGE_CURVE ( 'NONE', #23373, #3569, #5325, .T. ) ;
#21888=CARTESIAN_POINT ( 'NONE',  ( 6.000000000000000888, 1.743066579297358182E-13, -71.16367513459481131 ) ) ;
#21890=CARTESIAN_POINT ( 'NONE',  ( 6.350852961086080661, -9.614813431917819062E-14, -175.8750000000000284 ) ) ;
#21892=ORIENTED_EDGE ( 'NONE', *, *, #27707, .F. ) ;
#21893=CARTESIAN_POINT ( 'NONE',  ( 2.775557561562891351E-14, 6.250000000000033751, -152.5669872981077901 ) ) ;
#21895=CARTESIAN_POINT ( 'NONE',  ( 4.763139720814407951, 2.750000000000002665, -81.25000000000004263 ) ) ;
#21898=CARTESIAN_POINT ( 'NONE',  ( -3.608439182435052128, -6.250000000000110134, -103.3080127018922383 ) ) ;
#21903=CARTESIAN_POINT ( 'NONE',  ( 2.686045755586594197, -10.67338275482132204, -19.62059632520456276 ) ) ;
#21906=CARTESIAN_POINT ( 'NONE',  ( -2.775557561562891351E-14, -5.500000000000115463, -167.2500000000000000 ) ) ;
#21907=CARTESIAN_POINT ( 'NONE',  ( -3.175426480542816510, -5.500000000000057732, -150.8750000000000000 ) ) ;
#21908=DIRECTION ( 'NONE',  ( 1.000000000000000000, -5.551115123125773458E-17, -1.260129944081490338E-35 ) ) ;
#21910=CARTESIAN_POINT ( 'NONE',  ( 4.763139720814407951, -2.749999999999988454, -92.00000000000002842 ) ) ;
#21911=CARTESIAN_POINT ( 'NONE',  ( 0.000000000000000000, 0.000000000000000000, 0.000000000000000000 ) ) ;
#21912=ADVANCED_FACE ( 'NONE', ( #6565 ), #16443, .T. ) ;
#21913=CARTESIAN_POINT ( 'NONE',  ( 3.175426480543072749, 5.499999999999865885, -78.12500000000001421 ) ) ;
#21914=DIRECTION ( 'NONE',  ( 1.000000000000000000, -5.551115123125773458E-17, -1.260129944081490338E-35 ) ) ;
#21922=FACE_BOUND ( 'NONE', #16640, .T. ) ;
#21923=CARTESIAN_POINT ( 'NONE',  ( -3.464101615137725076, 5.999999999999979572, -80.58632486540516027 ) ) ;
#21925=VERTEX_POINT ( 'NONE', #27031 ) ;
#21928=CARTESIAN_POINT ( 'NONE',  ( -6.350852961085760029, -1.281975124255709124E-13, -107.6250000000000426 ) ) ;
#21929=CARTESIAN_POINT ( 'NONE',  ( 7.216878364870455975, -6.409875621278545621E-14, -126.8080127018922383 ) ) ;
#21930=CARTESIAN_POINT ( 'NONE',  ( 6.000000000000052403, -1.607695154586662678, -60.73066243270260856 ) ) ;
#21931=CARTESIAN_POINT ( 'NONE',  ( 3.608439182435180470, 6.249999999999982236, -160.1919872981078470 ) ) ;
#21934=CARTESIAN_POINT ( 'NONE',  ( 5.412658773652712085, -3.125000000000086153, -56.43301270189227381 ) ) ;
#21935=ORIENTED_EDGE ( 'NONE', *, *, #18895, .F. ) ;
#21937=CARTESIAN_POINT ( 'NONE',  ( -1.580833713216677205, 10.88751498504595361, -19.20858708930976988 ) ) ;
#21938=CARTESIAN_POINT ( 'NONE',  ( 5.196152422706629359, 3.000000000000002665, -137.9613248654052313 ) ) ;
#21940=CARTESIAN_POINT ( 'NONE',  ( 6.350852961086080661, -9.614813431917819062E-14, -172.8750000000000284 ) ) ;
#21943=CARTESIAN_POINT ( 'NONE',  ( -5.412658773652684552, -3.125000000000099920, -167.9330127018922099 ) ) ;
#21947=CARTESIAN_POINT ( 'NONE',  ( -3.175426480542816066, 5.499999999999865885, -115.3750000000000000 ) ) ;
#21949=EDGE_CURVE ( 'NONE', #25259, #29296, #21024, .T. ) ;
#21950=CARTESIAN_POINT ( 'NONE',  ( -6.350852961085760029, -1.281975124255709124E-13, -107.6250000000000426 ) ) ;
#21951=VECTOR ( 'NONE', #1285, 1000.000000000000000 ) ;
#21952=CARTESIAN_POINT ( 'NONE',  ( 6.000000000000000888, -1.859271017917181981E-14, -101.1636751345948397 ) ) ;
#21955=CARTESIAN_POINT ( 'NONE',  ( 6.000000000000000888, 1.743066579297358182E-13, -75.66367513459485394 ) ) ;
#21956=( BOUNDED_CURVE ( )  B_SPLINE_CURVE ( 2, ( #19818, #781, #24261, #17541, #7826, #19387, #17242, #24125, #19238 ),
 .UNSPECIFIED., .F., .T. ) 
 B_SPLINE_CURVE_WITH_KNOTS ( ( 3, 2, 2, 2, 3 ),
 ( 0.8583333333333332815, 0.8592592592592592782, 0.8611111111111111605, 0.8629629629629629317, 0.8638888888888889284 ),
 .UNSPECIFIED. ) 
 CURVE ( )  GEOMETRIC_REPRESENTATION_ITEM ( )  RATIONAL_B_SPLINE_CURVE ( ( 0.9330127018922194093, 0.9330127018922154125, 1.000000000000000000, 0.8660254037844388186, 1.000000000000000000, 0.8660254037844388186, 1.000000000000000000, 0.9330127018922154125, 0.9330127018922194093 ) ) 
 REPRESENTATION_ITEM ( '' )  );
#21957=CARTESIAN_POINT ( 'NONE',  ( -5.999999999999919176, 1.607695154586804565, -86.40331216351303567 ) ) ;
#21959=CARTESIAN_POINT ( 'NONE',  ( -7.216878364870328078, 0.000000000000000000, -78.69198729810784698 ) ) ;
#21962=CARTESIAN_POINT ( 'NONE',  ( 6.000000000000000888, -3.330669073875464691E-16, -7.560779664488942560E-35 ) ) ;
#21963=VECTOR ( 'NONE', #29844, 1000.000000000000000 ) ;
#21967=CARTESIAN_POINT ( 'NONE',  ( 2.775557561562891351E-14, -6.250000000000061284, -132.3169872981078186 ) ) ;
#21969=CARTESIAN_POINT ( 'NONE',  ( 0.000000000000000000, 5.999999999999977796, -83.71132486540521711 ) ) ;
#21970=CARTESIAN_POINT ( 'NONE',  ( 6.000000000000000888, -1.859271017917181981E-14, -116.1636751345948255 ) ) ;
#21971=AXIS2_PLACEMENT_3D ( 'NONE', #9442, #11777, #11150 ) ;
#21972=ORIENTED_EDGE ( 'NONE', *, *, #3756, .F. ) ;
#21974=CARTESIAN_POINT ( 'NONE',  ( -5.999999999999963585, -1.487416814333745711E-14, -134.9136751345948255 ) ) ;
#21975=CARTESIAN_POINT ( 'NONE',  ( 5.196152422706629359, -2.999999999999988898, -138.7886751345947971 ) ) ;
#21978=CARTESIAN_POINT ( 'NONE',  ( 3.464101615137757051, -5.999999999999979572, -46.83632486540521001 ) ) ;
#21979=CARTESIAN_POINT ( 'NONE',  ( -5.412658773652684552, -3.125000000000099920, -69.56698729810784698 ) ) ;
#21980=CARTESIAN_POINT ( 'NONE',  ( -3.464101615137757051, -5.999999999999979572, -64.16367513459478289 ) ) ;
#21982=CARTESIAN_POINT ( 'NONE',  ( -5.999999999999971578, 1.607695154586715303, -127.4806624327025872 ) ) ;
#21983=EDGE_CURVE ( 'NONE', #341, #20441, #26387, .T. ) ;
#21984=CARTESIAN_POINT ( 'NONE',  ( 0.000000000000000000, 5.499999999999991118, -136.5000000000000000 ) ) ;
#21985=CARTESIAN_POINT ( 'NONE',  ( 3.464101615137852974, 5.999999999999884537, -166.9136751345947971 ) ) ;
#21986=ORIENTED_EDGE ( 'NONE', *, *, #27334, .T. ) ;
#21988=CARTESIAN_POINT ( 'NONE',  ( 3.175426480543072749, 5.499999999999865885, -46.62500000000006395 ) ) ;
#21989=CARTESIAN_POINT ( 'NONE',  ( 6.000000000000000888, -1.607695154586752384, -159.7306624327026157 ) ) ;
#21993=CARTESIAN_POINT ( 'NONE',  ( -5.412658773652684552, -3.125000000000099920, -98.06698729810780435 ) ) ;
#22000=EDGE_CURVE ( 'NONE', #15423, #17032, #25446, .T. ) ;
#22001=CARTESIAN_POINT ( 'NONE',  ( 4.763139720814407951, 2.750000000000002665, -58.75000000000002132 ) ) ;
#22002=CARTESIAN_POINT ( 'NONE',  ( -5.999999999999963585, 1.780251999655701777E-13, -68.91367513459482552 ) ) ;
#22003=CARTESIAN_POINT ( 'NONE',  ( -5.999999999999963585, 1.780251999655701777E-13, -62.33632486540522422 ) ) ;
#22004=CARTESIAN_POINT ( 'NONE',  ( 1.584453406822469601, 10.89233254831497177, -19.19936552286312903 ) ) ;
#22005=CARTESIAN_POINT ( 'NONE',  ( -5.412658773652684552, -3.125000000000099920, -77.93301270189223828 ) ) ;
#22008=FACE_OUTER_BOUND ( 'NONE', #18104, .T. ) ;
#22009=CARTESIAN_POINT ( 'NONE',  ( -5.999999999999919176, 1.607695154586804565, -79.48066243270261566 ) ) ;
#22011=CARTESIAN_POINT ( 'NONE',  ( -3.464101615137725076, 5.999999999999979572, -104.5863248654052029 ) ) ;
#22012=EDGE_CURVE ( 'NONE', #20142, #27374, #11369, .T. ) ;
#22013=EDGE_CURVE ( 'NONE', #1699, #25773, #12476, .T. ) ;
#22014=CARTESIAN_POINT ( 'NONE',  ( 6.350852961086080661, -9.614813431917819062E-14, -138.3750000000000568 ) ) ;
#22015=CARTESIAN_POINT ( 'NONE',  ( 3.464101615137852974, 5.999999999999884537, -68.83632486540518869 ) ) ;
#22016=LINE ( 'NONE', #5408, #5668 ) ;
#22017=CARTESIAN_POINT ( 'NONE',  ( 5.196152422706629359, 3.000000000000002665, -67.46132486540523132 ) ) ;
#22018=CARTESIAN_POINT ( 'NONE',  ( 3.175426480543072749, 5.499999999999865885, -72.12500000000005684 ) ) ;
#22019=CARTESIAN_POINT ( 'NONE',  ( 3.175426480543072749, 5.499999999999865885, -57.12500000000004974 ) ) ;
#22023=CARTESIAN_POINT ( 'NONE',  ( 3.464101615137852974, 5.999999999999884537, -97.91367513459481131 ) ) ;
#22027=ORIENTED_EDGE ( 'NONE', *, *, #27221, .F. ) ;
#22029=CARTESIAN_POINT ( 'NONE',  ( -5.999999999999963585, -1.487416814333745711E-14, -122.3363248654052029 ) ) ;
#22032=CARTESIAN_POINT ( 'NONE',  ( 6.000000000000052403, -1.607695154586662678, -102.1533121635129646 ) ) ;
#22033=AXIS2_PLACEMENT_3D ( 'NONE', #5339, #12460, #28835 ) ;
#22034=CARTESIAN_POINT ( 'NONE',  ( 6.350852961086080661, -9.614813431917819062E-14, -177.3750000000000284 ) ) ;
#22036=CARTESIAN_POINT ( 'NONE',  ( -7.216878364870328078, 0.000000000000000000, -150.6919872981077901 ) ) ;
#22039=CARTESIAN_POINT ( 'NONE',  ( 4.763139720814407951, -2.749999999999988454, -84.50000000000001421 ) ) ;
#22040=CARTESIAN_POINT ( 'NONE',  ( 3.608439182435180470, -6.249999999999997335, -94.05801270189226670 ) ) ;
#22041=( BOUNDED_CURVE ( )  B_SPLINE_CURVE ( 2, ( #19508, #14329, #17065, #5345, #28390, #753, #26540, #10140, #26394 ),
 .UNSPECIFIED., .F., .T. ) 
 B_SPLINE_CURVE_WITH_KNOTS ( ( 3, 2, 2, 2, 3 ),
 ( 0.4638888888888889062, 0.4648148148148147918, 0.4666666666666666741, 0.4685185185185185563, 0.4694444444444444420 ),
 .UNSPECIFIED. ) 
 CURVE ( )  GEOMETRIC_REPRESENTATION_ITEM ( )  RATIONAL_B_SPLINE_CURVE ( ( 0.9330127018922194093, 0.9330127018922234061, 1.000000000000000000, 0.8660254037844388186, 1.000000000000000000, 0.8660254037844388186, 1.000000000000000000, 0.9330127018922194093, 0.9330127018922194093 ) ) 
 REPRESENTATION_ITEM ( '' )  );
#22047=ADVANCED_FACE ( 'NONE', ( #16296 ), #25617, .T. ) ;
#22050=CARTESIAN_POINT ( 'NONE',  ( 3.175426480543072749, 5.499999999999865885, -168.1250000000000000 ) ) ;
#22052=CARTESIAN_POINT ( 'NONE',  ( 6.350852961086080661, -9.614813431917819062E-14, -147.3750000000000284 ) ) ;
#22053=CARTESIAN_POINT ( 'NONE',  ( 0.000000000000000000, 0.000000000000000000, 0.000000000000000000 ) ) ;
#22055=CARTESIAN_POINT ( 'NONE',  ( -2.775557561562891351E-14, -5.500000000000115463, -95.25000000000000000 ) ) ;
#22057=DIRECTION ( 'NONE',  ( -7.147005652999508048E-36, 5.642372883946980038E-36, 1.000000000000000000 ) ) ;
#22058=CARTESIAN_POINT ( 'NONE',  ( 3.175426480543072749, -5.500000000000105693, -78.62500000000001421 ) ) ;
#22059=AXIS2_PLACEMENT_3D ( 'NONE', #21383, #25974, #7243 ) ;
#22062=CARTESIAN_POINT ( 'NONE',  ( -3.464101615137725076, 5.999999999999979572, -155.5863248654052029 ) ) ;
#22064=CARTESIAN_POINT ( 'NONE',  ( 5.196152422706629359, 3.000000000000002665, -125.0386751345948255 ) ) ;
#22065=CARTESIAN_POINT ( 'NONE',  ( -5.999999999999963585, 1.780251999655701777E-13, -74.33632486540523132 ) ) ;
#22066=DIRECTION ( 'NONE',  ( 1.000000000000000000, -5.551115123125773458E-17, -1.260129944081490338E-35 ) ) ;
#22070=CARTESIAN_POINT ( 'NONE',  ( -5.196152422706601826, 2.999999999999975131, -82.53867513459483973 ) ) ;
#22072=CARTESIAN_POINT ( 'NONE',  ( -5.999999999999956479, -1.607695154586745057, -116.2693375672974270 ) ) ;
#22074=EDGE_LOOP ( 'NONE', ( #3058, #6620, #21186, #26521 ) ) ;
#22076=CARTESIAN_POINT ( 'NONE',  ( -4.763139720814407951, 2.749999999999946709, -101.7500000000000000 ) ) ;
#22078=CARTESIAN_POINT ( 'NONE',  ( -3.608439182435115633, 6.249999999999965361, -117.3080127018922525 ) ) ;
#22079=ORIENTED_EDGE ( 'NONE', *, *, #26126, .F. ) ;
#22080=CARTESIAN_POINT ( 'NONE',  ( 3.464101615137757051, -5.999999999999979572, -60.91367513459483263 ) ) ;
#22082=CARTESIAN_POINT ( 'NONE',  ( -7.216878364870328078, 0.000000000000000000, -158.1919872981078186 ) ) ;
#22083=LINE ( 'NONE', #5770, #17670 ) ;
#22084=CARTESIAN_POINT ( 'NONE',  ( -3.608439182435115633, 6.249999999999965361, -58.80801270189223118 ) ) ;
#22085=ORIENTED_EDGE ( 'NONE', *, *, #20751, .T. ) ;
#22086=CARTESIAN_POINT ( 'NONE',  ( -5.999999999999963585, 8.134310703387671600E-14, -116.9136751345948539 ) ) ;
#22089=CARTESIAN_POINT ( 'NONE',  ( -5.380303083296078093, 9.596003543682472881, -22.31547897336682951 ) ) ;
#22091=CARTESIAN_POINT ( 'NONE',  ( 6.350852961086080661, -9.614813431917819062E-14, -174.3750000000000284 ) ) ;
#22094=CARTESIAN_POINT ( 'NONE',  ( -7.216878364870328078, 0.000000000000000000, -168.0580127018922383 ) ) ;
#22097=( BOUNDED_CURVE ( )  B_SPLINE_CURVE ( 2, ( #18953, #5073, #4784, #23840, #12202, #28122, #11745, #16657, #12339 ),
 .UNSPECIFIED., .F., .F. ) 
 B_SPLINE_CURVE_WITH_KNOTS ( ( 3, 2, 2, 2, 3 ),
 ( 0.4972222222222222321, 0.4981481481481481177, 0.5000000000000000000, 0.5018518518518517713, 0.5027777777777777679 ),
 .UNSPECIFIED. ) 
 CURVE ( )  GEOMETRIC_REPRESENTATION_ITEM ( )  RATIONAL_B_SPLINE_CURVE ( ( 0.9330127018922194093, 0.9330127018922194093, 1.000000000000000000, 0.8660254037844388186, 1.000000000000000000, 0.8660254037844388186, 1.000000000000000000, 0.9330127018922194093, 0.9330127018922194093 ) ) 
 REPRESENTATION_ITEM ( '' )  );
#22098=CARTESIAN_POINT ( 'NONE',  ( -3.175426480542816066, 5.499999999999865885, -118.3750000000000284 ) ) ;
#22100=CARTESIAN_POINT ( 'NONE',  ( -3.175426480542816510, -5.500000000000057732, -105.8750000000000284 ) ) ;
#22103=CARTESIAN_POINT ( 'NONE',  ( 6.000000000000000888, 1.607695154586715303, -118.5193375672974412 ) ) ;
#22104=VERTEX_POINT ( 'NONE', #712 ) ;
#22107=VECTOR ( 'NONE', #9015, 1000.000000000000000 ) ;
#22108=CARTESIAN_POINT ( 'NONE',  ( -3.464101615137757051, -5.999999999999979572, -76.16367513459483973 ) ) ;
#22110=CARTESIAN_POINT ( 'NONE',  ( -5.412658773652739619, 3.124999999999975131, -80.31698729810781856 ) ) ;
#22111=CARTESIAN_POINT ( 'NONE',  ( 5.999999999999949374, -1.607695154586841868, -129.1533121635129930 ) ) ;
#22112=ORIENTED_EDGE ( 'NONE', *, *, #26330, .T. ) ;
#22113=CARTESIAN_POINT ( 'NONE',  ( -5.999999999999963585, 1.780251999655701777E-13, -61.41367513459483973 ) ) ;
#22117=EDGE_CURVE ( 'NONE', #16860, #15423, #15802, .T. ) ;
#22120=CARTESIAN_POINT ( 'NONE',  ( 5.412658773652739619, 3.124999999999988898, -134.8169872981078186 ) ) ;
#22121=CARTESIAN_POINT ( 'NONE',  ( 6.000000000000000888, 1.607695154586715303, -131.0966878364870922 ) ) ;
#22123=VECTOR ( 'NONE', #7818, 1000.000000000000000 ) ;
#22124=ORIENTED_EDGE ( 'NONE', *, *, #13988, .F. ) ;
#22132=CARTESIAN_POINT ( 'NONE',  ( 3.608439182435180470, 6.249999999999982236, -68.69198729810780435 ) ) ;
#22133=CARTESIAN_POINT ( 'NONE',  ( -3.608439182435115633, 6.249999999999965361, -54.94198729810780435 ) ) ;
#22135=CARTESIAN_POINT ( 'NONE',  ( 5.999999999999949374, 1.607695154586804565, -75.01933756729745539 ) ) ;
#22137=CARTESIAN_POINT ( 'NONE',  ( 3.175426480543072749, -5.500000000000105693, -128.1249999999999716 ) ) ;
#22139=CARTESIAN_POINT ( 'NONE',  ( 5.999999999999988454, 1.607695154586737729, -158.0966878364870922 ) ) ;
#22140=DIRECTION ( 'NONE',  ( -7.147005652999508048E-36, 5.642372883946980038E-36, 1.000000000000000000 ) ) ;
#22141=CARTESIAN_POINT ( 'NONE',  ( 5.196152422706629359, -2.999999999999988898, -159.7886751345948255 ) ) ;
#22147=CARTESIAN_POINT ( 'NONE',  ( -5.412658773652739619, 3.124999999999975131, -96.81698729810783277 ) ) ;
#22157=CIRCLE ( 'NONE', #3493, 11.00000000000001599 ) ;
#22159=CARTESIAN_POINT ( 'NONE',  ( 4.763139720814407951, 2.750000000000002665, -48.25000000000001421 ) ) ;
#22161=CARTESIAN_POINT ( 'NONE',  ( 5.196152422706629359, -2.999999999999988898, -134.2886751345947971 ) ) ;
#22162=CARTESIAN_POINT ( 'NONE',  ( 2.775557561562891351E-14, -6.250000000000061284, -76.18301270189226670 ) ) ;
#22163=CARTESIAN_POINT ( 'NONE',  ( -5.999999999999904965, -1.607695154586834541, -173.2693375672974412 ) ) ;
#22165=AXIS2_PLACEMENT_3D ( 'NONE', #993, #17021, #21914 ) ;
#22166=CARTESIAN_POINT ( 'NONE',  ( -5.999999999999962697, 3.323446944526963260E-14, -149.3363248654052313 ) ) ;
#22167=DIRECTION ( 'NONE',  ( -7.147005652999508048E-36, 5.642372883946980038E-36, 1.000000000000000000 ) ) ;
#22168=CARTESIAN_POINT ( 'NONE',  ( -5.999999999999963585, 1.780251999655701777E-13, -47.91367513459483973 ) ) ;
#22170=CARTESIAN_POINT ( 'NONE',  ( -6.350852961085760029, -1.281975124255709124E-13, -128.6250000000000000 ) ) ;
#22171=CARTESIAN_POINT ( 'NONE',  ( 5.196152422706629359, 3.000000000000002665, -68.96132486540523132 ) ) ;
#22173=CARTESIAN_POINT ( 'NONE',  ( 6.000000000000000888, 1.607695154586715303, -67.51933756729745539 ) ) ;
#22174=CARTESIAN_POINT ( 'NONE',  ( 3.175426480543072749, -5.500000000000105693, -60.62500000000000000 ) ) ;
#22175=CARTESIAN_POINT ( 'NONE',  ( -4.763139720814407951, -2.750000000000016431, -55.00000000000004974 ) ) ;
#22181=ADVANCED_FACE ( 'NONE', ( #26494 ), #21476, .T. ) ;
#22188=CARTESIAN_POINT ( 'NONE',  ( -2.775557561562891351E-14, -5.500000000000115463, -144.7500000000000568 ) ) ;
#22189=EDGE_CURVE ( 'NONE', #9271, #13246, #2039, .T. ) ;
#22190=CARTESIAN_POINT ( 'NONE',  ( 3.608439182435180470, 6.249999999999982236, -50.69198729810784698 ) ) ;
#22193=CARTESIAN_POINT ( 'NONE',  ( -3.608439182435115633, 6.249999999999965361, -147.9419872981078470 ) ) ;
#22194=CARTESIAN_POINT ( 'NONE',  ( -3.175426480542816510, -5.500000000000057732, -80.37500000000002842 ) ) ;
#22196=VERTEX_POINT ( 'NONE', #18883 ) ;
#22197=CARTESIAN_POINT ( 'NONE',  ( -5.999999999999964473, 9.063946212346262433E-15, -175.4136751345948824 ) ) ;
#22202=CARTESIAN_POINT ( 'NONE',  ( -2.775557561562891351E-14, -5.500000000000115463, -159.7500000000000568 ) ) ;
#22203=LINE ( 'NONE', #29708, #23665 ) ;
#22204=CARTESIAN_POINT ( 'NONE',  ( -3.175426480542816510, -5.500000000000057732, -143.3750000000000000 ) ) ;
#22207=CARTESIAN_POINT ( 'NONE',  ( 3.175426480543072749, 5.499999999999865885, -94.62500000000002842 ) ) ;
#22209=DIRECTION ( 'NONE',  ( -7.147005652999508048E-36, 5.642372883946980038E-36, 1.000000000000000000 ) ) ;
#22210=CARTESIAN_POINT ( 'NONE',  ( -6.350852961085760029, -1.281975124255709124E-13, -79.12500000000001421 ) ) ;
#22212=CARTESIAN_POINT ( 'NONE',  ( 6.000000000000000888, -1.859271017917181981E-14, -114.6636751345948255 ) ) ;
#22213=DIRECTION ( 'NONE',  ( 1.000000000000000000, -5.551115123125774074E-17, 0.000000000000000000 ) ) ;
#22215=CARTESIAN_POINT ( 'NONE',  ( 0.000000000000000000, 0.000000000000000000, 0.000000000000000000 ) ) ;
#22216=DIRECTION ( 'NONE',  ( 1.000000000000000000, -5.551115123125773458E-17, -1.260129944081490338E-35 ) ) ;
#22220=CARTESIAN_POINT ( 'NONE',  ( 6.000000000000000888, 1.743066579297358182E-13, -73.58632486540520290 ) ) ;
#22221=CARTESIAN_POINT ( 'NONE',  ( -5.999999999999963585, 8.134310703387671600E-14, -131.3363248654052313 ) ) ;
#22223=VERTEX_POINT ( 'NONE', #25914 ) ;
#22225=( BOUNDED_CURVE ( )  B_SPLINE_CURVE ( 2, ( #15880, #6910, #21060, #16332, #25178, #25652, #22903, #13722, #1847 ),
 .UNSPECIFIED., .F., .T. ) 
 B_SPLINE_CURVE_WITH_KNOTS ( ( 3, 2, 2, 2, 3 ),
 ( 0.5638888888888888840, 0.5648148148148148806, 0.5666666666666666519, 0.5685185185185185341, 0.5694444444444444198 ),
 .UNSPECIFIED. ) 
 CURVE ( )  GEOMETRIC_REPRESENTATION_ITEM ( )  RATIONAL_B_SPLINE_CURVE ( ( 0.9330127018922194093, 0.9330127018922194093, 1.000000000000000000, 0.8660254037844388186, 1.000000000000000000, 0.8660254037844388186, 1.000000000000000000, 0.9330127018922234061, 0.9330127018922194093 ) ) 
 REPRESENTATION_ITEM ( '' )  );
#22226=CARTESIAN_POINT ( 'NONE',  ( -3.175426480542816510, 5.499999999999865885, -107.8750000000000284 ) ) ;
#22228=CARTESIAN_POINT ( 'NONE',  ( -5.412658773652684552, -3.125000000000099920, -118.4330127018922099 ) ) ;
#22230=ORIENTED_EDGE ( 'NONE', *, *, #11577, .F. ) ;
#22231=FACE_OUTER_BOUND ( 'NONE', #1397, .T. ) ;
#22233=DIRECTION ( 'NONE',  ( -7.147005652999508048E-36, 5.642372883946980038E-36, 1.000000000000000000 ) ) ;
#22234=CARTESIAN_POINT ( 'NONE',  ( -3.608439182435052128, -6.250000000000110134, -50.80801270189224539 ) ) ;
#22236=CARTESIAN_POINT ( 'NONE',  ( -5.999999999999963585, -1.487416814333745711E-14, -167.3363248654052029 ) ) ;
#22240=CARTESIAN_POINT ( 'NONE',  ( 4.000000000000004441, -2.220446049250312095E-16, -5.040519776325966696E-35 ) ) ;
#22241=CARTESIAN_POINT ( 'NONE',  ( 3.175426480543072749, -5.500000000000105693, -167.1250000000000000 ) ) ;
#22243=CARTESIAN_POINT ( 'NONE',  ( -5.999999999999962697, 3.323446944526963260E-14, -158.3363248654052313 ) ) ;
#22244=CARTESIAN_POINT ( 'NONE',  ( 2.775557561562891351E-14, -6.250000000000061284, -169.1830127018922383 ) ) ;
#22245=CARTESIAN_POINT ( 'NONE',  ( -5.999999999999963585, 1.780251999655701777E-13, -47.91367513459483973 ) ) ;
#22246=CARTESIAN_POINT ( 'NONE',  ( 4.763139720814407951, -2.749999999999988454, -115.9999999999999858 ) ) ;
#22248=CARTESIAN_POINT ( 'NONE',  ( -3.175426480542816510, 5.499999999999865885, -104.8750000000000142 ) ) ;
#22252=ORIENTED_EDGE ( 'NONE', *, *, #2849, .T. ) ;
#22258=CARTESIAN_POINT ( 'NONE',  ( -4.763139720814407951, 2.749999999999946709, -158.7500000000000568 ) ) ;
#22261=CARTESIAN_POINT ( 'NONE',  ( 2.775557561562891351E-14, 6.250000000000033751, -82.06698729810779014 ) ) ;
#22262=ORIENTED_EDGE ( 'NONE', *, *, #2860, .F. ) ;
#22263=ADVANCED_FACE ( 'NONE', ( #8212 ), #12725, .T. ) ;
#22264=FACE_OUTER_BOUND ( 'NONE', #19223, .T. ) ;
#22269=CARTESIAN_POINT ( 'NONE',  ( 2.775557561562891351E-14, -6.250000000000061284, -136.1830127018922667 ) ) ;
#22271=CARTESIAN_POINT ( 'NONE',  ( -3.608439182435115633, 6.249999999999965361, -123.9419872981078043 ) ) ;
#22272=CARTESIAN_POINT ( 'NONE',  ( 3.175426480543072749, -5.500000000000105693, -170.1250000000000000 ) ) ;
#22273=CARTESIAN_POINT ( 'NONE',  ( 6.000000000000000888, -1.859271017917181981E-14, -167.1636751345948539 ) ) ;
#22275=ORIENTED_EDGE ( 'NONE', *, *, #24287, .F. ) ;
#22277=CARTESIAN_POINT ( 'NONE',  ( -5.999999999999971578, 1.607695154586715303, -134.9806624327026157 ) ) ;
#22278=CARTESIAN_POINT ( 'NONE',  ( 5.196152422706629359, 3.000000000000002665, -164.0386751345947971 ) ) ;
#22280=CARTESIAN_POINT ( 'NONE',  ( -3.464101615137725076, 5.999999999999979572, -90.16367513459483973 ) ) ;
#22282=CARTESIAN_POINT ( 'NONE',  ( 0.000000000000000000, 5.999999999999977796, -46.21132486540524553 ) ) ;
#22283=CARTESIAN_POINT ( 'NONE',  ( 2.775557561562891351E-14, -6.250000000000061284, -67.81698729810781856 ) ) ;
#22284=CARTESIAN_POINT ( 'NONE',  ( -3.608439182435115633, 6.249999999999965361, -56.44198729810781145 ) ) ;
#22285=DIRECTION ( 'NONE',  ( 1.000000000000000000, -5.551115123125773458E-17, -1.260129944081490338E-35 ) ) ;
#22288=CYLINDRICAL_SURFACE ( 'NONE', #3924, 6.000000000000000888 ) ;
#22289=CARTESIAN_POINT ( 'NONE',  ( 0.000000000000000000, 5.499999999999991118, -127.5000000000000568 ) ) ;
#22290=CARTESIAN_POINT ( 'NONE',  ( -5.999999999999963585, 1.780251999655701777E-13, -91.41367513459486815 ) ) ;
#22296=EDGE_CURVE ( 'NONE', #8435, #20245, #14616, .T. ) ;
#22297=VERTEX_POINT ( 'NONE', #10548 ) ;
#22299=CARTESIAN_POINT ( 'NONE',  ( 0.000000000000000000, 0.000000000000000000, 0.000000000000000000 ) ) ;
#22300=CARTESIAN_POINT ( 'NONE',  ( 2.775557561562891351E-14, -6.250000000000061284, -94.81698729810783277 ) ) ;
#22301=CARTESIAN_POINT ( 'NONE',  ( 3.464101615137757051, -5.999999999999979572, -173.4136751345948255 ) ) ;
#22304=CARTESIAN_POINT ( 'NONE',  ( -5.999999999999919176, 1.607695154586804565, -77.40331216351302146 ) ) ;
#22306=ORIENTED_EDGE ( 'NONE', *, *, #17953, .F. ) ;
#22309=CARTESIAN_POINT ( 'NONE',  ( -2.775557561562891351E-14, -5.500000000000115463, -47.25000000000001421 ) ) ;
#22310=CARTESIAN_POINT ( 'NONE',  ( 3.464101615137757051, -5.999999999999979572, -59.41367513459481842 ) ) ;
#22311=CARTESIAN_POINT ( 'NONE',  ( -5.196152422706573404, -3.000000000000002665, -80.21132486540521711 ) ) ;
#22312=CARTESIAN_POINT ( 'NONE',  ( 3.608439182435180470, 6.249999999999982236, -77.05801270189225249 ) ) ;
#22314=DIRECTION ( 'NONE',  ( -7.147005652999508048E-36, 5.642372883946980038E-36, 1.000000000000000000 ) ) ;
#22318=LINE ( 'NONE', #16976, #14344 ) ;
#22320=CARTESIAN_POINT ( 'NONE',  ( -3.175426480542816066, -5.500000000000057732, -132.8750000000000284 ) ) ;
#22321=CARTESIAN_POINT ( 'NONE',  ( 0.000000000000000000, -5.999999999999991118, -177.4613248654052313 ) ) ;
#22322=CARTESIAN_POINT ( 'NONE',  ( 3.608439182435180470, -6.249999999999997335, -149.5580127018922951 ) ) ;
#22325=CARTESIAN_POINT ( 'NONE',  ( 4.763139720814407951, -2.749999999999988454, -66.50000000000000000 ) ) ;
#22326=CYLINDRICAL_SURFACE ( 'NONE', #14901, 6.000000000000000888 ) ;
#22327=CARTESIAN_POINT ( 'NONE',  ( 3.175426480543072749, -5.500000000000105693, -59.12499999999999289 ) ) ;
#22328=EDGE_CURVE ( 'NONE', #15344, #26402, #28296, .T. ) ;
#22329=CARTESIAN_POINT ( 'NONE',  ( -5.196152422706601826, 2.999999999999975131, -170.4613248654052313 ) ) ;
#22330=ORIENTED_EDGE ( 'NONE', *, *, #4387, .F. ) ;
#22334=CARTESIAN_POINT ( 'NONE',  ( -5.999999999999964473, 9.063946212346262433E-15, -175.4136751345948824 ) ) ;
#22338=CARTESIAN_POINT ( 'NONE',  ( -6.000000000000000888, 1.067854986875958443E-15, 7.560779664488942560E-35 ) ) ;
#22341=CARTESIAN_POINT ( 'NONE',  ( 3.175426480543072749, 5.499999999999865885, -148.6250000000000284 ) ) ;
#22342=CARTESIAN_POINT ( 'NONE',  ( -5.412658773652684552, -3.125000000000099920, -48.56698729810781856 ) ) ;
#22344=ORIENTED_EDGE ( 'NONE', *, *, #29597, .T. ) ;
#22345=CARTESIAN_POINT ( 'NONE',  ( 7.216878364870455975, -6.409875621278545621E-14, -146.9419872981078470 ) ) ;
#22346=CARTESIAN_POINT ( 'NONE',  ( 3.175426480543072749, 5.499999999999865885, -75.12500000000001421 ) ) ;
#22348=CARTESIAN_POINT ( 'NONE',  ( 2.775557561562891351E-14, -6.250000000000061284, -92.68301270189222407 ) ) ;
#22349=ORIENTED_EDGE ( 'NONE', *, *, #24634, .F. ) ;
#22352=CYLINDRICAL_SURFACE ( 'NONE', #4770, 6.000000000000000888 ) ;
#22353=CYLINDRICAL_SURFACE ( 'NONE', #472, 6.000000000000000888 ) ;
#22354=CARTESIAN_POINT ( 'NONE',  ( -4.763139720814407951, -2.750000000000016431, -152.5000000000000284 ) ) ;
#22355=CARTESIAN_POINT ( 'NONE',  ( 0.000000000000000000, 0.000000000000000000, 0.000000000000000000 ) ) ;
#22356=CARTESIAN_POINT ( 'NONE',  ( 4.763139720814407951, -2.749999999999988454, -149.0000000000000284 ) ) ;
#22357=CARTESIAN_POINT ( 'NONE',  ( -2.308094007022951200, 5.188356418780102786, -180.0000000000000568 ) ) ;
#22360=CARTESIAN_POINT ( 'NONE',  ( 3.175426480543072749, -5.500000000000105693, -83.12500000000004263 ) ) ;
#22361=DIRECTION ( 'NONE',  ( -7.147005652999508048E-36, 5.642372883946980038E-36, 1.000000000000000000 ) ) ;
#22362=CARTESIAN_POINT ( 'NONE',  ( -4.763139720814407951, 2.749999999999946709, -83.74999999999998579 ) ) ;
#22363=EDGE_CURVE ( 'NONE', #29150, #651, #5149, .T. ) ;
#22364=LINE ( 'NONE', #15481, #27053 ) ;
#22366=CARTESIAN_POINT ( 'NONE',  ( 6.000000000000000888, -3.330669073875464691E-16, -7.560779664488942560E-35 ) ) ;
#22367=DIRECTION ( 'NONE',  ( 1.000000000000000000, -5.551115123125773458E-17, -1.260129944081490338E-35 ) ) ;
#22371=LINE ( 'NONE', #29409, #5166 ) ;
#22373=CARTESIAN_POINT ( 'NONE',  ( -3.464101615137725076, 5.999999999999979572, -73.08632486540520290 ) ) ;
#22374=CARTESIAN_POINT ( 'NONE',  ( -5.999999999999963585, 1.780251999655701777E-13, -79.41367513459482552 ) ) ;
#22377=EDGE_LOOP ( 'NONE', ( #20021, #27753, #26412, #5341 ) ) ;
#22379=CARTESIAN_POINT ( 'NONE',  ( 3.175426480543072749, -5.500000000000105693, -98.12500000000004263 ) ) ;
#22381=CARTESIAN_POINT ( 'NONE',  ( 5.412658773652712085, -3.125000000000086153, -113.4330127018922099 ) ) ;
#22382=VERTEX_POINT ( 'NONE', #15334 ) ;
#22383=CARTESIAN_POINT ( 'NONE',  ( 0.000000000000000000, 5.999999999999977796, -94.21132486540523132 ) ) ;
#22384=CARTESIAN_POINT ( 'NONE',  ( -5.999999999999963585, 1.780251999655701777E-13, -49.41367513459484684 ) ) ;
#22387=EDGE_CURVE ( 'NONE', #24608, #15772, #2998, .T. ) ;
#22388=CARTESIAN_POINT ( 'NONE',  ( -5.412658773652684552, -3.125000000000099920, -49.43301270189226670 ) ) ;
#22389=ORIENTED_EDGE ( 'NONE', *, *, #907, .T. ) ;
#22391=CARTESIAN_POINT ( 'NONE',  ( -6.000000000000000888, 1.067854986875958443E-15, 7.560779664488942560E-35 ) ) ;
#22392=DIRECTION ( 'NONE',  ( -7.147005652999508048E-36, 5.642372883946980038E-36, 1.000000000000000000 ) ) ;
#22393=CARTESIAN_POINT ( 'NONE',  ( 3.175426480543072749, 5.499999999999865885, -172.6250000000000000 ) ) ;
#22396=CARTESIAN_POINT ( 'NONE',  ( -3.608439182435115633, 6.249999999999965361, -169.8080127018922383 ) ) ;
#22398=CARTESIAN_POINT ( 'NONE',  ( 0.000000000000000000, 5.499999999999991118, -107.9999999999999858 ) ) ;
#22399=DIRECTION ( 'NONE',  ( 1.000000000000000000, -5.551115123125773458E-17, -1.260129944081490338E-35 ) ) ;
#22401=( BOUNDED_CURVE ( )  B_SPLINE_CURVE ( 2, ( #7869, #21727, #23870, #10204, #5262, #17582, #19427, #24451, #17428 ),
 .UNSPECIFIED., .F., .T. ) 
 B_SPLINE_CURVE_WITH_KNOTS ( ( 3, 2, 2, 2, 3 ),
 ( 0.1805555555555554692, 0.1814814814814814659, 0.1833333333333333481, 0.1851851851851852304, 0.1861111111111111160 ),
 .UNSPECIFIED. ) 
 CURVE ( )  GEOMETRIC_REPRESENTATION_ITEM ( )  RATIONAL_B_SPLINE_CURVE ( ( 0.9330127018922194093, 0.9330127018922154125, 1.000000000000000000, 0.8660254037844388186, 1.000000000000000000, 0.8660254037844388186, 1.000000000000000000, 0.9330127018922194093, 0.9330127018922194093 ) ) 
 REPRESENTATION_ITEM ( '' )  );
#22402=CARTESIAN_POINT ( 'NONE',  ( -6.350852961085760029, -1.281975124255709124E-13, -101.6250000000000000 ) ) ;
#22404=DIRECTION ( 'NONE',  ( 1.000000000000000000, -5.551115123125773458E-17, -1.260129944081490338E-35 ) ) ;
#22405=CARTESIAN_POINT ( 'NONE',  ( -5.196152422706573404, -3.000000000000002665, -112.2886751345948397 ) ) ;
#22408=CARTESIAN_POINT ( 'NONE',  ( -3.464101615137757051, -5.999999999999979572, -90.58632486540521711 ) ) ;
#22410=CARTESIAN_POINT ( 'NONE',  ( 6.000000000000000888, -1.859271017917181981E-14, -80.16367513459481131 ) ) ;
#22413=CARTESIAN_POINT ( 'NONE',  ( -3.175426480542816510, -5.500000000000057732, -158.3750000000000284 ) ) ;
#22415=CARTESIAN_POINT ( 'NONE',  ( -3.608439182435052128, -6.250000000000110134, -79.94198729810779014 ) ) ;
#22416=VERTEX_POINT ( 'NONE', #15799 ) ;
#22419=VERTEX_POINT ( 'NONE', #27706 ) ;
#22421=CARTESIAN_POINT ( 'NONE',  ( -4.763139720814407951, 2.749999999999946709, -119.7500000000000284 ) ) ;
#22422=CARTESIAN_POINT ( 'NONE',  ( 2.775557561562891351E-14, 6.250000000000033751, -141.4330127018922383 ) ) ;
#22423=ORIENTED_EDGE ( 'NONE', *, *, #6007, .F. ) ;
#22425=CARTESIAN_POINT ( 'NONE',  ( 3.608439182435180470, 6.249999999999982236, -125.6919872981078186 ) ) ;
#22427=AXIS2_PLACEMENT_3D ( 'NONE', #22532, #17477, #15649 ) ;
#22428=CARTESIAN_POINT ( 'NONE',  ( 4.763139720814407951, 2.750000000000002665, -172.7500000000000284 ) ) ;
#22431=EDGE_CURVE ( 'NONE', #28690, #3077, #14790, .T. ) ;
#22432=ORIENTED_EDGE ( 'NONE', *, *, #28854, .T. ) ;
#22435=CARTESIAN_POINT ( 'NONE',  ( 0.000000000000000000, -5.999999999999991118, -117.4613248654052313 ) ) ;
#22436=CARTESIAN_POINT ( 'NONE',  ( 5.196152422706629359, 3.000000000000002665, -92.96132486540520290 ) ) ;
#22439=CARTESIAN_POINT ( 'NONE',  ( 3.608439182435180470, -6.249999999999997335, -67.69198729810779014 ) ) ;
#22440=CARTESIAN_POINT ( 'NONE',  ( -7.216878364870328078, 0.000000000000000000, -53.19198729810779724 ) ) ;
#22442=CYLINDRICAL_SURFACE ( 'NONE', #2205, 6.000000000000000888 ) ;
#22444=CARTESIAN_POINT ( 'NONE',  ( 0.000000000000000000, 5.999999999999977796, -74.71132486540521711 ) ) ;
#22446=CARTESIAN_POINT ( 'NONE',  ( -4.763139720814407951, 2.749999999999946709, -130.2500000000000284 ) ) ;
#22448=CARTESIAN_POINT ( 'NONE',  ( 5.196152422706629359, 3.000000000000002665, -138.5386751345948255 ) ) ;
#22453=CARTESIAN_POINT ( 'NONE',  ( -5.196152422706601826, 2.999999999999975131, -129.9613248654052313 ) ) ;
#22457=CARTESIAN_POINT ( 'NONE',  ( 6.000000000000000888, 1.607695154586715303, -72.01933756729744118 ) ) ;
#22458=CARTESIAN_POINT ( 'NONE',  ( -3.608439182435052128, -6.250000000000110134, -114.4419872981078186 ) ) ;
#22459=CARTESIAN_POINT ( 'NONE',  ( 5.196152422706629359, -2.999999999999988898, -173.2886751345948255 ) ) ;
#22461=ORIENTED_EDGE ( 'NONE', *, *, #27420, .T. ) ;
#22462=FACE_OUTER_BOUND ( 'NONE', #15067, .T. ) ;
#22464=CARTESIAN_POINT ( 'NONE',  ( -5.999999999999963585, -1.487416814333745711E-14, -138.8363248654052597 ) ) ;
#22465=CARTESIAN_POINT ( 'NONE',  ( -4.763139720814407951, 2.749999999999946709, -47.75000000000001421 ) ) ;
#22466=EDGE_CURVE ( 'NONE', #11750, #25219, #17753, .T. ) ;
#22467=CARTESIAN_POINT ( 'NONE',  ( 5.196152422706629359, 3.000000000000002665, -69.53867513459482552 ) ) ;
#22468=CARTESIAN_POINT ( 'NONE',  ( 6.000000000000000888, 7.762456499804234384E-14, -134.1636751345948539 ) ) ;
#22469=CARTESIAN_POINT ( 'NONE',  ( -3.464101615137757051, -5.999999999999979572, -80.08632486540513185 ) ) ;
#22470=CARTESIAN_POINT ( 'NONE',  ( 5.412658773652712085, -3.125000000000086153, -78.93301270189223828 ) ) ;
#22473=FACE_OUTER_BOUND ( 'NONE', #30143, .T. ) ;
#22477=DIRECTION ( 'NONE',  ( -7.147005652999508048E-36, 5.642372883946980038E-36, 1.000000000000000000 ) ) ;
#22478=CARTESIAN_POINT ( 'NONE',  ( 6.000000000000000888, -1.859271017917181981E-14, -105.0863248654052313 ) ) ;
#22480=CARTESIAN_POINT ( 'NONE',  ( 0.000000000000000000, 5.499999999999991118, -129.0000000000000000 ) ) ;
#22481=CARTESIAN_POINT ( 'NONE',  ( 2.000000000000003109, -1.110223024625156540E-16, -200.0000000000000000 ) ) ;
#22482=CARTESIAN_POINT ( 'NONE',  ( 2.775557561562891351E-14, -6.250000000000061284, -149.6830127018922099 ) ) ;
#22483=DIRECTION ( 'NONE',  ( 1.000000000000000000, -5.551115123125773458E-17, -1.260129944081490338E-35 ) ) ;
#22487=CARTESIAN_POINT ( 'NONE',  ( -2.775557561562891351E-14, -5.500000000000115463, -63.75000000000002842 ) ) ;
#22489=CARTESIAN_POINT ( 'NONE',  ( -6.000000000000023093, 1.607695154586625819, -170.4033121635129930 ) ) ;
#22493=CARTESIAN_POINT ( 'NONE',  ( 6.000000000000000888, 7.762456499804234384E-14, -117.6636751345948255 ) ) ;
#22495=CARTESIAN_POINT ( 'NONE',  ( -6.000000000000000888, 1.067854986875958443E-15, 7.560779664488942560E-35 ) ) ;
#22499=EDGE_LOOP ( 'NONE', ( #14908, #6502, #12462, #12070 ) ) ;
#22500=CARTESIAN_POINT ( 'NONE',  ( 0.000000000000000000, 5.499999999999991118, -142.5000000000000284 ) ) ;
#22503=CARTESIAN_POINT ( 'NONE',  ( -5.412658773652739619, 3.124999999999975131, -48.81698729810779724 ) ) ;
#22505=ORIENTED_EDGE ( 'NONE', *, *, #11654, .F. ) ;
#22506=CARTESIAN_POINT ( 'NONE',  ( 0.000000000000000000, 5.499999999999991118, -76.50000000000001421 ) ) ;
#22509=CARTESIAN_POINT ( 'NONE',  ( -5.412658773652684552, -3.125000000000099920, -97.43301270189225249 ) ) ;
#22512=CARTESIAN_POINT ( 'NONE',  ( -3.682280293032447194, -10.37087330740123825, -29.75307074678473640 ) ) ;
#22513=CARTESIAN_POINT ( 'NONE',  ( 6.000000000000052403, -1.607695154586662678, -83.23066243270257303 ) ) ;
#22515=CARTESIAN_POINT ( 'NONE',  ( -3.464101615137757051, -5.999999999999979572, -86.66367513459481131 ) ) ;
#22516=DIRECTION ( 'NONE',  ( -7.147005652999508048E-36, 5.642372883946980038E-36, 1.000000000000000000 ) ) ;
#22518=CARTESIAN_POINT ( 'NONE',  ( 4.763139720814407951, -2.749999999999988454, -159.5000000000000284 ) ) ;
#22520=FACE_OUTER_BOUND ( 'NONE', #20844, .T. ) ;
#22521=CARTESIAN_POINT ( 'NONE',  ( -6.350852961085760029, -1.281975124255709124E-13, -88.12500000000000000 ) ) ;
#22522=DIRECTION ( 'NONE',  ( -7.147005652999508048E-36, 5.642372883946980038E-36, 1.000000000000000000 ) ) ;
#22524=CARTESIAN_POINT ( 'NONE',  ( -2.775557561562891351E-14, -5.500000000000115463, -83.25000000000004263 ) ) ;
#22527=CARTESIAN_POINT ( 'NONE',  ( -5.999999999999968026, -1.607695154586722186, -149.8466878364870354 ) ) ;
#22528=DIRECTION ( 'NONE',  ( 1.000000000000000000, -5.551115123125773458E-17, -1.260129944081490338E-35 ) ) ;
#22530=CARTESIAN_POINT ( 'NONE',  ( -3.464101615137725076, 5.999999999999979572, -75.16367513459483973 ) ) ;
#22532=CARTESIAN_POINT ( 'NONE',  ( 0.000000000000000000, 0.000000000000000000, 0.000000000000000000 ) ) ;
#22533=CARTESIAN_POINT ( 'NONE',  ( -5.999999999999956479, -1.607695154586745057, -172.3466878364870922 ) ) ;
#22535=VERTEX_POINT ( 'NONE', #25730 ) ;
#22536=VERTEX_POINT ( 'NONE', #18997 ) ;
#22537=CARTESIAN_POINT ( 'NONE',  ( -2.775557561562891351E-14, -5.500000000000115463, -98.25000000000000000 ) ) ;
#22538=CARTESIAN_POINT ( 'NONE',  ( -5.999999999999919176, 1.607695154586804565, -70.48066243270261566 ) ) ;
#22539=EDGE_CURVE ( 'NONE', #10886, #26998, #7141, .T. ) ;
#22540=CARTESIAN_POINT ( 'NONE',  ( -5.412658773652739619, 3.124999999999975131, -117.1830127018922383 ) ) ;
#22544=CARTESIAN_POINT ( 'NONE',  ( 6.000000000000000888, -3.330669073875464691E-16, -7.560779664488942560E-35 ) ) ;
#22545=CARTESIAN_POINT ( 'NONE',  ( -5.412658773652739619, 3.124999999999975131, -51.18301270189223828 ) ) ;
#22546=VECTOR ( 'NONE', #26296, 1000.000000000000000 ) ;
#22548=CARTESIAN_POINT ( 'NONE',  ( -3.464101615137725076, 5.999999999999979572, -160.0863248654052313 ) ) ;
#22553=CARTESIAN_POINT ( 'NONE',  ( -3.175426480542816510, -5.500000000000057732, -171.8750000000000284 ) ) ;
#22557=CARTESIAN_POINT ( 'NONE',  ( 3.175426480543072749, 5.499999999999865885, -111.1249999999999858 ) ) ;
#22558=CARTESIAN_POINT ( 'NONE',  ( -6.000000000000000888, 1.067854986875958443E-15, 7.560779664488942560E-35 ) ) ;
#22559=CARTESIAN_POINT ( 'NONE',  ( -3.175426480542816510, -5.500000000000057732, -107.3750000000000284 ) ) ;
#22563=EDGE_LOOP ( 'NONE', ( #24693, #17381, #20476, #13508 ) ) ;
#22567=ORIENTED_EDGE ( 'NONE', *, *, #22789, .T. ) ;
#22568=CARTESIAN_POINT ( 'NONE',  ( 0.000000000000000000, 5.499999999999991118, -159.0000000000000284 ) ) ;
#22571=CARTESIAN_POINT ( 'NONE',  ( 3.608439182435180470, -6.249999999999997335, -81.19198729810786119 ) ) ;
#22572=VECTOR ( 'NONE', #21536, 1000.000000000000000 ) ;
#22575=CARTESIAN_POINT ( 'NONE',  ( -3.464101615137757051, -5.999999999999979572, -75.58632486540521711 ) ) ;
#22577=ORIENTED_EDGE ( 'NONE', *, *, #13022, .F. ) ;
#22578=ORIENTED_EDGE ( 'NONE', *, *, #9223, .F. ) ;
#22580=CARTESIAN_POINT ( 'NONE',  ( -4.763139720814407951, 2.749999999999946709, -121.2500000000000284 ) ) ;
#22581=EDGE_CURVE ( 'NONE', #8028, #4636, #4782, .T. ) ;
#22582=CARTESIAN_POINT ( 'NONE',  ( -7.216878364870328078, 0.000000000000000000, -136.5580127018922099 ) ) ;
#22583=CARTESIAN_POINT ( 'NONE',  ( 3.464101615137852974, 5.999999999999884537, -57.41367513459481842 ) ) ;
#22584=CARTESIAN_POINT ( 'NONE',  ( 2.775557561562891351E-14, 6.250000000000033751, -127.0669872981078328 ) ) ;
#22585=CARTESIAN_POINT ( 'NONE',  ( -3.608439182435115633, 6.249999999999965361, -177.9419872981078186 ) ) ;
#22586=CARTESIAN_POINT ( 'NONE',  ( 3.175426480543072749, 5.499999999999865885, -174.1250000000000284 ) ) ;
#22588=EDGE_LOOP ( 'NONE', ( #29551, #23775, #5493, #16155 ) ) ;
#22590=( BOUNDED_CURVE ( )  B_SPLINE_CURVE ( 2, ( #13518, #21016, #22856, #18570, #6865, #15977, #2270, #28047, #11674 ),
 .UNSPECIFIED., .F., .T. ) 
 B_SPLINE_CURVE_WITH_KNOTS ( ( 3, 2, 2, 2, 3 ),
 ( 0.6972222222222222987, 0.6981481481481481843, 0.6999999999999999556, 0.7018518518518518379, 0.7027777777777777235 ),
 .UNSPECIFIED. ) 
 CURVE ( )  GEOMETRIC_REPRESENTATION_ITEM ( )  RATIONAL_B_SPLINE_CURVE ( ( 0.9330127018922194093, 0.9330127018922234061, 1.000000000000000000, 0.8660254037844388186, 1.000000000000000000, 0.8660254037844388186, 1.000000000000000000, 0.9330127018922234061, 0.9330127018922194093 ) ) 
 REPRESENTATION_ITEM ( '' )  );
#22592=CARTESIAN_POINT ( 'NONE',  ( 6.000000000000000888, 1.607695154586715303, -171.5966878364870638 ) ) ;
#22593=CARTESIAN_POINT ( 'NONE',  ( 5.196152422706629359, -2.999999999999988898, -46.71132486540518869 ) ) ;
#22595=CARTESIAN_POINT ( 'NONE',  ( -5.412658773652684552, -3.125000000000099920, -66.56698729810783277 ) ) ;
#22597=CARTESIAN_POINT ( 'NONE',  ( 4.763139720814407951, 2.750000000000002665, -52.75000000000002132 ) ) ;
#22598=CARTESIAN_POINT ( 'NONE',  ( 5.196152422706629359, 3.000000000000002665, -56.03867513459481842 ) ) ;
#22599=CARTESIAN_POINT ( 'NONE',  ( 5.999999999999999112, 2.951592740943527306E-14, -153.0863248654052313 ) ) ;
#22600=CARTESIAN_POINT ( 'NONE',  ( 4.763139720814407951, 2.750000000000002665, -129.2500000000000284 ) ) ;
#22601=CARTESIAN_POINT ( 'NONE',  ( 3.464101615137852974, 5.999999999999884537, -138.4136751345947971 ) ) ;
#22606=DIRECTION ( 'NONE',  ( -7.147005652999508048E-36, 5.642372883946980038E-36, 1.000000000000000000 ) ) ;
#22611=CARTESIAN_POINT ( 'NONE',  ( -11.00000000000001599, 1.957734142605926671E-15, 1.386142938489641429E-34 ) ) ;
#22612=EDGE_CURVE ( 'NONE', #14180, #2929, #25358, .T. ) ;
#22613=CARTESIAN_POINT ( 'NONE',  ( -3.608439182435115633, 6.249999999999965361, -119.4419872981078612 ) ) ;
#22614=CARTESIAN_POINT ( 'NONE',  ( -3.464101615137757051, -5.999999999999979572, -110.0863248654051887 ) ) ;
#22620=EDGE_CURVE ( 'NONE', #6123, #3196, #24006, .T. ) ;
#22621=VECTOR ( 'NONE', #15832, 1000.000000000000000 ) ;
#22622=ORIENTED_EDGE ( 'NONE', *, *, #29407, .F. ) ;
#22623=VERTEX_POINT ( 'NONE', #13592 ) ;
#22624=DIRECTION ( 'NONE',  ( -7.147005652999508048E-36, 5.642372883946980038E-36, 1.000000000000000000 ) ) ;
#22628=CARTESIAN_POINT ( 'NONE',  ( -3.608439182435115633, 6.249999999999965361, -69.30801270189220986 ) ) ;
#22630=CARTESIAN_POINT ( 'NONE',  ( 5.196152422706629359, 3.000000000000002665, -102.5386751345948539 ) ) ;
#22631=DIRECTION ( 'NONE',  ( 1.000000000000000000, -5.551115123125773458E-17, -1.260129944081490338E-35 ) ) ;
#22632=CARTESIAN_POINT ( 'NONE',  ( 0.000000000000000000, 5.499999999999991118, -130.5000000000000000 ) ) ;
#22635=APPLICATION_CONTEXT ( 'automotive_design' ) ;
#22636=CARTESIAN_POINT ( 'NONE',  ( -3.175426480542816066, -5.500000000000057732, -62.37500000000001421 ) ) ;
#22638=CARTESIAN_POINT ( 'NONE',  ( 0.000000000000000000, 5.999999999999977796, -70.21132486540521711 ) ) ;
#22650=ORIENTED_EDGE ( 'NONE', *, *, #26065, .F. ) ;
#22652=CARTESIAN_POINT ( 'NONE',  ( 4.763139720814407951, 2.750000000000002665, -148.7500000000000568 ) ) ;
#22655=CARTESIAN_POINT ( 'NONE',  ( -4.763139720814407951, -2.750000000000016431, -77.50000000000001421 ) ) ;
#22656=AXIS2_PLACEMENT_3D ( 'NONE', #4479, #11275, #16504 ) ;
#22658=CARTESIAN_POINT ( 'NONE',  ( 3.608439182435180470, -6.249999999999997335, -95.55801270189226670 ) ) ;
#22659=CARTESIAN_POINT ( 'NONE',  ( -5.197786390520544586, -9.697480688945354643, -28.02189831943639220 ) ) ;
#22660=DIRECTION ( 'NONE',  ( -7.147005652999508048E-36, 5.642372883946980038E-36, 1.000000000000000000 ) ) ;
#22661=CARTESIAN_POINT ( 'NONE',  ( 5.999999999999949374, 1.607695154586804565, -99.01933756729741276 ) ) ;
#22662=CARTESIAN_POINT ( 'NONE',  ( -5.999999999999963585, 1.780251999655701777E-13, -65.33632486540521711 ) ) ;
#22663=CARTESIAN_POINT ( 'NONE',  ( 4.763139720814407951, -2.749999999999988454, -156.5000000000000284 ) ) ;
#22666=CARTESIAN_POINT ( 'NONE',  ( 3.175426480543072749, -5.500000000000105693, -84.62499999999997158 ) ) ;
#22667=CARTESIAN_POINT ( 'NONE',  ( -5.999999999999963585, -1.487416814333745711E-14, -154.4136751345947971 ) ) ;
#22669=CARTESIAN_POINT ( 'NONE',  ( -6.350852961085760029, -1.281975124255709124E-13, -74.62500000000000000 ) ) ;
#22672=CARTESIAN_POINT ( 'NONE',  ( -5.999999999999963585, 8.134310703387671600E-14, -140.3363248654052313 ) ) ;
#22678=CYLINDRICAL_SURFACE ( 'NONE', #9731, 6.000000000000000888 ) ;
#22679=CARTESIAN_POINT ( 'NONE',  ( -5.196152422706601826, 2.999999999999975131, -174.0386751345948255 ) ) ;
#22680=EDGE_CURVE ( 'NONE', #899, #25744, #4173, .T. ) ;
#22681=( BOUNDED_CURVE ( )  B_SPLINE_CURVE ( 2, ( #27298, #9191, #18430, #8577, #18585, #22575, #3804, #13232, #22873 ),
 .UNSPECIFIED., .F., .T. ) 
 B_SPLINE_CURVE_WITH_KNOTS ( ( 3, 2, 2, 2, 3 ),
 ( 0.2138888888888887951, 0.2148148148148147918, 0.2166666666666666741, 0.2185185185185185563, 0.2194444444444444420 ),
 .UNSPECIFIED. ) 
 CURVE ( )  GEOMETRIC_REPRESENTATION_ITEM ( )  RATIONAL_B_SPLINE_CURVE ( ( 0.9330127018922194093, 0.9330127018922154125, 1.000000000000000000, 0.8660254037844388186, 1.000000000000000000, 0.8660254037844388186, 1.000000000000000000, 0.9330127018922194093, 0.9330127018922194093 ) ) 
 REPRESENTATION_ITEM ( '' )  );
#22682=EDGE_LOOP ( 'NONE', ( #24027, #14619, #6771, #22275 ) ) ;
#22687=CARTESIAN_POINT ( 'NONE',  ( 6.000000000000052403, -1.607695154586662678, -115.6533121635129930 ) ) ;
#22690=CARTESIAN_POINT ( 'NONE',  ( 3.175426480543072749, -5.500000000000105693, -93.62500000000002842 ) ) ;
#22692=CARTESIAN_POINT ( 'NONE',  ( -7.216878364870328078, 0.000000000000000000, -118.5580127018922525 ) ) ;
#22694=CARTESIAN_POINT ( 'NONE',  ( 6.000000000000000888, 7.762456499804234384E-14, -123.6636751345948255 ) ) ;
#22696=CARTESIAN_POINT ( 'NONE',  ( -3.464101615137725076, 5.999999999999979572, -52.08632486540516737 ) ) ;
#22697=CARTESIAN_POINT ( 'NONE',  ( -7.216878364870328078, 0.000000000000000000, -55.55801270189220986 ) ) ;
#22698=ORIENTED_EDGE ( 'NONE', *, *, #19693, .F. ) ;
#22701=CARTESIAN_POINT ( 'NONE',  ( 0.000000000000000000, -5.999999999999991118, -166.9613248654052029 ) ) ;
#22702=CARTESIAN_POINT ( 'NONE',  ( -4.763139720814407951, -2.750000000000016431, -160.0000000000000284 ) ) ;
#22704=CARTESIAN_POINT ( 'NONE',  ( 0.000000000000000000, 0.000000000000000000, 0.000000000000000000 ) ) ;
#22705=CARTESIAN_POINT ( 'NONE',  ( -3.175426480542816066, 5.499999999999865885, -109.3750000000000426 ) ) ;
#22708=CARTESIAN_POINT ( 'NONE',  ( -4.763139720814407951, -2.750000000000016431, -100.0000000000000284 ) ) ;
#22710=CARTESIAN_POINT ( 'NONE',  ( -3.464101615137725076, 5.999999999999979572, -118.0863248654052029 ) ) ;
#22715=EDGE_CURVE ( 'NONE', #9072, #10931, #12647, .T. ) ;
#22716=VERTEX_POINT ( 'NONE', #27659 ) ;
#22717=CARTESIAN_POINT ( 'NONE',  ( -5.196152422706573404, -3.000000000000002665, -170.2113248654052313 ) ) ;
#22718=CARTESIAN_POINT ( 'NONE',  ( 3.608439182435180470, 6.249999999999982236, -88.19198729810783277 ) ) ;
#22721=DIRECTION ( 'NONE',  ( 1.000000000000000000, -5.551115123125773458E-17, -1.260129944081490338E-35 ) ) ;
#22722=VECTOR ( 'NONE', #19967, 1000.000000000000000 ) ;
#22726=( BOUNDED_CURVE ( )  B_SPLINE_CURVE ( 2, ( #667, #19571, #951, #28600, #16838, #5560, #15119, #8024, #7568 ),
 .UNSPECIFIED., .F., .F. ) 
 B_SPLINE_CURVE_WITH_KNOTS ( ( 3, 2, 2, 2, 3 ),
 ( 0.9638888888888889062, 0.9648148148148147918, 0.9666666666666666741, 0.9685185185185185563, 0.9694444444444444420 ),
 .UNSPECIFIED. ) 
 CURVE ( )  GEOMETRIC_REPRESENTATION_ITEM ( )  RATIONAL_B_SPLINE_CURVE ( ( 0.9330127018922194093, 0.9330127018922234061, 1.000000000000000000, 0.8660254037844388186, 1.000000000000000000, 0.8660254037844388186, 1.000000000000000000, 0.9330127018922194093, 0.9330127018922194093 ) ) 
 REPRESENTATION_ITEM ( '' )  );
#22727=CARTESIAN_POINT ( 'NONE',  ( 6.350852961086080661, -9.614813431917819062E-14, -118.8750000000000142 ) ) ;
#22728=CARTESIAN_POINT ( 'NONE',  ( 3.608439182435180470, 6.249999999999982236, -141.5580127018922099 ) ) ;
#22729=VERTEX_POINT ( 'NONE', #23091 ) ;
#22731=CARTESIAN_POINT ( 'NONE',  ( 2.775557561562891351E-14, -6.250000000000061284, -120.3169872981078043 ) ) ;
#22732=CARTESIAN_POINT ( 'NONE',  ( 3.608439182435180470, -6.249999999999997335, -174.1919872981077901 ) ) ;
#22733=CARTESIAN_POINT ( 'NONE',  ( -4.763139720814407951, -2.750000000000016431, -172.0000000000000284 ) ) ;
#22738=CARTESIAN_POINT ( 'NONE',  ( 3.464101615137852974, 5.999999999999884537, -163.9136751345947971 ) ) ;
#22741=CARTESIAN_POINT ( 'NONE',  ( 0.000000000000000000, 0.000000000000000000, -180.0000000000000568 ) ) ;
#22743=CARTESIAN_POINT ( 'NONE',  ( -5.412658773652684552, -3.125000000000099920, -77.06698729810779014 ) ) ;
#22744=CARTESIAN_POINT ( 'NONE',  ( 3.608439182435180470, -6.249999999999997335, -55.69198729810780435 ) ) ;
#22745=EDGE_CURVE ( 'NONE', #25700, #24608, #20786, .T. ) ;
#22747=CARTESIAN_POINT ( 'NONE',  ( 3.175426480543072749, -5.500000000000105693, -53.12500000000002842 ) ) ;
#22750=CARTESIAN_POINT ( 'NONE',  ( -4.763139720814407951, 2.749999999999946709, -128.7500000000000284 ) ) ;
#22753=ORIENTED_EDGE ( 'NONE', *, *, #1551, .F. ) ;
#22754=CARTESIAN_POINT ( 'NONE',  ( 6.000000000000000888, 7.762456499804234384E-14, -118.5863248654052313 ) ) ;
#22761=CARTESIAN_POINT ( 'NONE',  ( -5.412658773652739619, 3.124999999999975131, -117.8169872981078612 ) ) ;
#22764=CARTESIAN_POINT ( 'NONE',  ( 6.000000000000000888, -3.330669073875464691E-16, -7.560779664488942560E-35 ) ) ;
#22766=( BOUNDED_CURVE ( )  B_SPLINE_CURVE ( 2, ( #23583, #214, #29795, #15879, #11092, #17550, #15722, #3525, #3677 ),
 .UNSPECIFIED., .F., .T. ) 
 B_SPLINE_CURVE_WITH_KNOTS ( ( 3, 2, 2, 2, 3 ),
 ( 0.3638888888888889284, 0.3648148148148148140, 0.3666666666666666408, 0.3685185185185185230, 0.3694444444444444087 ),
 .UNSPECIFIED. ) 
 CURVE ( )  GEOMETRIC_REPRESENTATION_ITEM ( )  RATIONAL_B_SPLINE_CURVE ( ( 0.9330127018922194093, 0.9330127018922214077, 1.000000000000000000, 0.8660254037844388186, 1.000000000000000000, 0.8660254037844388186, 1.000000000000000000, 0.9330127018922214077, 0.9330127018922194093 ) ) 
 REPRESENTATION_ITEM ( '' )  );
#22768=ORIENTED_EDGE ( 'NONE', *, *, #9855, .T. ) ;
#22769=CARTESIAN_POINT ( 'NONE',  ( -4.763139720814407951, 2.749999999999946709, -50.75000000000001421 ) ) ;
#22773=CARTESIAN_POINT ( 'NONE',  ( -3.608439182435115633, 6.249999999999965361, -64.80801270189225249 ) ) ;
#22775=( BOUNDED_CURVE ( )  B_SPLINE_CURVE ( 2, ( #21394, #25982, #9867, #4926, #7535, #5225, #2925, #3074, #19390 ),
 .UNSPECIFIED., .F., .T. ) 
 B_SPLINE_CURVE_WITH_KNOTS ( ( 3, 2, 2, 2, 3 ),
 ( 0.7138888888888887951, 0.7148148148148147918, 0.7166666666666666741, 0.7185185185185185563, 0.7194444444444444420 ),
 .UNSPECIFIED. ) 
 CURVE ( )  GEOMETRIC_REPRESENTATION_ITEM ( )  RATIONAL_B_SPLINE_CURVE ( ( 0.9330127018922194093, 0.9330127018922114157, 1.000000000000000000, 0.8660254037844388186, 1.000000000000000000, 0.8660254037844388186, 1.000000000000000000, 0.9330127018922194093, 0.9330127018922194093 ) ) 
 REPRESENTATION_ITEM ( '' )  );
#22777=CYLINDRICAL_SURFACE ( 'NONE', #11931, 6.000000000000000888 ) ;
#22778=CARTESIAN_POINT ( 'NONE',  ( -5.999999999999963585, 1.780251999655701777E-13, -107.3363248654052455 ) ) ;
#22781=CARTESIAN_POINT ( 'NONE',  ( -5.999999999999963585, -1.487416814333745711E-14, -67.41367513459481131 ) ) ;
#22782=CARTESIAN_POINT ( 'NONE',  ( -3.175426480542816066, -5.500000000000057732, -125.3749999999999858 ) ) ;
#22784=CARTESIAN_POINT ( 'NONE',  ( 5.412658773652712085, -3.125000000000086153, -146.4330127018922383 ) ) ;
#22786=ORIENTED_EDGE ( 'NONE', *, *, #1788, .T. ) ;
#22787=CARTESIAN_POINT ( 'NONE',  ( -3.175426480542816066, -5.500000000000057732, -65.37500000000001421 ) ) ;
#22788=CARTESIAN_POINT ( 'NONE',  ( -5.196152422706601826, 2.999999999999975131, -123.9613248654052313 ) ) ;
#22789=EDGE_CURVE ( 'NONE', #3881, #16950, #30286, .T. ) ;
#22793=EDGE_CURVE ( 'NONE', #27302, #15456, #9304, .T. ) ;
#22796=LINE ( 'NONE', #3725, #16821 ) ;
#22798=CARTESIAN_POINT ( 'NONE',  ( -5.999999999999963585, 1.780251999655701777E-13, -49.41367513459484684 ) ) ;
#22801=VERTEX_POINT ( 'NONE', #12048 ) ;
#22802=CARTESIAN_POINT ( 'NONE',  ( -6.350852961085760029, -1.281975124255709124E-13, -146.6250000000000284 ) ) ;
#22804=ORIENTED_EDGE ( 'NONE', *, *, #21365, .T. ) ;
#22805=CARTESIAN_POINT ( 'NONE',  ( 4.763139720814407951, -2.749999999999988454, -74.00000000000001421 ) ) ;
#22807=CARTESIAN_POINT ( 'NONE',  ( 5.412658773652712085, -3.125000000000086153, -87.93301270189223828 ) ) ;
#22808=CARTESIAN_POINT ( 'NONE',  ( -5.681812044562425612, -9.420575401947244742, -23.03339967402432720 ) ) ;
#22809=EDGE_CURVE ( 'NONE', #29768, #13111, #28563, .T. ) ;
#22810=FACE_OUTER_BOUND ( 'NONE', #17226, .T. ) ;
#22813=CARTESIAN_POINT ( 'NONE',  ( -4.763139720814407951, -2.750000000000016431, -155.5000000000000284 ) ) ;
#22815=CARTESIAN_POINT ( 'NONE',  ( -5.999999999999963585, 1.780251999655701777E-13, -82.41367513459481131 ) ) ;
#22816=CARTESIAN_POINT ( 'NONE',  ( -4.763139720814407951, 2.749999999999946709, -89.75000000000000000 ) ) ;
#22819=CARTESIAN_POINT ( 'NONE',  ( 3.175426480543072749, -5.500000000000105693, -77.12500000000001421 ) ) ;
#22822=CARTESIAN_POINT ( 'NONE',  ( 6.000000000000000888, 5.577813053751546416E-15, -165.0863248654052029 ) ) ;
#22823=CARTESIAN_POINT ( 'NONE',  ( 6.000000000000001776, 5.345404176511898156E-15, -174.6636751345948539 ) ) ;
#22827=CARTESIAN_POINT ( 'NONE',  ( -5.999999999999963585, -1.487416814333745711E-14, -54.83632486540523132 ) ) ;
#22828=CARTESIAN_POINT ( 'NONE',  ( -5.999999999999963585, -1.487416814333745711E-14, -134.3363248654052313 ) ) ;
#22829=CARTESIAN_POINT ( 'NONE',  ( 6.000000000000000888, 1.607695154586715303, -170.0966878364870354 ) ) ;
#22832=CARTESIAN_POINT ( 'NONE',  ( -6.000000000000007105, -1.607695154586655129, -109.3466878364870354 ) ) ;
#22834=CARTESIAN_POINT ( 'NONE',  ( -5.196152422706601826, 2.999999999999975131, -156.9613248654052597 ) ) ;
#22839=CARTESIAN_POINT ( 'NONE',  ( -2.775557561562891351E-14, -5.500000000000115463, -101.2500000000000000 ) ) ;
#22841=CARTESIAN_POINT ( 'NONE',  ( 3.608439182435180470, -6.249999999999997335, -104.5580127018922525 ) ) ;
#22843=CARTESIAN_POINT ( 'NONE',  ( 0.1999138633143864585, 11.00000000000000533, -19.00000000000001066 ) ) ;
#22845=AXIS2_PLACEMENT_3D ( 'NONE', #17474, #8534, #8696 ) ;
#22846=CARTESIAN_POINT ( 'NONE',  ( 3.175426480543072749, 5.499999999999865885, -163.6249999999999716 ) ) ;
#22847=EDGE_CURVE ( 'NONE', #2600, #18174, #467, .T. ) ;
#22848=DIRECTION ( 'NONE',  ( -7.147005652999508048E-36, 5.642372883946980038E-36, 1.000000000000000000 ) ) ;
#22849=ORIENTED_EDGE ( 'NONE', *, *, #25577, .F. ) ;
#22850=CARTESIAN_POINT ( 'NONE',  ( -5.196152422706601826, 2.999999999999975131, -153.0386751345948539 ) ) ;
#22852=CARTESIAN_POINT ( 'NONE',  ( -4.763139720814407951, -2.750000000000016431, -166.0000000000000284 ) ) ;
#22854=CARTESIAN_POINT ( 'NONE',  ( 3.175426480543072749, -5.500000000000105693, -105.6250000000000284 ) ) ;
#22856=CARTESIAN_POINT ( 'NONE',  ( 5.196152422706629359, 3.000000000000002665, -87.53867513459483973 ) ) ;
#22857=EDGE_CURVE ( 'NONE', #18615, #14907, #28124, .T. ) ;
#22858=CARTESIAN_POINT ( 'NONE',  ( -3.175426480542816510, 5.499999999999865885, -97.37499999999998579 ) ) ;
#22859=( BOUNDED_CURVE ( )  B_SPLINE_CURVE ( 2, ( #22828, #3763, #1769, #15336, #11172, #24656, #1149, #10549, #20062 ),
 .UNSPECIFIED., .F., .T. ) 
 B_SPLINE_CURVE_WITH_KNOTS ( ( 3, 2, 2, 2, 3 ),
 ( 0.6527777777777777901, 0.6537037037037036757, 0.6555555555555555580, 0.6574074074074074403, 0.6583333333333333259 ),
 .UNSPECIFIED. ) 
 CURVE ( )  GEOMETRIC_REPRESENTATION_ITEM ( )  RATIONAL_B_SPLINE_CURVE ( ( 0.9330127018922194093, 0.9330127018922194093, 1.000000000000000000, 0.8660254037844388186, 1.000000000000000000, 0.8660254037844388186, 1.000000000000000000, 0.9330127018922194093, 0.9330127018922194093 ) ) 
 REPRESENTATION_ITEM ( '' )  );
#22867=CARTESIAN_POINT ( 'NONE',  ( 6.000000000000000888, 7.762456499804234384E-14, -133.5863248654052029 ) ) ;
#22871=CARTESIAN_POINT ( 'NONE',  ( 5.412658773652712085, -3.125000000000086153, -87.06698729810780435 ) ) ;
#22872=ORIENTED_EDGE ( 'NONE', *, *, #18669, .T. ) ;
#22873=CARTESIAN_POINT ( 'NONE',  ( -5.999999999999963585, -1.487416814333745711E-14, -75.83632486540521711 ) ) ;
#22874=EDGE_LOOP ( 'NONE', ( #17916, #9375, #4872, #9548 ) ) ;
#22876=CARTESIAN_POINT ( 'NONE',  ( 0.000000000000000000, 5.499999999999991118, -121.5000000000000568 ) ) ;
#22878=CARTESIAN_POINT ( 'NONE',  ( -3.608439182435115633, 6.249999999999965361, -129.3080127018922383 ) ) ;
#22880=CARTESIAN_POINT ( 'NONE',  ( 5.196152422706629359, 3.000000000000002665, -57.53867513459481842 ) ) ;
#22881=CARTESIAN_POINT ( 'NONE',  ( 2.775557561562891351E-14, 6.250000000000033751, -121.0669872981078328 ) ) ;
#22882=CARTESIAN_POINT ( 'NONE',  ( 5.412658773652739619, 3.124999999999988898, -179.8169872981077901 ) ) ;
#22885=EDGE_CURVE ( 'NONE', #4758, #6403, #9490, .T. ) ;
#22892=CARTESIAN_POINT ( 'NONE',  ( 5.196152422706629359, 3.000000000000002665, -133.4613248654052313 ) ) ;
#22894=CARTESIAN_POINT ( 'NONE',  ( -7.216878364870328078, 0.000000000000000000, -77.19198729810784698 ) ) ;
#22895=CARTESIAN_POINT ( 'NONE',  ( -5.412658773652684552, -3.125000000000099920, -62.06698729810783277 ) ) ;
#22897=CARTESIAN_POINT ( 'NONE',  ( 4.763139720814407951, -2.749999999999988454, -47.00000000000004263 ) ) ;
#22898=CYLINDRICAL_SURFACE ( 'NONE', #967, 6.000000000000000888 ) ;
#22899=CARTESIAN_POINT ( 'NONE',  ( 3.175426480543072749, 5.499999999999865885, -121.6250000000000284 ) ) ;
#22901=EDGE_LOOP ( 'NONE', ( #17176, #27558, #29069, #15817 ) ) ;
#22903=CARTESIAN_POINT ( 'NONE',  ( 5.196152422706629359, 3.000000000000002665, -122.9613248654052313 ) ) ;
#22911=CARTESIAN_POINT ( 'NONE',  ( -3.608439182435115633, 6.249999999999965361, -114.9419872981078328 ) ) ;
#22913=CARTESIAN_POINT ( 'NONE',  ( 5.196152422706629359, -2.999999999999988898, -109.7113248654052455 ) ) ;
#22916=VERTEX_POINT ( 'NONE', #24873 ) ;
#22919=CARTESIAN_POINT ( 'NONE',  ( -3.608439182435052128, -6.250000000000110134, -145.9419872981078470 ) ) ;
#22926=CARTESIAN_POINT ( 'NONE',  ( -5.999999999999963585, 1.780251999655701777E-13, -61.41367513459483973 ) ) ;
#22927=CARTESIAN_POINT ( 'NONE',  ( -7.216878364870328078, 0.000000000000000000, -70.55801270189220986 ) ) ;
#22931=CARTESIAN_POINT ( 'NONE',  ( -3.464101615137757051, -5.999999999999979572, -178.1636751345948255 ) ) ;
#22932=DIRECTION ( 'NONE',  ( 1.000000000000000000, -5.551115123125774690E-17, 0.000000000000000000 ) ) ;
#22933=CARTESIAN_POINT ( 'NONE',  ( -3.464101615137757051, -5.999999999999979572, -155.6636751345947971 ) ) ;
#22935=LINE ( 'NONE', #2036, #8662 ) ;
#22937=CARTESIAN_POINT ( 'NONE',  ( 3.175426480543072749, -5.500000000000105693, -128.1250000000000000 ) ) ;
#22938=CYLINDRICAL_SURFACE ( 'NONE', #11756, 6.000000000000000888 ) ;
#22939=CARTESIAN_POINT ( 'NONE',  ( -3.608439182435115633, 6.249999999999965361, -145.8080127018922383 ) ) ;
#22940=CARTESIAN_POINT ( 'NONE',  ( -5.999999999999963585, 1.780251999655701777E-13, -65.33632486540521711 ) ) ;
#22941=ORIENTED_EDGE ( 'NONE', *, *, #8773, .T. ) ;
#22942=CARTESIAN_POINT ( 'NONE',  ( -3.175426480542816066, 5.499999999999865885, -52.37500000000002842 ) ) ;
#22943=CARTESIAN_POINT ( 'NONE',  ( 5.999999999999999112, 2.951592740943527306E-14, -153.6636751345948539 ) ) ;
#22946=EDGE_LOOP ( 'NONE', ( #3171, #22505, #28952, #30231 ) ) ;
#22955=ORIENTED_EDGE ( 'NONE', *, *, #10762, .F. ) ;
#22957=CARTESIAN_POINT ( 'NONE',  ( 4.763139720814407951, 2.750000000000002665, -136.7500000000000284 ) ) ;
#22960=ORIENTED_EDGE ( 'NONE', *, *, #28099, .T. ) ;
#22961=CARTESIAN_POINT ( 'NONE',  ( -4.763139720814407951, -2.750000000000016431, -68.50000000000000000 ) ) ;
#22963=EDGE_CURVE ( 'NONE', #3491, #26834, #24260, .T. ) ;
#22964=CARTESIAN_POINT ( 'NONE',  ( 2.775557561562891351E-14, -11.00000000000001066, -31.00000000000002842 ) ) ;
#22972=CARTESIAN_POINT ( 'NONE',  ( 6.350852961086080661, -9.614813431917819062E-14, -145.8750000000000284 ) ) ;
#22974=CARTESIAN_POINT ( 'NONE',  ( -5.412658773652739619, 3.124999999999975131, -157.6830127018922099 ) ) ;
#22975=DIRECTION ( 'NONE',  ( -1.000000000000000000, -3.330669073875465184E-16, 6.770847460736368028E-36 ) ) ;
#22976=CARTESIAN_POINT ( 'NONE',  ( -4.763139720814407951, 2.749999999999946709, -86.75000000000000000 ) ) ;
#22978=CARTESIAN_POINT ( 'NONE',  ( 4.763139720814407951, 2.750000000000002665, -73.75000000000004263 ) ) ;
#22979=FACE_OUTER_BOUND ( 'NONE', #2783, .T. ) ;
#22981=CARTESIAN_POINT ( 'NONE',  ( 6.000000000000000888, -3.330669073875464691E-16, -7.560779664488942560E-35 ) ) ;
#22982=CARTESIAN_POINT ( 'NONE',  ( 0.000000000000000000, 0.000000000000000000, 0.000000000000000000 ) ) ;
#22984=CARTESIAN_POINT ( 'NONE',  ( -5.196152422706601826, 2.999999999999975131, -118.5386751345948113 ) ) ;
#22985=CARTESIAN_POINT ( 'NONE',  ( -5.999999999999963585, 8.134310703387671600E-14, -146.3363248654052313 ) ) ;
#22992=CARTESIAN_POINT ( 'NONE',  ( 0.000000000000000000, -5.999999999999991118, -85.03867513459483973 ) ) ;
#22993=ORIENTED_EDGE ( 'NONE', *, *, #30161, .T. ) ;
#22995=ORIENTED_EDGE ( 'NONE', *, *, #10478, .F. ) ;
#22996=CARTESIAN_POINT ( 'NONE',  ( -4.763139720814407951, 2.749999999999946709, -98.75000000000000000 ) ) ;
#22997=EDGE_CURVE ( 'NONE', #6403, #25123, #8483, .T. ) ;
#22998=CARTESIAN_POINT ( 'NONE',  ( -3.608439182435052128, -6.250000000000110134, -110.8080127018922099 ) ) ;
#23000=DIRECTION ( 'NONE',  ( -7.147005652999508048E-36, 5.642372883946980038E-36, 1.000000000000000000 ) ) ;
#23001=DIRECTION ( 'NONE',  ( -7.147005652999508048E-36, 5.642372883946980038E-36, 1.000000000000000000 ) ) ;
#23003=CARTESIAN_POINT ( 'NONE',  ( -5.999999999999956479, -1.607695154586745057, -106.3466878364870354 ) ) ;
#23004=ORIENTED_EDGE ( 'NONE', *, *, #21290, .T. ) ;
#23005=FACE_OUTER_BOUND ( 'NONE', #19954, .T. ) ;
#23007=CARTESIAN_POINT ( 'NONE',  ( 0.000000000000000000, 5.499999999999991118, -171.0000000000000284 ) ) ;
#23009=CARTESIAN_POINT ( 'NONE',  ( -3.175426480542816510, 5.499999999999865885, -160.3750000000000000 ) ) ;
#23011=CARTESIAN_POINT ( 'NONE',  ( 0.000000000000000000, 5.499999999999991118, -109.5000000000000426 ) ) ;
#23013=CARTESIAN_POINT ( 'NONE',  ( 6.000000000000000888, -3.330669073875464691E-16, -7.560779664488942560E-35 ) ) ;
#23014=CARTESIAN_POINT ( 'NONE',  ( 6.350852961086080661, -9.614813431917819062E-14, -97.87499999999998579 ) ) ;
#23016=ORIENTED_EDGE ( 'NONE', *, *, #13974, .T. ) ;
#23024=CARTESIAN_POINT ( 'NONE',  ( -3.608439182435052128, -6.250000000000110134, -87.44198729810781856 ) ) ;
#23027=ORIENTED_EDGE ( 'NONE', *, *, #25722, .F. ) ;
#23029=ORIENTED_EDGE ( 'NONE', *, *, #21101, .T. ) ;
#23032=ORIENTED_EDGE ( 'NONE', *, *, #22857, .T. ) ;
#23033=CARTESIAN_POINT ( 'NONE',  ( -3.175426480542816510, 5.499999999999865885, -121.3750000000000284 ) ) ;
#23036=( BOUNDED_CURVE ( )  B_SPLINE_CURVE ( 2, ( #7733, #14409, #16994, #17141, #14681, #14258, #7437, #5421, #21437 ),
 .UNSPECIFIED., .F., .T. ) 
 B_SPLINE_CURVE_WITH_KNOTS ( ( 3, 2, 2, 2, 3 ),
 ( 0.2638888888888889506, 0.2648148148148148362, 0.2666666666666667185, 0.2685185185185184897, 0.2694444444444443754 ),
 .UNSPECIFIED. ) 
 CURVE ( )  GEOMETRIC_REPRESENTATION_ITEM ( )  RATIONAL_B_SPLINE_CURVE ( ( 0.9330127018922194093, 0.9330127018922234061, 1.000000000000000000, 0.8660254037844388186, 1.000000000000000000, 0.8660254037844388186, 1.000000000000000000, 0.9330127018922234061, 0.9330127018922194093 ) ) 
 REPRESENTATION_ITEM ( '' )  );
#23037=CARTESIAN_POINT ( 'NONE',  ( 5.412658773652712085, -3.125000000000086153, -128.4330127018922099 ) ) ;
#23039=AXIS2_PLACEMENT_3D ( 'NONE', #3367, #12345, #3215 ) ;
#23040=CARTESIAN_POINT ( 'NONE',  ( -5.412658773652739619, 3.124999999999975131, -165.8169872981077901 ) ) ;
#23041=CARTESIAN_POINT ( 'NONE',  ( 5.412658773652739619, 3.124999999999988898, -173.8169872981077901 ) ) ;
#23043=CARTESIAN_POINT ( 'NONE',  ( -5.999999999999944933, 1.607695154586759934, -146.9806624327026157 ) ) ;
#23047=( BOUNDED_CURVE ( )  B_SPLINE_CURVE ( 2, ( #30045, #17958, #6547, #15663, #11190, #1634, #3923, #29887, #18407 ),
 .UNSPECIFIED., .F., .T. ) 
 B_SPLINE_CURVE_WITH_KNOTS ( ( 3, 2, 2, 2, 3 ),
 ( 0.2805555555555555580, 0.2814814814814814992, 0.2833333333333333259, 0.2851851851851852082, 0.2861111111111111494 ),
 .UNSPECIFIED. ) 
 CURVE ( )  GEOMETRIC_REPRESENTATION_ITEM ( )  RATIONAL_B_SPLINE_CURVE ( ( 0.9330127018922194093, 0.9330127018922194093, 1.000000000000000000, 0.8660254037844388186, 1.000000000000000000, 0.8660254037844388186, 1.000000000000000000, 0.9330127018922174109, 0.9330127018922194093 ) ) 
 REPRESENTATION_ITEM ( '' )  );
#23048=CARTESIAN_POINT ( 'NONE',  ( -6.000000000000023093, 1.607695154586625819, -132.9033121635129930 ) ) ;
#23051=CARTESIAN_POINT ( 'NONE',  ( 5.412658773652739619, 3.124999999999988898, -76.31698729810781856 ) ) ;
#23052=CARTESIAN_POINT ( 'NONE',  ( 2.775557561562891351E-14, -6.250000000000061284, -58.81698729810780435 ) ) ;
#23053=CARTESIAN_POINT ( 'NONE',  ( 3.175426480543072749, 5.499999999999865885, -52.62500000000002842 ) ) ;
#23054=FACE_OUTER_BOUND ( 'NONE', #4843, .T. ) ;
#23055=CARTESIAN_POINT ( 'NONE',  ( 6.000000000000000888, -1.859271017917181981E-14, -47.16367513459483263 ) ) ;
#23057=CARTESIAN_POINT ( 'NONE',  ( -3.175426480542816510, 5.499999999999865885, -118.3750000000000142 ) ) ;
#23058=CARTESIAN_POINT ( 'NONE',  ( 3.175426480543072749, 5.499999999999865885, -156.1250000000000000 ) ) ;
#23060=ORIENTED_EDGE ( 'NONE', *, *, #26796, .F. ) ;
#23067=ORIENTED_EDGE ( 'NONE', *, *, #10270, .T. ) ;
#23071=CARTESIAN_POINT ( 'NONE',  ( 7.216878364870455975, -6.409875621278545621E-14, -116.9419872981078328 ) ) ;
#23075=DIRECTION ( 'NONE',  ( -7.147005652999508048E-36, 5.642372883946980038E-36, 1.000000000000000000 ) ) ;
#23076=ORIENTED_EDGE ( 'NONE', *, *, #24941, .T. ) ;
#23077=ORIENTED_EDGE ( 'NONE', *, *, #20343, .F. ) ;
#23080=CARTESIAN_POINT ( 'NONE',  ( 7.216878364870455975, -6.409875621278545621E-14, -151.4419872981078186 ) ) ;
#23082=CARTESIAN_POINT ( 'NONE',  ( 0.000000000000000000, -5.999999999999991118, -93.46132486540520290 ) ) ;
#23086=CARTESIAN_POINT ( 'NONE',  ( -5.999999999999963585, -1.487416814333745711E-14, -137.9136751345947971 ) ) ;
#23087=CARTESIAN_POINT ( 'NONE',  ( 5.412658773652739619, 3.124999999999988898, -65.18301270189225249 ) ) ;
#23090=CARTESIAN_POINT ( 'NONE',  ( -5.999999999999971578, 1.607695154586715303, -101.9806624327026441 ) ) ;
#23091=CARTESIAN_POINT ( 'NONE',  ( 6.000000000000000888, -1.859271017917181981E-14, -89.16367513459483973 ) ) ;
#23093=CARTESIAN_POINT ( 'NONE',  ( 3.464101615137852974, 5.999999999999884537, -115.3363248654052029 ) ) ;
#23096=CARTESIAN_POINT ( 'NONE',  ( -3.175426480542816066, -5.500000000000057732, -120.8750000000000284 ) ) ;
#23097=CARTESIAN_POINT ( 'NONE',  ( 5.412658773652712085, -3.125000000000086153, -143.4330127018922383 ) ) ;
#23098=CARTESIAN_POINT ( 'NONE',  ( 5.196152422706629359, 3.000000000000002665, -113.0386751345948682 ) ) ;
#23100=ORIENTED_EDGE ( 'NONE', *, *, #26482, .F. ) ;
#23101=CARTESIAN_POINT ( 'NONE',  ( -6.350852961085760029, -1.281975124255709124E-13, -53.62500000000002842 ) ) ;
#23104=CARTESIAN_POINT ( 'NONE',  ( -5.999999999999963585, 0.000000000000000000, -179.3363248654052313 ) ) ;
#23105=EDGE_LOOP ( 'NONE', ( #13118, #17434 ) ) ;
#23109=CARTESIAN_POINT ( 'NONE',  ( 0.000000000000000000, 0.000000000000000000, 0.000000000000000000 ) ) ;
#23113=CARTESIAN_POINT ( 'NONE',  ( -6.350852961085760029, -1.281975124255709124E-13, -137.6250000000000568 ) ) ;
#23118=CARTESIAN_POINT ( 'NONE',  ( -3.175426480542816510, 5.499999999999865885, -67.37500000000002842 ) ) ;
#23119=CARTESIAN_POINT ( 'NONE',  ( -3.464101615137757051, -5.999999999999979572, -164.6636751345947687 ) ) ;
#23121=CYLINDRICAL_SURFACE ( 'NONE', #28937, 6.000000000000000888 ) ;
#23127=CARTESIAN_POINT ( 'NONE',  ( 6.350852961086080661, -9.614813431917819062E-14, -147.3750000000000284 ) ) ;
#23129=CARTESIAN_POINT ( 'NONE',  ( 4.763139720814407951, -2.749999999999988454, -141.5000000000000284 ) ) ;
#23131=CARTESIAN_POINT ( 'NONE',  ( 5.412658773652712085, -3.125000000000086153, -158.4330127018922383 ) ) ;
#23133=EDGE_CURVE ( 'NONE', #26392, #25470, #17339, .T. ) ;
#23134=CARTESIAN_POINT ( 'NONE',  ( -3.175426480542816066, -5.500000000000057732, -78.87500000000002842 ) ) ;
#23135=FACE_OUTER_BOUND ( 'NONE', #22901, .T. ) ;
#23136=CARTESIAN_POINT ( 'NONE',  ( -6.350852961085760029, -1.281975124255709124E-13, -70.12500000000005684 ) ) ;
#23137=( BOUNDED_CURVE ( )  B_SPLINE_CURVE ( 2, ( #4486, #5896, #25365, #26935, #8805, #11448, #10390, #10540, #11283 ),
 .UNSPECIFIED., .F., .T. ) 
 B_SPLINE_CURVE_WITH_KNOTS ( ( 3, 2, 2, 2, 3 ),
 ( 0.6583333333333333259, 0.6592592592592592116, 0.6611111111111110938, 0.6629629629629629761, 0.6638888888888889728 ),
 .UNSPECIFIED. ) 
 CURVE ( )  GEOMETRIC_REPRESENTATION_ITEM ( )  RATIONAL_B_SPLINE_CURVE ( ( 0.9330127018922194093, 0.9330127018922194093, 1.000000000000000000, 0.8660254037844388186, 1.000000000000000000, 0.8660254037844388186, 1.000000000000000000, 0.9330127018922154125, 0.9330127018922194093 ) ) 
 REPRESENTATION_ITEM ( '' )  );
#23148=VERTEX_POINT ( 'NONE', #4591 ) ;
#23150=CARTESIAN_POINT ( 'NONE',  ( -5.196152422706573404, -3.000000000000002665, -109.2886751345948397 ) ) ;
#23153=CARTESIAN_POINT ( 'NONE',  ( -5.196152422706573404, -3.000000000000002665, -85.28867513459481131 ) ) ;
#23155=ORIENTED_EDGE ( 'NONE', *, *, #24746, .T. ) ;
#23158=CARTESIAN_POINT ( 'NONE',  ( 0.000000000000000000, 5.499999999999991118, -90.00000000000002842 ) ) ;
#23159=CARTESIAN_POINT ( 'NONE',  ( 7.216878364870455975, -6.409875621278545621E-14, -110.3080127018922099 ) ) ;
#23163=CARTESIAN_POINT ( 'NONE',  ( 5.197562551122876684, -9.697615191485738251, -28.02238803416290480 ) ) ;
#23164=EDGE_LOOP ( 'NONE', ( #22349, #14043, #19370, #5652, #26904 ) ) ;
#23165=FACE_OUTER_BOUND ( 'NONE', #11343, .T. ) ;
#23166=CARTESIAN_POINT ( 'NONE',  ( 4.763139720814407951, 2.750000000000002665, -172.7500000000000284 ) ) ;
#23168=CARTESIAN_POINT ( 'NONE',  ( -6.350852961085760029, -1.281975124255709124E-13, -166.1249999999999716 ) ) ;
#23171=AXIS2_PLACEMENT_3D ( 'NONE', #24600, #3550, #27205 ) ;
#23172=CARTESIAN_POINT ( 'NONE',  ( -4.763139720814407951, 2.749999999999946709, -100.2500000000000000 ) ) ;
#23173=CARTESIAN_POINT ( 'NONE',  ( 0.000000000000000000, -5.999999999999991118, -159.4613248654052029 ) ) ;
#23175=CARTESIAN_POINT ( 'NONE',  ( 3.175426480543072749, 5.499999999999865885, -97.62500000000004263 ) ) ;
#23177=ORIENTED_EDGE ( 'NONE', *, *, #16372, .F. ) ;
#23184=ORIENTED_EDGE ( 'NONE', *, *, #11549, .T. ) ;
#23187=( BOUNDED_CURVE ( )  B_SPLINE_CURVE ( 2, ( #10078, #19450, #5432, #7895, #5886, #15145, #24476, #17308, #2840 ),
 .UNSPECIFIED., .F., .F. ) 
 B_SPLINE_CURVE_WITH_KNOTS ( ( 3, 2, 2, 2, 3 ),
 ( 0.6027777777777777457, 0.6037037037037036313, 0.6055555555555556246, 0.6074074074074073959, 0.6083333333333333925 ),
 .UNSPECIFIED. ) 
 CURVE ( )  GEOMETRIC_REPRESENTATION_ITEM ( )  RATIONAL_B_SPLINE_CURVE ( ( 0.9330127018922194093, 0.9330127018922194093, 1.000000000000000000, 0.8660254037844388186, 1.000000000000000000, 0.8660254037844388186, 1.000000000000000000, 0.9330127018922154125, 0.9330127018922194093 ) ) 
 REPRESENTATION_ITEM ( '' )  );
#23192=CARTESIAN_POINT ( 'NONE',  ( -6.350852961085760029, -1.281975124255709124E-13, -113.6249999999999858 ) ) ;
#23194=CARTESIAN_POINT ( 'NONE',  ( 5.412658773652739619, 3.124999999999988898, -131.1830127018922667 ) ) ;
#23196=CARTESIAN_POINT ( 'NONE',  ( 3.608439182435180470, -6.249999999999997335, -166.6919872981078186 ) ) ;
#23197=CARTESIAN_POINT ( 'NONE',  ( 5.412658773652712085, -3.125000000000086153, -175.5669872981078186 ) ) ;
#23205=CARTESIAN_POINT ( 'NONE',  ( -3.464101615137757051, -5.999999999999979572, -150.5863248654051461 ) ) ;
#23207=CARTESIAN_POINT ( 'NONE',  ( 2.775557561562891351E-14, 6.250000000000033751, -74.56698729810784698 ) ) ;
#23208=CARTESIAN_POINT ( 'NONE',  ( 3.608439182435180470, 6.249999999999982236, -59.69198729810782567 ) ) ;
#23209=CARTESIAN_POINT ( 'NONE',  ( -3.175426480542816510, -5.500000000000057732, -53.37500000000002842 ) ) ;
#23211=EDGE_CURVE ( 'NONE', #24771, #14641, #19503, .T. ) ;
#23213=CARTESIAN_POINT ( 'NONE',  ( -5.196152422706601826, 2.999999999999975131, -159.0386751345948539 ) ) ;
#23214=CARTESIAN_POINT ( 'NONE',  ( 4.763139720814407951, 2.750000000000002665, -120.2500000000000284 ) ) ;
#23216=CARTESIAN_POINT ( 'NONE',  ( 0.000000000000000000, 5.999999999999977796, -154.2113248654052313 ) ) ;
#23220=EDGE_CURVE ( 'NONE', #4196, #14683, #846, .T. ) ;
#23226=CARTESIAN_POINT ( 'NONE',  ( 3.608439182435180470, 6.249999999999982236, -110.6919872981078043 ) ) ;
#23227=CARTESIAN_POINT ( 'NONE',  ( 3.464101615137852974, 5.999999999999884537, -108.4136751345947971 ) ) ;
#23228=( BOUNDED_CURVE ( )  B_SPLINE_CURVE ( 2, ( #10550, #1150, #15337, #27108, #10401, #13337, #22679, #24814, #20231 ),
 .UNSPECIFIED., .F., .T. ) 
 B_SPLINE_CURVE_WITH_KNOTS ( ( 3, 2, 2, 2, 3 ),
 ( 0.05277777777777778456, 0.05370370370370370489, 0.05555555555555555247, 0.05740740740740740700, 0.05833333333333332732 ),
 .UNSPECIFIED. ) 
 CURVE ( )  GEOMETRIC_REPRESENTATION_ITEM ( )  RATIONAL_B_SPLINE_CURVE ( ( 0.9330127018922194093, 0.9330127018922198534, 1.000000000000000000, 0.8660254037844388186, 1.000000000000000000, 0.8660254037844388186, 1.000000000000000000, 0.9330127018922199644, 0.9330127018922194093 ) ) 
 REPRESENTATION_ITEM ( '' )  );
#23232=VERTEX_POINT ( 'NONE', #24082 ) ;
#23235=( BOUNDED_CURVE ( )  B_SPLINE_CURVE ( 2, ( #25812, #9078, #2609, #23227, #16039, #21366, #18325, #11422, #27639 ),
 .UNSPECIFIED., .F., .F. ) 
 B_SPLINE_CURVE_WITH_KNOTS ( ( 3, 2, 2, 2, 3 ),
 ( 0.5416666666666667407, 0.5425925925925926263, 0.5444444444444443976, 0.5462962962962962798, 0.5472222222222221655 ),
 .UNSPECIFIED. ) 
 CURVE ( )  GEOMETRIC_REPRESENTATION_ITEM ( )  RATIONAL_B_SPLINE_CURVE ( ( 0.9330127018922194093, 0.9330127018922234061, 1.000000000000000000, 0.8660254037844388186, 1.000000000000000000, 0.8660254037844388186, 1.000000000000000000, 0.9330127018922234061, 0.9330127018922194093 ) ) 
 REPRESENTATION_ITEM ( '' )  );
#23236=CARTESIAN_POINT ( 'NONE',  ( -3.608439182435052128, -6.250000000000110134, -138.4419872981078186 ) ) ;
#23238=CARTESIAN_POINT ( 'NONE',  ( -5.999999999999963585, 1.780251999655701777E-13, -93.83632486540518869 ) ) ;
#23240=CYLINDRICAL_SURFACE ( 'NONE', #29889, 6.000000000000000888 ) ;
#23241=CARTESIAN_POINT ( 'NONE',  ( -5.412658773652684552, -3.125000000000099920, -67.43301270189222407 ) ) ;
#23245=CARTESIAN_POINT ( 'NONE',  ( 0.000000000000000000, 5.999999999999977796, -73.78867513459485394 ) ) ;
#23249=DIRECTION ( 'NONE',  ( -7.147005652999508048E-36, 5.642372883946980038E-36, 1.000000000000000000 ) ) ;
#23251=ADVANCED_FACE ( 'NONE', ( #25937 ), #5328, .T. ) ;
#23252=CARTESIAN_POINT ( 'NONE',  ( -5.999999999999963585, 1.780251999655701777E-13, -95.33632486540520290 ) ) ;
#23253=ADVANCED_FACE ( 'NONE', ( #740 ), #8540, .T. ) ;
#23254=CARTESIAN_POINT ( 'NONE',  ( -2.775557561562891351E-14, -5.500000000000115463, -120.7500000000000284 ) ) ;
#23256=CARTESIAN_POINT ( 'NONE',  ( 3.608439182435180470, 6.249999999999982236, -144.5580127018922383 ) ) ;
#23258=ORIENTED_EDGE ( 'NONE', *, *, #15356, .T. ) ;
#23259=CARTESIAN_POINT ( 'NONE',  ( -2.775557561562891351E-14, -5.500000000000115463, -57.75000000000002132 ) ) ;
#23264=CARTESIAN_POINT ( 'NONE',  ( -5.412658773652739619, 3.124999999999975131, -104.3169872981078470 ) ) ;
#23267=CARTESIAN_POINT ( 'NONE',  ( 6.000000000000000888, -1.859271017917181981E-14, -84.08632486540520290 ) ) ;
#23269=CARTESIAN_POINT ( 'NONE',  ( 4.763139720814407951, -2.749999999999988454, -140.0000000000000000 ) ) ;
#23272=ORIENTED_EDGE ( 'NONE', *, *, #20991, .T. ) ;
#23274=CARTESIAN_POINT ( 'NONE',  ( 3.175426480543072749, 5.499999999999865885, -63.12500000000001421 ) ) ;
#23276=CARTESIAN_POINT ( 'NONE',  ( -5.999999999999919176, 1.607695154586804565, -93.90331216351297883 ) ) ;
#23277=ORIENTED_EDGE ( 'NONE', *, *, #17077, .T. ) ;
#23281=( BOUNDED_CURVE ( )  B_SPLINE_CURVE ( 2, ( #4024, #27515, #20798, #20475, #1577, #8491, #25372, #6493, #13757 ),
 .UNSPECIFIED., .F., .T. ) 
 B_SPLINE_CURVE_WITH_KNOTS ( ( 3, 2, 2, 2, 3 ),
 ( 0.2249999999999999778, 0.2259259259259259744, 0.2277777777777777457, 0.2296296296296296280, 0.2305555555555556246 ),
 .UNSPECIFIED. ) 
 CURVE ( )  GEOMETRIC_REPRESENTATION_ITEM ( )  RATIONAL_B_SPLINE_CURVE ( ( 0.9330127018922194093, 0.9330127018922154125, 1.000000000000000000, 0.8660254037844388186, 1.000000000000000000, 0.8660254037844388186, 1.000000000000000000, 0.9330127018922154125, 0.9330127018922194093 ) ) 
 REPRESENTATION_ITEM ( '' )  );
#23282=EDGE_CURVE ( 'NONE', #17182, #9697, #3987, .T. ) ;
#23283=CYLINDRICAL_SURFACE ( 'NONE', #28470, 6.000000000000000888 ) ;
#23286=CARTESIAN_POINT ( 'NONE',  ( 4.763139720814407951, 2.750000000000002665, -144.2500000000000000 ) ) ;
#23288=CARTESIAN_POINT ( 'NONE',  ( -3.175426480542816510, 5.499999999999865885, -136.3750000000000568 ) ) ;
#23289=CARTESIAN_POINT ( 'NONE',  ( 2.775557561562891351E-14, -6.250000000000061284, -157.1830127018922667 ) ) ;
#23290=CARTESIAN_POINT ( 'NONE',  ( 6.000000000000000888, 7.762456499804234384E-14, -117.0863248654052171 ) ) ;
#23291=CARTESIAN_POINT ( 'NONE',  ( 3.175426480543072749, 5.499999999999865885, -81.12500000000002842 ) ) ;
#23293=CARTESIAN_POINT ( 'NONE',  ( 3.175426480543072749, 5.499999999999865885, -75.12500000000001421 ) ) ;
#23294=CARTESIAN_POINT ( 'NONE',  ( -5.999999999999963585, -1.487416814333745711E-14, -76.41367513459481131 ) ) ;
#23302=CARTESIAN_POINT ( 'NONE',  ( -3.464101615137725076, 5.999999999999979572, -139.0863248654051745 ) ) ;
#23303=ORIENTED_EDGE ( 'NONE', *, *, #8147, .F. ) ;
#23307=CARTESIAN_POINT ( 'NONE',  ( 3.175426480543072749, 5.499999999999865885, -153.1250000000000284 ) ) ;
#23309=ORIENTED_EDGE ( 'NONE', *, *, #24446, .T. ) ;
#23310=EDGE_CURVE ( 'NONE', #27987, #28056, #24178, .T. ) ;
#23311=CARTESIAN_POINT ( 'NONE',  ( -4.763139720814407951, 2.749999999999946709, -89.75000000000000000 ) ) ;
#23312=AXIS2_PLACEMENT_3D ( 'NONE', #22299, #5999, #29499 ) ;
#23313=CARTESIAN_POINT ( 'NONE',  ( -3.608439182435052128, -6.250000000000110134, -109.3080127018922809 ) ) ;
#23316=CARTESIAN_POINT ( 'NONE',  ( 5.999486246981976301, -9.219878802943842544, -25.40874315777524828 ) ) ;
#23317=ORIENTED_EDGE ( 'NONE', *, *, #10694, .F. ) ;
#23318=( BOUNDED_CURVE ( )  B_SPLINE_CURVE ( 2, ( #15205, #24237, #26539, #29444, #13075, #22408, #1345, #8419, #10756 ),
 .UNSPECIFIED., .F., .T. ) 
 B_SPLINE_CURVE_WITH_KNOTS ( ( 3, 2, 2, 2, 3 ),
 ( 0.3249999999999999556, 0.3259259259259259522, 0.3277777777777777235, 0.3296296296296296058, 0.3305555555555556024 ),
 .UNSPECIFIED. ) 
 CURVE ( )  GEOMETRIC_REPRESENTATION_ITEM ( )  RATIONAL_B_SPLINE_CURVE ( ( 0.9330127018922194093, 0.9330127018922154125, 1.000000000000000000, 0.8660254037844388186, 1.000000000000000000, 0.8660254037844388186, 1.000000000000000000, 0.9330127018922154125, 0.9330127018922194093 ) ) 
 REPRESENTATION_ITEM ( '' )  );
#23319=EDGE_CURVE ( 'NONE', #6844, #19684, #25274, .T. ) ;
#23320=CARTESIAN_POINT ( 'NONE',  ( -4.763139720814407951, 2.749999999999946709, -170.7500000000000000 ) ) ;
#23321=CARTESIAN_POINT ( 'NONE',  ( -3.464101615137757051, -5.999999999999979572, -80.66367513459479710 ) ) ;
#23322=CARTESIAN_POINT ( 'NONE',  ( -6.350852961085760029, -1.281975124255709124E-13, -157.1250000000000284 ) ) ;
#23324=CARTESIAN_POINT ( 'NONE',  ( 3.175426480543072749, 5.499999999999865885, -99.12500000000005684 ) ) ;
#23327=CARTESIAN_POINT ( 'NONE',  ( 4.763139720814407951, 2.750000000000002665, -96.25000000000000000 ) ) ;
#23330=CARTESIAN_POINT ( 'NONE',  ( -6.000000000000000888, 1.067854986875958443E-15, 7.560779664488942560E-35 ) ) ;
#23334=CARTESIAN_POINT ( 'NONE',  ( -5.999999999999968026, -1.607695154586722186, -161.8466878364870354 ) ) ;
#23336=CARTESIAN_POINT ( 'NONE',  ( 5.196152422706629359, -2.999999999999988898, -85.71132486540523132 ) ) ;
#23337=EDGE_LOOP ( 'NONE', ( #14211, #22389, #8736, #9430 ) ) ;
#23338=VECTOR ( 'NONE', #8470, 1000.000000000000000 ) ;
#23340=CARTESIAN_POINT ( 'NONE',  ( 3.464101615137757051, -5.999999999999979572, -169.8363248654052029 ) ) ;
#23342=DIRECTION ( 'NONE',  ( -7.147005652999508048E-36, 5.642372883946980038E-36, 1.000000000000000000 ) ) ;
#23344=DIRECTION ( 'NONE',  ( -7.147005652999508048E-36, 5.642372883946980038E-36, 1.000000000000000000 ) ) ;
#23347=ORIENTED_EDGE ( 'NONE', *, *, #1434, .F. ) ;
#23350=CARTESIAN_POINT ( 'NONE',  ( 0.000000000000000000, 5.499999999999991118, -112.5000000000000426 ) ) ;
#23352=CARTESIAN_POINT ( 'NONE',  ( -5.412658773652684552, -3.125000000000099920, -128.9330127018922383 ) ) ;
#23353=EDGE_LOOP ( 'NONE', ( #30194, #3497 ) ) ;
#23355=CARTESIAN_POINT ( 'NONE',  ( 7.216878364870455975, -6.409875621278545621E-14, -170.9419872981078470 ) ) ;
#23357=ADVANCED_FACE ( 'NONE', ( #14989 ), #19595, .T. ) ;
#23359=DIRECTION ( 'NONE',  ( -7.147005652999508048E-36, 5.642372883946980038E-36, 1.000000000000000000 ) ) ;
#23362=CARTESIAN_POINT ( 'NONE',  ( -5.412658773652739619, 3.124999999999975131, -177.1830127018922383 ) ) ;
#23366=CARTESIAN_POINT ( 'NONE',  ( 4.763139720814407951, -2.749999999999988454, -125.0000000000000000 ) ) ;
#23368=CARTESIAN_POINT ( 'NONE',  ( 5.999999999999999112, 2.951592740943527306E-14, -154.5863248654052029 ) ) ;
#23369=VERTEX_POINT ( 'NONE', #241 ) ;
#23372=CARTESIAN_POINT ( 'NONE',  ( 6.000000000000000888, 1.743066579297358182E-13, -83.16367513459481131 ) ) ;
#23373=VERTEX_POINT ( 'NONE', #28778 ) ;
#23377=CARTESIAN_POINT ( 'NONE',  ( 2.775557561562891351E-14, 6.250000000000033751, -109.0669872981078186 ) ) ;
#23379=FACE_OUTER_BOUND ( 'NONE', #24136, .T. ) ;
#23380=EDGE_LOOP ( 'NONE', ( #29617, #28140, #12477, #8860 ) ) ;
#23385=CARTESIAN_POINT ( 'NONE',  ( 2.775557561562891351E-14, -6.250000000000061284, -138.3169872981078186 ) ) ;
#23389=CARTESIAN_POINT ( 'NONE',  ( 6.000000000000000888, -1.859271017917181981E-14, -171.0863248654052029 ) ) ;
#23391=CARTESIAN_POINT ( 'NONE',  ( -5.412658773652739619, 3.124999999999975131, -61.68301270189224539 ) ) ;
#23392=EDGE_CURVE ( 'NONE', #11534, #17549, #27305, .T. ) ;
#23395=CARTESIAN_POINT ( 'NONE',  ( 0.000000000000000000, -5.999999999999991118, -160.9613248654052597 ) ) ;
#23396=CARTESIAN_POINT ( 'NONE',  ( -3.464101615137757051, -5.999999999999979572, -146.6636751345948255 ) ) ;
#23399=CARTESIAN_POINT ( 'NONE',  ( -5.999999999999963585, 8.134310703387671600E-14, -114.8363248654052171 ) ) ;
#23403=ORIENTED_EDGE ( 'NONE', *, *, #12845, .F. ) ;
#23405=CARTESIAN_POINT ( 'NONE',  ( -6.350852961085760029, -1.281975124255709124E-13, -56.62500000000003553 ) ) ;
#23406=FACE_OUTER_BOUND ( 'NONE', #20115, .T. ) ;
#23407=CARTESIAN_POINT ( 'NONE',  ( 5.196152422706629359, 3.000000000000002665, -62.96132486540523132 ) ) ;
#23409=ORIENTED_EDGE ( 'NONE', *, *, #2385, .T. ) ;
#23412=CARTESIAN_POINT ( 'NONE',  ( -3.608439182435052128, -6.250000000000110134, -105.4419872981078612 ) ) ;
#23413=CARTESIAN_POINT ( 'NONE',  ( -5.999999999999963585, -1.487416814333745711E-14, -153.8363248654052313 ) ) ;
#23414=( BOUNDED_CURVE ( )  B_SPLINE_CURVE ( 2, ( #19510, #21957, #10286, #28841, #890, #28991, #16778, #14476, #2748 ),
 .UNSPECIFIED., .F., .T. ) 
 B_SPLINE_CURVE_WITH_KNOTS ( ( 3, 2, 2, 2, 3 ),
 ( 0.2972222222222222765, 0.2981481481481481621, 0.3000000000000000444, 0.3018518518518518157, 0.3027777777777777013 ),
 .UNSPECIFIED. ) 
 CURVE ( )  GEOMETRIC_REPRESENTATION_ITEM ( )  RATIONAL_B_SPLINE_CURVE ( ( 0.9330127018922194093, 0.9330127018922234061, 1.000000000000000000, 0.8660254037844388186, 1.000000000000000000, 0.8660254037844388186, 1.000000000000000000, 0.9330127018922234061, 0.9330127018922194093 ) ) 
 REPRESENTATION_ITEM ( '' )  );
#23417=VERTEX_POINT ( 'NONE', #9778 ) ;
#23418=ADVANCED_FACE ( 'NONE', ( #19155 ), #5287, .T. ) ;
#23419=CARTESIAN_POINT ( 'NONE',  ( -4.763139720814407951, -2.750000000000016431, -134.5000000000000000 ) ) ;
#23420=ORIENTED_EDGE ( 'NONE', *, *, #2385, .F. ) ;
#23421=ORIENTED_EDGE ( 'NONE', *, *, #19695, .F. ) ;
#23422=CARTESIAN_POINT ( 'NONE',  ( 3.175426480543072749, 5.499999999999865885, -61.62500000000000000 ) ) ;
#23423=CARTESIAN_POINT ( 'NONE',  ( 3.464101615137757051, -5.999999999999979572, -164.4136751345947971 ) ) ;
#23426=CARTESIAN_POINT ( 'NONE',  ( 2.775557561562891351E-14, 6.250000000000033751, -81.43301270189223828 ) ) ;
#23427=CARTESIAN_POINT ( 'NONE',  ( 3.464101615137852974, 5.999999999999884537, -139.9136751345948255 ) ) ;
#23429=CYLINDRICAL_SURFACE ( 'NONE', #16621, 6.000000000000000888 ) ;
#23432=CARTESIAN_POINT ( 'NONE',  ( 6.350852961086080661, -9.614813431917819062E-14, -148.8750000000000284 ) ) ;
#23435=CARTESIAN_POINT ( 'NONE',  ( -2.775557561562891351E-14, -5.500000000000115463, -134.2500000000000284 ) ) ;
#23436=CARTESIAN_POINT ( 'NONE',  ( 7.216878364870455975, -6.409875621278545621E-14, -161.3080127018922667 ) ) ;
#23437=CARTESIAN_POINT ( 'NONE',  ( 0.000000000000000000, 0.000000000000000000, 0.000000000000000000 ) ) ;
#23438=CARTESIAN_POINT ( 'NONE',  ( 4.763139720814407951, 2.750000000000002665, -75.25000000000004263 ) ) ;
#23441=CARTESIAN_POINT ( 'NONE',  ( -2.775557561562891351E-14, -5.500000000000115463, -65.25000000000002842 ) ) ;
#23442=CARTESIAN_POINT ( 'NONE',  ( 5.196152422706629359, 3.000000000000002665, -155.0386751345948539 ) ) ;
#23447=VECTOR ( 'NONE', #13700, 1000.000000000000000 ) ;
#23448=DIRECTION ( 'NONE',  ( -7.147005652999508048E-36, 5.642372883946980038E-36, 1.000000000000000000 ) ) ;
#23453=CARTESIAN_POINT ( 'NONE',  ( 5.999999999999999112, 2.951592740943527306E-14, -156.6636751345948255 ) ) ;
#23455=( BOUNDED_CURVE ( )  B_SPLINE_CURVE ( 2, ( #26809, #10271, #19092, #29274, #15357, #28415, #27127, #24520, #13057 ),
 .UNSPECIFIED., .F., .F. ) 
 B_SPLINE_CURVE_WITH_KNOTS ( ( 3, 2, 2, 2, 3 ),
 ( 0.4583333333333333148, 0.4592592592592592560, 0.4611111111111111382, 0.4629629629629629650, 0.4638888888888889062 ),
 .UNSPECIFIED. ) 
 CURVE ( )  GEOMETRIC_REPRESENTATION_ITEM ( )  RATIONAL_B_SPLINE_CURVE ( ( 0.9330127018922194093, 0.9330127018922174109, 1.000000000000000000, 0.8660254037844388186, 1.000000000000000000, 0.8660254037844388186, 1.000000000000000000, 0.9330127018922174109, 0.9330127018922194093 ) ) 
 REPRESENTATION_ITEM ( '' )  );
#23456=ADVANCED_FACE ( 'NONE', ( #29391 ), #22352, .T. ) ;
#23457=CARTESIAN_POINT ( 'NONE',  ( 6.000000000000000888, -1.607695154586752384, -84.73066243270260145 ) ) ;
#23459=VERTEX_POINT ( 'NONE', #29703 ) ;
#23462=CARTESIAN_POINT ( 'NONE',  ( -3.175426480542816510, 5.499999999999865885, -91.37500000000001421 ) ) ;
#23463=VECTOR ( 'NONE', #7119, 1000.000000000000000 ) ;
#23465=CARTESIAN_POINT ( 'NONE',  ( -3.608439182435115633, 6.249999999999965361, -108.3080127018922667 ) ) ;
#23466=CARTESIAN_POINT ( 'NONE',  ( 3.031145847945201588, 10.57562584360013780, -30.18173774084347727 ) ) ;
#23468=CARTESIAN_POINT ( 'NONE',  ( -4.763139720814407951, 2.749999999999946709, -163.2500000000000000 ) ) ;
#23469=CARTESIAN_POINT ( 'NONE',  ( -7.216878364870328078, 0.000000000000000000, -48.05801270189223118 ) ) ;
#23471=FILL_AREA_STYLE_COLOUR ( '', #27580 ) ;
#23472=CARTESIAN_POINT ( 'NONE',  ( 4.763139720814407951, -2.749999999999988454, -170.0000000000000284 ) ) ;
#23475=CARTESIAN_POINT ( 'NONE',  ( 4.763139720814407951, -2.749999999999988454, -155.0000000000000284 ) ) ;
#23477=CARTESIAN_POINT ( 'NONE',  ( -4.763139720814407951, 2.749999999999946709, -98.75000000000000000 ) ) ;
#23479=CARTESIAN_POINT ( 'NONE',  ( 0.000000000000000000, 5.999999999999977796, 0.000000000000000000 ) ) ;
#23480=CARTESIAN_POINT ( 'NONE',  ( 3.175426480543072749, -5.500000000000105693, -87.62500000000000000 ) ) ;
#23487=CARTESIAN_POINT ( 'NONE',  ( -5.196152422706573404, -3.000000000000002665, -86.21132486540523132 ) ) ;
#23489=CYLINDRICAL_SURFACE ( 'NONE', #6436, 6.000000000000000888 ) ;
#23491=ORIENTED_EDGE ( 'NONE', *, *, #25251, .F. ) ;
#23492=EDGE_CURVE ( 'NONE', #3683, #14517, #1132, .T. ) ;
#23495=CARTESIAN_POINT ( 'NONE',  ( -4.763139720814407951, -2.750000000000016431, -113.5000000000000426 ) ) ;
#23497=( BOUNDED_CURVE ( )  B_SPLINE_CURVE ( 2, ( #24885, #19687, #17400, #26576, #15413, #15087, #22141, #21989, #26715 ),
 .UNSPECIFIED., .F., .F. ) 
 B_SPLINE_CURVE_WITH_KNOTS ( ( 3, 2, 2, 2, 3 ),
 ( 0.1583333333333333259, 0.1592592592592592671, 0.1611111111111111216, 0.1629629629629629761, 0.1638888888888888895 ),
 .UNSPECIFIED. ) 
 CURVE ( )  GEOMETRIC_REPRESENTATION_ITEM ( )  RATIONAL_B_SPLINE_CURVE ( ( 0.9330127018922196314, 0.9330127018922185211, 1.000000000000000000, 0.8660254037844388186, 1.000000000000000000, 0.8660254037844388186, 1.000000000000000000, 0.9330127018922194093, 0.9330127018922194093 ) ) 
 REPRESENTATION_ITEM ( '' )  );
#23498=CARTESIAN_POINT ( 'NONE',  ( 2.775557561562891351E-14, 6.250000000000033751, -133.9330127018922383 ) ) ;
#23499=ORIENTED_EDGE ( 'NONE', *, *, #19209, .T. ) ;
#23501=CARTESIAN_POINT ( 'NONE',  ( -3.608439182435052128, -6.250000000000110134, -171.4419872981078470 ) ) ;
#23503=ORIENTED_EDGE ( 'NONE', *, *, #2815, .T. ) ;
#23506=CARTESIAN_POINT ( 'NONE',  ( 0.000000000000000000, 5.999999999999977796, -95.71132486540523132 ) ) ;
#23507=CARTESIAN_POINT ( 'NONE',  ( 6.000000000000000888, -1.859271017917181981E-14, -137.1636751345948255 ) ) ;
#23508=CARTESIAN_POINT ( 'NONE',  ( 4.763139720814407951, -2.749999999999988454, -177.5000000000000000 ) ) ;
#23510=CARTESIAN_POINT ( 'NONE',  ( -3.608439182435115633, 6.249999999999965361, -174.3080127018922667 ) ) ;
#23513=CARTESIAN_POINT ( 'NONE',  ( 5.196152422706629359, 3.000000000000002665, -123.5386751345948255 ) ) ;
#23514=CARTESIAN_POINT ( 'NONE',  ( 3.175426480543072749, 5.499999999999865885, -123.1250000000000426 ) ) ;
#23527=DIRECTION ( 'NONE',  ( -7.147005652999508048E-36, 5.642372883946980038E-36, 1.000000000000000000 ) ) ;
#23529=ORIENTED_EDGE ( 'NONE', *, *, #17395, .F. ) ;
#23533=CARTESIAN_POINT ( 'NONE',  ( 3.608439182435180470, -6.249999999999997335, -138.1919872981077901 ) ) ;
#23534=LINE ( 'NONE', #9550, #27951 ) ;
#23538=CARTESIAN_POINT ( 'NONE',  ( -6.000000000000007105, -1.607695154586655129, -171.7693375672974128 ) ) ;
#23541=CARTESIAN_POINT ( 'NONE',  ( 6.000000000000000888, -1.859271017917181981E-14, -124.5863248654052171 ) ) ;
#23543=CARTESIAN_POINT ( 'NONE',  ( 5.196152422706629359, -2.999999999999988898, -139.7113248654052313 ) ) ;
#23545=FILL_AREA_STYLE ('',( #14355 ) ) ;
#23551=VERTEX_POINT ( 'NONE', #8674 ) ;
#23553=CARTESIAN_POINT ( 'NONE',  ( -2.775557561562891351E-14, -5.500000000000115463, -54.75000000000002132 ) ) ;
#23557=CARTESIAN_POINT ( 'NONE',  ( 3.608439182435180470, -6.249999999999997335, -102.1919872981078328 ) ) ;
#23558=DIRECTION ( 'NONE',  ( -7.147005652999508048E-36, 5.642372883946980038E-36, 1.000000000000000000 ) ) ;
#23563=CARTESIAN_POINT ( 'NONE',  ( 3.175426480543072749, 5.499999999999865885, -133.6250000000000284 ) ) ;
#23564=AXIS2_PLACEMENT_3D ( 'NONE', #17311, #29390, #3281 ) ;
#23566=ORIENTED_EDGE ( 'NONE', *, *, #10585, .F. ) ;
#23567=CARTESIAN_POINT ( 'NONE',  ( -3.464101615137725076, 5.999999999999979572, -163.0863248654051745 ) ) ;
#23568=CARTESIAN_POINT ( 'NONE',  ( 4.763139720814407951, 2.750000000000002665, -64.75000000000002842 ) ) ;
#23569=DIRECTION ( 'NONE',  ( -7.147005652999508048E-36, 5.642372883946980038E-36, 1.000000000000000000 ) ) ;
#23571=CARTESIAN_POINT ( 'NONE',  ( 3.608439182435180470, -6.249999999999997335, -80.55801270189219565 ) ) ;
#23574=CARTESIAN_POINT ( 'NONE',  ( 6.000000000000000888, -6.507448562710137091E-15, -175.5863248654052029 ) ) ;
#23577=CARTESIAN_POINT ( 'NONE',  ( -6.350852961085760029, -1.281975124255709124E-13, -148.1250000000000284 ) ) ;
#23578=CARTESIAN_POINT ( 'NONE',  ( 6.000000000000000888, -1.859271017917181981E-14, -105.0863248654052313 ) ) ;
#23579=CARTESIAN_POINT ( 'NONE',  ( -3.608439182435115633, 6.249999999999965361, -160.8080127018922667 ) ) ;
#23580=CARTESIAN_POINT ( 'NONE',  ( -5.999999999999904965, -1.607695154586834541, -149.2693375672974128 ) ) ;
#23582=CARTESIAN_POINT ( 'NONE',  ( 6.350852961086080661, -9.614813431917819062E-14, -78.37500000000001421 ) ) ;
#23583=CARTESIAN_POINT ( 'NONE',  ( 6.000000000000000888, 7.762456499804234384E-14, -132.6636751345948539 ) ) ;
#23584=CARTESIAN_POINT ( 'NONE',  ( 3.175426480543072749, -5.500000000000105693, -65.12500000000001421 ) ) ;
#23588=CARTESIAN_POINT ( 'NONE',  ( 6.000000000000000000, 2.951592740943527306E-14, -148.5863248654052313 ) ) ;
#23595=ADVANCED_FACE ( 'NONE', ( #27088 ), #26927, .T. ) ;
#23596=LINE ( 'NONE', #2533, #19438 ) ;
#23597=ORIENTED_EDGE ( 'NONE', *, *, #15662, .F. ) ;
#23604=CARTESIAN_POINT ( 'NONE',  ( 5.412658773652712085, -3.125000000000086153, -154.5669872981078186 ) ) ;
#23605=EDGE_LOOP ( 'NONE', ( #18135, #27445, #21294, #19616 ) ) ;
#23606=CARTESIAN_POINT ( 'NONE',  ( 3.175426480543072749, 5.499999999999865885, -85.62500000000000000 ) ) ;
#23609=CARTESIAN_POINT ( 'NONE',  ( 3.608439182435180470, -6.249999999999997335, -101.5580127018922383 ) ) ;
#23611=VECTOR ( 'NONE', #22209, 1000.000000000000000 ) ;
#23614=CARTESIAN_POINT ( 'NONE',  ( -3.608439182435115633, 6.249999999999965361, -48.30801270189223828 ) ) ;
#23616=CARTESIAN_POINT ( 'NONE',  ( 6.350852961086080661, -9.614813431917819062E-14, -171.3750000000000000 ) ) ;
#23617=CARTESIAN_POINT ( 'NONE',  ( 5.196152422706629359, 3.000000000000002665, -161.9613248654052597 ) ) ;
#23618=CARTESIAN_POINT ( 'NONE',  ( -4.763139720814407951, 2.749999999999946709, -157.2500000000000000 ) ) ;
#23620=EDGE_CURVE ( 'NONE', #6372, #12915, #1022, .T. ) ;
#23621=CARTESIAN_POINT ( 'NONE',  ( 3.175426480543072749, 5.499999999999865885, -105.1250000000000284 ) ) ;
#23623=ADVANCED_FACE ( 'NONE', ( #22810 ), #4659, .T. ) ;
#23624=CARTESIAN_POINT ( 'NONE',  ( -3.175426480542816510, -5.500000000000057732, -156.8750000000000284 ) ) ;
#23625=CARTESIAN_POINT ( 'NONE',  ( 4.763139720814407951, 2.750000000000002665, -88.75000000000000000 ) ) ;
#23629=ORIENTED_EDGE ( 'NONE', *, *, #23986, .F. ) ;
#23635=CARTESIAN_POINT ( 'NONE',  ( 0.000000000000000000, 0.000000000000000000, 0.000000000000000000 ) ) ;
#23640=CARTESIAN_POINT ( 'NONE',  ( 5.196152422706629359, -2.999999999999988898, -52.71132486540519579 ) ) ;
#23641=AXIS2_PLACEMENT_3D ( 'NONE', #25032, #8775, #4304 ) ;
#23644=CARTESIAN_POINT ( 'NONE',  ( -2.775557561562891351E-14, -5.500000000000115463, -111.7500000000000142 ) ) ;
#23646=CARTESIAN_POINT ( 'NONE',  ( -5.412658773652739619, 3.124999999999975131, -121.6830127018922525 ) ) ;
#23648=CARTESIAN_POINT ( 'NONE',  ( -5.999999999999963585, 1.780251999655701777E-13, -56.91367513459483973 ) ) ;
#23649=CARTESIAN_POINT ( 'NONE',  ( -5.412658773652739619, 3.124999999999975131, -170.3169872981078470 ) ) ;
#23653=ORIENTED_EDGE ( 'NONE', *, *, #19259, .T. ) ;
#23655=CARTESIAN_POINT ( 'NONE',  ( -3.175426480542816510, 5.499999999999865885, -176.8750000000000568 ) ) ;
#23657=CARTESIAN_POINT ( 'NONE',  ( 5.412658773652712085, -3.125000000000086153, -174.9330127018922099 ) ) ;
#23662=CARTESIAN_POINT ( 'NONE',  ( 4.763139720814407951, 2.750000000000002665, -115.7500000000000142 ) ) ;
#23663=ORIENTED_EDGE ( 'NONE', *, *, #26401, .T. ) ;
#23665=VECTOR ( 'NONE', #5893, 1000.000000000000000 ) ;
#23667=CARTESIAN_POINT ( 'NONE',  ( 6.000000000000000888, -3.330669073875464691E-16, -7.560779664488942560E-35 ) ) ;
#23668=CARTESIAN_POINT ( 'NONE',  ( -5.999999999999963585, 8.134310703387671600E-14, -131.3363248654052313 ) ) ;
#23669=VERTEX_POINT ( 'NONE', #13468 ) ;
#23671=CARTESIAN_POINT ( 'NONE',  ( -6.350852961085760029, -1.281975124255709124E-13, -178.1250000000000284 ) ) ;
#23678=CARTESIAN_POINT ( 'NONE',  ( 6.000000000000000888, -1.859271017917181981E-14, -141.6636751345948255 ) ) ;
#23680=CARTESIAN_POINT ( 'NONE',  ( -5.412658773652684552, -3.125000000000099920, -138.5669872981077901 ) ) ;
#23684=CARTESIAN_POINT ( 'NONE',  ( 5.196152422706629359, 3.000000000000002665, -129.5386751345948255 ) ) ;
#23686=CYLINDRICAL_SURFACE ( 'NONE', #21585, 6.000000000000000888 ) ;
#23688=CYLINDRICAL_SURFACE ( 'NONE', #26468, 6.000000000000000888 ) ;
#23690=CARTESIAN_POINT ( 'NONE',  ( 5.196152422706629359, 3.000000000000002665, -99.53867513459479710 ) ) ;
#23692=CARTESIAN_POINT ( 'NONE',  ( 6.000000000000000888, -1.859271017917181981E-14, -147.0863248654052313 ) ) ;
#23694=CARTESIAN_POINT ( 'NONE',  ( -5.999999999999963585, 1.780251999655701777E-13, -69.83632486540523132 ) ) ;
#23696=DIRECTION ( 'NONE',  ( -7.147005652999508048E-36, 5.642372883946980038E-36, 1.000000000000000000 ) ) ;
#23701=CARTESIAN_POINT ( 'NONE',  ( 0.000000000000000000, 5.499999999999991118, -46.49999999999998579 ) ) ;
#23707=CARTESIAN_POINT ( 'NONE',  ( -7.216878364870328078, 0.000000000000000000, -104.1919872981078470 ) ) ;
#23710=CARTESIAN_POINT ( 'NONE',  ( -3.175426480542816510, -5.500000000000057732, -126.8749999999999858 ) ) ;
#23714=CARTESIAN_POINT ( 'NONE',  ( -4.763139720814407951, -2.750000000000016431, -59.50000000000000000 ) ) ;
#23716=CARTESIAN_POINT ( 'NONE',  ( 0.000000000000000000, 0.000000000000000000, 0.000000000000000000 ) ) ;
#23718=CARTESIAN_POINT ( 'NONE',  ( 7.216878364870455975, -6.409875621278545621E-14, -83.30801270189226670 ) ) ;
#23726=CARTESIAN_POINT ( 'NONE',  ( -4.763139720814407951, -2.750000000000016431, -140.5000000000000000 ) ) ;
#23728=CARTESIAN_POINT ( 'NONE',  ( -5.412658773652684552, -3.125000000000099920, -152.9330127018922383 ) ) ;
#23729=CARTESIAN_POINT ( 'NONE',  ( 2.570750408560660700E-15, 10.49588505988223375, 2.088097429759527849E-50 ) ) ;
#23730=CARTESIAN_POINT ( 'NONE',  ( -3.464101615137757051, -5.999999999999979572, -73.16367513459482552 ) ) ;
#23731=CARTESIAN_POINT ( 'NONE',  ( -3.175426480542816066, -5.500000000000057732, -71.37499999999998579 ) ) ;
#23732=CARTESIAN_POINT ( 'NONE',  ( -5.999999999999963585, -1.487416814333745711E-14, -113.9136751345948255 ) ) ;
#23734=CARTESIAN_POINT ( 'NONE',  ( 4.763139720814407951, -2.749999999999988454, -65.00000000000000000 ) ) ;
#23736=CARTESIAN_POINT ( 'NONE',  ( 6.000000000000000888, 7.762456499804234384E-14, -144.0863248654052313 ) ) ;
#23744=CARTESIAN_POINT ( 'NONE',  ( -5.196152422706573404, -3.000000000000002665, -145.2886751345948255 ) ) ;
#23745=ORIENTED_EDGE ( 'NONE', *, *, #2849, .F. ) ;
#23747=CARTESIAN_POINT ( 'NONE',  ( -5.999999999999919176, 1.607695154586804565, -63.90331216351301435 ) ) ;
#23748=CARTESIAN_POINT ( 'NONE',  ( -2.775557561562891351E-14, -5.500000000000115463, -180.7500000000000284 ) ) ;
#23751=EDGE_CURVE ( 'NONE', #26686, #24771, #8650, .T. ) ;
#23752=CARTESIAN_POINT ( 'NONE',  ( 3.175426480543072749, 5.499999999999865885, -87.12500000000000000 ) ) ;
#23753=( BOUNDED_CURVE ( )  B_SPLINE_CURVE ( 2, ( #4354, #9129, #13467, #6512, #18521, #20497, #11004, #8832, #15784 ),
 .UNSPECIFIED., .F., .T. ) 
 B_SPLINE_CURVE_WITH_KNOTS ( ( 3, 2, 2, 2, 3 ),
 ( 0.2305555555555555691, 0.2314814814814814825, 0.2333333333333333370, 0.2351851851851851916, 0.2361111111111111049 ),
 .UNSPECIFIED. ) 
 CURVE ( )  GEOMETRIC_REPRESENTATION_ITEM ( )  RATIONAL_B_SPLINE_CURVE ( ( 0.9330127018922194093, 0.9330127018922204085, 1.000000000000000000, 0.8660254037844388186, 1.000000000000000000, 0.8660254037844388186, 1.000000000000000000, 0.9330127018922205195, 0.9330127018922196314 ) ) 
 REPRESENTATION_ITEM ( '' )  );
#23754=CARTESIAN_POINT ( 'NONE',  ( 2.775557561562891351E-14, 6.250000000000033751, -100.9330127018922525 ) ) ;
#23755=CYLINDRICAL_SURFACE ( 'NONE', #19179, 6.000000000000000888 ) ;
#23758=CARTESIAN_POINT ( 'NONE',  ( -5.999999999999963585, 1.780251999655701777E-13, -58.41367513459482552 ) ) ;
#23760=EDGE_CURVE ( 'NONE', #2905, #2098, #13642, .T. ) ;
#23762=ADVANCED_FACE ( 'NONE', ( #15785 ), #23429, .T. ) ;
#23763=CARTESIAN_POINT ( 'NONE',  ( -3.175426480542816066, 5.499999999999865885, -163.3750000000000568 ) ) ;
#23764=CARTESIAN_POINT ( 'NONE',  ( -3.464101615137725076, 5.999999999999979572, -58.08632486540519579 ) ) ;
#23765=CARTESIAN_POINT ( 'NONE',  ( 3.175426480543072749, 5.499999999999865885, -156.1250000000000000 ) ) ;
#23767=CARTESIAN_POINT ( 'NONE',  ( -3.175426480542816510, -5.500000000000057732, -92.37500000000002842 ) ) ;
#23768=CARTESIAN_POINT ( 'NONE',  ( 3.464101615137757051, -5.999999999999979572, -135.9136751345947971 ) ) ;
#23772=CARTESIAN_POINT ( 'NONE',  ( 3.464101615137852974, 5.999999999999884537, -126.4136751345948113 ) ) ;
#23774=DIRECTION ( 'NONE',  ( 1.000000000000000000, -5.551115123125773458E-17, -1.260129944081490338E-35 ) ) ;
#23775=ORIENTED_EDGE ( 'NONE', *, *, #14701, .T. ) ;
#23776=FILL_AREA_STYLE ('',( #19041 ) ) ;
#23777=LINE ( 'NONE', #12138, #28004 ) ;
#23779=ORIENTED_EDGE ( 'NONE', *, *, #12207, .T. ) ;
#23781=EDGE_CURVE ( 'NONE', #25470, #22801, #19064, .T. ) ;
#23782=CARTESIAN_POINT ( 'NONE',  ( -4.763139720814407951, 2.749999999999946709, -110.7500000000000142 ) ) ;
#23784=CARTESIAN_POINT ( 'NONE',  ( -5.412658773652684552, -3.125000000000099920, -119.9330127018922667 ) ) ;
#23787=CARTESIAN_POINT ( 'NONE',  ( -5.412658773652739619, 3.124999999999975131, -162.8169872981078470 ) ) ;
#23792=CARTESIAN_POINT ( 'NONE',  ( 6.000000000000000888, 1.743066579297358182E-13, -96.66367513459479710 ) ) ;
#23793=DIRECTION ( 'NONE',  ( 1.000000000000000000, -5.551115123125773458E-17, -1.260129944081490338E-35 ) ) ;
#23794=CARTESIAN_POINT ( 'NONE',  ( -3.175426480542816510, -5.500000000000057732, -177.8750000000000568 ) ) ;
#23797=CARTESIAN_POINT ( 'NONE',  ( -3.608439182435052128, -6.250000000000110134, -175.3080127018922667 ) ) ;
#23800=CARTESIAN_POINT ( 'NONE',  ( -4.763139720814407951, -2.750000000000016431, -124.0000000000000000 ) ) ;
#23802=UNCERTAINTY_MEASURE_WITH_UNIT (LENGTH_MEASURE( 1.000000000000000082E-05 ), #29198, 'distance_accuracy_value', 'NONE');
#23803=CARTESIAN_POINT ( 'NONE',  ( 3.175426480543072749, 5.499999999999865885, -117.1250000000000142 ) ) ;
#23804=CARTESIAN_POINT ( 'NONE',  ( -6.000000000000000888, 1.067854986875958443E-15, 7.560779664488942560E-35 ) ) ;
#23805=CARTESIAN_POINT ( 'NONE',  ( 6.000000000000000888, -1.859271017917181981E-14, -131.1636751345948539 ) ) ;
#23808=DIRECTION ( 'NONE',  ( -7.147005652999508048E-36, 5.642372883946980038E-36, 1.000000000000000000 ) ) ;
#23809=CARTESIAN_POINT ( 'NONE',  ( 5.196152422706629359, -2.999999999999988898, -55.71132486540519579 ) ) ;
#23813=CARTESIAN_POINT ( 'NONE',  ( -6.350852961085760029, -1.281975124255709124E-13, -176.6250000000000284 ) ) ;
#23815=ORIENTED_EDGE ( 'NONE', *, *, #27603, .T. ) ;
#23816=CARTESIAN_POINT ( 'NONE',  ( -6.000000000000007105, -1.607695154586655129, -77.84668783648702117 ) ) ;
#23817=ORIENTED_EDGE ( 'NONE', *, *, #20072, .F. ) ;
#23818=EDGE_LOOP ( 'NONE', ( #19870, #29958, #26688, #5 ) ) ;
#23819=CARTESIAN_POINT ( 'NONE',  ( -5.999999999999963585, -2.788906526875773208E-15, -176.3363248654052029 ) ) ;
#23822=AXIS2_PLACEMENT_3D ( 'NONE', #30225, #23342, #16450 ) ;
#23825=CARTESIAN_POINT ( 'NONE',  ( -3.608439182435115633, 6.249999999999965361, -138.9419872981077901 ) ) ;
#23827=CARTESIAN_POINT ( 'NONE',  ( -3.464101615137725076, 5.999999999999979572, -175.0863248654052029 ) ) ;
#23831=CARTESIAN_POINT ( 'NONE',  ( 0.000000000000000000, -5.999999999999991118, -130.0386751345948824 ) ) ;
#23832=LINE ( 'NONE', #29009, #10797 ) ;
#23833=CARTESIAN_POINT ( 'NONE',  ( -2.000000000000000000, 3.559516622919861969E-16, -185.0000000000000000 ) ) ;
#23835=CARTESIAN_POINT ( 'NONE',  ( -5.999999999999919176, 1.607695154586804565, -98.98066243270261566 ) ) ;
#23837=CARTESIAN_POINT ( 'NONE',  ( 6.000000000000000888, 1.607695154586715303, -147.0193375672974696 ) ) ;
#23840=CARTESIAN_POINT ( 'NONE',  ( -3.464101615137725076, 5.999999999999979572, -113.5863248654051887 ) ) ;
#23842=VERTEX_POINT ( 'NONE', #16977 ) ;
#23843=DIRECTION ( 'NONE',  ( -7.147005652999508048E-36, 5.642372883946980038E-36, 1.000000000000000000 ) ) ;
#23844=CARTESIAN_POINT ( 'NONE',  ( -3.464101615137725076, 5.999999999999979572, -62.58632486540521711 ) ) ;
#23850=CARTESIAN_POINT ( 'NONE',  ( -5.412658773652684552, -3.125000000000099920, -105.5669872981078186 ) ) ;
#23854=CARTESIAN_POINT ( 'NONE',  ( 0.000000000000000000, 5.499999999999991118, -129.0000000000000000 ) ) ;
#23855=EDGE_CURVE ( 'NONE', #27302, #22419, #2806, .T. ) ;
#23859=CARTESIAN_POINT ( 'NONE',  ( 4.763139720814407951, -2.749999999999988454, -54.49999999999999289 ) ) ;
#23860=CARTESIAN_POINT ( 'NONE',  ( -5.999999999999963585, 0.000000000000000000, -179.9136751345948255 ) ) ;
#23862=CARTESIAN_POINT ( 'NONE',  ( -5.412658773652684552, -3.125000000000099920, -80.93301270189223828 ) ) ;
#23864=CARTESIAN_POINT ( 'NONE',  ( 5.196152422706629359, 3.000000000000002665, -149.9613248654052597 ) ) ;
#23867=CARTESIAN_POINT ( 'NONE',  ( -3.175426480542816066, 5.499999999999865885, -139.3750000000000568 ) ) ;
#23869=CARTESIAN_POINT ( 'NONE',  ( -3.608439182435115633, 6.249999999999965361, -150.3080127018922099 ) ) ;
#23870=CARTESIAN_POINT ( 'NONE',  ( 5.196152422706629359, -2.999999999999988898, -70.71132486540521711 ) ) ;
#23872=CARTESIAN_POINT ( 'NONE',  ( -3.175426480542816066, 5.499999999999865885, -70.37500000000004263 ) ) ;
#23873=CARTESIAN_POINT ( 'NONE',  ( 0.000000000000000000, 5.499999999999991118, -64.50000000000000000 ) ) ;
#23882=CARTESIAN_POINT ( 'NONE',  ( 6.000000000000000888, 7.762456499804234384E-14, -144.6636751345948255 ) ) ;
#23883=VERTEX_POINT ( 'NONE', #19271 ) ;
#23888=CARTESIAN_POINT ( 'NONE',  ( 3.464101615137757051, -5.999999999999979572, -102.3363248654052171 ) ) ;
#23890=CARTESIAN_POINT ( 'NONE',  ( -3.175426480542816510, 5.499999999999865885, -178.3750000000000568 ) ) ;
#23892=ORIENTED_EDGE ( 'NONE', *, *, #4341, .T. ) ;
#23893=CARTESIAN_POINT ( 'NONE',  ( 7.216878364870455975, -6.409875621278545621E-14, -155.9419872981078470 ) ) ;
#23894=VERTEX_POINT ( 'NONE', #16539 ) ;
#23895=CARTESIAN_POINT ( 'NONE',  ( -6.350852961085760029, -1.281975124255709124E-13, -83.62499999999998579 ) ) ;
#23896=CARTESIAN_POINT ( 'NONE',  ( -7.216878364870328078, 0.000000000000000000, -99.05801270189222407 ) ) ;
#23897=ORIENTED_EDGE ( 'NONE', *, *, #7417, .T. ) ;
#23898=VECTOR ( 'NONE', #11932, 1000.000000000000000 ) ;
#23899=DIRECTION ( 'NONE',  ( -7.147005652999508048E-36, 5.642372883946980038E-36, 1.000000000000000000 ) ) ;
#23900=CARTESIAN_POINT ( 'NONE',  ( 5.950275682033426605, -9.251745015924175419, -24.20335556275641054 ) ) ;
#23904=CARTESIAN_POINT ( 'NONE',  ( 4.763139720814407951, 2.750000000000002665, -163.7500000000000000 ) ) ;
#23906=CARTESIAN_POINT ( 'NONE',  ( 0.000000000000000000, 5.499999999999991118, -154.5000000000000284 ) ) ;
#23907=CARTESIAN_POINT ( 'NONE',  ( 0.000000000000000000, 5.999999999999977796, -76.78867513459481131 ) ) ;
#23909=CARTESIAN_POINT ( 'NONE',  ( -3.175426480542816066, 5.499999999999865885, -91.37500000000001421 ) ) ;
#23912=CARTESIAN_POINT ( 'NONE',  ( -2.775557561562891351E-14, -5.500000000000115463, -86.25000000000004263 ) ) ;
#23918=EDGE_CURVE ( 'NONE', #29310, #8028, #27001, .T. ) ;
#23919=CARTESIAN_POINT ( 'NONE',  ( 3.464101615137757051, -5.999999999999979572, -66.33632486540516027 ) ) ;
#23920=CYLINDRICAL_SURFACE ( 'NONE', #27705, 6.000000000000000888 ) ;
#23922=( LENGTH_UNIT ( ) NAMED_UNIT ( * ) SI_UNIT ( .MILLI., .METRE. ) );
#23923=CYLINDRICAL_SURFACE ( 'NONE', #536, 6.000000000000000888 ) ;
#23929=ADVANCED_FACE ( 'NONE', ( #20008 ), #3553, .T. ) ;
#23932=CARTESIAN_POINT ( 'NONE',  ( -2.775557561562891351E-14, -5.500000000000115463, -108.7500000000000142 ) ) ;
#23934=CARTESIAN_POINT ( 'NONE',  ( 4.763139720814407951, -2.749999999999988454, -150.5000000000000284 ) ) ;
#23935=CARTESIAN_POINT ( 'NONE',  ( 5.412658773652712085, -3.125000000000086153, -122.4330127018922241 ) ) ;
#23937=CARTESIAN_POINT ( 'NONE',  ( -5.999999999999963585, 1.780251999655701777E-13, -110.9136751345948255 ) ) ;
#23938=CARTESIAN_POINT ( 'NONE',  ( 2.775557561562891351E-14, 6.250000000000033751, -164.5669872981078186 ) ) ;
#23940=VECTOR ( 'NONE', #10954, 1000.000000000000000 ) ;
#23942=CARTESIAN_POINT ( 'NONE',  ( 2.775557561562891351E-14, 6.250000000000033751, -57.43301270189227381 ) ) ;
#23943=ORIENTED_EDGE ( 'NONE', *, *, #23918, .T. ) ;
#23944=CARTESIAN_POINT ( 'NONE',  ( 6.000000000000000888, 1.607695154586715303, -168.0193375672974128 ) ) ;
#23947=CARTESIAN_POINT ( 'NONE',  ( 4.763139720814407951, 2.750000000000002665, -178.7500000000000284 ) ) ;
#23949=CARTESIAN_POINT ( 'NONE',  ( -3.464101615137757051, -5.999999999999979572, -169.1636751345948255 ) ) ;
#23950=CARTESIAN_POINT ( 'NONE',  ( 3.608439182435180470, 6.249999999999982236, -179.0580127018922667 ) ) ;
#23952=CARTESIAN_POINT ( 'NONE',  ( -3.464101615137757051, -5.999999999999979572, -48.58632486540521711 ) ) ;
#23953=CARTESIAN_POINT ( 'NONE',  ( 6.350852961086080661, -9.614813431917819062E-14, -114.3750000000000000 ) ) ;
#23954=CARTESIAN_POINT ( 'NONE',  ( 3.464101615137852974, 5.999999999999884537, -84.41367513459481131 ) ) ;
#23955=CARTESIAN_POINT ( 'NONE',  ( 0.000000000000000000, 5.499999999999991118, -109.5000000000000426 ) ) ;
#23957=ORIENTED_EDGE ( 'NONE', *, *, #29482, .T. ) ;
#23959=CARTESIAN_POINT ( 'NONE',  ( 2.775557561562891351E-14, 20.00000000000001776, -25.00000000000002132 ) ) ;
#23961=CYLINDRICAL_SURFACE ( 'NONE', #28290, 6.000000000000000888 ) ;
#23962=CARTESIAN_POINT ( 'NONE',  ( 5.999999999999949374, -1.607695154586841868, -145.6533121635130499 ) ) ;
#23966=ADVANCED_FACE ( 'NONE', ( #24448 ), #5706, .T. ) ;
#23968=VERTEX_POINT ( 'NONE', #17578 ) ;
#23969=VERTEX_POINT ( 'NONE', #22168 ) ;
#23973=CARTESIAN_POINT ( 'NONE',  ( 3.608439182435180470, -6.249999999999997335, -127.6919872981078328 ) ) ;
#23976=CARTESIAN_POINT ( 'NONE',  ( 6.000000000000000888, 7.762456499804234384E-14, -129.6636751345948255 ) ) ;
#23977=CARTESIAN_POINT ( 'NONE',  ( 6.000000000000000888, -3.330669073875464691E-16, -7.560779664488942560E-35 ) ) ;
#23981=DIRECTION ( 'NONE',  ( 1.000000000000000000, -5.551115123125773458E-17, -1.260129944081490338E-35 ) ) ;
#23983=CARTESIAN_POINT ( 'NONE',  ( -6.350852961085760029, -1.281975124255709124E-13, -137.6250000000000568 ) ) ;
#23985=ORIENTED_EDGE ( 'NONE', *, *, #3829, .T. ) ;
#23986=EDGE_CURVE ( 'NONE', #10258, #124, #6183, .T. ) ;
#23991=ORIENTED_EDGE ( 'NONE', *, *, #933, .T. ) ;
#23994=CARTESIAN_POINT ( 'NONE',  ( -3.608439182435115633, 6.249999999999965361, -98.44198729810783277 ) ) ;
#23999=CARTESIAN_POINT ( 'NONE',  ( 4.763139720814407951, 2.750000000000002665, -126.2500000000000284 ) ) ;
#24002=CARTESIAN_POINT ( 'NONE',  ( -3.175426480542816510, 5.499999999999865885, -61.37500000000000000 ) ) ;
#24003=CARTESIAN_POINT ( 'NONE',  ( 6.000000000000000888, 1.607695154586715303, -116.0966878364870496 ) ) ;
#24005=CARTESIAN_POINT ( 'NONE',  ( 5.196552517144625405, 9.698180938751583824, -21.97571210926420093 ) ) ;
#24006=( BOUNDED_CURVE ( )  B_SPLINE_CURVE ( 2, ( #15908, #28119, #11743, #23396, #21087, #7090, #2034, #9406, #4168 ),
 .UNSPECIFIED., .F., .F. ) 
 B_SPLINE_CURVE_WITH_KNOTS ( ( 3, 2, 2, 2, 3 ),
 ( 0.2583333333333333037, 0.2592592592592592449, 0.2611111111111111271, 0.2629629629629629539, 0.2638888888888888951 ),
 .UNSPECIFIED. ) 
 CURVE ( )  GEOMETRIC_REPRESENTATION_ITEM ( )  RATIONAL_B_SPLINE_CURVE ( ( 0.9330127018922194093, 0.9330127018922174109, 1.000000000000000000, 0.8660254037844388186, 1.000000000000000000, 0.8660254037844388186, 1.000000000000000000, 0.9330127018922194093, 0.9330127018922194093 ) ) 
 REPRESENTATION_ITEM ( '' )  );
#24007=CARTESIAN_POINT ( 'NONE',  ( 3.608439182435180470, 6.249999999999982236, -86.05801270189222407 ) ) ;
#24008=DIRECTION ( 'NONE',  ( -0.7071067811865477948, 3.925231146709432986E-17, -0.7071067811865472397 ) ) ;
#24009=CARTESIAN_POINT ( 'NONE',  ( 5.999999999999949374, 1.607695154586804565, -150.0193375672974128 ) ) ;
#24013=( BOUNDED_CURVE ( )  B_SPLINE_CURVE ( 2, ( #10644, #22304, #19840, #10181, #24436, #14654, #10333, #19552, #28885 ),
 .UNSPECIFIED., .F., .T. ) 
 B_SPLINE_CURVE_WITH_KNOTS ( ( 3, 2, 2, 2, 3 ),
 ( 0.2305555555555556246, 0.2314814814814815103, 0.2333333333333332815, 0.2351851851851851638, 0.2361111111111110494 ),
 .UNSPECIFIED. ) 
 CURVE ( )  GEOMETRIC_REPRESENTATION_ITEM ( )  RATIONAL_B_SPLINE_CURVE ( ( 0.9330127018922194093, 0.9330127018922234061, 1.000000000000000000, 0.8660254037844388186, 1.000000000000000000, 0.8660254037844388186, 1.000000000000000000, 0.9330127018922234061, 0.9330127018922194093 ) ) 
 REPRESENTATION_ITEM ( '' )  );
#24014=CARTESIAN_POINT ( 'NONE',  ( -3.175426480542816066, -5.500000000000057732, -137.3750000000000568 ) ) ;
#24016=CARTESIAN_POINT ( 'NONE',  ( -7.216878364870328078, 0.000000000000000000, -153.0580127018922383 ) ) ;
#24017=CARTESIAN_POINT ( 'NONE',  ( 4.763139720814407951, 2.750000000000002665, -67.75000000000002842 ) ) ;
#24018=CARTESIAN_POINT ( 'NONE',  ( -4.763139720814407951, 2.749999999999946709, -65.75000000000002842 ) ) ;
#24019=EDGE_CURVE ( 'NONE', #23883, #14503, #15862, .T. ) ;
#24023=CARTESIAN_POINT ( 'NONE',  ( -3.464101615137725076, 5.999999999999979572, -127.0863248654051887 ) ) ;
#24025=CARTESIAN_POINT ( 'NONE',  ( 3.464101615137757051, -5.999999999999979572, -104.4136751345948539 ) ) ;
#24026=CYLINDRICAL_SURFACE ( 'NONE', #15533, 6.000000000000000888 ) ;
#24027=ORIENTED_EDGE ( 'NONE', *, *, #4350, .F. ) ;
#24031=CARTESIAN_POINT ( 'NONE',  ( -5.999999999999962697, 3.323446944526963891E-14, -158.9136751345947971 ) ) ;
#24032=CARTESIAN_POINT ( 'NONE',  ( 4.763139720814407951, 2.750000000000002665, -177.2500000000000284 ) ) ;
#24034=ORIENTED_EDGE ( 'NONE', *, *, #8120, .F. ) ;
#24035=CARTESIAN_POINT ( 'NONE',  ( 3.608439182435180470, 6.249999999999982236, -154.1919872981078186 ) ) ;
#24036=ORIENTED_EDGE ( 'NONE', *, *, #23282, .F. ) ;
#24037=CARTESIAN_POINT ( 'NONE',  ( -4.763139720814407951, 2.749999999999946709, -80.74999999999998579 ) ) ;
#24038=CARTESIAN_POINT ( 'NONE',  ( 3.608439182435180470, 6.249999999999982236, -101.0580127018922241 ) ) ;
#24042=CARTESIAN_POINT ( 'NONE',  ( 6.350852961086080661, -9.614813431917819062E-14, -168.3750000000000568 ) ) ;
#24044=CARTESIAN_POINT ( 'NONE',  ( 5.920437777358367626, -9.270953676058775628, -24.00610273346770640 ) ) ;
#24045=CARTESIAN_POINT ( 'NONE',  ( 3.175426480543072749, -5.500000000000105693, -167.1250000000000000 ) ) ;
#24046=CARTESIAN_POINT ( 'NONE',  ( 3.464101615137757051, -5.999999999999979572, -60.33632486540521001 ) ) ;
#24047=CARTESIAN_POINT ( 'NONE',  ( 4.763139720814407951, 2.750000000000002665, -147.2500000000000000 ) ) ;
#24048=CYLINDRICAL_SURFACE ( 'NONE', #13031, 6.000000000000000888 ) ;
#24050=CARTESIAN_POINT ( 'NONE',  ( 3.175426480543072749, 5.499999999999865885, -97.62500000000004263 ) ) ;
#24052=CARTESIAN_POINT ( 'NONE',  ( 4.763139720814407951, 2.750000000000002665, -91.75000000000000000 ) ) ;
#24053=EDGE_CURVE ( 'NONE', #5313, #2934, #8162, .T. ) ;
#24054=CARTESIAN_POINT ( 'NONE',  ( 6.000000000000000888, 1.743066579297358182E-13, -99.66367513459479710 ) ) ;
#24055=CARTESIAN_POINT ( 'NONE',  ( -5.196152422706601826, 2.999999999999975131, -64.53867513459482552 ) ) ;
#24056=CARTESIAN_POINT ( 'NONE',  ( 6.000000000000000888, -1.859271017917181981E-14, -93.66367513459481131 ) ) ;
#24059=CARTESIAN_POINT ( 'NONE',  ( -3.464101615137725076, 5.999999999999979572, -126.1636751345948113 ) ) ;
#24062=ORIENTED_EDGE ( 'NONE', *, *, #8222, .F. ) ;
#24063=CARTESIAN_POINT ( 'NONE',  ( 0.000000000000000000, 0.000000000000000000, 0.000000000000000000 ) ) ;
#24066=EDGE_LOOP ( 'NONE', ( #4688, #1625, #23503, #22955 ) ) ;
#24068=CARTESIAN_POINT ( 'NONE',  ( -3.175426480542816510, -5.500000000000057732, -104.3750000000000142 ) ) ;
#24070=CARTESIAN_POINT ( 'NONE',  ( -3.608439182435115633, 6.249999999999965361, -123.3080127018922099 ) ) ;
#24074=CARTESIAN_POINT ( 'NONE',  ( 7.216878364870455975, -6.409875621278545621E-14, -157.4419872981077901 ) ) ;
#24077=EDGE_CURVE ( 'NONE', #14503, #14874, #22935, .T. ) ;
#24078=CARTESIAN_POINT ( 'NONE',  ( 5.412658773652712085, -3.125000000000086153, -57.93301270189221697 ) ) ;
#24080=CARTESIAN_POINT ( 'NONE',  ( 5.196152422706629359, 3.000000000000002665, -117.5386751345948113 ) ) ;
#24082=CARTESIAN_POINT ( 'NONE',  ( 6.000000000000000888, 7.762456499804235646E-14, -142.5863248654051745 ) ) ;
#24085=CARTESIAN_POINT ( 'NONE',  ( -3.608439182435052128, -6.250000000000110134, -167.8080127018922951 ) ) ;
#24089=CARTESIAN_POINT ( 'NONE',  ( -4.763139720814407951, -2.750000000000016431, -114.9999999999999858 ) ) ;
#24091=CARTESIAN_POINT ( 'NONE',  ( 3.175426480543072749, -5.500000000000105693, -114.6250000000000000 ) ) ;
#24093=CARTESIAN_POINT ( 'NONE',  ( 0.000000000000000000, 5.999999999999977796, -100.7886751345948255 ) ) ;
#24094=VECTOR ( 'NONE', #19328, 1000.000000000000000 ) ;
#24095=EDGE_LOOP ( 'NONE', ( #24465, #15044, #27760, #6298 ) ) ;
#24099=( BOUNDED_CURVE ( )  B_SPLINE_CURVE ( 2, ( #2128, #2283, #18583, #8890, #18427, #20400, #16301, #11054, #13842 ),
 .UNSPECIFIED., .F., .T. ) 
 B_SPLINE_CURVE_WITH_KNOTS ( ( 3, 2, 2, 2, 3 ),
 ( 0.4861111111111111605, 0.4870370370370370461, 0.4888888888888889284, 0.4907407407407406996, 0.4916666666666665853 ),
 .UNSPECIFIED. ) 
 CURVE ( )  GEOMETRIC_REPRESENTATION_ITEM ( )  RATIONAL_B_SPLINE_CURVE ( ( 0.9330127018922194093, 0.9330127018922234061, 1.000000000000000000, 0.8660254037844388186, 1.000000000000000000, 0.8660254037844388186, 1.000000000000000000, 0.9330127018922234061, 0.9330127018922194093 ) ) 
 REPRESENTATION_ITEM ( '' )  );
#24104=CARTESIAN_POINT ( 'NONE',  ( -5.999999999999963585, 8.134310703387671600E-14, -125.9136751345948397 ) ) ;
#24111=CARTESIAN_POINT ( 'NONE',  ( -3.608439182435052128, -6.250000000000110134, -129.4419872981078186 ) ) ;
#24113=DIRECTION ( 'NONE',  ( 1.000000000000000000, -5.551115123125773458E-17, -1.260129944081490338E-35 ) ) ;
#24114=DIRECTION ( 'NONE',  ( 1.000000000000000000, -5.551115123125773458E-17, -1.260129944081490338E-35 ) ) ;
#24118=CARTESIAN_POINT ( 'NONE',  ( -5.999999999999963585, 1.780251999655701777E-13, -84.83632486540523132 ) ) ;
#24119=DIRECTION ( 'NONE',  ( -7.147005652999508048E-36, 5.642372883946980038E-36, 1.000000000000000000 ) ) ;
#24123=CARTESIAN_POINT ( 'NONE',  ( -3.464101615137725076, 5.999999999999979572, -146.5863248654052313 ) ) ;
#24125=CARTESIAN_POINT ( 'NONE',  ( -6.000000000000007105, -1.607695154586655129, -162.7693375672974128 ) ) ;
#24126=CARTESIAN_POINT ( 'NONE',  ( -5.196152422706573404, -3.000000000000002665, -115.2886751345948397 ) ) ;
#24128=CARTESIAN_POINT ( 'NONE',  ( 4.763139720814407951, 2.750000000000002665, -133.7500000000000284 ) ) ;
#24132=ORIENTED_EDGE ( 'NONE', *, *, #6128, .F. ) ;
#24136=EDGE_LOOP ( 'NONE', ( #9926, #4272, #3524, #3714 ) ) ;
#24139=CARTESIAN_POINT ( 'NONE',  ( -7.216878364870328078, 0.000000000000000000, -98.19198729810781856 ) ) ;
#24145=CARTESIAN_POINT ( 'NONE',  ( 4.763139720814407951, -2.749999999999988454, -132.5000000000000000 ) ) ;
#24146=ORIENTED_EDGE ( 'NONE', *, *, #27994, .F. ) ;
#24149=CARTESIAN_POINT ( 'NONE',  ( -2.775557561562891351E-14, -5.500000000000115463, -54.75000000000002132 ) ) ;
#24152=CARTESIAN_POINT ( 'NONE',  ( 5.196152422706629359, -2.999999999999988898, -62.28867513459485394 ) ) ;
#24153=CARTESIAN_POINT ( 'NONE',  ( 5.381246803625141517, 9.595437032880905548, -22.31808132294488445 ) ) ;
#24155=CARTESIAN_POINT ( 'NONE',  ( -5.412658773652684552, -3.125000000000099920, -74.93301270189223828 ) ) ;
#24156=DIRECTION ( 'NONE',  ( 1.000000000000000000, -5.551115123125773458E-17, -1.260129944081490338E-35 ) ) ;
#24157=CARTESIAN_POINT ( 'NONE',  ( 0.000000000000000000, 0.000000000000000000, -14.99152654425661702 ) ) ;
#24159=DIRECTION ( 'NONE',  ( -7.147005652999508048E-36, 5.642372883946980038E-36, 1.000000000000000000 ) ) ;
#24161=CARTESIAN_POINT ( 'NONE',  ( 0.000000000000000000, 5.499999999999991118, -141.0000000000000000 ) ) ;
#24163=CARTESIAN_POINT ( 'NONE',  ( 7.216878364870455975, -6.409875621278545621E-14, -155.3080127018922099 ) ) ;
#24166=CARTESIAN_POINT ( 'NONE',  ( -6.350852961085760029, -1.281975124255709124E-13, -67.12500000000002842 ) ) ;
#24167=CARTESIAN_POINT ( 'NONE',  ( 5.196152422706629359, 3.000000000000002665, -86.03867513459483973 ) ) ;
#24168=CARTESIAN_POINT ( 'NONE',  ( -3.175426480542816510, -5.500000000000057732, -54.87500000000003553 ) ) ;
#24170=EDGE_LOOP ( 'NONE', ( #4652, #11574, #18673, #21097 ) ) ;
#24175=DIRECTION ( 'NONE',  ( -7.147005652999508048E-36, 5.642372883946980038E-36, 1.000000000000000000 ) ) ;
#24176=EDGE_LOOP ( 'NONE', ( #18878, #15703, #21046, #21197 ) ) ;
#24178=( BOUNDED_CURVE ( )  B_SPLINE_CURVE ( 2, ( #27569, #23003, #25749, #9480, #6706, #15969, #25267, #4239, #4695 ),
 .UNSPECIFIED., .F., .F. ) 
 B_SPLINE_CURVE_WITH_KNOTS ( ( 3, 2, 2, 2, 3 ),
 ( 0.5583333333333333481, 0.5592592592592592338, 0.5611111111111111160, 0.5629629629629629983, 0.5638888888888888840 ),
 .UNSPECIFIED. ) 
 CURVE ( )  GEOMETRIC_REPRESENTATION_ITEM ( )  RATIONAL_B_SPLINE_CURVE ( ( 0.9330127018922194093, 0.9330127018922194093, 1.000000000000000000, 0.8660254037844388186, 1.000000000000000000, 0.8660254037844388186, 1.000000000000000000, 0.9330127018922194093, 0.9330127018922194093 ) ) 
 REPRESENTATION_ITEM ( '' )  );
#24180=CARTESIAN_POINT ( 'NONE',  ( 3.608439182435180470, -6.249999999999997335, -46.69198729810783277 ) ) ;
#24183=CARTESIAN_POINT ( 'NONE',  ( 4.763139720814407951, -2.749999999999988454, -81.50000000000001421 ) ) ;
#24184=EDGE_CURVE ( 'NONE', #23551, #16922, #18801, .T. ) ;
#24185=EDGE_CURVE ( 'NONE', #12143, #26678, #22097, .T. ) ;
#24186=( BOUNDED_CURVE ( )  B_SPLINE_CURVE ( 2, ( #28468, #2824, #14541, #12247, #18845, #18541, #6835, #16259, #28168 ),
 .UNSPECIFIED., .F., .T. ) 
 B_SPLINE_CURVE_WITH_KNOTS ( ( 3, 2, 2, 2, 3 ),
 ( 0.7472222222222222321, 0.7481481481481482287, 0.7500000000000000000, 0.7518518518518518823, 0.7527777777777777679 ),
 .UNSPECIFIED. ) 
 CURVE ( )  GEOMETRIC_REPRESENTATION_ITEM ( )  RATIONAL_B_SPLINE_CURVE ( ( 0.9330127018922194093, 0.9330127018922194093, 1.000000000000000000, 0.8660254037844388186, 1.000000000000000000, 0.8660254037844388186, 1.000000000000000000, 0.9330127018922234061, 0.9330127018922194093 ) ) 
 REPRESENTATION_ITEM ( '' )  );
#24187=CARTESIAN_POINT ( 'NONE',  ( 5.196152422706629359, 3.000000000000002665, -176.0386751345948255 ) ) ;
#24188=CARTESIAN_POINT ( 'NONE',  ( 6.000000000000000888, -3.330669073875464691E-16, -7.560779664488942560E-35 ) ) ;
#24189=CARTESIAN_POINT ( 'NONE',  ( 5.990257846049584778, -9.225907948257320967, -24.60347258678507387 ) ) ;
#24192=VECTOR ( 'NONE', #24740, 1000.000000000000000 ) ;
#24193=CARTESIAN_POINT ( 'NONE',  ( -2.775557561562891351E-14, -5.500000000000115463, -165.7500000000000000 ) ) ;
#24194=CARTESIAN_POINT ( 'NONE',  ( 4.763139720814407951, -2.749999999999988454, -150.5000000000000284 ) ) ;
#24196=CARTESIAN_POINT ( 'NONE',  ( -3.175426480542816066, 5.499999999999865885, -95.87500000000004263 ) ) ;
#24197=CARTESIAN_POINT ( 'NONE',  ( 6.000000000000000888, -1.859271017917181981E-14, -130.5863248654052313 ) ) ;
#24198=CARTESIAN_POINT ( 'NONE',  ( -3.175426480542816510, 5.499999999999865885, -79.37500000000001421 ) ) ;
#24200=CARTESIAN_POINT ( 'NONE',  ( -3.464101615137757051, -5.999999999999979572, -136.1636751345947971 ) ) ;
#24203=DIRECTION ( 'NONE',  ( -7.147005652999508048E-36, 5.642372883946980038E-36, 1.000000000000000000 ) ) ;
#24206=DIRECTION ( 'NONE',  ( -7.147005652999508048E-36, 5.642372883946980038E-36, 1.000000000000000000 ) ) ;
#24207=CARTESIAN_POINT ( 'NONE',  ( 3.464101615137757051, -5.999999999999979572, -78.91367513459476868 ) ) ;
#24212=CARTESIAN_POINT ( 'NONE',  ( -6.350852961085760029, -1.281975124255709124E-13, -103.1250000000000000 ) ) ;
#24214=ADVANCED_FACE ( 'NONE', ( #4924 ), #323, .T. ) ;
#24215=CARTESIAN_POINT ( 'NONE',  ( -3.608439182435115633, 6.249999999999965361, -124.8080127018922099 ) ) ;
#24216=VERTEX_POINT ( 'NONE', #26420 ) ;
#24217=CARTESIAN_POINT ( 'NONE',  ( 0.000000000000000000, -5.999999999999991118, -110.5386751345948113 ) ) ;
#24218=CARTESIAN_POINT ( 'NONE',  ( 3.608439182435180470, 6.249999999999982236, -164.6919872981078754 ) ) ;
#24220=( BOUNDED_CURVE ( )  B_SPLINE_CURVE ( 2, ( #12046, #320, #1023, #8080, #10574, #19927, #9709, #11195, #11512 ),
 .UNSPECIFIED., .F., .F. ) 
 B_SPLINE_CURVE_WITH_KNOTS ( ( 3, 2, 2, 2, 3 ),
 ( 0.9249999999999999334, 0.9259259259259259300, 0.9277777777777778123, 0.9296296296296295836, 0.9305555555555555802 ),
 .UNSPECIFIED. ) 
 CURVE ( )  GEOMETRIC_REPRESENTATION_ITEM ( )  RATIONAL_B_SPLINE_CURVE ( ( 0.9330127018922194093, 0.9330127018922154125, 1.000000000000000000, 0.8660254037844388186, 1.000000000000000000, 0.8660254037844388186, 1.000000000000000000, 0.9330127018922154125, 0.9330127018922194093 ) ) 
 REPRESENTATION_ITEM ( '' )  );
#24221=CARTESIAN_POINT ( 'NONE',  ( 3.608439182435180470, 6.249999999999982236, -57.55801270189221697 ) ) ;
#24222=ORIENTED_EDGE ( 'NONE', *, *, #9401, .F. ) ;
#24224=CYLINDRICAL_SURFACE ( 'NONE', #16520, 6.000000000000000888 ) ;
#24226=CARTESIAN_POINT ( 'NONE',  ( 3.175426480543072749, -5.500000000000105693, -168.6250000000000000 ) ) ;
#24228=CARTESIAN_POINT ( 'NONE',  ( -5.412658773652739619, 3.124999999999975131, -168.1830127018922383 ) ) ;
#24231=CARTESIAN_POINT ( 'NONE',  ( 6.350852961086080661, -9.614813431917819062E-14, -118.8750000000000426 ) ) ;
#24233=CARTESIAN_POINT ( 'NONE',  ( -2.775557561562891351E-14, -5.500000000000115463, -108.7500000000000142 ) ) ;
#24237=CARTESIAN_POINT ( 'NONE',  ( 6.000000000000052403, -1.607695154586662678, -90.15331216351299304 ) ) ;
#24238=CARTESIAN_POINT ( 'NONE',  ( 6.000000000000052403, -1.607695154586662678, -75.73066243270262987 ) ) ;
#24239=ORIENTED_EDGE ( 'NONE', *, *, #8455, .F. ) ;
#24240=CARTESIAN_POINT ( 'NONE',  ( -3.464101615137757051, -5.999999999999979572, -127.1636751345948113 ) ) ;
#24241=ADVANCED_FACE ( 'NONE', ( #25834, #21090 ), #21, .T. ) ;
#24242=ADVANCED_FACE ( 'NONE', ( #5518 ), #22442, .T. ) ;
#24243=CARTESIAN_POINT ( 'NONE',  ( 7.216878364870455975, -6.409875621278545621E-14, -79.44198729810779014 ) ) ;
#24251=CARTESIAN_POINT ( 'NONE',  ( 3.608439182435180470, 6.249999999999982236, -128.6919872981078186 ) ) ;
#24253=LINE ( 'NONE', #5974, #21453 ) ;
#24257=CARTESIAN_POINT ( 'NONE',  ( 6.000000000000000888, 7.762456499804235646E-14, -134.1636751345948539 ) ) ;
#24258=CARTESIAN_POINT ( 'NONE',  ( 6.000000000000052403, -1.607695154586662678, -91.65331216351299304 ) ) ;
#24260=LINE ( 'NONE', #20131, #22722 ) ;
#24261=CARTESIAN_POINT ( 'NONE',  ( 5.196152422706629359, -2.999999999999988898, -162.2113248654052313 ) ) ;
#24264=( BOUNDED_CURVE ( )  B_SPLINE_CURVE ( 2, ( #10911, #5494, #14900, #24240, #3191, #12616, #892, #19652, #28992 ),
 .UNSPECIFIED., .F., .T. ) 
 B_SPLINE_CURVE_WITH_KNOTS ( ( 3, 2, 2, 2, 3 ),
 ( 0.4027777777777777901, 0.4037037037037037313, 0.4055555555555555580, 0.4074074074074073848, 0.4083333333333333259 ),
 .UNSPECIFIED. ) 
 CURVE ( )  GEOMETRIC_REPRESENTATION_ITEM ( )  RATIONAL_B_SPLINE_CURVE ( ( 0.9330127018922194093, 0.9330127018922194093, 1.000000000000000000, 0.8660254037844388186, 1.000000000000000000, 0.8660254037844388186, 1.000000000000000000, 0.9330127018922194093, 0.9330127018922194093 ) ) 
 REPRESENTATION_ITEM ( '' )  );
#24265=CARTESIAN_POINT ( 'NONE',  ( -6.350852961085760029, -1.281975124255709124E-13, -140.6249999999999716 ) ) ;
#24268=ORIENTED_EDGE ( 'NONE', *, *, #3195, .F. ) ;
#24269=CARTESIAN_POINT ( 'NONE',  ( -5.196152422706601826, 2.999999999999975131, -173.4613248654052313 ) ) ;
#24271=CARTESIAN_POINT ( 'NONE',  ( -6.350852961085760029, -1.281975124255709124E-13, -50.62500000000001421 ) ) ;
#24274=CARTESIAN_POINT ( 'NONE',  ( -3.464101615137725076, 5.999999999999979572, -152.5863248654051745 ) ) ;
#24280=CARTESIAN_POINT ( 'NONE',  ( 2.775557561562891351E-14, -6.250000000000061284, -93.31698729810783277 ) ) ;
#24281=CARTESIAN_POINT ( 'NONE',  ( -5.999999999999963585, -1.487416814333745711E-14, -50.91367513459483973 ) ) ;
#24287=EDGE_CURVE ( 'NONE', #14937, #21073, #7202, .T. ) ;
#24289=CARTESIAN_POINT ( 'NONE',  ( 5.999999999999949374, -1.607695154586841868, -138.1533121635129930 ) ) ;
#24290=AXIS2_PLACEMENT_3D ( 'NONE', #20836, #4680, #18847 ) ;
#24291=CARTESIAN_POINT ( 'NONE',  ( 3.175426480543072749, 5.499999999999865885, -57.12500000000004974 ) ) ;
#24294=CARTESIAN_POINT ( 'NONE',  ( -5.412658773652739619, 3.124999999999975131, -72.18301270189225249 ) ) ;
#24296=CYLINDRICAL_SURFACE ( 'NONE', #3966, 6.000000000000000888 ) ;
#24297=CARTESIAN_POINT ( 'NONE',  ( 3.464101615137757051, -5.999999999999979572, -168.3363248654051745 ) ) ;
#24299=CARTESIAN_POINT ( 'NONE',  ( 3.175426480543072749, -5.500000000000105693, -140.1250000000000000 ) ) ;
#24302=CARTESIAN_POINT ( 'NONE',  ( 2.775557561562891351E-14, -6.250000000000061284, -151.1830127018922667 ) ) ;
#24304=CARTESIAN_POINT ( 'NONE',  ( -3.175426480542816066, -5.500000000000057732, -74.37500000000000000 ) ) ;
#24305=CARTESIAN_POINT ( 'NONE',  ( -2.775557561562891351E-14, -5.500000000000115463, -56.25000000000002132 ) ) ;
#24312=EDGE_CURVE ( 'NONE', #12019, #21812, #13514, .T. ) ;
#24316=CARTESIAN_POINT ( 'NONE',  ( 0.000000000000000000, -5.999999999999991118, -121.9613248654052313 ) ) ;
#24319=CARTESIAN_POINT ( 'NONE',  ( -6.350852961085760029, -1.281975124255709124E-13, -181.1249999999999716 ) ) ;
#24321=CARTESIAN_POINT ( 'NONE',  ( -7.216878364870328078, 0.000000000000000000, -147.6919872981077901 ) ) ;
#24322=ORIENTED_EDGE ( 'NONE', *, *, #8741, .T. ) ;
#24323=CARTESIAN_POINT ( 'NONE',  ( 0.000000000000000000, 5.499999999999991118, -85.50000000000001421 ) ) ;
#24325=CARTESIAN_POINT ( 'NONE',  ( -7.216878364870328078, 0.000000000000000000, -93.05801270189225249 ) ) ;
#24331=CARTESIAN_POINT ( 'NONE',  ( 0.000000000000000000, 5.499999999999991118, -162.0000000000000284 ) ) ;
#24332=CARTESIAN_POINT ( 'NONE',  ( -5.999999999999963585, -1.487416814333745711E-14, -133.4136751345948255 ) ) ;
#24333=CARTESIAN_POINT ( 'NONE',  ( -4.763139720814407951, -2.750000000000016431, -148.0000000000000284 ) ) ;
#24334=CARTESIAN_POINT ( 'NONE',  ( 5.196152422706629359, 3.000000000000002665, -77.03867513459483973 ) ) ;
#24335=CARTESIAN_POINT ( 'NONE',  ( 6.000000000000000888, 1.743066579297358182E-13, -103.5863248654052171 ) ) ;
#24336=CARTESIAN_POINT ( 'NONE',  ( 4.763139720814407951, -2.749999999999988454, -98.00000000000002842 ) ) ;
#24339=CARTESIAN_POINT ( 'NONE',  ( -4.763139720814407951, -2.750000000000016431, -83.50000000000001421 ) ) ;
#24341=CARTESIAN_POINT ( 'NONE',  ( 6.000000000000000888, 1.743066579297358182E-13, -60.08632486540520290 ) ) ;
#24344=CARTESIAN_POINT ( 'NONE',  ( 3.464101615137852974, 5.999999999999884537, -155.8363248654052029 ) ) ;
#24346=CARTESIAN_POINT ( 'NONE',  ( 3.464101615137852974, 5.999999999999884537, -128.8363248654052029 ) ) ;
#24347=EDGE_CURVE ( 'NONE', #23842, #23894, #29088, .T. ) ;
#24349=CARTESIAN_POINT ( 'NONE',  ( 3.464101615137852974, 5.999999999999884537, -78.41367513459479710 ) ) ;
#24350=( BOUNDED_CURVE ( )  B_SPLINE_CURVE ( 2, ( #13801, #22829, #7140, #11173, #6837, #16261, #8853, #18236, #4224 ),
 .UNSPECIFIED., .F., .T. ) 
 B_SPLINE_CURVE_WITH_KNOTS ( ( 3, 2, 2, 2, 3 ),
 ( 0.08611111111111111049, 0.08703703703703703776, 0.08888888888888889228, 0.09074074074074074681, 0.09166666666666666019 ),
 .UNSPECIFIED. ) 
 CURVE ( )  GEOMETRIC_REPRESENTATION_ITEM ( )  RATIONAL_B_SPLINE_CURVE ( ( 0.9330127018922194093, 0.9330127018922194093, 1.000000000000000000, 0.8660254037844388186, 1.000000000000000000, 0.8660254037844388186, 1.000000000000000000, 0.9330127018922198534, 0.9330127018922194093 ) ) 
 REPRESENTATION_ITEM ( '' )  );
#24357=CARTESIAN_POINT ( 'NONE',  ( 0.000000000000000000, 0.000000000000000000, 0.000000000000000000 ) ) ;
#24358=ORIENTED_EDGE ( 'NONE', *, *, #10873, .T. ) ;
#24359=( BOUNDED_CURVE ( )  B_SPLINE_CURVE ( 2, ( #20447, #5840, #15420, #15887, #25186, #4152, #17561, #26878, #24585 ),
 .UNSPECIFIED., .F., .T. ) 
 B_SPLINE_CURVE_WITH_KNOTS ( ( 3, 2, 2, 2, 3 ),
 ( 0.05833333333333334814, 0.05925925925925923377, 0.06111111111111111605, 0.06296296296296299833, 0.06388888888888888395 ),
 .UNSPECIFIED. ) 
 CURVE ( )  GEOMETRIC_REPRESENTATION_ITEM ( )  RATIONAL_B_SPLINE_CURVE ( ( 0.9330127018922194093, 0.9330127018922194093, 1.000000000000000000, 0.8660254037844388186, 1.000000000000000000, 0.8660254037844388186, 1.000000000000000000, 0.9330127018922194093, 0.9330127018922194093 ) ) 
 REPRESENTATION_ITEM ( '' )  );
#24360=AXIS2_PLACEMENT_3D ( 'NONE', #14914, #3350, #24113 ) ;
#24362=ORIENTED_EDGE ( 'NONE', *, *, #25790, .T. ) ;
#24363=CARTESIAN_POINT ( 'NONE',  ( 4.763139720814407951, 2.750000000000002665, -102.2500000000000142 ) ) ;
#24366=CARTESIAN_POINT ( 'NONE',  ( -5.412658773652739619, 3.124999999999975131, -112.6830127018922383 ) ) ;
#24368=CARTESIAN_POINT ( 'NONE',  ( 5.999999999999949374, 1.607695154586804565, -111.5966878364870212 ) ) ;
#24369=CARTESIAN_POINT ( 'NONE',  ( 5.412658773652739619, 3.124999999999988898, -160.3169872981078470 ) ) ;
#24373=CARTESIAN_POINT ( 'NONE',  ( 2.775557561562891351E-14, -6.250000000000061284, -59.68301270189224539 ) ) ;
#24375=CARTESIAN_POINT ( 'NONE',  ( 6.000000000000000888, 7.762456499804234384E-14, -117.6636751345948255 ) ) ;
#24376=CARTESIAN_POINT ( 'NONE',  ( -5.999999999999963585, -1.487416814333745711E-14, -105.8363248654052313 ) ) ;
#24377=CARTESIAN_POINT ( 'NONE',  ( -2.686045755586558670, 10.67338275482133092, -19.62059632520456631 ) ) ;
#24380=CARTESIAN_POINT ( 'NONE',  ( -2.775557561562891351E-14, -5.500000000000115463, -171.7500000000000000 ) ) ;
#24382=CARTESIAN_POINT ( 'NONE',  ( -5.999999999999962697, -1.607695154586733288, -169.3466878364870354 ) ) ;
#24383=CARTESIAN_POINT ( 'NONE',  ( -3.608439182435052128, -6.250000000000110134, -172.3080127018922383 ) ) ;
#24385=CYLINDRICAL_SURFACE ( 'NONE', #17766, 6.000000000000000888 ) ;
#24386=CARTESIAN_POINT ( 'NONE',  ( 3.175426480543072749, 5.499999999999865885, -115.6249999999999858 ) ) ;
#24388=CARTESIAN_POINT ( 'NONE',  ( 3.175426480543072749, -5.500000000000105693, -108.6250000000000284 ) ) ;
#24389=CARTESIAN_POINT ( 'NONE',  ( 6.000000000000052403, -1.607695154586662678, -111.7306624327026014 ) ) ;
#24391=CARTESIAN_POINT ( 'NONE',  ( 3.464101615137757051, -5.999999999999979572, -84.33632486540518869 ) ) ;
#24397=ORIENTED_EDGE ( 'NONE', *, *, #533, .T. ) ;
#24398=CARTESIAN_POINT ( 'NONE',  ( -4.763139720814407951, -2.750000000000016431, -161.5000000000000284 ) ) ;
#24399=CARTESIAN_POINT ( 'NONE',  ( 3.464101615137852974, 5.999999999999884537, -65.83632486540516027 ) ) ;
#24400=CARTESIAN_POINT ( 'NONE',  ( 3.608439182435180470, 6.249999999999982236, -85.19198729810781856 ) ) ;
#24402=CARTESIAN_POINT ( 'NONE',  ( 6.000000000000000888, 1.743066579297358182E-13, -75.66367513459485394 ) ) ;
#24407=CARTESIAN_POINT ( 'NONE',  ( -5.412658773652684552, -3.125000000000099920, -132.5669872981078470 ) ) ;
#24410=ORIENTED_EDGE ( 'NONE', *, *, #20529, .T. ) ;
#24414=STYLED_ITEM ( 'NONE', ( #469 ), #24241 ) ;
#24416=CARTESIAN_POINT ( 'NONE',  ( 7.216878364870455975, -6.409875621278545621E-14, -70.44198729810780435 ) ) ;
#24417=CARTESIAN_POINT ( 'NONE',  ( -3.608439182435115633, 6.249999999999965361, -51.94198729810779014 ) ) ;
#24420=CARTESIAN_POINT ( 'NONE',  ( -5.196152422706601826, 2.999999999999975131, -102.9613248654052171 ) ) ;
#24421=DIRECTION ( 'NONE',  ( 1.000000000000000000, -5.551115123125773458E-17, -1.260129944081490338E-35 ) ) ;
#24422=CARTESIAN_POINT ( 'NONE',  ( 4.763139720814407951, 2.750000000000002665, -126.2500000000000284 ) ) ;
#24425=DIRECTION ( 'NONE',  ( 1.000000000000000000, -5.551115123125773458E-17, -1.260129944081490338E-35 ) ) ;
#24428=ADVANCED_FACE ( 'NONE', ( #12714 ), #24048, .T. ) ;
#24432=CARTESIAN_POINT ( 'NONE',  ( 2.775557561562891351E-14, 6.250000000000033751, -98.56698729810780435 ) ) ;
#24435=CARTESIAN_POINT ( 'NONE',  ( -6.000000000000000888, 1.067854986875958443E-15, 7.560779664488942560E-35 ) ) ;
#24436=CARTESIAN_POINT ( 'NONE',  ( 0.000000000000000000, 5.999999999999977796, -77.71132486540521711 ) ) ;
#24437=ORIENTED_EDGE ( 'NONE', *, *, #4350, .T. ) ;
#24439=CARTESIAN_POINT ( 'NONE',  ( 3.175426480543072749, -5.500000000000105693, -53.12500000000002842 ) ) ;
#24440=CARTESIAN_POINT ( 'NONE',  ( 6.000000000000000888, -1.859271017917181981E-14, -59.16367513459483263 ) ) ;
#24441=CARTESIAN_POINT ( 'NONE',  ( 3.608439182435180470, 6.249999999999982236, -74.05801270189222407 ) ) ;
#24445=DIRECTION ( 'NONE',  ( -7.147005652999508048E-36, 5.642372883946980038E-36, 1.000000000000000000 ) ) ;
#24446=EDGE_CURVE ( 'NONE', #4859, #14973, #16662, .T. ) ;
#24447=CARTESIAN_POINT ( 'NONE',  ( -3.464101615137725076, 5.999999999999979572, -79.66367513459485394 ) ) ;
#24448=FACE_OUTER_BOUND ( 'NONE', #12488, .T. ) ;
#24449=CARTESIAN_POINT ( 'NONE',  ( 3.175426480543072749, -5.500000000000105693, -132.6250000000000284 ) ) ;
#24450=CARTESIAN_POINT ( 'NONE',  ( 6.000000000000000888, -1.607695154586752384, -177.1533121635130499 ) ) ;
#24451=CARTESIAN_POINT ( 'NONE',  ( -5.999999999999956479, -1.607695154586745057, -71.26933756729742697 ) ) ;
#24452=CARTESIAN_POINT ( 'NONE',  ( -3.175426480542816066, 5.499999999999865885, -64.37500000000001421 ) ) ;
#24454=CARTESIAN_POINT ( 'NONE',  ( 6.350852961086080661, -9.614813431917819062E-14, -57.37500000000004974 ) ) ;
#24456=EDGE_LOOP ( 'NONE', ( #10919, #13849, #22085, #5346 ) ) ;
#24458=CARTESIAN_POINT ( 'NONE',  ( 6.000000000000000888, 1.743066579297358182E-13, -102.6636751345948397 ) ) ;
#24465=ORIENTED_EDGE ( 'NONE', *, *, #4660, .F. ) ;
#24467=CARTESIAN_POINT ( 'NONE',  ( -4.763139720814407951, -2.750000000000016431, -148.0000000000000284 ) ) ;
#24470=CARTESIAN_POINT ( 'NONE',  ( -3.608439182435115633, 6.249999999999965361, -144.9419872981078470 ) ) ;
#24471=CARTESIAN_POINT ( 'NONE',  ( -6.350852961085760029, -1.281975124255709124E-13, -77.62500000000001421 ) ) ;
#24474=CARTESIAN_POINT ( 'NONE',  ( -5.412658773652684552, -3.125000000000099920, -94.43301270189225249 ) ) ;
#24476=CARTESIAN_POINT ( 'NONE',  ( -5.196152422706573404, -3.000000000000002665, -128.2113248654052029 ) ) ;
#24482=CARTESIAN_POINT ( 'NONE',  ( 3.175426480543072749, 5.499999999999865885, -156.1250000000000000 ) ) ;
#24484=CARTESIAN_POINT ( 'NONE',  ( -3.175426480542816510, -5.500000000000057732, -149.3750000000000284 ) ) ;
#24486=AXIS2_PLACEMENT_3D ( 'NONE', #11353, #10892, #20699 ) ;
#24487=CARTESIAN_POINT ( 'NONE',  ( -3.175426480542816066, 5.499999999999865885, -92.87500000000002842 ) ) ;
#24489=ADVANCED_FACE ( 'NONE', ( #28788 ), #14702, .T. ) ;
#24490=CARTESIAN_POINT ( 'NONE',  ( 4.763139720814407951, -2.749999999999988454, -78.50000000000001421 ) ) ;
#24498=CARTESIAN_POINT ( 'NONE',  ( -5.196152422706573404, -3.000000000000002665, -165.7113248654051745 ) ) ;
#24500=CARTESIAN_POINT ( 'NONE',  ( -5.999999999999963585, -1.487416814333745711E-14, -138.8363248654052597 ) ) ;
#24501=ORIENTED_EDGE ( 'NONE', *, *, #3958, .F. ) ;
#24502=CARTESIAN_POINT ( 'NONE',  ( -5.999999999999963585, 3.021315404115421074E-15, -178.4136751345948255 ) ) ;
#24503=CARTESIAN_POINT ( 'NONE',  ( -5.196152422706573404, -3.000000000000002665, -157.2886751345948824 ) ) ;
#24505=CARTESIAN_POINT ( 'NONE',  ( 0.000000000000000000, -5.999999999999991118, -115.9613248654052313 ) ) ;
#24507=ORIENTED_EDGE ( 'NONE', *, *, #6658, .T. ) ;
#24508=CARTESIAN_POINT ( 'NONE',  ( 0.000000000000000000, 5.499999999999991118, -102.0000000000000284 ) ) ;
#24509=CYLINDRICAL_SURFACE ( 'NONE', #9703, 6.000000000000000888 ) ;
#24510=CARTESIAN_POINT ( 'NONE',  ( -3.608439182435052128, -6.250000000000110134, -112.3080127018922241 ) ) ;
#24512=CARTESIAN_POINT ( 'NONE',  ( 5.196152422706629359, 3.000000000000002665, -111.5386751345948113 ) ) ;
#24517=CARTESIAN_POINT ( 'NONE',  ( 2.775557561562891351E-14, 6.250000000000033751, -54.43301270189226670 ) ) ;
#24518=ORIENTED_EDGE ( 'NONE', *, *, #6714, .F. ) ;
#24520=CARTESIAN_POINT ( 'NONE',  ( 6.000000000000026645, -1.607695154586707753, -119.2306624327025872 ) ) ;
#24521=CARTESIAN_POINT ( 'NONE',  ( -3.464101615137725076, 5.999999999999979572, -136.0863248654051745 ) ) ;
#24523=CARTESIAN_POINT ( 'NONE',  ( -4.763139720814407951, -2.750000000000016431, -167.4999999999999716 ) ) ;
#24525=CARTESIAN_POINT ( 'NONE',  ( 7.216878364870455975, -6.409875621278545621E-14, -170.3080127018922667 ) ) ;
#24526=CARTESIAN_POINT ( 'NONE',  ( -5.999999999999919176, 1.607695154586804565, -47.98066243270260856 ) ) ;
#24528=CARTESIAN_POINT ( 'NONE',  ( 0.000000000000000000, 5.499999999999991118, -120.0000000000000000 ) ) ;
#24530=( BOUNDED_CURVE ( )  B_SPLINE_CURVE ( 2, ( #21952, #2599, #2739, #12166, #24093, #5040, #885, #28836, #16773 ),
 .UNSPECIFIED., .F., .T. ) 
 B_SPLINE_CURVE_WITH_KNOTS ( ( 3, 2, 2, 2, 3 ),
 ( 0.5972222222222222099, 0.5981481481481480955, 0.5999999999999999778, 0.6018518518518518601, 0.6027777777777777457 ),
 .UNSPECIFIED. ) 
 CURVE ( )  GEOMETRIC_REPRESENTATION_ITEM ( )  RATIONAL_B_SPLINE_CURVE ( ( 0.9330127018922194093, 0.9330127018922194093, 1.000000000000000000, 0.8660254037844388186, 1.000000000000000000, 0.8660254037844388186, 1.000000000000000000, 0.9330127018922234061, 0.9330127018922194093 ) ) 
 REPRESENTATION_ITEM ( '' )  );
#24531=CARTESIAN_POINT ( 'NONE',  ( 0.000000000000000000, 5.499999999999991118, -102.0000000000000284 ) ) ;
#24533=CARTESIAN_POINT ( 'NONE',  ( 6.000000000000000888, 1.743066579297358182E-13, -111.6636751345948255 ) ) ;
#24535=CARTESIAN_POINT ( 'NONE',  ( 0.000000000000000000, -5.999999999999991118, -84.46132486540524553 ) ) ;
#24540=AXIS2_PLACEMENT_3D ( 'NONE', #19080, #23527, #18935 ) ;
#24542=CARTESIAN_POINT ( 'NONE',  ( -3.175426480542816510, 5.499999999999865885, -161.8750000000000568 ) ) ;
#24544=CARTESIAN_POINT ( 'NONE',  ( 7.216878364870455975, -6.409875621278545621E-14, -77.94198729810779014 ) ) ;
#24545=CARTESIAN_POINT ( 'NONE',  ( -3.464101615137757051, -5.999999999999979572, -129.5863248654052029 ) ) ;
#24546=EDGE_LOOP ( 'NONE', ( #15381, #1787, #13961, #10832 ) ) ;
#24547=CARTESIAN_POINT ( 'NONE',  ( -5.196152422706601826, 2.999999999999975131, -144.0386751345948539 ) ) ;
#24548=ORIENTED_EDGE ( 'NONE', *, *, #3648, .T. ) ;
#24549=ORIENTED_EDGE ( 'NONE', *, *, #13108, .F. ) ;
#24551=CARTESIAN_POINT ( 'NONE',  ( -3.608439182435052128, -6.250000000000110134, -136.3080127018922667 ) ) ;
#24553=CARTESIAN_POINT ( 'NONE',  ( 5.412658773652739619, 3.124999999999988898, -127.3169872981078043 ) ) ;
#24554=CARTESIAN_POINT ( 'NONE',  ( -4.763139720814407951, -2.750000000000016431, -175.0000000000000568 ) ) ;
#24555=CARTESIAN_POINT ( 'NONE',  ( -3.464101615137757051, -5.999999999999979572, -167.6636751345948255 ) ) ;
#24560=CARTESIAN_POINT ( 'NONE',  ( -5.999999999999963585, -1.487416814333745711E-14, -171.8363248654052313 ) ) ;
#24561=DIRECTION ( 'NONE',  ( 1.000000000000000000, -5.551115123125773458E-17, -1.260129944081490338E-35 ) ) ;
#24565=CARTESIAN_POINT ( 'NONE',  ( -3.464101615137757051, -5.999999999999979572, -107.6636751345948539 ) ) ;
#24567=CARTESIAN_POINT ( 'NONE',  ( 2.775557561562891351E-14, 6.250000000000033751, -67.06698729810783277 ) ) ;
#24568=CARTESIAN_POINT ( 'NONE',  ( 3.608439182435180470, -6.249999999999997335, -54.19198729810779724 ) ) ;
#24572=CARTESIAN_POINT ( 'NONE',  ( 3.464101615137852974, 5.999999999999884537, -127.9136751345948113 ) ) ;
#24573=CARTESIAN_POINT ( 'NONE',  ( 0.000000000000000000, 5.499999999999991118, -126.0000000000000000 ) ) ;
#24577=CARTESIAN_POINT ( 'NONE',  ( -5.196152422706601826, 2.999999999999975131, -119.4613248654052313 ) ) ;
#24578=CARTESIAN_POINT ( 'NONE',  ( 5.196152422706629359, 3.000000000000002665, -97.46132486540525974 ) ) ;
#24579=CARTESIAN_POINT ( 'NONE',  ( 0.000000000000000000, -5.999999999999991118, -100.0386751345948539 ) ) ;
#24580=CARTESIAN_POINT ( 'NONE',  ( 5.196152422706629359, -2.999999999999988898, -144.2113248654052313 ) ) ;
#24583=CARTESIAN_POINT ( 'NONE',  ( 5.412658773652712085, -3.125000000000086153, -94.56698729810780435 ) ) ;
#24585=CARTESIAN_POINT ( 'NONE',  ( -5.999999999999963585, -1.487416814333745711E-14, -54.83632486540523132 ) ) ;
#24589=EDGE_CURVE ( 'NONE', #17182, #20541, #4052, .T. ) ;
#24590=VERTEX_POINT ( 'NONE', #22815 ) ;
#24591=VECTOR ( 'NONE', #14243, 1000.000000000000000 ) ;
#24593=CARTESIAN_POINT ( 'NONE',  ( -4.763139720814407951, 2.749999999999946709, -52.25000000000002132 ) ) ;
#24594=CARTESIAN_POINT ( 'NONE',  ( 6.000000000000000888, -1.607695154586752384, -59.23066243270262277 ) ) ;
#24595=CARTESIAN_POINT ( 'NONE',  ( 6.000000000000000888, 1.743066579297358182E-13, -62.16367513459481131 ) ) ;
#24596=CARTESIAN_POINT ( 'NONE',  ( -7.216878364870328078, 0.000000000000000000, -72.05801270189223828 ) ) ;
#24597=ADVANCED_FACE ( 'NONE', ( #22520 ), #17928, .F. ) ;
#24598=CARTESIAN_POINT ( 'NONE',  ( -5.999999999999964473, 9.063946212346262433E-15, -173.3363248654052597 ) ) ;
#24600=CARTESIAN_POINT ( 'NONE',  ( 0.000000000000000000, 0.000000000000000000, 0.000000000000000000 ) ) ;
#24601=CARTESIAN_POINT ( 'NONE',  ( 0.000000000000000000, 0.000000000000000000, 0.000000000000000000 ) ) ;
#24602=CARTESIAN_POINT ( 'NONE',  ( -5.999999999999962697, 3.323446944526963891E-14, -152.9136751345948255 ) ) ;
#24604=CARTESIAN_POINT ( 'NONE',  ( 0.000000000000000000, 5.499999999999991118, -132.0000000000000000 ) ) ;
#24606=CYLINDRICAL_SURFACE ( 'NONE', #17008, 6.000000000000000888 ) ;
#24607=CARTESIAN_POINT ( 'NONE',  ( -5.196152422706601826, 2.999999999999975131, -177.9613248654052313 ) ) ;
#24608=VERTEX_POINT ( 'NONE', #15941 ) ;
#24609=CARTESIAN_POINT ( 'NONE',  ( -3.175426480542816066, -5.500000000000057732, -66.87500000000002842 ) ) ;
#24610=CARTESIAN_POINT ( 'NONE',  ( -3.175426480542816510, 5.499999999999865885, -59.87500000000005684 ) ) ;
#24624=ADVANCED_FACE ( 'NONE', ( #8521 ), #1914, .T. ) ;
#24625=CARTESIAN_POINT ( 'NONE',  ( -3.175426480542816510, 5.499999999999865885, -143.8750000000000000 ) ) ;
#24626=( BOUNDED_CURVE ( )  B_SPLINE_CURVE ( 2, ( #549, #9938, #10246, #5594, #19314, #28634, #7605, #17018, #2997 ),
 .UNSPECIFIED., .F., .T. ) 
 B_SPLINE_CURVE_WITH_KNOTS ( ( 3, 2, 2, 2, 3 ),
 ( 0.5861111111111111382, 0.5870370370370370239, 0.5888888888888889062, 0.5907407407407407884, 0.5916666666666666741 ),
 .UNSPECIFIED. ) 
 CURVE ( )  GEOMETRIC_REPRESENTATION_ITEM ( )  RATIONAL_B_SPLINE_CURVE ( ( 0.9330127018922194093, 0.9330127018922194093, 1.000000000000000000, 0.8660254037844388186, 1.000000000000000000, 0.8660254037844388186, 1.000000000000000000, 0.9330127018922194093, 0.9330127018922194093 ) ) 
 REPRESENTATION_ITEM ( '' )  );
#24629=CARTESIAN_POINT ( 'NONE',  ( 3.608439182435180470, 6.249999999999982236, -149.6919872981077901 ) ) ;
#24630=CARTESIAN_POINT ( 'NONE',  ( 4.763139720814407951, 2.750000000000002665, -70.75000000000002842 ) ) ;
#24633=CARTESIAN_POINT ( 'NONE',  ( -7.216878364870328078, 0.000000000000000000, -94.55801270189226670 ) ) ;
#24634=EDGE_CURVE ( 'NONE', #29849, #2905, #14983, .T. ) ;
#24637=CARTESIAN_POINT ( 'NONE',  ( -4.767949350811372611, -9.915884935901891239, -28.66271918150853537 ) ) ;
#24638=CARTESIAN_POINT ( 'NONE',  ( 0.000000000000000000, 0.000000000000000000, 0.000000000000000000 ) ) ;
#24640=CARTESIAN_POINT ( 'NONE',  ( -5.999999999999963585, 8.134310703387671600E-14, -131.9136751345948255 ) ) ;
#24642=CARTESIAN_POINT ( 'NONE',  ( -2.775557561562891351E-14, -5.500000000000115463, -155.2500000000000000 ) ) ;
#24644=CARTESIAN_POINT ( 'NONE',  ( 4.763139720814407951, -2.749999999999988454, -143.0000000000000284 ) ) ;
#24646=CARTESIAN_POINT ( 'NONE',  ( -4.763139720814407951, -2.750000000000016431, -83.50000000000001421 ) ) ;
#24647=CARTESIAN_POINT ( 'NONE',  ( 0.000000000000000000, 0.000000000000000000, 0.000000000000000000 ) ) ;
#24649=CARTESIAN_POINT ( 'NONE',  ( -3.175426480542816510, -5.500000000000057732, -78.87500000000002842 ) ) ;
#24650=CARTESIAN_POINT ( 'NONE',  ( 3.464101615137757051, -5.999999999999979572, -74.41367513459483973 ) ) ;
#24652=CARTESIAN_POINT ( 'NONE',  ( 5.999999999999949374, 1.607695154586804565, -165.0193375672974128 ) ) ;
#24653=CARTESIAN_POINT ( 'NONE',  ( -5.999999999999963585, 1.780251999655701777E-13, -108.8363248654052313 ) ) ;
#24654=CARTESIAN_POINT ( 'NONE',  ( -5.196152422706573404, -3.000000000000002665, -149.7886751345948255 ) ) ;
#24656=CARTESIAN_POINT ( 'NONE',  ( 3.464101615137852974, 5.999999999999884537, -134.8363248654052313 ) ) ;
#24657=DIRECTION ( 'NONE',  ( 1.000000000000000000, -5.551115123125782702E-17, 0.000000000000000000 ) ) ;
#24661=CARTESIAN_POINT ( 'NONE',  ( 6.000000000000000888, 1.743066579297358182E-13, -56.16367513459481842 ) ) ;
#24664=EDGE_CURVE ( 'NONE', #10035, #10886, #25681, .T. ) ;
#24666=ORIENTED_EDGE ( 'NONE', *, *, #15317, .T. ) ;
#24667=CARTESIAN_POINT ( 'NONE',  ( 4.763139720814407951, -2.749999999999988454, -99.50000000000002842 ) ) ;
#24669=EDGE_CURVE ( 'NONE', #21789, #6076, #18437, .T. ) ;
#24670=CARTESIAN_POINT ( 'NONE',  ( 5.412658773652739619, 3.124999999999988898, -116.1830127018922383 ) ) ;
#24674=CARTESIAN_POINT ( 'NONE',  ( -11.00000000000000000, 1.957734142605923910E-15, -43.99152654425658682 ) ) ;
#24676=( BOUNDED_CURVE ( )  B_SPLINE_CURVE ( 2, ( #22236, #1166, #10573, #19926, #29273, #9967, #5178, #23944, #2881 ),
 .UNSPECIFIED., .F., .F. ) 
 B_SPLINE_CURVE_WITH_KNOTS ( ( 3, 2, 2, 2, 3 ),
 ( 0.8972222222222222543, 0.8981481481481481399, 0.9000000000000000222, 0.9018518518518519045, 0.9027777777777777901 ),
 .UNSPECIFIED. ) 
 CURVE ( )  GEOMETRIC_REPRESENTATION_ITEM ( )  RATIONAL_B_SPLINE_CURVE ( ( 0.9330127018922194093, 0.9330127018922234061, 1.000000000000000000, 0.8660254037844388186, 1.000000000000000000, 0.8660254037844388186, 1.000000000000000000, 0.9330127018922194093, 0.9330127018922194093 ) ) 
 REPRESENTATION_ITEM ( '' )  );
#24677=CARTESIAN_POINT ( 'NONE',  ( 5.412658773652712085, -3.125000000000086153, -48.93301270189220986 ) ) ;
#24678=ORIENTED_EDGE ( 'NONE', *, *, #22012, .F. ) ;
#24680=CARTESIAN_POINT ( 'NONE',  ( -5.196152422706601826, 2.999999999999975131, -99.03867513459485394 ) ) ;
#24681=CARTESIAN_POINT ( 'NONE',  ( -6.000000000000000888, 1.067854986875958443E-15, 7.560779664488942560E-35 ) ) ;
#24683=CARTESIAN_POINT ( 'NONE',  ( 0.000000000000000000, 5.499999999999991118, -174.0000000000000568 ) ) ;
#24685=CARTESIAN_POINT ( 'NONE',  ( -5.999999999999963585, 1.780251999655701777E-13, -107.3363248654052455 ) ) ;
#24686=CARTESIAN_POINT ( 'NONE',  ( 5.412658773652739619, 3.124999999999988898, -171.6830127018922383 ) ) ;
#24688=CARTESIAN_POINT ( 'NONE',  ( -2.775557561562891351E-14, -5.500000000000115463, -108.7500000000000142 ) ) ;
#24689=CYLINDRICAL_SURFACE ( 'NONE', #9509, 6.000000000000000888 ) ;
#24690=CARTESIAN_POINT ( 'NONE',  ( 0.000000000000000000, 5.499999999999991118, -105.0000000000000426 ) ) ;
#24692=CARTESIAN_POINT ( 'NONE',  ( 3.464101615137852974, 5.999999999999884537, -162.4136751345947971 ) ) ;
#24693=ORIENTED_EDGE ( 'NONE', *, *, #22793, .F. ) ;
#24695=FACE_OUTER_BOUND ( 'NONE', #18739, .T. ) ;
#24698=CARTESIAN_POINT ( 'NONE',  ( -5.196152422706573404, -3.000000000000002665, -146.2113248654052313 ) ) ;
#24700=CARTESIAN_POINT ( 'NONE',  ( 3.175426480543072749, 5.499999999999865885, -162.1250000000000284 ) ) ;
#24702=CARTESIAN_POINT ( 'NONE',  ( 5.412658773652739619, 3.124999999999988898, -85.31698729810783277 ) ) ;
#24703=EDGE_CURVE ( 'NONE', #2458, #799, #20979, .T. ) ;
#24704=CARTESIAN_POINT ( 'NONE',  ( 5.196152422706629359, -2.999999999999988898, -102.7886751345948255 ) ) ;
#24709=CARTESIAN_POINT ( 'NONE',  ( -2.775557561562891351E-14, -5.500000000000115463, -132.7500000000000284 ) ) ;
#24711=CARTESIAN_POINT ( 'NONE',  ( 3.608439182435180470, -6.249999999999997335, -136.0580127018922099 ) ) ;
#24712=ORIENTED_EDGE ( 'NONE', *, *, #1538, .T. ) ;
#24713=CARTESIAN_POINT ( 'NONE',  ( 5.196152422706629359, -2.999999999999988898, -57.21132486540525264 ) ) ;
#24714=CARTESIAN_POINT ( 'NONE',  ( -3.608439182435115633, 6.249999999999965361, -120.9419872981077901 ) ) ;
#24716=CARTESIAN_POINT ( 'NONE',  ( -3.175426480542816510, -5.500000000000057732, -168.8750000000000568 ) ) ;
#24717=CARTESIAN_POINT ( 'NONE',  ( 3.464101615137852974, 5.999999999999884537, -175.3363248654051461 ) ) ;
#24718=CARTESIAN_POINT ( 'NONE',  ( -3.464101615137725076, 5.999999999999979572, -47.58632486540521711 ) ) ;
#24719=ORIENTED_EDGE ( 'NONE', *, *, #14704, .F. ) ;
#24721=CARTESIAN_POINT ( 'NONE',  ( -5.999999999999962697, 3.323446944526963260E-14, -147.8363248654052313 ) ) ;
#24722=( BOUNDED_CURVE ( )  B_SPLINE_CURVE ( 2, ( #23086, #11897, #2028, #20780, #9090, #18486, #16200, #25671, #9555 ),
 .UNSPECIFIED., .F., .T. ) 
 B_SPLINE_CURVE_WITH_KNOTS ( ( 3, 2, 2, 2, 3 ),
 ( 0.3250000000000000111, 0.3259259259259259522, 0.3277777777777777790, 0.3296296296296296058, 0.3305555555555555469 ),
 .UNSPECIFIED. ) 
 CURVE ( )  GEOMETRIC_REPRESENTATION_ITEM ( )  RATIONAL_B_SPLINE_CURVE ( ( 0.9330127018922194093, 0.9330127018922194093, 1.000000000000000000, 0.8660254037844388186, 1.000000000000000000, 0.8660254037844388186, 1.000000000000000000, 0.9330127018922194093, 0.9330127018922194093 ) ) 
 REPRESENTATION_ITEM ( '' )  );
#24723=CARTESIAN_POINT ( 'NONE',  ( 6.000000000000103917, -1.607695154586573416, -117.1533121635129788 ) ) ;
#24724=FACE_OUTER_BOUND ( 'NONE', #12999, .T. ) ;
#24727=CARTESIAN_POINT ( 'NONE',  ( 2.775557561562891351E-14, -6.250000000000061284, -64.81698729810780435 ) ) ;
#24728=CARTESIAN_POINT ( 'NONE',  ( 3.608439182435180470, -6.249999999999997335, -52.69198729810779014 ) ) ;
#24729=CARTESIAN_POINT ( 'NONE',  ( 6.000000000000000888, -1.607695154586752384, -120.7306624327026157 ) ) ;
#24730=DIRECTION ( 'NONE',  ( 1.000000000000000000, -5.551115123125774690E-17, -1.260129944081490338E-35 ) ) ;
#24731=CARTESIAN_POINT ( 'NONE',  ( 3.464101615137852974, 5.999999999999884537, -55.91367513459481131 ) ) ;
#24732=CARTESIAN_POINT ( 'NONE',  ( 6.350852961086080661, -9.614813431917819062E-14, -129.3750000000000284 ) ) ;
#24733=( BOUNDED_CURVE ( )  B_SPLINE_CURVE ( 2, ( #11722, #20764, #2321, #16336, #9074, #18467, #13727, #8932, #25810 ),
 .UNSPECIFIED., .F., .T. ) 
 B_SPLINE_CURVE_WITH_KNOTS ( ( 3, 2, 2, 2, 3 ),
 ( 0.4416666666666667074, 0.4425925925925925930, 0.4444444444444444198, 0.4462962962962963021, 0.4472222222222221877 ),
 .UNSPECIFIED. ) 
 CURVE ( )  GEOMETRIC_REPRESENTATION_ITEM ( )  RATIONAL_B_SPLINE_CURVE ( ( 0.9330127018922194093, 0.9330127018922214077, 1.000000000000000000, 0.8660254037844388186, 1.000000000000000000, 0.8660254037844388186, 1.000000000000000000, 0.9330127018922214077, 0.9330127018922194093 ) ) 
 REPRESENTATION_ITEM ( '' )  );
#24734=CARTESIAN_POINT ( 'NONE',  ( -5.999999999999971578, 1.607695154586715303, -50.40331216351300725 ) ) ;
#24736=ORIENTED_EDGE ( 'NONE', *, *, #29228, .T. ) ;
#24740=DIRECTION ( 'NONE',  ( -7.147005652999508048E-36, 5.642372883946980038E-36, 1.000000000000000000 ) ) ;
#24745=CARTESIAN_POINT ( 'NONE',  ( 3.608439182435180470, 6.249999999999982236, -115.1919872981078328 ) ) ;
#24746=EDGE_CURVE ( 'NONE', #16950, #7068, #27196, .T. ) ;
#24748=EDGE_CURVE ( 'NONE', #17985, #23417, #13335, .T. ) ;
#24749=CARTESIAN_POINT ( 'NONE',  ( -5.999999999999919176, 1.607695154586804565, -90.90331216351299304 ) ) ;
#24751=ORIENTED_EDGE ( 'NONE', *, *, #30195, .T. ) ;
#24756=CARTESIAN_POINT ( 'NONE',  ( 3.464101615137757051, -5.999999999999979572, -138.3363248654051745 ) ) ;
#24757=CARTESIAN_POINT ( 'NONE',  ( 0.000000000000000000, 5.499999999999991118, -51.00000000000004263 ) ) ;
#24759=CARTESIAN_POINT ( 'NONE',  ( 5.196152422706629359, -2.999999999999988898, -59.28867513459484684 ) ) ;
#24760=CARTESIAN_POINT ( 'NONE',  ( 0.000000000000000000, 5.999999999999977796, -61.78867513459485394 ) ) ;
#24761=CARTESIAN_POINT ( 'NONE',  ( 2.775557561562891351E-14, 6.250000000000033751, -76.93301270189223828 ) ) ;
#24764=DIRECTION ( 'NONE',  ( -7.147005652999508048E-36, 5.642372883946980038E-36, 1.000000000000000000 ) ) ;
#24765=( NAMED_UNIT ( * ) SI_UNIT ( $, .STERADIAN. ) SOLID_ANGLE_UNIT ( ) );
#24766=CARTESIAN_POINT ( 'NONE',  ( -5.999999999999963585, 8.134310703387671600E-14, -125.9136751345948397 ) ) ;
#24767=CARTESIAN_POINT ( 'NONE',  ( -3.175426480542816066, 5.499999999999865885, -131.8750000000000284 ) ) ;
#24769=CARTESIAN_POINT ( 'NONE',  ( -3.608439182435115633, 6.249999999999965361, -148.8080127018922667 ) ) ;
#24770=LINE ( 'NONE', #20013, #9138 ) ;
#24771=VERTEX_POINT ( 'NONE', #28457 ) ;
#24773=CARTESIAN_POINT ( 'NONE',  ( 4.763139720814407951, -2.749999999999988454, -60.50000000000000000 ) ) ;
#24774=CARTESIAN_POINT ( 'NONE',  ( 0.000000000000000000, 5.999999999999977796, -172.2113248654052597 ) ) ;
#24781=EDGE_CURVE ( 'NONE', #269, #11050, #22726, .T. ) ;
#24782=ORIENTED_EDGE ( 'NONE', *, *, #8154, .F. ) ;
#24785=ORIENTED_EDGE ( 'NONE', *, *, #7678, .T. ) ;
#24787=CARTESIAN_POINT ( 'NONE',  ( 6.350852961086080661, -9.614813431917819062E-14, -145.8750000000000284 ) ) ;
#24791=CARTESIAN_POINT ( 'NONE',  ( -3.175426480542816510, 5.499999999999865885, -71.87500000000000000 ) ) ;
#24792=CARTESIAN_POINT ( 'NONE',  ( 2.775557561562891351E-14, -6.250000000000061284, -91.18301270189222407 ) ) ;
#24795=CARTESIAN_POINT ( 'NONE',  ( -5.999999999999962697, 3.323446944526963891E-14, -151.4136751345948255 ) ) ;
#24797=CARTESIAN_POINT ( 'NONE',  ( 5.196152422706629359, -2.999999999999988898, -64.71132486540520290 ) ) ;
#24798=CARTESIAN_POINT ( 'NONE',  ( -3.175426480542816066, -5.500000000000057732, -153.8749999999999716 ) ) ;
#24803=EDGE_CURVE ( 'NONE', #15423, #26042, #9001, .T. ) ;
#24804=CARTESIAN_POINT ( 'NONE',  ( 6.350852961086080661, -9.614813431917819062E-14, -88.87500000000001421 ) ) ;
#24805=CARTESIAN_POINT ( 'NONE',  ( -5.999999999999982236, -1.607695154586700426, -140.8466878364870354 ) ) ;
#24806=CARTESIAN_POINT ( 'NONE',  ( 6.000000000000000888, -1.607695154586752384, -130.6533121635130215 ) ) ;
#24807=CARTESIAN_POINT ( 'NONE',  ( 3.175426480543072749, 5.499999999999865885, -82.62500000000004263 ) ) ;
#24808=DIRECTION ( 'NONE',  ( -7.147005652999508048E-36, 5.642372883946980038E-36, 1.000000000000000000 ) ) ;
#24812=CARTESIAN_POINT ( 'NONE',  ( -5.999999999999963585, -1.487416814333745711E-14, -165.8363248654052029 ) ) ;
#24814=CARTESIAN_POINT ( 'NONE',  ( -5.999999999999964473, 1.607695154586726405, -173.9806624327026157 ) ) ;
#24815=( BOUNDED_CURVE ( )  B_SPLINE_CURVE ( 2, ( #12913, #1179, #29287, #8244, #24842, #17657, #26981, #15520, #5945 ),
 .UNSPECIFIED., .F., .T. ) 
 B_SPLINE_CURVE_WITH_KNOTS ( ( 3, 2, 2, 2, 3 ),
 ( 0.3027777777777777013, 0.3037037037037036979, 0.3055555555555555802, 0.3074074074074074625, 0.3083333333333333481 ),
 .UNSPECIFIED. ) 
 CURVE ( )  GEOMETRIC_REPRESENTATION_ITEM ( )  RATIONAL_B_SPLINE_CURVE ( ( 0.9330127018922194093, 0.9330127018922154125, 1.000000000000000000, 0.8660254037844388186, 1.000000000000000000, 0.8660254037844388186, 1.000000000000000000, 0.9330127018922194093, 0.9330127018922194093 ) ) 
 REPRESENTATION_ITEM ( '' )  );
#24820=VECTOR ( 'NONE', #1479, 1000.000000000000000 ) ;
#24823=VERTEX_POINT ( 'NONE', #19714 ) ;
#24825=CARTESIAN_POINT ( 'NONE',  ( 4.763139720814407951, -2.749999999999988454, -95.00000000000002842 ) ) ;
#24826=CARTESIAN_POINT ( 'NONE',  ( -3.464101615137725076, 5.999999999999979572, -70.66367513459481131 ) ) ;
#24827=CARTESIAN_POINT ( 'NONE',  ( -3.608439182435052128, -6.250000000000110134, -113.8080127018922241 ) ) ;
#24828=ORIENTED_EDGE ( 'NONE', *, *, #28948, .T. ) ;
#24829=CARTESIAN_POINT ( 'NONE',  ( -6.000000000000000888, 1.067854986875958443E-15, 7.560779664488942560E-35 ) ) ;
#24830=CARTESIAN_POINT ( 'NONE',  ( -5.412658773652739619, 3.124999999999975131, -54.18301270189223828 ) ) ;
#24834=CARTESIAN_POINT ( 'NONE',  ( -4.763139720814407951, -2.750000000000016431, -170.4999999999999716 ) ) ;
#24837=CARTESIAN_POINT ( 'NONE',  ( -3.608439182435052128, -6.250000000000110134, -158.8080127018922383 ) ) ;
#24840=CARTESIAN_POINT ( 'NONE',  ( -3.175426480542816066, 5.499999999999865885, -112.3750000000000568 ) ) ;
#24841=CARTESIAN_POINT ( 'NONE',  ( -3.175426480542816510, 5.499999999999865885, -109.3750000000000284 ) ) ;
#24842=CARTESIAN_POINT ( 'NONE',  ( 0.000000000000000000, -5.999999999999991118, -87.46132486540525974 ) ) ;
#24843=CARTESIAN_POINT ( 'NONE',  ( -3.464101615137725076, 5.999999999999979572, -145.0863248654052029 ) ) ;
#24849=CARTESIAN_POINT ( 'NONE',  ( -5.999999999999956479, -1.607695154586745057, -134.2693375672974412 ) ) ;
#24850=EDGE_CURVE ( 'NONE', #10258, #17334, #17269, .T. ) ;
#24851=VERTEX_POINT ( 'NONE', #26556 ) ;
#24852=CARTESIAN_POINT ( 'NONE',  ( 0.000000000000000000, 5.999999999999977796, -156.2886751345948824 ) ) ;
#24853=CARTESIAN_POINT ( 'NONE',  ( -7.216878364870328078, 0.000000000000000000, -83.19198729810780435 ) ) ;
#24854=CARTESIAN_POINT ( 'NONE',  ( 0.000000000000000000, -5.999999999999991118, -129.4613248654052313 ) ) ;
#24856=CARTESIAN_POINT ( 'NONE',  ( -6.000000000000007105, -1.607695154586655129, -65.84668783648703538 ) ) ;
#24860=CARTESIAN_POINT ( 'NONE',  ( 0.000000000000000000, 5.499999999999991118, -123.0000000000000000 ) ) ;
#24861=CARTESIAN_POINT ( 'NONE',  ( -3.608439182435115633, 6.249999999999965361, -135.3080127018922667 ) ) ;
#24864=CARTESIAN_POINT ( 'NONE',  ( 5.412658773652712085, -3.125000000000086153, -123.0669872981078328 ) ) ;
#24865=CARTESIAN_POINT ( 'NONE',  ( -4.763139720814407951, -2.750000000000016431, -170.4999999999999716 ) ) ;
#24871=CARTESIAN_POINT ( 'NONE',  ( -5.196152422706573404, -3.000000000000002665, -117.7113248654052597 ) ) ;
#24873=CARTESIAN_POINT ( 'NONE',  ( 0.000000000000000000, 0.000000000000000000, 0.000000000000000000 ) ) ;
#24875=CARTESIAN_POINT ( 'NONE',  ( 2.775557561562891351E-14, 6.250000000000033751, -70.06698729810784698 ) ) ;
#24876=DIRECTION ( 'NONE',  ( -7.147005652999508048E-36, 5.642372883946980038E-36, 1.000000000000000000 ) ) ;
#24877=CARTESIAN_POINT ( 'NONE',  ( 4.763139720814407951, 2.750000000000002665, -48.25000000000001421 ) ) ;
#24881=CARTESIAN_POINT ( 'NONE',  ( -4.763139720814407951, -2.750000000000016431, -133.0000000000000000 ) ) ;
#24882=ORIENTED_EDGE ( 'NONE', *, *, #10693, .T. ) ;
#24884=DIRECTION ( 'NONE',  ( -7.147005652999508048E-36, 5.642372883946980038E-36, 1.000000000000000000 ) ) ;
#24885=CARTESIAN_POINT ( 'NONE',  ( -5.999999999999962697, 3.323446944526963891E-14, -160.4136751345948255 ) ) ;
#24889=CARTESIAN_POINT ( 'NONE',  ( 6.000000000000000888, 7.762456499804235646E-14, -133.5863248654052029 ) ) ;
#24891=CARTESIAN_POINT ( 'NONE',  ( 2.775557561562891351E-14, -6.250000000000061284, -117.3169872981078043 ) ) ;
#24899=ORIENTED_EDGE ( 'NONE', *, *, #1925, .F. ) ;
#24903=CARTESIAN_POINT ( 'NONE',  ( -5.999999999999944933, 1.607695154586759934, -119.9806624327026157 ) ) ;
#24905=CARTESIAN_POINT ( 'NONE',  ( 2.775557561562891351E-14, 6.250000000000033751, -64.93301270189222407 ) ) ;
#24907=CYLINDRICAL_SURFACE ( 'NONE', #23171, 6.000000000000000888 ) ;
#24908=CARTESIAN_POINT ( 'NONE',  ( 0.000000000000000000, 0.000000000000000000, 0.000000000000000000 ) ) ;
#24910=EDGE_CURVE ( 'NONE', #14303, #9700, #11226, .T. ) ;
#24912=CARTESIAN_POINT ( 'NONE',  ( 6.350852961086080661, -9.614813431917819062E-14, -130.8750000000000284 ) ) ;
#24913=CARTESIAN_POINT ( 'NONE',  ( 5.412658773652739619, 3.124999999999988898, -149.1830127018922667 ) ) ;
#24917=CARTESIAN_POINT ( 'NONE',  ( -6.350852961085760029, -1.281975124255709124E-13, -65.62500000000002842 ) ) ;
#24919=CARTESIAN_POINT ( 'NONE',  ( -5.999999999999962697, 3.323446944526963891E-14, -149.9136751345948255 ) ) ;
#24923=CARTESIAN_POINT ( 'NONE',  ( 5.196152422706629359, -2.999999999999988898, -117.7886751345948397 ) ) ;
#24925=CARTESIAN_POINT ( 'NONE',  ( 6.000000000000052403, -1.607695154586662678, -48.73066243270260856 ) ) ;
#24926=ORIENTED_EDGE ( 'NONE', *, *, #12170, .T. ) ;
#24930=CARTESIAN_POINT ( 'NONE',  ( 3.175426480543072749, 5.499999999999865885, -145.6250000000000284 ) ) ;
#24932=ORIENTED_EDGE ( 'NONE', *, *, #24634, .T. ) ;
#24933=CARTESIAN_POINT ( 'NONE',  ( -4.763139720814407951, -2.750000000000016431, -70.00000000000000000 ) ) ;
#24935=CARTESIAN_POINT ( 'NONE',  ( 5.412658773652712085, -3.125000000000086153, -92.43301270189225249 ) ) ;
#24936=CARTESIAN_POINT ( 'NONE',  ( -5.999340830937887503, -9.219973438021447976, -24.59179872956897839 ) ) ;
#24937=CARTESIAN_POINT ( 'NONE',  ( -5.196152422706601826, 2.999999999999975131, -106.5386751345948113 ) ) ;
#24939=CARTESIAN_POINT ( 'NONE',  ( 3.464101615137852974, 5.999999999999884537, -98.83632486540518869 ) ) ;
#24941=EDGE_CURVE ( 'NONE', #20441, #23894, #5649, .T. ) ;
#24942=CARTESIAN_POINT ( 'NONE',  ( -4.763139720814407951, -2.750000000000016431, -160.0000000000000284 ) ) ;
#24943=CARTESIAN_POINT ( 'NONE',  ( 0.000000000000000000, 0.000000000000000000, 0.000000000000000000 ) ) ;
#24944=CARTESIAN_POINT ( 'NONE',  ( -4.763139720814407951, -2.750000000000016431, -85.00000000000001421 ) ) ;
#24947=CARTESIAN_POINT ( 'NONE',  ( -2.775557561562891351E-14, -5.500000000000115463, -71.25000000000002842 ) ) ;
#24948=FACE_OUTER_BOUND ( 'NONE', #15992, .T. ) ;
#24950=CARTESIAN_POINT ( 'NONE',  ( 5.999999999999949374, 1.607695154586804565, -106.5193375672974696 ) ) ;
#24952=CARTESIAN_POINT ( 'NONE',  ( 5.999999999999999112, 2.951592740943527306E-14, -149.1636751345948824 ) ) ;
#24959=CARTESIAN_POINT ( 'NONE',  ( -5.999999999999963585, 1.780251999655701777E-13, -52.41367513459481842 ) ) ;
#24960=ORIENTED_EDGE ( 'NONE', *, *, #8813, .T. ) ;
#24961=EDGE_LOOP ( 'NONE', ( #29881, #19481, #25034, #23027 ) ) ;
#24963=CARTESIAN_POINT ( 'NONE',  ( -3.175426480542816510, -5.500000000000057732, -93.87500000000002842 ) ) ;
#24964=CARTESIAN_POINT ( 'NONE',  ( 0.000000000000000000, -5.999999999999991118, -89.53867513459485394 ) ) ;
#24965=CARTESIAN_POINT ( 'NONE',  ( 2.775557561562891351E-14, 6.250000000000033751, -114.4330127018922099 ) ) ;
#24966=ORIENTED_EDGE ( 'NONE', *, *, #7561, .T. ) ;
#24967=DIRECTION ( 'NONE',  ( -7.147005652999508048E-36, 5.642372883946980038E-36, 1.000000000000000000 ) ) ;
#24970=CARTESIAN_POINT ( 'NONE',  ( -3.608439182435115633, 6.249999999999965361, -55.80801270189227381 ) ) ;
#24974=EDGE_CURVE ( 'NONE', #651, #21812, #17681, .T. ) ;
#24977=CARTESIAN_POINT ( 'NONE',  ( -4.763139720814407951, 2.749999999999946709, -160.2500000000000000 ) ) ;
#24979=CARTESIAN_POINT ( 'NONE',  ( 5.999999999999949374, 1.607695154586804565, -108.0193375672974128 ) ) ;
#24980=CARTESIAN_POINT ( 'NONE',  ( -3.175426480542816066, -5.500000000000057732, -105.8750000000000284 ) ) ;
#24982=CARTESIAN_POINT ( 'NONE',  ( 4.763139720814407951, 2.750000000000002665, -97.75000000000000000 ) ) ;
#24983=( BOUNDED_CURVE ( )  B_SPLINE_CURVE ( 2, ( #6542, #27265, #3458, #15501, #24964, #12892, #20375, #8547, #6381 ),
 .UNSPECIFIED., .F., .T. ) 
 B_SPLINE_CURVE_WITH_KNOTS ( ( 3, 2, 2, 2, 3 ),
 ( 0.6805555555555554692, 0.6814814814814814659, 0.6833333333333333481, 0.6851851851851852304, 0.6861111111111111160 ),
 .UNSPECIFIED. ) 
 CURVE ( )  GEOMETRIC_REPRESENTATION_ITEM ( )  RATIONAL_B_SPLINE_CURVE ( ( 0.9330127018922194093, 0.9330127018922154125, 1.000000000000000000, 0.8660254037844388186, 1.000000000000000000, 0.8660254037844388186, 1.000000000000000000, 0.9330127018922194093, 0.9330127018922194093 ) ) 
 REPRESENTATION_ITEM ( '' )  );
#24984=CARTESIAN_POINT ( 'NONE',  ( -3.464101615137725076, 5.999999999999979572, -151.6636751345947971 ) ) ;
#24985=SURFACE_STYLE_USAGE ( .BOTH. , #3635 ) ;
#24986=CARTESIAN_POINT ( 'NONE',  ( 6.000000000000000888, 7.762456499804234384E-14, -118.5863248654052313 ) ) ;
#24987=EDGE_LOOP ( 'NONE', ( #20335, #18514, #29924, #18286 ) ) ;
#24991=DIRECTION ( 'NONE',  ( 1.260129944081490070E-35, 5.642372883946978702E-36, 1.000000000000000000 ) ) ;
#24992=VERTEX_POINT ( 'NONE', #1673 ) ;
#24994=CARTESIAN_POINT ( 'NONE',  ( -7.216878364870328078, 0.000000000000000000, -87.69198729810783277 ) ) ;
#24996=CARTESIAN_POINT ( 'NONE',  ( -5.999999999999963585, -1.487416814333745711E-14, -167.3363248654052029 ) ) ;
#24997=ORIENTED_EDGE ( 'NONE', *, *, #23760, .F. ) ;
#24998=CARTESIAN_POINT ( 'NONE',  ( -1.966823652257158273, 10.82907957849943337, -30.68208441639941952 ) ) ;
#24999=CARTESIAN_POINT ( 'NONE',  ( -4.763139720814407951, 2.749999999999946709, -151.2500000000000000 ) ) ;
#25001=ORIENTED_EDGE ( 'NONE', *, *, #18154, .F. ) ;
#25003=EDGE_CURVE ( 'NONE', #9617, #28281, #19413, .T. ) ;
#25004=CARTESIAN_POINT ( 'NONE',  ( -2.775557561562891351E-14, -5.500000000000115463, -120.7500000000000284 ) ) ;
#25005=CARTESIAN_POINT ( 'NONE',  ( 3.608439182435180470, -6.249999999999997335, -139.0580127018922099 ) ) ;
#25007=CARTESIAN_POINT ( 'NONE',  ( 3.464101615137852974, 5.999999999999884537, -160.9136751345947971 ) ) ;
#25008=CARTESIAN_POINT ( 'NONE',  ( 5.412658773652739619, 3.124999999999988898, -121.3169872981078043 ) ) ;
#25009=CARTESIAN_POINT ( 'NONE',  ( 3.608439182435180470, -6.249999999999997335, -180.1919872981078186 ) ) ;
#25010=CARTESIAN_POINT ( 'NONE',  ( 4.763139720814407951, -2.749999999999988454, -171.5000000000000000 ) ) ;
#25015=CARTESIAN_POINT ( 'NONE',  ( 5.999999999999999112, 2.951592740943527306E-14, -164.1636751345948824 ) ) ;
#25017=CARTESIAN_POINT ( 'NONE',  ( -5.196152422706573404, -3.000000000000002665, -55.28867513459484684 ) ) ;
#25020=CARTESIAN_POINT ( 'NONE',  ( -7.216878364870328078, 0.000000000000000000, -71.19198729810781856 ) ) ;
#25021=CARTESIAN_POINT ( 'NONE',  ( -7.216878364870328078, 0.000000000000000000, -51.69198729810779014 ) ) ;
#25023=CARTESIAN_POINT ( 'NONE',  ( -3.175426480542816510, 5.499999999999865885, -52.37500000000002842 ) ) ;
#25024=CARTESIAN_POINT ( 'NONE',  ( -5.999999999999963585, -1.487416814333745711E-14, -55.41367513459483973 ) ) ;
#25025=CARTESIAN_POINT ( 'NONE',  ( 2.775557561562891351E-14, 20.00000000000001776, -25.00000000000002132 ) ) ;
#25027=CARTESIAN_POINT ( 'NONE',  ( 4.763139720814407951, 2.750000000000002665, -132.2500000000000284 ) ) ;
#25032=CARTESIAN_POINT ( 'NONE',  ( 0.000000000000000000, 0.000000000000000000, 0.000000000000000000 ) ) ;
#25034=ORIENTED_EDGE ( 'NONE', *, *, #12299, .T. ) ;
#25036=CARTESIAN_POINT ( 'NONE',  ( 6.000000000000000888, -3.330669073875464691E-16, -7.560779664488942560E-35 ) ) ;
#25038=CARTESIAN_POINT ( 'NONE',  ( 3.608439182435180470, 6.249999999999982236, -112.1919872981078186 ) ) ;
#25042=DIRECTION ( 'NONE',  ( -7.147005652999508048E-36, 5.642372883946980038E-36, 1.000000000000000000 ) ) ;
#25045=VECTOR ( 'NONE', #9055, 1000.000000000000000 ) ;
#25046=ORIENTED_EDGE ( 'NONE', *, *, #221, .F. ) ;
#25048=CARTESIAN_POINT ( 'NONE',  ( -6.350852961085760029, -1.281975124255709124E-13, -49.12500000000000711 ) ) ;
#25053=CARTESIAN_POINT ( 'NONE',  ( -5.412658773652684552, -3.125000000000099920, -70.43301270189222407 ) ) ;
#25054=EDGE_CURVE ( 'NONE', #16378, #3967, #27629, .T. ) ;
#25061=CARTESIAN_POINT ( 'NONE',  ( -6.350852961085760029, -1.281975124255709124E-13, -131.6250000000000284 ) ) ;
#25065=CARTESIAN_POINT ( 'NONE',  ( -6.350852961085760029, -1.281975124255709124E-13, -64.12500000000001421 ) ) ;
#25066=CARTESIAN_POINT ( 'NONE',  ( 5.196152422706629359, -2.999999999999988898, -154.7113248654052313 ) ) ;
#25072=CARTESIAN_POINT ( 'NONE',  ( 3.464101615137757051, -5.999999999999979572, -117.9136751345948255 ) ) ;
#25073=CARTESIAN_POINT ( 'NONE',  ( 6.000000000000000888, 1.743066579297358182E-13, -85.58632486540523132 ) ) ;
#25074=( BOUNDED_CURVE ( )  B_SPLINE_CURVE ( 2, ( #24685, #3473, #10579, #26973, #3931, #6102, #13218, #24979, #20251 ),
 .UNSPECIFIED., .F., .T. ) 
 B_SPLINE_CURVE_WITH_KNOTS ( ( 3, 2, 2, 2, 3 ),
 ( 0.4527777777777778345, 0.4537037037037037202, 0.4555555555555556024, 0.4574074074074073737, 0.4583333333333332593 ),
 .UNSPECIFIED. ) 
 CURVE ( )  GEOMETRIC_REPRESENTATION_ITEM ( )  RATIONAL_B_SPLINE_CURVE ( ( 0.9330127018922194093, 0.9330127018922234061, 1.000000000000000000, 0.8660254037844388186, 1.000000000000000000, 0.8660254037844388186, 1.000000000000000000, 0.9330127018922234061, 0.9330127018922194093 ) ) 
 REPRESENTATION_ITEM ( '' )  );
#25075=ORIENTED_EDGE ( 'NONE', *, *, #13799, .T. ) ;
#25077=CARTESIAN_POINT ( 'NONE',  ( -5.999999999999963585, 1.780251999655701777E-13, -109.4136751345948113 ) ) ;
#25080=ADVANCED_FACE ( 'NONE', ( #16609 ), #9357, .T. ) ;
#25081=CARTESIAN_POINT ( 'NONE',  ( 4.763139720814407951, 2.750000000000002665, -144.2500000000000000 ) ) ;
#25084=CARTESIAN_POINT ( 'NONE',  ( -4.763139720814407951, 2.749999999999946709, -74.75000000000004263 ) ) ;
#25086=CARTESIAN_POINT ( 'NONE',  ( -5.999999999999963585, 9.296355089585909904E-15, -164.9136751345948255 ) ) ;
#25089=CARTESIAN_POINT ( 'NONE',  ( -0.8083154347085889091, -10.97740844234573387, -30.95886765600326029 ) ) ;
#25090=CARTESIAN_POINT ( 'NONE',  ( -5.630955349224697315, 2.071796769723730058, -179.9999999999999432 ) ) ;
#25091=CARTESIAN_POINT ( 'NONE',  ( -5.196152422706573404, -3.000000000000002665, -91.28867513459482552 ) ) ;
#25093=CARTESIAN_POINT ( 'NONE',  ( -3.175426480542816066, 5.499999999999865885, -155.8750000000000000 ) ) ;
#25095=CARTESIAN_POINT ( 'NONE',  ( -1.170107792542705694, 5.489964307952521771, -180.0000000000000000 ) ) ;
#25097=CARTESIAN_POINT ( 'NONE',  ( 4.763139720814407951, 2.750000000000002665, -85.75000000000000000 ) ) ;
#25100=CARTESIAN_POINT ( 'NONE',  ( -2.775557561562891351E-14, -5.500000000000115463, -69.75000000000002842 ) ) ;
#25103=CARTESIAN_POINT ( 'NONE',  ( 0.000000000000000000, 0.000000000000000000, 0.000000000000000000 ) ) ;
#25104=CARTESIAN_POINT ( 'NONE',  ( 6.000000000000007105, -1.607695154586741060, -174.7306624327025872 ) ) ;
#25105=CARTESIAN_POINT ( 'NONE',  ( 0.000000000000000000, 0.000000000000000000, 0.000000000000000000 ) ) ;
#25106=CARTESIAN_POINT ( 'NONE',  ( 6.000000000000000888, 1.743066579297358182E-13, -104.1636751345948397 ) ) ;
#25109=ORIENTED_EDGE ( 'NONE', *, *, #15348, .F. ) ;
#25111=CARTESIAN_POINT ( 'NONE',  ( -6.000000000000000888, 1.067854986875958443E-15, 7.560779664488942560E-35 ) ) ;
#25112=ADVANCED_FACE ( 'NONE', ( #26079 ), #21191, .T. ) ;
#25115=CARTESIAN_POINT ( 'NONE',  ( -2.775557561562891351E-14, -5.500000000000115463, -96.75000000000000000 ) ) ;
#25116=CARTESIAN_POINT ( 'NONE',  ( 5.412658773652712085, -3.125000000000086153, -108.9330127018922667 ) ) ;
#25117=CARTESIAN_POINT ( 'NONE',  ( 6.000000000000000888, 1.743066579297358182E-13, -94.58632486540521711 ) ) ;
#25120=CARTESIAN_POINT ( 'NONE',  ( -2.775557561562891351E-14, -5.500000000000115463, -165.7500000000000000 ) ) ;
#25121=CARTESIAN_POINT ( 'NONE',  ( 3.608439182435180470, -6.249999999999997335, -52.05801270189225960 ) ) ;
#25123=VERTEX_POINT ( 'NONE', #25786 ) ;
#25124=CARTESIAN_POINT ( 'NONE',  ( -5.999999999999962697, 3.323446944526963891E-14, -152.9136751345948255 ) ) ;
#25126=CARTESIAN_POINT ( 'NONE',  ( -4.763139720814407951, 2.749999999999946709, -161.7500000000000568 ) ) ;
#25129=CARTESIAN_POINT ( 'NONE',  ( 0.000000000000000000, 5.499999999999991118, -106.5000000000000426 ) ) ;
#25132=CARTESIAN_POINT ( 'NONE',  ( -4.763139720814407951, 2.749999999999946709, -94.25000000000000000 ) ) ;
#25136=ORIENTED_EDGE ( 'NONE', *, *, #20072, .T. ) ;
#25141=ORIENTED_EDGE ( 'NONE', *, *, #3057, .T. ) ;
#25144=CARTESIAN_POINT ( 'NONE',  ( 2.775557561562891351E-14, -6.250000000000061284, -90.31698729810783277 ) ) ;
#25147=CARTESIAN_POINT ( 'NONE',  ( -5.197562551122842933, 9.697615191485752462, -28.02238803416286927 ) ) ;
#25148=ADVANCED_FACE ( 'NONE', ( #4877 ), #11853, .T. ) ;
#25152=CARTESIAN_POINT ( 'NONE',  ( 3.175426480543072749, 5.499999999999865885, -118.6250000000000284 ) ) ;
#25154=CARTESIAN_POINT ( 'NONE',  ( 2.775557561562891351E-14, 6.250000000000033751, -136.9330127018922383 ) ) ;
#25155=ORIENTED_EDGE ( 'NONE', *, *, #18397, .F. ) ;
#25157=CARTESIAN_POINT ( 'NONE',  ( -3.608439182435052128, -6.250000000000110134, -124.9419872981078186 ) ) ;
#25158=CARTESIAN_POINT ( 'NONE',  ( 5.412658773652712085, -3.125000000000086153, -180.0669872981078186 ) ) ;
#25159=ORIENTED_EDGE ( 'NONE', *, *, #29977, .T. ) ;
#25162=( BOUNDED_CURVE ( )  B_SPLINE_CURVE ( 2, ( #5080, #21551, #19247, #24274, #28576, #26282, #21701, #17101, #12467 ),
 .UNSPECIFIED., .F., .T. ) 
 B_SPLINE_CURVE_WITH_KNOTS ( ( 3, 2, 2, 2, 3 ),
 ( 0.7861111111111110938, 0.7870370370370369795, 0.7888888888888888618, 0.7907407407407407440, 0.7916666666666666297 ),
 .UNSPECIFIED. ) 
 CURVE ( )  GEOMETRIC_REPRESENTATION_ITEM ( )  RATIONAL_B_SPLINE_CURVE ( ( 0.9330127018922194093, 0.9330127018922194093, 1.000000000000000000, 0.8660254037844388186, 1.000000000000000000, 0.8660254037844388186, 1.000000000000000000, 0.9330127018922234061, 0.9330127018922194093 ) ) 
 REPRESENTATION_ITEM ( '' )  );
#25167=CARTESIAN_POINT ( 'NONE',  ( -5.412658773652739619, 3.124999999999975131, -74.31698729810781856 ) ) ;
#25168=CARTESIAN_POINT ( 'NONE',  ( -3.608439182435052128, -6.250000000000110134, -63.44198729810784698 ) ) ;
#25169=CARTESIAN_POINT ( 'NONE',  ( 3.464101615137852974, 5.999999999999884537, -110.8363248654052455 ) ) ;
#25170=CARTESIAN_POINT ( 'NONE',  ( -6.350852961085760029, -1.281975124255709124E-13, -47.62500000000000000 ) ) ;
#25172=CARTESIAN_POINT ( 'NONE',  ( -3.464101615137757051, -5.999999999999979572, -153.5863248654051461 ) ) ;
#25173=CARTESIAN_POINT ( 'NONE',  ( -4.763139720814407951, 2.749999999999946709, -119.7500000000000284 ) ) ;
#25178=CARTESIAN_POINT ( 'NONE',  ( 0.000000000000000000, 5.999999999999977796, -122.7113248654052597 ) ) ;
#25185=CARTESIAN_POINT ( 'NONE',  ( 3.608439182435180470, -6.249999999999997335, -112.6919872981078328 ) ) ;
#25186=CARTESIAN_POINT ( 'NONE',  ( 0.000000000000000000, -5.999999999999991118, -54.46132486540522422 ) ) ;
#25189=ORIENTED_EDGE ( 'NONE', *, *, #5691, .T. ) ;
#25192=CARTESIAN_POINT ( 'NONE',  ( 3.608439182435180470, 6.249999999999982236, -143.6919872981078470 ) ) ;
#25194=AXIS2_PLACEMENT_3D ( 'NONE', #27972, #2048, #20641 ) ;
#25196=CARTESIAN_POINT ( 'NONE',  ( 5.196152422706629359, -2.999999999999988898, -93.21132486540523132 ) ) ;
#25200=CARTESIAN_POINT ( 'NONE',  ( 7.216878364870455975, -6.409875621278545621E-14, -69.80801270189220986 ) ) ;
#25203=FACE_OUTER_BOUND ( 'NONE', #1187, .T. ) ;
#25204=CARTESIAN_POINT ( 'NONE',  ( -2.910268709469100014E-14, -10.99999999999998224, -14.99152654425661702 ) ) ;
#25205=CARTESIAN_POINT ( 'NONE',  ( -5.196152422706573404, -3.000000000000002665, -155.7886751345948255 ) ) ;
#25208=CARTESIAN_POINT ( 'NONE',  ( -6.350852961085760029, -1.281975124255709124E-13, -121.1250000000000426 ) ) ;
#25210=CARTESIAN_POINT ( 'NONE',  ( -5.412658773652739619, 3.124999999999975131, -144.1830127018922667 ) ) ;
#25211=LINE ( 'NONE', #11285, #29213 ) ;
#25212=FACE_OUTER_BOUND ( 'NONE', #5465, .T. ) ;
#25213=ORIENTED_EDGE ( 'NONE', *, *, #27082, .T. ) ;
#25215=CARTESIAN_POINT ( 'NONE',  ( -3.175426480542816066, 5.499999999999865885, -56.87500000000004263 ) ) ;
#25216=CARTESIAN_POINT ( 'NONE',  ( 5.999999999999949374, 1.607695154586804565, -124.5193375672974412 ) ) ;
#25218=CARTESIAN_POINT ( 'NONE',  ( 5.196152422706629359, 3.000000000000002665, -170.9613248654052313 ) ) ;
#25219=VERTEX_POINT ( 'NONE', #3022 ) ;
#25223=ADVANCED_FACE ( 'NONE', ( #15177 ), #9961, .T. ) ;
#25225=CARTESIAN_POINT ( 'NONE',  ( -3.175426480542816510, 5.499999999999865885, -137.8750000000000568 ) ) ;
#25227=ORIENTED_EDGE ( 'NONE', *, *, #4426, .F. ) ;
#25228=CARTESIAN_POINT ( 'NONE',  ( -2.775557561562891351E-14, -5.500000000000115463, -74.25000000000004263 ) ) ;
#25229=CARTESIAN_POINT ( 'NONE',  ( -5.803206942314495187, -9.345129262100574152, -26.57517091834633050 ) ) ;
#25230=DIRECTION ( 'NONE',  ( 1.000000000000000000, -5.551115123125773458E-17, -1.260129944081490338E-35 ) ) ;
#25231=CARTESIAN_POINT ( 'NONE',  ( 0.000000000000000000, 0.000000000000000000, 0.000000000000000000 ) ) ;
#25232=CARTESIAN_POINT ( 'NONE',  ( -6.000000000000000000, 1.067854986875958245E-15, -180.0000000000000568 ) ) ;
#25234=CARTESIAN_POINT ( 'NONE',  ( -4.763139720814407951, 2.749999999999946709, -146.7500000000000568 ) ) ;
#25237=CARTESIAN_POINT ( 'NONE',  ( 6.350852961086080661, -9.614813431917819062E-14, -142.8750000000000568 ) ) ;
#25239=EDGE_CURVE ( 'NONE', #18212, #799, #14334, .T. ) ;
#25240=CARTESIAN_POINT ( 'NONE',  ( 3.175426480543072749, 5.499999999999865885, -84.12499999999997158 ) ) ;
#25242=CARTESIAN_POINT ( 'NONE',  ( 6.350852961086080661, -9.614813431917819062E-14, -75.37500000000000000 ) ) ;
#25243=( BOUNDED_CURVE ( )  B_SPLINE_CURVE ( 2, ( #6442, #18307, #15871, #1687, #15712, #20135, #29325, #24729, #1378 ),
 .UNSPECIFIED., .F., .T. ) 
 B_SPLINE_CURVE_WITH_KNOTS ( ( 3, 2, 2, 2, 3 ),
 ( 0.4472222222222221877, 0.4481481481481481288, 0.4500000000000000111, 0.4518518518518518379, 0.4527777777777777790 ),
 .UNSPECIFIED. ) 
 CURVE ( )  GEOMETRIC_REPRESENTATION_ITEM ( )  RATIONAL_B_SPLINE_CURVE ( ( 0.9330127018922194093, 0.9330127018922174109, 1.000000000000000000, 0.8660254037844388186, 1.000000000000000000, 0.8660254037844388186, 1.000000000000000000, 0.9330127018922194093, 0.9330127018922194093 ) ) 
 REPRESENTATION_ITEM ( '' )  );
#25244=CARTESIAN_POINT ( 'NONE',  ( -5.999999999999963585, 1.780251999655701777E-13, -74.91367513459485394 ) ) ;
#25246=CARTESIAN_POINT ( 'NONE',  ( 3.464101615137757051, -5.999999999999979572, -87.91367513459483973 ) ) ;
#25249=CARTESIAN_POINT ( 'NONE',  ( -5.196152422706601826, 2.999999999999975131, -54.96132486540522422 ) ) ;
#25251=EDGE_CURVE ( 'NONE', #8489, #15139, #1539, .T. ) ;
#25256=CARTESIAN_POINT ( 'NONE',  ( 6.000000000000000888, 1.743066579297358182E-13, -97.58632486540524553 ) ) ;
#25259=VERTEX_POINT ( 'NONE', #17341 ) ;
#25260=CARTESIAN_POINT ( 'NONE',  ( -4.763139720814407951, -2.750000000000016431, -98.50000000000002842 ) ) ;
#25262=CARTESIAN_POINT ( 'NONE',  ( 3.608439182435180470, 6.249999999999982236, -107.0580127018922667 ) ) ;
#25264=LINE ( 'NONE', #9164, #1259 ) ;
#25266=CARTESIAN_POINT ( 'NONE',  ( -3.175426480542816510, -5.500000000000057732, -162.8750000000000284 ) ) ;
#25267=CARTESIAN_POINT ( 'NONE',  ( 5.196152422706629359, -2.999999999999988898, -105.7886751345948397 ) ) ;
#25269=CARTESIAN_POINT ( 'NONE',  ( -5.999999999999957367, 1.607695154586737507, -152.9806624327025872 ) ) ;
#25272=CARTESIAN_POINT ( 'NONE',  ( 3.175426480543072749, -5.500000000000105693, -159.6250000000000284 ) ) ;
#25274=B_SPLINE_CURVE_WITH_KNOTS ( 'NONE', 3,
 ( #7006, #13660, #16124, #1945, #20697, #9018, #18408, #27727, #25427, #4552, #4391, #13818, #13976, #23163, #2105, #11510, #20850, #9165, #23316, #11666, #24189, #23900, #24044, #12410, #5435, #21301, #14846, #7747, #10234, #10081, #2989, #2692, #26047, #7897, #12556, #3134, #21903, #19015, #4991, #12117, #19454, #5584, #16865, #837 ),
 .UNSPECIFIED., .F., .F.,
 ( 4, 2, 2, 2, 2, 2, 2, 2, 2, 2, 2, 2, 2, 2, 2, 2, 2, 2, 2, 2, 2, 4 ),
 ( 0.000000000000000000, 0.001197331758471049034, 0.002394663516942098069, 0.003591995275413146886, 0.004789327033884196137, 0.005387992913119717293, 0.005986658792355239317, 0.007183990550826290303, 0.008381322309297341289, 0.009578654067768392275, 0.01017731994700391690, 0.01077598582623943979, 0.01137465170547496615, 0.01197331758471049078, 0.01317064934318154697, 0.01376931522241707680, 0.01436798110165260489, 0.01556531286012365588, 0.01676264461859470686, 0.01736131049783023322, 0.01795997637706575611, 0.01915730813553680537 ),
 .UNSPECIFIED. ) ;
#25275=EDGE_CURVE ( 'NONE', #799, #1357, #4677, .T. ) ;
#25276=CARTESIAN_POINT ( 'NONE',  ( -3.175426480542816066, -5.500000000000057732, -110.3750000000000426 ) ) ;
#25278=CARTESIAN_POINT ( 'NONE',  ( 0.000000000000000000, -5.999999999999991118, -122.5386751345948255 ) ) ;
#25280=CARTESIAN_POINT ( 'NONE',  ( -4.763139720814407951, 2.749999999999946709, -98.75000000000000000 ) ) ;
#25282=ORIENTED_EDGE ( 'NONE', *, *, #9293, .F. ) ;
#25288=CARTESIAN_POINT ( 'NONE',  ( -6.000000000000007105, -1.607695154586655129, -86.26933756729742697 ) ) ;
#25290=CARTESIAN_POINT ( 'NONE',  ( 5.196152422706629359, -2.999999999999988898, -169.7113248654051745 ) ) ;
#25292=( GEOMETRIC_REPRESENTATION_CONTEXT ( 3 ) GLOBAL_UNCERTAINTY_ASSIGNED_CONTEXT ( ( #29397 ) ) GLOBAL_UNIT_ASSIGNED_CONTEXT ( ( #18830, #4819, #25715 ) ) REPRESENTATION_CONTEXT ( 'NONE', 'WORKASPACE' ) );
#25293=CARTESIAN_POINT ( 'NONE',  ( 3.608439182435180470, -6.249999999999997335, -87.19198729810783277 ) ) ;
#25296=ORIENTED_EDGE ( 'NONE', *, *, #6658, .F. ) ;
#25299=ORIENTED_EDGE ( 'NONE', *, *, #9261, .F. ) ;
#25302=CARTESIAN_POINT ( 'NONE',  ( 0.000000000000000000, 5.499999999999991118, -124.5000000000000568 ) ) ;
#25304=CARTESIAN_POINT ( 'NONE',  ( 3.608439182435180470, -6.249999999999997335, -130.0580127018922383 ) ) ;
#25307=CARTESIAN_POINT ( 'NONE',  ( 3.608439182435180470, 6.249999999999982236, -172.1919872981078470 ) ) ;
#25308=CARTESIAN_POINT ( 'NONE',  ( 7.216878364870455975, -6.409875621278545621E-14, -179.9419872981078186 ) ) ;
#25310=ORIENTED_EDGE ( 'NONE', *, *, #3829, .F. ) ;
#25311=CARTESIAN_POINT ( 'NONE',  ( 0.000000000000000000, 0.000000000000000000, 0.000000000000000000 ) ) ;
#25315=CARTESIAN_POINT ( 'NONE',  ( 2.775557561562891351E-14, 6.250000000000033751, -77.56698729810784698 ) ) ;
#25316=CARTESIAN_POINT ( 'NONE',  ( -7.216878364870328078, 0.000000000000000000, -59.19198729810781856 ) ) ;
#25317=CARTESIAN_POINT ( 'NONE',  ( 5.196152422706629359, -2.999999999999988898, -170.2886751345948255 ) ) ;
#25318=CARTESIAN_POINT ( 'NONE',  ( 6.350852961086080661, -9.614813431917819062E-14, -51.37500000000002132 ) ) ;
#25319=CARTESIAN_POINT ( 'NONE',  ( -5.999999999999963585, 1.780251999655701777E-13, -111.8363248654052313 ) ) ;
#25320=CARTESIAN_POINT ( 'NONE',  ( 5.196152422706629359, -2.999999999999988898, -153.2113248654052313 ) ) ;
#25323=CARTESIAN_POINT ( 'NONE',  ( -3.175426480542816510, 5.499999999999865885, -121.3750000000000284 ) ) ;
#25324=CARTESIAN_POINT ( 'NONE',  ( -4.763139720814407951, -2.750000000000016431, -157.0000000000000284 ) ) ;
#25335=CARTESIAN_POINT ( 'NONE',  ( -5.412658773652739619, 3.124999999999975131, -111.8169872981078470 ) ) ;
#25343=( BOUNDED_CURVE ( )  B_SPLINE_CURVE ( 2, ( #26100, #7506, #14474, #26245, #12171, #9831, #21516, #442, #5198 ),
 .UNSPECIFIED., .F., .T. ) 
 B_SPLINE_CURVE_WITH_KNOTS ( ( 3, 2, 2, 2, 3 ),
 ( 0.6694444444444445086, 0.6703703703703703942, 0.6722222222222222765, 0.6740740740740740478, 0.6750000000000000444 ),
 .UNSPECIFIED. ) 
 CURVE ( )  GEOMETRIC_REPRESENTATION_ITEM ( )  RATIONAL_B_SPLINE_CURVE ( ( 0.9330127018922194093, 0.9330127018922234061, 1.000000000000000000, 0.8660254037844388186, 1.000000000000000000, 0.8660254037844388186, 1.000000000000000000, 0.9330127018922154125, 0.9330127018922194093 ) ) 
 REPRESENTATION_ITEM ( '' )  );
#25344=CARTESIAN_POINT ( 'NONE',  ( 2.775557561562891351E-14, 6.250000000000033751, -151.0669872981078470 ) ) ;
#25346=EDGE_CURVE ( 'NONE', #5496, #23148, #734, .T. ) ;
#25349=VECTOR ( 'NONE', #28320, 1000.000000000000000 ) ;
#25354=CARTESIAN_POINT ( 'NONE',  ( -5.412658773652739619, 3.124999999999975131, -67.68301270189225249 ) ) ;
#25356=CARTESIAN_POINT ( 'NONE',  ( 6.000000000000052403, -1.607695154586662678, -124.6533121635129930 ) ) ;
#25358=LINE ( 'NONE', #25517, #21738 ) ;
#25361=CARTESIAN_POINT ( 'NONE',  ( -3.464101615137757051, -5.999999999999979572, -95.08632486540521711 ) ) ;
#25362=EDGE_CURVE ( 'NONE', #14907, #17914, #29796, .T. ) ;
#25363=CARTESIAN_POINT ( 'NONE',  ( -4.763139720814407951, 2.749999999999946709, -121.2500000000000284 ) ) ;
#25365=CARTESIAN_POINT ( 'NONE',  ( -5.196152422706573404, -3.000000000000002665, -92.78867513459482552 ) ) ;
#25366=CARTESIAN_POINT ( 'NONE',  ( 3.608439182435180470, -6.249999999999997335, -143.5580127018922667 ) ) ;
#25368=CARTESIAN_POINT ( 'NONE',  ( 5.999999999999974243, 1.607695154586759934, -143.0966878364870354 ) ) ;
#25369=VERTEX_POINT ( 'NONE', #20242 ) ;
#25370=CARTESIAN_POINT ( 'NONE',  ( 3.175426480543072749, -5.500000000000105693, -57.62500000000004974 ) ) ;
#25371=CARTESIAN_POINT ( 'NONE',  ( -5.999999999999962697, 3.323446944526963260E-14, -155.3363248654052313 ) ) ;
#25372=CARTESIAN_POINT ( 'NONE',  ( -5.196152422706573404, -3.000000000000002665, -77.21132486540521711 ) ) ;
#25383=CARTESIAN_POINT ( 'NONE',  ( -2.775557561562891351E-14, -5.500000000000115463, -137.2499999999999716 ) ) ;
#25387=ADVANCED_FACE ( 'NONE', ( #22231 ), #29423, .T. ) ;
#25388=CARTESIAN_POINT ( 'NONE',  ( 4.763139720814407951, -2.749999999999988454, -63.50000000000000000 ) ) ;
#25390=CARTESIAN_POINT ( 'NONE',  ( 7.216878364870455975, -6.409875621278545621E-14, -89.30801270189223828 ) ) ;
#25391=CARTESIAN_POINT ( 'NONE',  ( 3.464101615137757051, -5.999999999999979572, -113.4136751345948113 ) ) ;
#25396=( GEOMETRIC_REPRESENTATION_CONTEXT ( 3 ) GLOBAL_UNCERTAINTY_ASSIGNED_CONTEXT ( ( #2564 ) ) GLOBAL_UNIT_ASSIGNED_CONTEXT ( ( #28419, #2775, #28564 ) ) REPRESENTATION_CONTEXT ( 'NONE', 'WORKASPACE' ) );
#25397=CARTESIAN_POINT ( 'NONE',  ( 4.763139720814407951, -2.749999999999988454, -152.0000000000000284 ) ) ;
#25399=CARTESIAN_POINT ( 'NONE',  ( -4.763139720814407951, 2.749999999999946709, -142.2500000000000000 ) ) ;
#25400=CARTESIAN_POINT ( 'NONE',  ( 3.608439182435180470, 6.249999999999982236, -161.0580127018921814 ) ) ;
#25402=CARTESIAN_POINT ( 'NONE',  ( -3.175426480542816066, 5.499999999999865885, -80.87500000000002842 ) ) ;
#25404=CARTESIAN_POINT ( 'NONE',  ( 6.350852961086080661, -9.614813431917819062E-14, -72.37499999999998579 ) ) ;
#25411=CARTESIAN_POINT ( 'NONE',  ( 0.000000000000000000, 5.999999999999977796, -94.78867513459482552 ) ) ;
#25418=VERTEX_POINT ( 'NONE', #11031 ) ;
#25422=CARTESIAN_POINT ( 'NONE',  ( -4.763139720814407951, 2.749999999999946709, -91.25000000000005684 ) ) ;
#25423=CARTESIAN_POINT ( 'NONE',  ( -5.412658773652684552, -3.125000000000099920, -106.4330127018922667 ) ) ;
#25427=CARTESIAN_POINT ( 'NONE',  ( 3.978158145384761202, -10.25965056898453653, -29.50791791133373820 ) ) ;
#25429=CARTESIAN_POINT ( 'NONE',  ( 0.000000000000000000, 5.999999999999977796, -93.28867513459482552 ) ) ;
#25430=EDGE_CURVE ( 'NONE', #10812, #30268, #20571, .T. ) ;
#25433=CARTESIAN_POINT ( 'NONE',  ( 3.175426480543072749, -5.500000000000105693, -171.6250000000000000 ) ) ;
#25434=CARTESIAN_POINT ( 'NONE',  ( 6.000000000000000888, 7.762456499804235646E-14, -127.5863248654052171 ) ) ;
#25435=CARTESIAN_POINT ( 'NONE',  ( 4.763139720814407951, -2.749999999999988454, -162.5000000000000284 ) ) ;
#25437=CARTESIAN_POINT ( 'NONE',  ( 0.000000000000000000, 5.499999999999991118, -105.0000000000000426 ) ) ;
#25439=CARTESIAN_POINT ( 'NONE',  ( -5.999999999999956479, -1.607695154586745057, -166.3466878364870354 ) ) ;
#25440=CARTESIAN_POINT ( 'NONE',  ( 4.763139720814407951, -2.749999999999988454, -96.50000000000002842 ) ) ;
#25446=LINE ( 'NONE', #30219, #5542 ) ;
#25448=CARTESIAN_POINT ( 'NONE',  ( 6.000000000000000888, 1.743066579297358182E-13, -103.5863248654052171 ) ) ;
#25449=ORIENTED_EDGE ( 'NONE', *, *, #11257, .F. ) ;
#25452=CARTESIAN_POINT ( 'NONE',  ( -3.608439182435052128, -6.250000000000110134, -85.94198729810781856 ) ) ;
#25458=EDGE_CURVE ( 'NONE', #29150, #1827, #29268, .T. ) ;
#25459=CARTESIAN_POINT ( 'NONE',  ( -4.763139720814407951, -2.750000000000016431, -125.5000000000000568 ) ) ;
#25462=EDGE_CURVE ( 'NONE', #18067, #14341, #3858, .T. ) ;
#25463=CARTESIAN_POINT ( 'NONE',  ( -3.608439182435052128, -6.250000000000110134, -127.3080127018922383 ) ) ;
#25464=EDGE_LOOP ( 'NONE', ( #14073, #15584, #490, #6870 ) ) ;
#25465=CARTESIAN_POINT ( 'NONE',  ( -5.196152422706601826, 2.999999999999975131, -57.03867513459481842 ) ) ;
#25466=CARTESIAN_POINT ( 'NONE',  ( 5.412658773652739619, 3.124999999999988898, -166.3169872981078470 ) ) ;
#25467=CARTESIAN_POINT ( 'NONE',  ( -3.608439182435115633, 6.249999999999965361, -179.4419872981078470 ) ) ;
#25469=CARTESIAN_POINT ( 'NONE',  ( 0.000000000000000000, 0.000000000000000000, 0.000000000000000000 ) ) ;
#25470=VERTEX_POINT ( 'NONE', #24674 ) ;
#25472=CYLINDRICAL_SURFACE ( 'NONE', #8943, 6.000000000000000888 ) ;
#25473=CARTESIAN_POINT ( 'NONE',  ( -5.999999999999944933, 1.607695154586759934, -136.4806624327025872 ) ) ;
#25476=CARTESIAN_POINT ( 'NONE',  ( 5.412658773652739619, 3.124999999999988898, -74.81698729810781856 ) ) ;
#25477=CARTESIAN_POINT ( 'NONE',  ( -2.775557561562891351E-14, -5.500000000000115463, -50.25000000000001421 ) ) ;
#25479=CARTESIAN_POINT ( 'NONE',  ( -3.464101615137757051, -5.999999999999979572, -47.66367513459483973 ) ) ;
#25480=CARTESIAN_POINT ( 'NONE',  ( -5.196152422706601826, 2.999999999999975131, -123.0386751345948255 ) ) ;
#25481=CARTESIAN_POINT ( 'NONE',  ( 3.175426480543072749, -5.500000000000105693, -122.1250000000000284 ) ) ;
#25486=( BOUNDED_CURVE ( )  B_SPLINE_CURVE ( 2, ( #9237, #27950, #25196, #21228, #23082, #28109, #21079, #9552, #23238 ),
 .UNSPECIFIED., .F., .F. ) 
 B_SPLINE_CURVE_WITH_KNOTS ( ( 3, 2, 2, 2, 3 ),
 ( 0.3472222222222222099, 0.3481481481481480955, 0.3499999999999999778, 0.3518518518518518601, 0.3527777777777778567 ),
 .UNSPECIFIED. ) 
 CURVE ( )  GEOMETRIC_REPRESENTATION_ITEM ( )  RATIONAL_B_SPLINE_CURVE ( ( 0.9330127018922194093, 0.9330127018922194093, 1.000000000000000000, 0.8660254037844388186, 1.000000000000000000, 0.8660254037844388186, 1.000000000000000000, 0.9330127018922154125, 0.9330127018922194093 ) ) 
 REPRESENTATION_ITEM ( '' )  );
#25488=CARTESIAN_POINT ( 'NONE',  ( -3.464101615137725076, 5.999999999999979572, -105.1636751345948539 ) ) ;
#25493=LINE ( 'NONE', #2169, #18716 ) ;
#25495=AXIS2_PLACEMENT_3D ( 'NONE', #11739, #9556, #28114 ) ;
#25496=CARTESIAN_POINT ( 'NONE',  ( -7.216878364870328078, 0.000000000000000000, -110.1919872981078043 ) ) ;
#25497=CARTESIAN_POINT ( 'NONE',  ( -5.999999999999963585, -2.788906526875773208E-15, -176.9136751345948539 ) ) ;
#25499=ORIENTED_EDGE ( 'NONE', *, *, #2322, .T. ) ;
#25500=VERTEX_POINT ( 'NONE', #1476 ) ;
#25503=EDGE_CURVE ( 'NONE', #20245, #16482, #16309, .T. ) ;
#25505=CARTESIAN_POINT ( 'NONE',  ( 2.775557561562891351E-14, 6.250000000000033751, -142.0669872981078470 ) ) ;
#25507=CARTESIAN_POINT ( 'NONE',  ( -5.999999999999962697, 3.323446944526963260E-14, -150.8363248654052029 ) ) ;
#25511=CARTESIAN_POINT ( 'NONE',  ( 2.775557561562891351E-14, 6.250000000000033751, -67.93301270189222407 ) ) ;
#25516=CARTESIAN_POINT ( 'NONE',  ( 6.000000000000000888, 1.743066579297358182E-13, -74.16367513459483973 ) ) ;
#25517=CARTESIAN_POINT ( 'NONE',  ( -6.000000000000000888, 1.067854986875958443E-15, 7.560779664488942560E-35 ) ) ;
#25521=CARTESIAN_POINT ( 'NONE',  ( 0.000000000000000000, -5.999999999999991118, -94.96132486540520290 ) ) ;
#25522=CARTESIAN_POINT ( 'NONE',  ( -3.175426480542816066, 5.499999999999865885, -124.3749999999999858 ) ) ;
#25524=CARTESIAN_POINT ( 'NONE',  ( 5.412658773652739619, 3.124999999999988898, -146.1830127018922667 ) ) ;
#25527=CARTESIAN_POINT ( 'NONE',  ( 4.763139720814407951, 2.750000000000002665, -58.75000000000002132 ) ) ;
#25528=CARTESIAN_POINT ( 'NONE',  ( 0.000000000000000000, 0.000000000000000000, 0.000000000000000000 ) ) ;
#25530=( BOUNDED_CURVE ( )  B_SPLINE_CURVE ( 2, ( #22867, #8098, #8421, #17826, #27146, #15528, #29610, #24849, #3798 ),
 .UNSPECIFIED., .F., .F. ) 
 B_SPLINE_CURVE_WITH_KNOTS ( ( 3, 2, 2, 2, 3 ),
 ( 0.6472222222222221433, 0.6481481481481481399, 0.6500000000000000222, 0.6518518518518519045, 0.6527777777777777901 ),
 .UNSPECIFIED. ) 
 CURVE ( )  GEOMETRIC_REPRESENTATION_ITEM ( )  RATIONAL_B_SPLINE_CURVE ( ( 0.9330127018922194093, 0.9330127018922114157, 1.000000000000000000, 0.8660254037844388186, 1.000000000000000000, 0.8660254037844388186, 1.000000000000000000, 0.9330127018922194093, 0.9330127018922194093 ) ) 
 REPRESENTATION_ITEM ( '' )  );
#25536=EDGE_CURVE ( 'NONE', #2534, #16280, #11772, .T. ) ;
#25537=CARTESIAN_POINT ( 'NONE',  ( -5.412658773652684552, -3.125000000000099920, -101.0669872981078186 ) ) ;
#25538=VECTOR ( 'NONE', #22624, 1000.000000000000000 ) ;
#25540=( BOUNDED_CURVE ( )  B_SPLINE_CURVE ( 2, ( #4967, #9454, #23442, #16102, #4367, #16252, #68, #216, #2082 ),
 .UNSPECIFIED., .F., .T. ) 
 B_SPLINE_CURVE_WITH_KNOTS ( ( 3, 2, 2, 2, 3 ),
 ( 0.1972222222222222432, 0.1981481481481481566, 0.2000000000000000111, 0.2018518518518518656, 0.2027777777777777790 ),
 .UNSPECIFIED. ) 
 CURVE ( )  GEOMETRIC_REPRESENTATION_ITEM ( )  RATIONAL_B_SPLINE_CURVE ( ( 0.9330127018922194093, 0.9330127018922204085, 1.000000000000000000, 0.8660254037844388186, 1.000000000000000000, 0.8660254037844388186, 1.000000000000000000, 0.9330127018922194093, 0.9330127018922194093 ) ) 
 REPRESENTATION_ITEM ( '' )  );
#25543=CARTESIAN_POINT ( 'NONE',  ( -4.763139720814407951, -2.750000000000016431, -137.5000000000000000 ) ) ;
#25548=CARTESIAN_POINT ( 'NONE',  ( -4.763139720814407951, -2.750000000000016431, -67.00000000000000000 ) ) ;
#25550=CARTESIAN_POINT ( 'NONE',  ( 5.412658773652712085, -3.125000000000086153, -89.43301270189223828 ) ) ;
#25557=CARTESIAN_POINT ( 'NONE',  ( -6.350852961085760029, -1.281975124255709124E-13, -145.1250000000000000 ) ) ;
#25558=CARTESIAN_POINT ( 'NONE',  ( -5.999999999999963585, 8.134310703387671600E-14, -144.8363248654052029 ) ) ;
#25559=CARTESIAN_POINT ( 'NONE',  ( -2.775557561562891351E-14, -5.500000000000115463, -135.7500000000000284 ) ) ;
#25561=CARTESIAN_POINT ( 'NONE',  ( 7.216878364870455975, -6.409875621278545621E-14, -158.3080127018922667 ) ) ;
#25562=CARTESIAN_POINT ( 'NONE',  ( -5.999999999999963585, 8.134310703387671600E-14, -116.3363248654052313 ) ) ;
#25565=CARTESIAN_POINT ( 'NONE',  ( 4.763139720814407951, 2.750000000000002665, -78.25000000000004263 ) ) ;
#25567=CARTESIAN_POINT ( 'NONE',  ( 6.350852961086080661, -9.614813431917819062E-14, -73.87500000000000000 ) ) ;
#25568=CARTESIAN_POINT ( 'NONE',  ( 0.000000000000000000, -5.999999999999991118, -156.4613248654052029 ) ) ;
#25571=CYLINDRICAL_SURFACE ( 'NONE', #18929, 6.000000000000000888 ) ;
#25577=EDGE_CURVE ( 'NONE', #2682, #18067, #21114, .T. ) ;
#25579=CARTESIAN_POINT ( 'NONE',  ( -5.999999999999963585, 1.780251999655701777E-13, -98.91367513459483973 ) ) ;
#25586=CARTESIAN_POINT ( 'NONE',  ( 6.000000000000000888, -1.859271017917181981E-14, -84.66367513459482552 ) ) ;
#25587=ORIENTED_EDGE ( 'NONE', *, *, #12299, .F. ) ;
#25591=VECTOR ( 'NONE', #5042, 1000.000000000000000 ) ;
#25592=ORIENTED_EDGE ( 'NONE', *, *, #4629, .T. ) ;
#25593=CARTESIAN_POINT ( 'NONE',  ( 3.175426480543072749, 5.499999999999865885, -90.12500000000001421 ) ) ;
#25594=CARTESIAN_POINT ( 'NONE',  ( 5.412658773652712085, -3.125000000000086153, -104.4330127018922525 ) ) ;
#25596=CARTESIAN_POINT ( 'NONE',  ( 5.382374809129858662, 9.594851770513413314, -27.68068691953152083 ) ) ;
#25597=CARTESIAN_POINT ( 'NONE',  ( 3.464101615137852974, 5.999999999999884537, -52.33632486540523843 ) ) ;
#25599=CARTESIAN_POINT ( 'NONE',  ( -2.775557561562891351E-14, -5.500000000000115463, -164.2500000000000000 ) ) ;
#25600=CARTESIAN_POINT ( 'NONE',  ( -5.412658773652684552, -3.125000000000099920, -47.93301270189220986 ) ) ;
#25601=VERTEX_POINT ( 'NONE', #12227 ) ;
#25603=CARTESIAN_POINT ( 'NONE',  ( 6.350852961086080661, -9.614813431917819062E-14, -168.3750000000000568 ) ) ;
#25606=CARTESIAN_POINT ( 'NONE',  ( -3.175426480542816510, -5.500000000000057732, -162.8750000000000284 ) ) ;
#25610=CARTESIAN_POINT ( 'NONE',  ( -2.775557561562891351E-14, -5.500000000000115463, -98.25000000000000000 ) ) ;
#25617=CYLINDRICAL_SURFACE ( 'NONE', #1631, 6.000000000000000888 ) ;
#25620=ORIENTED_EDGE ( 'NONE', *, *, #2557, .F. ) ;
#25624=AXIS2_PLACEMENT_3D ( 'NONE', #1266, #8335, #27069 ) ;
#25627=CARTESIAN_POINT ( 'NONE',  ( 0.000000000000000000, 0.000000000000000000, -180.0000000000000568 ) ) ;
#25629=ORIENTED_EDGE ( 'NONE', *, *, #5887, .T. ) ;
#25631=CARTESIAN_POINT ( 'NONE',  ( -2.775557561562891351E-14, -5.500000000000115463, -110.2500000000000142 ) ) ;
#25633=( BOUNDED_CURVE ( )  B_SPLINE_CURVE ( 2, ( #505, #16983, #29528, #5557, #3710, #22015, #22171, #26603, #6601 ),
 .UNSPECIFIED., .F., .T. ) 
 B_SPLINE_CURVE_WITH_KNOTS ( ( 3, 2, 2, 2, 3 ),
 ( 0.1638888888888889728, 0.1648148148148148584, 0.1666666666666666297, 0.1685185185185185119, 0.1694444444444443976 ),
 .UNSPECIFIED. ) 
 CURVE ( )  GEOMETRIC_REPRESENTATION_ITEM ( )  RATIONAL_B_SPLINE_CURVE ( ( 0.9330127018922194093, 0.9330127018922234061, 1.000000000000000000, 0.8660254037844388186, 1.000000000000000000, 0.8660254037844388186, 1.000000000000000000, 0.9330127018922234061, 0.9330127018922194093 ) ) 
 REPRESENTATION_ITEM ( '' )  );
#25634=CARTESIAN_POINT ( 'NONE',  ( 5.412658773652739619, 3.124999999999988898, -134.1830127018922667 ) ) ;
#25636=CARTESIAN_POINT ( 'NONE',  ( -3.608439182435052128, -6.250000000000110134, -168.4419872981078470 ) ) ;
#25637=CARTESIAN_POINT ( 'NONE',  ( 3.608439182435180470, 6.249999999999982236, -179.6919872981078186 ) ) ;
#25638=CARTESIAN_POINT ( 'NONE',  ( 0.5896198263044475363, 5.540201351793478501, -180.0000000000000853 ) ) ;
#25639=CARTESIAN_POINT ( 'NONE',  ( 0.000000000000000000, 5.999999999999977796, -133.2113248654052029 ) ) ;
#25642=CARTESIAN_POINT ( 'NONE',  ( -3.608439182435052128, -6.250000000000110134, -60.44198729810782567 ) ) ;
#25643=CARTESIAN_POINT ( 'NONE',  ( 7.216878364870455975, -6.409875621278545621E-14, -174.8080127018922667 ) ) ;
#25645=CARTESIAN_POINT ( 'NONE',  ( 7.147005652999508048E-33, -5.642372883946980038E-33, -1183.000000000000000 ) ) ;
#25646=CARTESIAN_POINT ( 'NONE',  ( 3.464101615137852974, 5.999999999999884537, -123.4136751345947829 ) ) ;
#25647=CARTESIAN_POINT ( 'NONE',  ( 4.763139720814407951, -2.749999999999988454, -117.5000000000000426 ) ) ;
#25649=ORIENTED_EDGE ( 'NONE', *, *, #4663, .T. ) ;
#25652=CARTESIAN_POINT ( 'NONE',  ( 3.464101615137852974, 5.999999999999884537, -122.8363248654051745 ) ) ;
#25653=CYLINDRICAL_SURFACE ( 'NONE', #23641, 6.000000000000000888 ) ;
#25657=CYLINDRICAL_SURFACE ( 'NONE', #27502, 6.000000000000000888 ) ;
#25658=CARTESIAN_POINT ( 'NONE',  ( -5.412658773652739619, 3.124999999999975131, -110.3169872981077901 ) ) ;
#25660=EDGE_CURVE ( 'NONE', #13261, #24590, #9890, .T. ) ;
#25662=DIRECTION ( 'NONE',  ( -7.147005652999508048E-36, 5.642372883946980038E-36, 1.000000000000000000 ) ) ;
#25664=ORIENTED_EDGE ( 'NONE', *, *, #3301, .F. ) ;
#25667=CARTESIAN_POINT ( 'NONE',  ( 7.216878364870455975, -6.409875621278545621E-14, -142.4419872981078186 ) ) ;
#25670=DIRECTION ( 'NONE',  ( -7.147005652999508048E-36, 5.642372883946980038E-36, 1.000000000000000000 ) ) ;
#25671=CARTESIAN_POINT ( 'NONE',  ( 6.000000000000000888, -1.607695154586752384, -137.2306624327026157 ) ) ;
#25672=CARTESIAN_POINT ( 'NONE',  ( -3.608439182435052128, -6.250000000000110134, -58.30801270189222407 ) ) ;
#25673=FACE_OUTER_BOUND ( 'NONE', #29220, .T. ) ;
#25677=DIRECTION ( 'NONE',  ( -7.147005652999508048E-36, 5.642372883946980038E-36, 1.000000000000000000 ) ) ;
#25679=CARTESIAN_POINT ( 'NONE',  ( -6.000000000000023093, 1.607695154586625819, -114.9033121635129646 ) ) ;
#25681=( BOUNDED_CURVE ( )  B_SPLINE_CURVE ( 2, ( #15633, #27096, #29709, #18078, #27391, #6357, #29860, #28157, #4363 ),
 .UNSPECIFIED., .F., .F. ) 
 B_SPLINE_CURVE_WITH_KNOTS ( ( 3, 2, 2, 2, 3 ),
 ( 0.01944444444444448639, 0.02037037037037037202, 0.02222222222222225430, 0.02407407407407402555, 0.02499999999999991118 ),
 .UNSPECIFIED. ) 
 CURVE ( )  GEOMETRIC_REPRESENTATION_ITEM ( )  RATIONAL_B_SPLINE_CURVE ( ( 0.9330127018922194093, 0.9330127018922234061, 1.000000000000000000, 0.8660254037844388186, 1.000000000000000000, 0.8660254037844388186, 1.000000000000000000, 0.9330127018922234061, 0.9330127018922194093 ) ) 
 REPRESENTATION_ITEM ( '' )  );
#25685=EDGE_CURVE ( 'NONE', #2934, #17032, #2530, .T. ) ;
#25686=CARTESIAN_POINT ( 'NONE',  ( -6.350852961085760029, -1.281975124255709124E-13, -58.12500000000004974 ) ) ;
#25689=CARTESIAN_POINT ( 'NONE',  ( -3.464101615137757051, -5.999999999999979572, -152.0863248654051461 ) ) ;
#25693=CARTESIAN_POINT ( 'NONE',  ( 5.412658773652739619, 3.124999999999988898, -100.3169872981078470 ) ) ;
#25694=CARTESIAN_POINT ( 'NONE',  ( -5.999999999999963585, 9.296355089585909904E-15, -164.3363248654052313 ) ) ;
#25698=CARTESIAN_POINT ( 'NONE',  ( -2.775557561562891351E-14, -5.500000000000115463, -135.7500000000000284 ) ) ;
#25700=VERTEX_POINT ( 'NONE', #20165 ) ;
#25701=CARTESIAN_POINT ( 'NONE',  ( -4.763139720814407951, 2.749999999999946709, -68.75000000000002842 ) ) ;
#25704=CARTESIAN_POINT ( 'NONE',  ( 3.608439182435180470, 6.249999999999982236, -90.55801270189225249 ) ) ;
#25711=CARTESIAN_POINT ( 'NONE',  ( 3.175426480543072749, 5.499999999999865885, -148.6250000000000284 ) ) ;
#25712=DIRECTION ( 'NONE',  ( -7.147005652999508048E-36, 5.642372883946980038E-36, 1.000000000000000000 ) ) ;
#25713=CARTESIAN_POINT ( 'NONE',  ( 0.000000000000000000, 5.499999999999991118, -138.0000000000000000 ) ) ;
#25714=CARTESIAN_POINT ( 'NONE',  ( 5.412658773652739619, 3.124999999999988898, -158.1830127018922667 ) ) ;
#25715=( NAMED_UNIT ( * ) SI_UNIT ( $, .STERADIAN. ) SOLID_ANGLE_UNIT ( ) );
#25716=CARTESIAN_POINT ( 'NONE',  ( -6.000000000000000888, 1.067854986875958443E-15, 7.560779664488942560E-35 ) ) ;
#25718=CARTESIAN_POINT ( 'NONE',  ( 4.763139720814407951, -2.749999999999988454, -75.50000000000001421 ) ) ;
#25721=CARTESIAN_POINT ( 'NONE',  ( -3.175426480542816510, 5.499999999999865885, -68.87500000000002842 ) ) ;
#25722=EDGE_CURVE ( 'NONE', #14585, #11534, #2699, .T. ) ;
#25723=( BOUNDED_CURVE ( )  B_SPLINE_CURVE ( 2, ( #28686, #14479, #2751, #21362, #12026, #3050, #16781, #19513, #10143, #7801, #26546, #16635, #5348, #14333, #9835, #23671, #28543, #12178, #303, #28395, #26250, #7374, #12323, #5201, #602, #9988, #26105, #23813, #21522, #445, #7512, #19365, #18866, #244, #14275, #7316, #9021, #26050, #9326, #4847, #28040, #16578, #1951, #2110, #7011, #11670, #14134, #30358, #21305, #4396, #20854, #30208, #18717, #16428, #9628, #6710, #13665, #13822, #23166, #25752, #16127, #25897, #28187, #19021, #21161, #4700, #11514, #25433, #16726, #23616, #2550, #11977, #23007, #11355, #23320, #20701, #30051, #2410, #18411, #7163, #23472, #18563, #99, #4556, #9168, #11822, #27731, #9483, #2264, #27887, #6858, #16284, #21012, #25603, #13980, #22050, #16870, #19598, #7900, #542, #3285, #14561, #21906, #24045, #700, #21611, #14848, #4993, #12413, #2845, #17012, #7459, #2694, #3137, #24193, #5142, #985, #9933, #12120, #28938, #10239, #21460, #10385, #21757, #19738, #17314, #28785, #10084, #17460, #29085, #23904, #19457, #26630, #23763, #12266, #12559, #5588, #14426, #839, #2992, #19307, #14992, #28627, #7599, #24331, #7749, #26341, #390, #12711, #5289, #8047, #14698, #9781, #19159, #28494, #26191, #17159, #26479, #5438, #8679, #24942, #11153, #22202, #8837, #22518, #18076, #10859, #6355, #3746, #11009, #29394, #29234, #4050, #27093, #29561, #8518, #5892, #29707, #17926, #1135, #13472, #19890, #26775, #26931, #15318, #27242, #8198, #15789, #22663, #10536, #1605, #24482, #27389, #25093, #6061, #6213, #22813, #13181, #24642, #8363, #20354, #17773, #1290, #17613, #15474, #15150, #12863, #10704, #3893, #24798, #3587, #15631, #13018, #20212, #1449, #1756, #29858, #20504, #13324, #5742, #22354, #3432, #20048, #2227, #25397, #4207, #11316, #27691, #4664, #6516, #6672, #11629, #16243, #18678, #4518, #25867, #8985, #4358, #13783, #13940, #20973, #2513, #7122, #27540, #28001, #15939, #14097, #30322, #59, #23432, #4816, #25711, #9283, #18376, #20664, #23577, #28153, #9445, #18827, #11943, #14242, #23127, #30168, #2075, #30015, #27849, #25234, #13624, #11479, #2376, #9132, #16091, #6971, #22972, #16389, #6818, #21121, #21268, #16545, #25557, #11780, #208, #18223, #1909, #20820, #18524, #23286, #2659, #19123, #26454, #28596, #5260, #17128, #16981, #5405, #28901, #3247, #19424, #5556, #12677, #17280, #26602, #26156, #7285, #3103, #14819, #12082, #810, #14960, #21422, #353, #16688, #24161, #5107, #2809, #9747, #23726, #10201, #28454, #24299, #19567, #12529, #9594, #28751, #7564, #23867, #18984, #26010, #21870, #10046, #12234, #21574, #7866, #22014, #14528, #7425, #16834, #504, #14667, #28307, #4957, #24014, #14390, #9899, #19275, #7720, #26305, #2959, #12376, #21724, #664, #5859, #8324, #3860, #5707, #18045, #15753, #20325, #10349, #1416, #19710, #3403, #29674, #27211, #15116, #6184, #29055, #1571, #8641, #10665, #3709, #27359, #17733, #19856, #12985, #15597, #26895, #22320, #15277, #24449, #20010, #10824, #26740, #29361, #24604, #24767, #27058, #25061, #20175, #4018, #8485, #12826, #6023, #24912, #15441, #13293, #22632, #10979, #29527, #13142, #8164, #6325, #13435, #948, #8022, #17580, #17893, #17426, #22480, #29202, #1255, #22170, #1105, #10502, #3555, #22937, #9823, #8958, #20469, #16768, #27965, #8804, #19200, #9100, #28529, #5034, #16211, #30138, #5189, #7498, #1877, #6789, #7362, #11121, #11282, #20940, #26094, #22782, #11598, #20791, #6642, #14467, #18349, #20635, #30290, #25522, #29980, #1726, #23800, #27662, #2734, #13750, #26236, #2192, #9251, #435, #27817, #29828, #16063, #12162, #18646, #16910, #18193, #27508, #18497, #21509, #4485, #6487, #13909, #15912, #25363, #25208, #4174, #23096, #23254, #13595, #4332, #2040, #11447, #19936, #24528, #882, #3039, #26533, #19782, #10131, #5484, #19500, #7648, #24231, #2891, #589, #28830, #22098, #14890, #17057, #15039, #9976, #28982, #3182, #17504, #3477, #12604, #3330, #5334, #1175, #26388, #29130, #26819, #7791, #12909, #8241, #22246, #8090, #747, #24386, #14601, #21947, #12456, #10280, #24089, #10583, #17653, #29282, #26977, #23953, #19353, #5782, #21799, #19643, #17206, #12311, #7949, #21654, #26673, #5634, #12757, #1032, #10432, #6105, #20389, #24840, #1956, #6558, #11361, #20706, #18265, #11200, #15976, #29601, #27576, #22557, #3788, #4094, #8722, #1488, #5942, #25276, #10899, #4247, #27279, #1645, #15364, #13669, #23011, #22705, #20253, #20546, #30055, #9025, #24688, #1337, #3630, #11043, #13067, #29746, #22398, #13360, #29899, #8561, #8409, #6396, #18110, #10749, #27136, #17966, #6253, #15830, #25129, #20093, #29437, #17816, #15671, #24980, #13516, #22854, #1794, #8877, #11518, #23621, #25437, #27891, #20859, #27735, #9634, #2269, #19027, #18721, #396, #7167, #16583, #4998, #2414, #9786, #21015, #28345, #25902, #14430, #4853, #4402, #30363, #16730, #11828, #26054, #4704, #11980, #7016, #30211, #12124, #16433, #106, #9487, #16287, #251, #18870, #2114, #21468, #13826, #23172, #9173, #28193, #14279, #18568, #4561, #2554, #13984, #21309, #23324, #25757, #14138, #23477, #21165, #15155, #5442, #7604, #705, #24336, #14706, #10091, #24050, #12272, #3290, #28943, #14564, #7753, #2996, #12565, #17164, #3436, #7905, #12867, #26635, #2853, #24196, #14996, #14853, #12716, #10392, #22055, #17319, #3142, #12417, #17464, #22207, #26779, #990, #5293, #5593, #19164, #26486, #17017, #19461, #21616, #16875, #19743, #29089, #19313, #24487, #21761, #26195, #8050, #28791, #5147, #1142, #21910, #28498, #7463, #843, #10245, #23909, #548, #28633, #19602, #9937, #26345, #20052, #8683, #13477, #10541, #29711, #8522, #3751, #22816, #27097, #29399, #18080, #13327, #17778, #17929, #24804, #19897, #17618, #4053, #11011, #13186, #22521, #1760, #29862, #6066, #8368, #15477, #13629, #20357, #27392, #18226, #15634, #22976, #1454, #11158, #6359, #27543, #15792, #29239, #10862, #25097, #29564, #27246, #20507, #8202, #6218, #24944, #6519, #3897, #22666, #1609, #8841, #15942, #25240, #15326, #4212, #26939, #5897, #24646, #3593, #13023, #22360, #1294, #10709, #7128, #9599, #9451, #2519, #213, #11635, #4668, #28312, #18683, #20825, #13946, #16551, #27854, #23291, #6824, #25402, #20981, #30021, #18380, #16249, #18832, #2233, #4364, #27696, #16395, #30328, #14246, #4964, #21272, #9289, #21127, #23134, #18988, #13789, #25872, #23582, #25565, #7290, #26015, #16693, #11949, #18531, #11787, #28007, #28159, #14395, #1915, #65, #11323, #8991, #6678, #16096, #2078, #11483, #30174, #9139, #6979, #4524, #25718, #14102, #23438, #2381, #17132, #9904, #16987, #16840, #7430, #24304, #12239, #19715, #3253, #29059, #8025, #5561, #28906, #26159, #28756, #19572, #10054, #7871, #14964, #26607, #12533, #12683, #19280, #22018, #17430, #952, #17285, #28602, #3108, #23731, #668, #21578, #5264, #5111, #21427, #21875, #813, #23872, #10354, #7571, #357, #14531, #14673, #9751, #26745, #19429, #5711, #2664, #26458, #7725, #12087, #19127, #2816, #5410, #28459, #509, #26310, #10206, #24017, #2963, #12382, #21729, #14823, #24166, #1260, #24609, #13295, #17897, #22325, #15121, #27364, #20016, #6329, #6028, #18196, #24917, #3866, #22787, #20181, #27513, #29365, #1729, #15758, #29833, #10506, #24452, #10829, #25065, #29534, #4022, #22487, #29677, #17738, #17584, #11125, #15446, #27214, #6188, #3559, #18050, #15603, #22636, #20473, #8168, #3407, #15282, #12990, #1576, #26901, #13441, #10983, #29206, #20328, #12830, #8810, #22174, #24773, #8646, #1108, #1421, #10670, #19860, #3716, #5863, #8329, #27063, #13147, #8490, #16364, #1881, #25527, #2047, #30295, #4491, #21242, #25686, #184, #14070, #23259, #25370, #18502, #16216, #9415, #18959, #4637, #25215, #21099, #23405, #11287, #13914, #11452, #9257, #2198, #9566, #2351, #6491, #11752, #20640, #11602, #27, #20944, #27668, #23553, #18352, #18802, #28128, #20796, #4788, #15917, #14212, #7097, #23101, #16515, #4180, #18652, #4335, #27823, #8963, #13598, #25841, #2490, #22942, #11913, #29987, #6648, #16067, #6793, #13755, #30144, #27971, #9106, #6946, #21697, #5229, #10320, #24271, #28425, #12348, #12502, #16663, #7403, #3219, #12644, #10172, #3078, #7838, #21548, #19541, #14504, #16811, #26426, #634, #5077, #28276, #28874, #2780, #17250, #19246, #921, #7690, #17098, #26575, #14642, #12208, #21841, #14933, #5528, #21988, #23701 ),
 .UNSPECIFIED., .F., .T. ) 
 B_SPLINE_CURVE_WITH_KNOTS ( ( 3, 2, 2, 2, 2, 2, 2, 2, 2, 2, 2, 2, 2, 2, 2, 2, 2, 2, 2, 2, 2, 2, 2, 2, 2, 2, 2, 2, 2, 2, 2, 2, 2, 2, 2, 2, 2, 2, 2, 2, 2, 2, 2, 2, 2, 2, 2, 2, 2, 2, 2, 2, 2, 2, 2, 2, 2, 2, 2, 2, 2, 2, 2, 2, 2, 2, 2, 2, 2, 2, 2, 2, 2, 2, 2, 2, 2, 2, 2, 2, 2, 2, 2, 2, 2, 2, 2, 2, 2, 2, 2, 2, 2, 2, 2, 2, 2, 2, 2, 2, 2, 2, 2, 2, 2, 2, 2, 2, 2, 2, 2, 2, 2, 2, 2, 2, 2, 2, 2, 2, 2, 2, 2, 2, 2, 2, 2, 2, 2, 2, 2, 2, 2, 2, 2, 2, 2, 2, 2, 2, 2, 2, 2, 2, 2, 2, 2, 2, 2, 2, 2, 2, 2, 2, 2, 2, 2, 2, 2, 2, 2, 2, 2, 2, 2, 2, 2, 2, 2, 2, 2, 2, 2, 2, 2, 2, 2, 2, 2, 2, 2, 2, 2, 2, 2, 2, 2, 2, 2, 2, 2, 2, 2, 2, 2, 2, 2, 2, 2, 2, 2, 2, 2, 2, 2, 2, 2, 2, 2, 2, 2, 2, 2, 2, 2, 2, 2, 2, 2, 2, 2, 2, 2, 2, 2, 2, 2, 2, 2, 2, 2, 2, 2, 2, 2, 2, 2, 2, 2, 2, 2, 2, 2, 2, 2, 2, 2, 2, 2, 2, 2, 2, 2, 2, 2, 2, 2, 2, 2, 2, 2, 2, 2, 2, 2, 2, 2, 2, 2, 2, 2, 2, 2, 2, 2, 2, 2, 2, 2, 2, 2, 2, 2, 2, 2, 2, 2, 2, 2, 2, 2, 2, 2, 2, 2, 2, 2, 2, 2, 2, 2, 2, 2, 2, 2, 2, 2, 2, 2, 2, 2, 2, 2, 2, 2, 2, 2, 2, 2, 2, 2, 2, 2, 2, 2, 2, 2, 2, 2, 2, 2, 2, 2, 2, 2, 2, 2, 2, 2, 2, 2, 2, 2, 2, 2, 2, 2, 2, 2, 2, 2, 2, 2, 2, 2, 2, 2, 2, 2, 2, 2, 2, 2, 2, 2, 2, 2, 2, 2, 2, 2, 2, 2, 2, 2, 2, 2, 2, 2, 2, 2, 2, 2, 2, 2, 2, 2, 2, 2, 2, 2, 2, 2, 2, 2, 2, 2, 2, 2, 2, 2, 2, 2, 2, 2, 2, 2, 2, 2, 2, 2, 2, 2, 2, 2, 2, 2, 2, 2, 2, 2, 2, 2, 2, 2, 2, 2, 2, 2, 2, 2, 2, 2, 2, 2, 2, 2, 2, 2, 2, 2, 2, 2, 2, 2, 2, 2, 2, 2, 2, 2, 2, 2, 2, 2, 2, 2, 2, 2, 2, 2, 2, 2, 2, 2, 2, 2, 2, 2, 2, 2, 2, 2, 2, 2, 2, 2, 2, 2, 2, 2, 2, 2, 2, 2, 2, 2, 2, 2, 2, 2, 2, 2, 2, 2, 2, 2, 2, 2, 2, 2, 2, 2, 2, 2, 2, 2, 2, 2, 2, 2, 2, 2, 2, 2, 2, 2, 2, 2, 2, 2, 2, 2, 2, 2, 2, 2, 2, 2, 2, 2, 2, 2, 2, 3 ),
 ( 0.01111111111111070908, 0.01296296296296256013, 0.01481481481481441466, 0.01666666666666626745, 0.01851851851851811850, 0.02037037037036997303, 0.02222222222222182408, 0.02407407407407367861, 0.02592592592592552619, 0.02777777777777737378, 0.02962962962962923524, 0.03148148148148108283, 0.03333333333333293735, 0.03518518518518479188, 0.03703703703703663946, 0.03888888888888849399, 0.04074074074074034851, 0.04259259259259220304, 0.04444444444444405062, 0.04629629629629590515, 0.04814814814814775967, 0.04999999999999961420, 0.05185185185185146178, 0.05370370370370331631, 0.05555555555555517083, 0.05740740740740701842, 0.05925925925925887988, 0.06111111111111072053, 0.06296296296296256811, 0.06481481481481442264, 0.06666666666666627716, 0.06851851851851813169, 0.07037037037036998621, 0.07222222222222182686, 0.07407407407407369526, 0.07592592592592554979, 0.07777777777777739043, 0.07962962962962924496, 0.08148148148148111336, 0.08333333333333295401, 0.08518518518518480853, 0.08703703703703666306, 0.08888888888888851758, 0.09074074074074037211, 0.09259259259259221275, 0.09444444444444406728, 0.09629629629629592180, 0.09814814814814777633, 0.09999999999999964473, 0.1018518518518514715, 0.1037037037037033260, 0.1055555555555551805, 0.1074074074074070489, 0.1092592592592588896, 0.1111111111111107302, 0.1129629629629625986, 0.1148148148148144532, 0.1166666666666662938, 0.1185185185185181483, 0.1203703703703700029, 0.1222222222222218574, 0.1240740740740737119, 0.1259259259259255248, 0.1277777777777774071, 0.1296296296296292616, 0.1314814814814811161, 0.1333333333333329707, 0.1351851851851848252, 0.1370370370370367075, 0.1388888888888885620, 0.1407407407407404165, 0.1425925925925922710, 0.1444444444444440701, 0.1462962962962959246, 0.1481481481481477791, 0.1499999999999996614, 0.1518518518518515159, 0.1537037037037033704, 0.1555555555555552250, 0.1574074074074070795, 0.1592592592592589340, 0.1611111111111107608, 0.1629629629629626431, 0.1648148148148144698, 0.1666666666666663243, 0.1685185185185181789, 0.1703703703703700334, 0.1722222222222218879, 0.1740740740740737424, 0.1759259259259255970, 0.1777777777777774515, 0.1796296296296293060, 0.1814814814814811605, 0.1833333333333329873, 0.1851851851851848418, 0.1870370370370366964, 0.1888888888888885786, 0.1907407407407404054, 0.1925925925925922599, 0.1944444444444441145, 0.1962962962962959690, 0.1981481481481478235, 0.1999999999999996780, 0.2018518518518515603, 0.2037037037037033871, 0.2055555555555552416, 0.2074074074074070684, 0.2092592592592589229, 0.2111111111111107774, 0.2129629629629626320, 0.2148148148148145142, 0.2166666666666663688, 0.2185185185185182233, 0.2203703703703700778, 0.2222222222222218768, 0.2240740740740737313, 0.2259259259259255859, 0.2277777777777774404, 0.2296296296296293227, 0.2314814814814811772, 0.2333333333333330317, 0.2351851851851848862, 0.2370370370370367408, 0.2388888888888885675, 0.2407407407407403943, 0.2425925925925922766, 0.2444444444444441311, 0.2462962962962959856, 0.2481481481481478402, 0.2499999999999996947, 0.2518518518518514937, 0.2537037037037033760, 0.2555555555555552028, 0.2574074074074070850, 0.2592592592592589118, 0.2611111111111107941, 0.2629629629629626208, 0.2648148148148144476, 0.2666666666666663299, 0.2685185185185181567, 0.2703703703703700389, 0.2722222222222218102, 0.2740740740740737480, 0.2759259259259255748, 0.2777777777777774015, 0.2796296296296292838, 0.2814814814814811106, 0.2833333333333329929, 0.2851851851851848196, 0.2870370370370367019, 0.2888888888888885287, 0.2907407407407404110, 0.2925925925925922377, 0.2944444444444440645, 0.2962962962962959468, 0.2981481481481477736, 0.2999999999999996558, 0.3018518518518515381, 0.3037037037037033649, 0.3055555555555552472, 0.3074074074074070739, 0.3092592592592589007, 0.3111111111111107275, 0.3129629629629626097, 0.3148148148148144920, 0.3166666666666663188, 0.3185185185185182011, 0.3203703703703700278, 0.3222222222222219101, 0.3240740740740736814, 0.3259259259259256192, 0.3277777777777774459, 0.3296296296296292727, 0.3314814814814811550, 0.3333333333333329818, 0.3351851851851848640, 0.3370370370370366908, 0.3388888888888885731, 0.3407407407407403999, 0.3425925925925922821, 0.3444444444444441089, 0.3462962962962959357, 0.3481481481481478180, 0.3499999999999996447, 0.3518518518518515270, 0.3537037037037034093, 0.3555555555555552361, 0.3574074074074070628, 0.3592592592592589451, 0.3611111111111107719, 0.3629629629629626542, 0.3648148148148144809, 0.3666666666666663632, 0.3685185185185181900, 0.3703703703703700723, 0.3722222222222218990, 0.3740740740740737258, 0.3759259259259256081, 0.3777777777777774348, 0.3796296296296293726, 0.3814814814814811439, 0.3833333333333330817, 0.3851851851851848529, 0.3870370370370366797, 0.3888888888888885620, 0.3907407407407403888, 0.3925925925925923266, 0.3944444444444440978, 0.3962962962962960356, 0.3981481481481478069, 0.3999999999999997446, 0.4018518518518515159, 0.4037037037037033982, 0.4055555555555552805, 0.4074074074074070517, 0.4092592592592589895, 0.4111111111111107608, 0.4129629629629626986, 0.4148148148148144698, 0.4166666666666664076, 0.4185185185185182344, 0.4203703703703700612, 0.4222222222222219434, 0.4240740740740737147, 0.4259259259259256525, 0.4277777777777774237, 0.4296296296296293615, 0.4314814814814811328, 0.4333333333333330151, 0.4351851851851848973, 0.4370370370370367241, 0.4388888888888886064, 0.4407407407407404332, 0.4425925925925923154, 0.4444444444444440867, 0.4462962962962960245, 0.4481481481481478513, 0.4499999999999996780, 0.4518518518518515603, 0.4537037037037033871, 0.4555555555555552694, 0.4574074074074070961, 0.4592592592592589784, 0.4611111111111108607, 0.4629629629629626875, 0.4648148148148145142, 0.4666666666666663410, 0.4685185185185182233, 0.4703703703703700501, 0.4722222222222219323, 0.4740740740740738146, 0.4759259259259256414, 0.4777777777777775237, 0.4796296296296293504, 0.4814814814814811772, 0.4833333333333330040, 0.4851851851851848862, 0.4870370370370367685, 0.4888888888888885953, 0.4907407407407404776, 0.4925925925925923043, 0.4944444444444441866, 0.4962962962962959579, 0.4981481481481478957, 0.4999999999999997224, 0.5018518518518516602, 0.5037037037037034315, 0.5055555555555553138, 0.5074074074074071961, 0.5092592592592590783, 0.5111111111111108496, 0.5129629629629627319, 0.5148148148148147252, 0.5166666666666664964, 0.5185185185185182677, 0.5203703703703702610, 0.5222222222222221433, 0.5240740740740739145, 0.5259259259259256858, 0.5277777777777775681, 0.5296296296296295614, 0.5314814814814813326, 0.5333333333333331039, 0.5351851851851849862, 0.5370370370370369795, 0.5388888888888887507, 0.5407407407407406330, 0.5425925925925924043, 0.5444444444444441755, 0.5462962962962961688, 0.5481481481481480511, 0.5499999999999999334, 0.5518518518518515936, 0.5537037037037035869, 0.5555555555555554692, 0.5574074074074073515, 0.5592592592592590117, 0.5611111111111108940, 0.5629629629629628873, 0.5648148148148146586, 0.5666666666666665408, 0.5685185185185183121, 0.5703703703703703054, 0.5722222222222220767, 0.5740740740740739589, 0.5759259259259258412, 0.5777777777777775015, 0.5796296296296294948, 0.5814814814814813770, 0.5833333333333332593, 0.5851851851851849196, 0.5870370370370369129, 0.5888888888888887951, 0.5907407407407406774, 0.5925925925925924487, 0.5944444444444442199, 0.5962962962962962132, 0.5981481481481479845, 0.5999999999999998668, 0.6018518518518516380, 0.6037037037037036313, 0.6055555555555554026, 0.6074074074074072849, 0.6092592592592591672, 0.6111111111111109384, 0.6129629629629628207, 0.6148148148148147030, 0.6166666666666665853, 0.6185185185185183565, 0.6203703703703701278, 0.6222222222222221211, 0.6240740740740740033, 0.6259259259259257746, 0.6277777777777775459, 0.6296296296296295392, 0.6314814814814814214, 0.6333333333333331927, 0.6351851851851850750, 0.6370370370370368462, 0.6388888888888887285, 0.6407407407407406108, 0.6425925925925924931, 0.6444444444444443754, 0.6462962962962961466, 0.6481481481481480289, 0.6499999999999999112, 0.6518518518518517935, 0.6537037037037034537, 0.6555555555555554470, 0.6574074074074073293, 0.6592592592592591005, 0.6611111111111109828, 0.6629629629629628651, 0.6648148148148147474, 0.6666666666666665186, 0.6685185185185184009, 0.6703703703703702832, 0.6722222222222221655, 0.6740740740740739367, 0.6759259259259258190, 0.6777777777777777013, 0.6796296296296294726, 0.6814814814814813548, 0.6833333333333332371, 0.6851851851851851194, 0.6870370370370368907, 0.6888888888888887729, 0.6907407407407406552, 0.6925925925925924265, 0.6944444444444443088, 0.6962962962962963021, 0.6981481481481480733, 0.6999999999999998446, 0.7018518518518517268, 0.7037037037037036091, 0.7055555555555554914, 0.7074074074074072627, 0.7092592592592591449, 0.7111111111111110272, 0.7129629629629629095, 0.7148148148148146808, 0.7166666666666665630, 0.7185185185185184453, 0.7203703703703702166, 0.7222222222222222099, 0.7240740740740739811, 0.7259259259259258634, 0.7277777777777776347, 0.7296296296296295170, 0.7314814814814813992, 0.7333333333333331705, 0.7351851851851850528, 0.7370370370370369351, 0.7388888888888889284, 0.7407407407407405886, 0.7425925925925924709, 0.7444444444444443532, 0.7462962962962962354, 0.7481481481481481177, 0.7499999999999998890, 0.7518518518518517713, 0.7537037037037035425, 0.7555555555555555358, 0.7574074074074073071, 0.7592592592592591894, 0.7611111111111109606, 0.7629629629629628429, 0.7648148148148148362, 0.7666666666666666075, 0.7685185185185183787, 0.7703703703703702610, 0.7722222222222222543, 0.7740740740740740256, 0.7759259259259257968, 0.7777777777777776791, 0.7796296296296295614, 0.7814814814814814437, 0.7833333333333332149, 0.7851851851851850972, 0.7870370370370369795, 0.7888888888888888618, 0.7907407407407407440, 0.7925925925925925153, 0.7944444444444442865, 0.7962962962962961688, 0.7981481481481481621, 0.8000000000000000444, 0.8018518518518517046, 0.8037037037037035869, 0.8055555555555555802, 0.8074074074074074625, 0.8092592592592591227, 0.8111111111111110050, 0.8129629629629628873, 0.8148148148148147696, 0.8166666666666666519, 0.8185185185185184231, 0.8203703703703703054, 0.8222222222222221877, 0.8240740740740740700, 0.8259259259259259522, 0.8277777777777776125, 0.8296296296296294948, 0.8314814814814814881, 0.8333333333333333703, 0.8351851851851850306, 0.8370370370370369129, 0.8388888888888887951, 0.8407407407407407884, 0.8425925925925925597, 0.8444444444444443310, 0.8462962962962962132, 0.8481481481481480955, 0.8499999999999999778, 0.8518518518518518601, 0.8537037037037036313, 0.8555555555555554026, 0.8574074074074073959, 0.8592592592592592782, 0.8611111111111110494, 0.8629629629629628207, 0.8648148148148148140, 0.8666666666666666963, 0.8685185185185184675, 0.8703703703703702388, 0.8722222222222221211, 0.8740740740740741144, 0.8759259259259258856, 0.8777777777777776569, 0.8796296296296295392, 0.8814814814814815325, 0.8833333333333333037, 0.8851851851851851860, 0.8870370370370369573, 0.8888888888888887285, 0.8907407407407407218, 0.8925925925925926041, 0.8944444444444444864, 0.8962962962962961466, 0.8981481481481481399, 0.9000000000000000222, 0.9018518518518519045, 0.9037037037037035647, 0.9055555555555554470, 0.9074074074074074403, 0.9092592592592592116, 0.9111111111111110938, 0.9129629629629628651, 0.9148148148148148584, 0.9166666666666666297, 0.9185185185185185119, 0.9203703703703703942, 0.9222222222222221655, 0.9240740740740740478, 0.9259259259259259300, 0.9277777777777778123, 0.9296296296296294726, 0.9314814814814814659, 0.9333333333333333481, 0.9351851851851852304, 0.9370370370370370017, 0.9388888888888887729, 0.9407407407407407662, 0.9425925925925925375, 0.9444444444444444198, 0.9462962962962963021, 0.9481481481481480733, 0.9499999999999999556, 0.9518518518518518379, 0.9537037037037037202, 0.9555555555555554914, 0.9574074074074073737, 0.9592592592592592560, 0.9611111111111111382, 0.9629629629629629095, 0.9648148148148146808, 0.9666666666666666741, 0.9685185185185185563, 0.9703703703703703276, 0.9722222222222222099, 0.9740740740740740922, 0.9759259259259259744, 0.9777777777777777457, 0.9796296296296296280, 0.9814814814814813992, 0.9833333333333332815, 0.9851851851851851638, 0.9870370370370370461, 0.9888888888888889284, 0.9907407407407406996, 0.9925925925925925819, 0.9944444444444444642, 0.9962962962962963465, 0.9981481481481481177, 1.000000000000000000 ),
 .UNSPECIFIED. ) 
 CURVE ( )  GEOMETRIC_REPRESENTATION_ITEM ( )  RATIONAL_B_SPLINE_CURVE ( ( 1.000000000000029088, 0.8660254037844096198, 1.000000000000000000, 0.8660254037844387076, 1.000000000000000000, 0.8660254037844387076, 1.000000000000000000, 0.8660254037844387076, 1.000000000000000000, 0.8660254037844387076, 1.000000000000000000, 0.8660254037844387076, 1.000000000000000000, 0.8660254037844387076, 1.000000000000000000, 0.8660254037844387076, 1.000000000000000000, 0.8660254037844387076, 1.000000000000000000, 0.8660254037844387076, 1.000000000000000000, 0.8660254037844387076, 1.000000000000000000, 0.8660254037844387076, 1.000000000000000000, 0.8660254037844387076, 1.000000000000000000, 0.8660254037844387076, 1.000000000000000000, 0.8660254037844387076, 1.000000000000000000, 0.8660254037844387076, 1.000000000000000000, 0.8660254037844387076, 1.000000000000000000, 0.8660254037844387076, 1.000000000000000000, 0.8660254037844387076, 1.000000000000000000, 0.8660254037844387076, 1.000000000000000000, 0.8660254037844387076, 1.000000000000000000, 0.8660254037844387076, 1.000000000000000000, 0.8660254037844387076, 1.000000000000000000, 0.8660254037844387076, 1.000000000000000000, 0.8660254037844387076, 1.000000000000000000, 0.8660254037844387076, 1.000000000000000000, 0.8660254037844387076, 1.000000000000000000, 0.8660254037844387076, 1.000000000000000000, 0.8660254037844387076, 1.000000000000000000, 0.8660254037844387076, 1.000000000000000000, 0.8660254037844387076, 1.000000000000000000, 0.8660254037844387076, 1.000000000000000000, 0.8660254037844387076, 1.000000000000000000, 0.8660254037844387076, 1.000000000000000000, 0.8660254037844387076, 1.000000000000000000, 0.8660254037844387076, 1.000000000000000000, 0.8660254037844387076, 1.000000000000000000, 0.8660254037844387076, 1.000000000000000000, 0.8660254037844387076, 1.000000000000000000, 0.8660254037844387076, 1.000000000000000000, 0.8660254037844387076, 1.000000000000000000, 0.8660254037844387076, 1.000000000000000000, 0.8660254037844387076, 1.000000000000000000, 0.8660254037844387076, 1.000000000000000000, 0.8660254037844387076, 1.000000000000000000, 0.8660254037844387076, 1.000000000000000000, 0.8660254037844387076, 1.000000000000000000, 0.8660254037844387076, 1.000000000000000000, 0.8660254037844387076, 1.000000000000000000, 0.8660254037844387076, 1.000000000000000000, 0.8660254037844387076, 1.000000000000000000, 0.8660254037844387076, 1.000000000000000000, 0.8660254037844387076, 1.000000000000000000, 0.8660254037844387076, 1.000000000000000000, 0.8660254037844387076, 1.000000000000000000, 0.8660254037844387076, 1.000000000000000000, 0.8660254037844387076, 1.000000000000000000, 0.8660254037844387076, 1.000000000000000000, 0.8660254037844387076, 1.000000000000000000, 0.8660254037844387076, 1.000000000000000000, 0.8660254037844387076, 1.000000000000000000, 0.8660254037844387076, 1.000000000000000000, 0.8660254037844387076, 1.000000000000000000, 0.8660254037844387076, 1.000000000000000000, 0.8660254037844387076, 1.000000000000000000, 0.8660254037844387076, 1.000000000000000000, 0.8660254037844387076, 1.000000000000000000, 0.8660254037844387076, 1.000000000000000000, 0.8660254037844387076, 1.000000000000000000, 0.8660254037844387076, 1.000000000000000000, 0.8660254037844387076, 1.000000000000000000, 0.8660254037844387076, 1.000000000000000000, 0.8660254037844387076, 1.000000000000000000, 0.8660254037844387076, 1.000000000000000000, 0.8660254037844387076, 1.000000000000000000, 0.8660254037844387076, 1.000000000000000000, 0.8660254037844387076, 1.000000000000000000, 0.8660254037844387076, 1.000000000000000000, 0.8660254037844387076, 1.000000000000000000, 0.8660254037844387076, 1.000000000000000000, 0.8660254037844387076, 1.000000000000000000, 0.8660254037844387076, 1.000000000000000000, 0.8660254037844387076, 1.000000000000000000, 0.8660254037844387076, 1.000000000000000000, 0.8660254037844387076, 1.000000000000000000, 0.8660254037844387076, 1.000000000000000000, 0.8660254037844387076, 1.000000000000000000, 0.8660254037844387076, 1.000000000000000000, 0.8660254037844387076, 1.000000000000000000, 0.8660254037844387076, 1.000000000000000000, 0.8660254037844387076, 1.000000000000000000, 0.8660254037844387076, 1.000000000000000000, 0.8660254037844387076, 1.000000000000000000, 0.8660254037844387076, 1.000000000000000000, 0.8660254037844387076, 1.000000000000000000, 0.8660254037844387076, 1.000000000000000000, 0.8660254037844387076, 1.000000000000000000, 0.8660254037844387076, 1.000000000000000000, 0.8660254037844387076, 1.000000000000000000, 0.8660254037844387076, 1.000000000000000000, 0.8660254037844387076, 1.000000000000000000, 0.8660254037844387076, 1.000000000000000000, 0.8660254037844387076, 1.000000000000000000, 0.8660254037844387076, 1.000000000000000000, 0.8660254037844387076, 1.000000000000000000, 0.8660254037844387076, 1.000000000000000000, 0.8660254037844387076, 1.000000000000000000, 0.8660254037844387076, 1.000000000000000000, 0.8660254037844387076, 1.000000000000000000, 0.8660254037844387076, 1.000000000000000000, 0.8660254037844387076, 1.000000000000000000, 0.8660254037844387076, 1.000000000000000000, 0.8660254037844387076, 1.000000000000000000, 0.8660254037844387076, 1.000000000000000000, 0.8660254037844387076, 1.000000000000000000, 0.8660254037844387076, 1.000000000000000000, 0.8660254037844387076, 1.000000000000000000, 0.8660254037844387076, 1.000000000000000000, 0.8660254037844387076, 1.000000000000000000, 0.8660254037844387076, 1.000000000000000000, 0.8660254037844387076, 1.000000000000000000, 0.8660254037844387076, 1.000000000000000000, 0.8660254037844387076, 1.000000000000000000, 0.8660254037844387076, 1.000000000000000000, 0.8660254037844387076, 1.000000000000000000, 0.8660254037844387076, 1.000000000000000000, 0.8660254037844387076, 1.000000000000000000, 0.8660254037844387076, 1.000000000000000000, 0.8660254037844387076, 1.000000000000000000, 0.8660254037844387076, 1.000000000000000000, 0.8660254037844387076, 1.000000000000000000, 0.8660254037844387076, 1.000000000000000000, 0.8660254037844387076, 1.000000000000000000, 0.8660254037844387076, 1.000000000000000000, 0.8660254037844387076, 1.000000000000000000, 0.8660254037844387076, 1.000000000000000000, 0.8660254037844387076, 1.000000000000000000, 0.8660254037844387076, 1.000000000000000000, 0.8660254037844387076, 1.000000000000000000, 0.8660254037844387076, 1.000000000000000000, 0.8660254037844387076, 1.000000000000000000, 0.8660254037844387076, 1.000000000000000000, 0.8660254037844387076, 1.000000000000000000, 0.8660254037844387076, 1.000000000000000000, 0.8660254037844387076, 1.000000000000000000, 0.8660254037844387076, 1.000000000000000000, 0.8660254037844387076, 1.000000000000000000, 0.8660254037844387076, 1.000000000000000000, 0.8660254037844387076, 1.000000000000000000, 0.8660254037844387076, 1.000000000000000000, 0.8660254037844387076, 1.000000000000000000, 0.8660254037844387076, 1.000000000000000000, 0.8660254037844387076, 1.000000000000000000, 0.8660254037844387076, 1.000000000000000000, 0.8660254037844387076, 1.000000000000000000, 0.8660254037844387076, 1.000000000000000000, 0.8660254037844387076, 1.000000000000000000, 0.8660254037844387076, 1.000000000000000000, 0.8660254037844387076, 1.000000000000000000, 0.8660254037844387076, 1.000000000000000000, 0.8660254037844387076, 1.000000000000000000, 0.8660254037844387076, 1.000000000000000000, 0.8660254037844387076, 1.000000000000000000, 0.8660254037844387076, 1.000000000000000000, 0.8660254037844387076, 1.000000000000000000, 0.8660254037844387076, 1.000000000000000000, 0.8660254037844387076, 1.000000000000000000, 0.8660254037844387076, 1.000000000000000000, 0.8660254037844387076, 1.000000000000000000, 0.8660254037844387076, 1.000000000000000000, 0.8660254037844387076, 1.000000000000000000, 0.8660254037844387076, 1.000000000000000000, 0.8660254037844387076, 1.000000000000000000, 0.8660254037844387076, 1.000000000000000000, 0.8660254037844387076, 1.000000000000000000, 0.8660254037844387076, 1.000000000000000000, 0.8660254037844387076, 1.000000000000000000, 0.8660254037844387076, 1.000000000000000000, 0.8660254037844387076, 1.000000000000000000, 0.8660254037844387076, 1.000000000000000000, 0.8660254037844387076, 1.000000000000000000, 0.8660254037844387076, 1.000000000000000000, 0.8660254037844387076, 1.000000000000000000, 0.8660254037844387076, 1.000000000000000000, 0.8660254037844387076, 1.000000000000000000, 0.8660254037844387076, 1.000000000000000000, 0.8660254037844387076, 1.000000000000000000, 0.8660254037844387076, 1.000000000000000000, 0.8660254037844387076, 1.000000000000000000, 0.8660254037844387076, 1.000000000000000000, 0.8660254037844387076, 1.000000000000000000, 0.8660254037844387076, 1.000000000000000000, 0.8660254037844387076, 1.000000000000000000, 0.8660254037844387076, 1.000000000000000000, 0.8660254037844387076, 1.000000000000000000, 0.8660254037844387076, 1.000000000000000000, 0.8660254037844387076, 1.000000000000000000, 0.8660254037844387076, 1.000000000000000000, 0.8660254037844387076, 1.000000000000000000, 0.8660254037844387076, 1.000000000000000000, 0.8660254037844387076, 1.000000000000000000, 0.8660254037844387076, 1.000000000000000000, 0.8660254037844387076, 1.000000000000000000, 0.8660254037844387076, 1.000000000000000000, 0.8660254037844387076, 1.000000000000000000, 0.8660254037844387076, 1.000000000000000000, 0.8660254037844387076, 1.000000000000000000, 0.8660254037844387076, 1.000000000000000000, 0.8660254037844387076, 1.000000000000000000, 0.8660254037844387076, 1.000000000000000000, 0.8660254037844387076, 1.000000000000000000, 0.8660254037844387076, 1.000000000000000000, 0.8660254037844387076, 1.000000000000000000, 0.8660254037844387076, 1.000000000000000000, 0.8660254037844387076, 1.000000000000000000, 0.8660254037844387076, 1.000000000000000000, 0.8660254037844387076, 1.000000000000000000, 0.8660254037844387076, 1.000000000000000000, 0.8660254037844387076, 1.000000000000000000, 0.8660254037844387076, 1.000000000000000000, 0.8660254037844387076, 1.000000000000000000, 0.8660254037844387076, 1.000000000000000000, 0.8660254037844387076, 1.000000000000000000, 0.8660254037844387076, 1.000000000000000000, 0.8660254037844387076, 1.000000000000000000, 0.8660254037844387076, 1.000000000000000000, 0.8660254037844387076, 1.000000000000000000, 0.8660254037844387076, 1.000000000000000000, 0.8660254037844387076, 1.000000000000000000, 0.8660254037844387076, 1.000000000000000000, 0.8660254037844387076, 1.000000000000000000, 0.8660254037844387076, 1.000000000000000000, 0.8660254037844387076, 1.000000000000000000, 0.8660254037844387076, 1.000000000000000000, 0.8660254037844387076, 1.000000000000000000, 0.8660254037844387076, 1.000000000000000000, 0.8660254037844387076, 1.000000000000000000, 0.8660254037844387076, 1.000000000000000000, 0.8660254037844387076, 1.000000000000000000, 0.8660254037844387076, 1.000000000000000000, 0.8660254037844387076, 1.000000000000000000, 0.8660254037844387076, 1.000000000000000000, 0.8660254037844387076, 1.000000000000000000, 0.8660254037844387076, 1.000000000000000000, 0.8660254037844387076, 1.000000000000000000, 0.8660254037844387076, 1.000000000000000000, 0.8660254037844387076, 1.000000000000000000, 0.8660254037844387076, 1.000000000000000000, 0.8660254037844387076, 1.000000000000000000, 0.8660254037844387076, 1.000000000000000000, 0.8660254037844387076, 1.000000000000000000, 0.8660254037844387076, 1.000000000000000000, 0.8660254037844387076, 1.000000000000000000, 0.8660254037844387076, 1.000000000000000000, 0.8660254037844387076, 1.000000000000000000, 0.8660254037844387076, 1.000000000000000000, 0.8660254037844387076, 1.000000000000000000, 0.8660254037844387076, 1.000000000000000000, 0.8660254037844387076, 1.000000000000000000, 0.8660254037844387076, 1.000000000000000000, 0.8660254037844387076, 1.000000000000000000, 0.8660254037844387076, 1.000000000000000000, 0.8660254037844387076, 1.000000000000000000, 0.8660254037844387076, 1.000000000000000000, 0.8660254037844387076, 1.000000000000000000, 0.8660254037844387076, 1.000000000000000000, 0.8660254037844387076, 1.000000000000000000, 0.8660254037844387076, 1.000000000000000000, 0.8660254037844387076, 1.000000000000000000, 0.8660254037844387076, 1.000000000000000000, 0.8660254037844387076, 1.000000000000000000, 0.8660254037844387076, 1.000000000000000000, 0.8660254037844387076, 1.000000000000000000, 0.8660254037844387076, 1.000000000000000000, 0.8660254037844387076, 1.000000000000000000, 0.8660254037844387076, 1.000000000000000000, 0.8660254037844387076, 1.000000000000000000, 0.8660254037844387076, 1.000000000000000000, 0.8660254037844387076, 1.000000000000000000, 0.8660254037844387076, 1.000000000000000000, 0.8660254037844387076, 1.000000000000000000, 0.8660254037844387076, 1.000000000000000000, 0.8660254037844387076, 1.000000000000000000, 0.8660254037844387076, 1.000000000000000000, 0.8660254037844387076, 1.000000000000000000, 0.8660254037844387076, 1.000000000000000000, 0.8660254037844387076, 1.000000000000000000, 0.8660254037844387076, 1.000000000000000000, 0.8660254037844387076, 1.000000000000000000, 0.8660254037844387076, 1.000000000000000000, 0.8660254037844387076, 1.000000000000000000, 0.8660254037844387076, 1.000000000000000000, 0.8660254037844387076, 1.000000000000000000, 0.8660254037844387076, 1.000000000000000000, 0.8660254037844387076, 1.000000000000000000, 0.8660254037844387076, 1.000000000000000000, 0.8660254037844387076, 1.000000000000000000, 0.8660254037844387076, 1.000000000000000000, 0.8660254037844387076, 1.000000000000000000, 0.8660254037844387076, 1.000000000000000000, 0.8660254037844387076, 1.000000000000000000, 0.8660254037844387076, 1.000000000000000000, 0.8660254037844387076, 1.000000000000000000, 0.8660254037844387076, 1.000000000000000000, 0.8660254037844387076, 1.000000000000000000, 0.8660254037844387076, 1.000000000000000000, 0.8660254037844387076, 1.000000000000000000, 0.8660254037844387076, 1.000000000000000000, 0.8660254037844387076, 1.000000000000000000, 0.8660254037844387076, 1.000000000000000000, 0.8660254037844387076, 1.000000000000000000, 0.8660254037844387076, 1.000000000000000000, 0.8660254037844387076, 1.000000000000000000, 0.8660254037844387076, 1.000000000000000000, 0.8660254037844387076, 1.000000000000000000, 0.8660254037844387076, 1.000000000000000000, 0.8660254037844387076, 1.000000000000000000, 0.8660254037844387076, 1.000000000000000000, 0.8660254037844387076, 1.000000000000000000, 0.8660254037844387076, 1.000000000000000000, 0.8660254037844387076, 1.000000000000000000, 0.8660254037844387076, 1.000000000000000000, 0.8660254037844387076, 1.000000000000000000, 0.8660254037844387076, 1.000000000000000000, 0.8660254037844387076, 1.000000000000000000, 0.8660254037844387076, 1.000000000000000000, 0.8660254037844387076, 1.000000000000000000, 0.8660254037844387076, 1.000000000000000000, 0.8660254037844387076, 1.000000000000000000, 0.8660254037844387076, 1.000000000000000000, 0.8660254037844387076, 1.000000000000000000, 0.8660254037844387076, 1.000000000000000000, 0.8660254037844387076, 1.000000000000000000, 0.8660254037844387076, 1.000000000000000000, 0.8660254037844387076, 1.000000000000000000, 0.8660254037844387076, 1.000000000000000000, 0.8660254037844387076, 1.000000000000000000, 0.8660254037844387076, 1.000000000000000000, 0.8660254037844387076, 1.000000000000000000, 0.8660254037844387076, 1.000000000000000000, 0.8660254037844387076, 1.000000000000000000, 0.8660254037844387076, 1.000000000000000000, 0.8660254037844387076, 1.000000000000000000, 0.8660254037844387076, 1.000000000000000000, 0.8660254037844387076, 1.000000000000000000, 0.8660254037844387076, 1.000000000000000000, 0.8660254037844387076, 1.000000000000000000, 0.8660254037844387076, 1.000000000000000000, 0.8660254037844387076, 1.000000000000000000, 0.8660254037844387076, 1.000000000000000000, 0.8660254037844387076, 1.000000000000000000, 0.8660254037844387076, 1.000000000000000000, 0.8660254037844387076, 1.000000000000000000, 0.8660254037844387076, 1.000000000000000000, 0.8660254037844387076, 1.000000000000000000, 0.8660254037844387076, 1.000000000000000000, 0.8660254037844387076, 1.000000000000000000, 0.8660254037844387076, 1.000000000000000000, 0.8660254037844387076, 1.000000000000000000, 0.8660254037844387076, 1.000000000000000000, 0.8660254037844387076, 1.000000000000000000, 0.8660254037844387076, 1.000000000000000000, 0.8660254037844387076, 1.000000000000000000, 0.8660254037844387076, 1.000000000000000000, 0.8660254037844387076, 1.000000000000000000, 0.8660254037844387076, 1.000000000000000000, 0.8660254037844387076, 1.000000000000000000, 0.8660254037844387076, 1.000000000000000000, 0.8660254037844387076, 1.000000000000000000, 0.8660254037844387076, 1.000000000000000000, 0.8660254037844387076, 1.000000000000000000, 0.8660254037844387076, 1.000000000000000000, 0.8660254037844387076, 1.000000000000000000, 0.8660254037844387076, 1.000000000000000000, 0.8660254037844387076, 1.000000000000000000, 0.8660254037844387076, 1.000000000000000000, 0.8660254037844387076, 1.000000000000000000, 0.8660254037844387076, 1.000000000000000000, 0.8660254037844387076, 1.000000000000000000, 0.8660254037844387076, 1.000000000000000000, 0.8660254037844387076, 1.000000000000000000, 0.8660254037844387076, 1.000000000000000000, 0.8660254037844387076, 1.000000000000000000, 0.8660254037844387076, 1.000000000000000000, 0.8660254037844387076, 1.000000000000000000, 0.8660254037844387076, 1.000000000000000000, 0.8660254037844387076, 1.000000000000000000, 0.8660254037844387076, 1.000000000000000000, 0.8660254037844387076, 1.000000000000000000, 0.8660254037844387076, 1.000000000000000000, 0.8660254037844387076, 1.000000000000000000, 0.8660254037844387076, 1.000000000000000000, 0.8660254037844387076, 1.000000000000000000, 0.8660254037844387076, 1.000000000000000000, 0.8660254037844387076, 1.000000000000000000, 0.8660254037844387076, 1.000000000000000000, 0.8660254037844387076, 1.000000000000000000, 0.8660254037844387076, 1.000000000000000000, 0.8660254037844387076, 1.000000000000000000, 0.8660254037844387076, 1.000000000000000000, 0.8660254037844387076, 1.000000000000000000, 0.8660254037844387076, 1.000000000000000000, 0.8660254037844387076, 1.000000000000000000, 0.8660254037844387076, 1.000000000000000000, 0.8660254037844387076, 1.000000000000000000, 0.8660254037844387076, 1.000000000000000000, 0.8660254037844387076, 1.000000000000000000, 0.8660254037844387076, 1.000000000000000000, 0.8660254037844387076, 1.000000000000000000, 0.8660254037844387076, 1.000000000000000000, 0.8660254037844387076, 1.000000000000000000, 0.8660254037844387076, 1.000000000000000000, 0.8660254037844387076, 1.000000000000000000, 0.8660254037844387076, 1.000000000000000000, 0.8660254037844387076, 1.000000000000000000, 0.8660254037844387076, 1.000000000000000000, 0.8660254037844387076, 1.000000000000000000, 0.8660254037844387076, 1.000000000000000000, 0.8660254037844387076, 1.000000000000000000, 0.8660254037844387076, 1.000000000000000000, 0.8660254037844387076, 1.000000000000000000, 0.8660254037844387076, 1.000000000000000000, 0.8660254037844387076, 1.000000000000000000, 0.8660254037844387076, 1.000000000000000000, 0.8660254037844387076, 1.000000000000000000, 0.8660254037844387076, 1.000000000000000000, 0.8660254037844387076, 1.000000000000000000, 0.8660254037844387076, 1.000000000000000000, 0.8660254037844387076, 1.000000000000000000, 0.8660254037844387076, 1.000000000000000000, 0.8660254037844387076, 1.000000000000000000, 0.8660254037844387076, 1.000000000000000000, 0.8660254037844387076, 1.000000000000000000, 0.8660254037844387076, 1.000000000000000000, 0.8660254037844387076, 1.000000000000000000, 0.8660254037844387076, 1.000000000000000000, 0.8660254037844387076, 1.000000000000000000, 0.8660254037844387076, 1.000000000000000000, 0.8660254037844387076, 1.000000000000000000, 0.8660254037844387076, 1.000000000000000000, 0.8660254037844387076, 1.000000000000000000, 0.8660254037844387076, 1.000000000000000000, 0.8660254037844387076, 1.000000000000000000, 0.8660254037844387076, 1.000000000000000000, 0.8660254037844387076, 1.000000000000000000, 0.8660254037844387076, 1.000000000000000000, 0.8660254037844387076, 1.000000000000000000, 0.8660254037844387076, 1.000000000000000000, 0.8660254037844387076, 1.000000000000000000, 0.8660254037844387076, 1.000000000000000000, 0.8660254037844387076, 1.000000000000000000, 0.8660254037844387076, 1.000000000000000000, 0.8660254037844387076, 1.000000000000000000, 0.8660254037844387076, 1.000000000000000000, 0.8660254037844387076, 1.000000000000000000, 0.8660254037844387076, 1.000000000000000000, 0.8660254037844387076, 1.000000000000000000, 0.8660254037844387076, 1.000000000000000000, 0.8660254037844387076, 1.000000000000000000, 0.8660254037844387076, 1.000000000000000000, 0.8660254037844387076, 1.000000000000000000, 0.8660254037844387076, 1.000000000000000000, 0.8660254037844387076, 1.000000000000000000, 0.8660254037844387076, 1.000000000000000000, 0.8660254037844387076, 1.000000000000000000, 0.8660254037844387076, 1.000000000000000000, 0.8660254037844387076, 1.000000000000000000, 0.8660254037844387076, 1.000000000000000000, 0.8660254037844387076, 1.000000000000000000, 0.8660254037844387076, 1.000000000000000000, 0.8660254037844387076, 1.000000000000000000, 0.8660254037844387076, 1.000000000000000000, 0.8660254037844387076, 1.000000000000000000, 0.8660254037844387076, 1.000000000000000000, 0.8660254037844387076, 1.000000000000000000, 0.8660254037844387076, 1.000000000000000000, 0.8660254037844387076, 1.000000000000000000, 0.8660254037844387076, 1.000000000000000000, 0.8660254037844387076, 1.000000000000000000, 0.8660254037844387076, 1.000000000000000000, 0.8660254037844387076, 1.000000000000000000, 0.8660254037844387076, 1.000000000000000000, 0.8660254037844387076, 1.000000000000000000, 0.8660254037844387076, 1.000000000000000000, 0.8660254037844387076, 1.000000000000000000, 0.8660254037844387076, 1.000000000000000000, 0.8660254037844387076, 1.000000000000000000, 0.8660254037844387076, 1.000000000000000000, 0.8660254037844387076, 1.000000000000000000, 0.8660254037844387076, 1.000000000000000000, 0.8660254037844387076, 1.000000000000000000, 0.8660254037844387076, 1.000000000000000000, 0.8660254037844387076, 1.000000000000000000, 0.8660254037844387076, 1.000000000000000000, 0.8660254037844387076, 1.000000000000000000, 0.8660254037844387076, 1.000000000000000000, 0.8660254037844387076, 1.000000000000000000, 0.8660254037844387076, 1.000000000000000000, 0.8660254037844387076, 1.000000000000000000, 0.8660254037844387076, 1.000000000000000000, 0.8660254037844387076, 1.000000000000000000, 0.8660254037844387076, 1.000000000000000000, 0.8660254037844387076, 1.000000000000000000, 0.8660254037844387076, 1.000000000000000000, 0.8660254037844387076, 1.000000000000000000, 0.8660254037844387076, 1.000000000000000000, 0.8660254037844387076, 1.000000000000000000, 0.8660254037844387076, 1.000000000000000000, 0.8660254037844387076, 1.000000000000000000, 0.8660254037844387076, 1.000000000000000000, 0.8660254037844387076, 1.000000000000000000, 0.8660254037844387076, 1.000000000000000000, 0.8660254037844387076, 1.000000000000000000, 0.8660254037844387076, 1.000000000000000000, 0.8660254037844387076, 1.000000000000000000, 0.8660254037844387076, 1.000000000000000000, 0.8660254037844387076, 1.000000000000000000, 0.8660254037844387076, 1.000000000000000000, 0.8660254037844387076, 1.000000000000000000, 0.8660254037844387076, 1.000000000000000000, 0.8660254037844387076, 1.000000000000000000, 0.8660254037844387076, 1.000000000000000000, 0.8660254037844387076, 1.000000000000000000, 0.8660254037844387076, 1.000000000000000000, 0.8660254037844387076, 1.000000000000000000, 0.8660254037844387076, 1.000000000000000000, 0.8660254037844387076, 1.000000000000000000, 0.8660254037844387076, 1.000000000000000000, 0.8660254037844387076, 1.000000000000000000, 0.8660254037844387076, 1.000000000000000000, 0.8660254037844387076, 1.000000000000000000, 0.8660254037844387076, 1.000000000000000000, 0.8660254037844387076, 1.000000000000000000, 0.8660254037844387076, 1.000000000000000000 ) ) 
 REPRESENTATION_ITEM ( '' )  );
#25726=CARTESIAN_POINT ( 'NONE',  ( 0.000000000000000000, 0.000000000000000000, 0.000000000000000000 ) ) ;
#25730=CARTESIAN_POINT ( 'NONE',  ( 6.000000000000000888, -1.859271017917181981E-14, -173.1636751345948539 ) ) ;
#25731=CARTESIAN_POINT ( 'NONE',  ( -5.999999999999963585, -1.487416814333745711E-14, -132.8363248654052597 ) ) ;
#25733=FACE_OUTER_BOUND ( 'NONE', #21637, .T. ) ;
#25738=LINE ( 'NONE', #18549, #7260 ) ;
#25739=EDGE_LOOP ( 'NONE', ( #20280, #27004, #27369, #3121 ) ) ;
#25740=VERTEX_POINT ( 'NONE', #29046 ) ;
#25742=CARTESIAN_POINT ( 'NONE',  ( 6.350852961086080661, -9.614813431917819062E-14, -88.87500000000000000 ) ) ;
#25743=CARTESIAN_POINT ( 'NONE',  ( 5.412658773652739619, 3.124999999999988898, -108.6830127018922383 ) ) ;
#25744=VERTEX_POINT ( 'NONE', #17723 ) ;
#25745=CARTESIAN_POINT ( 'NONE',  ( 1.971541444415901845, 10.82814027403869694, -30.68027829220103442 ) ) ;
#25747=ADVANCED_FACE ( 'NONE', ( #941 ), #26591, .T. ) ;
#25748=CARTESIAN_POINT ( 'NONE',  ( 4.763139720814407951, 2.750000000000002665, -166.7500000000000000 ) ) ;
#25749=CARTESIAN_POINT ( 'NONE',  ( -5.196152422706573404, -3.000000000000002665, -106.2886751345948397 ) ) ;
#25750=CARTESIAN_POINT ( 'NONE',  ( 3.464101615137852974, 5.999999999999884537, -46.91367513459483263 ) ) ;
#25751=FILL_AREA_STYLE ('',( #23471 ) ) ;
#25752=CARTESIAN_POINT ( 'NONE',  ( 3.175426480543072749, 5.499999999999865885, -172.6250000000000284 ) ) ;
#25754=CARTESIAN_POINT ( 'NONE',  ( 4.763139720814407951, 2.750000000000002665, -157.7500000000000568 ) ) ;
#25757=CARTESIAN_POINT ( 'NONE',  ( 0.000000000000000000, 5.499999999999991118, -99.00000000000002842 ) ) ;
#25758=CARTESIAN_POINT ( 'NONE',  ( -5.999999999999963585, 3.021315404115421074E-15, -177.8363248654052029 ) ) ;
#25760=CARTESIAN_POINT ( 'NONE',  ( -2.775557561562891351E-14, -5.500000000000115463, -90.75000000000000000 ) ) ;
#25761=EDGE_CURVE ( 'NONE', #3256, #20541, #16487, .T. ) ;
#25773=VERTEX_POINT ( 'NONE', #15432 ) ;
#25782=CARTESIAN_POINT ( 'NONE',  ( 3.175426480543072749, 5.499999999999865885, -111.1249999999999716 ) ) ;
#25784=CARTESIAN_POINT ( 'NONE',  ( 5.412658773652739619, 3.124999999999988898, -132.6830127018922667 ) ) ;
#25785=EDGE_LOOP ( 'NONE', ( #8871, #27554, #20837, #7525 ) ) ;
#25786=CARTESIAN_POINT ( 'NONE',  ( -5.999999999999963585, 1.780251999655701777E-13, -47.33632486540523132 ) ) ;
#25787=CARTESIAN_POINT ( 'NONE',  ( -5.412658773652739619, 3.124999999999975131, -171.8169872981077901 ) ) ;
#25790=EDGE_CURVE ( 'NONE', #27478, #14802, #12347, .T. ) ;
#25791=ORIENTED_EDGE ( 'NONE', *, *, #6195, .F. ) ;
#25792=CARTESIAN_POINT ( 'NONE',  ( -6.000000000000000888, 1.067854986875958443E-15, 7.560779664488942560E-35 ) ) ;
#25793=CARTESIAN_POINT ( 'NONE',  ( 6.000000000000000888, 7.762456499804234384E-14, -133.5863248654052029 ) ) ;
#25794=CARTESIAN_POINT ( 'NONE',  ( 3.175426480543072749, 5.499999999999865885, -178.6250000000000284 ) ) ;
#25796=CARTESIAN_POINT ( 'NONE',  ( 7.216878364870455975, -6.409875621278545621E-14, -176.3080127018922667 ) ) ;
#25798=CARTESIAN_POINT ( 'NONE',  ( 6.000000000000000888, -1.859271017917181981E-14, -105.0863248654052313 ) ) ;
#25799=CARTESIAN_POINT ( 'NONE',  ( 6.000000000000000888, 7.762456499804234384E-14, -123.6636751345948255 ) ) ;
#25800=EDGE_CURVE ( 'NONE', #29296, #26144, #7015, .T. ) ;
#25801=CARTESIAN_POINT ( 'NONE',  ( -3.175426480542816510, -5.500000000000057732, -119.3750000000000284 ) ) ;
#25802=ORIENTED_EDGE ( 'NONE', *, *, #21028, .T. ) ;
#25804=AXIS2_PLACEMENT_3D ( 'NONE', #15755, #27212, #15600 ) ;
#25810=CARTESIAN_POINT ( 'NONE',  ( -5.999999999999963585, 8.134310703387671600E-14, -121.4136751345948255 ) ) ;
#25812=CARTESIAN_POINT ( 'NONE',  ( 6.000000000000000888, 1.743066579297358182E-13, -108.6636751345948255 ) ) ;
#25813=ORIENTED_EDGE ( 'NONE', *, *, #9633, .F. ) ;
#25814=CARTESIAN_POINT ( 'NONE',  ( 0.000000000000000000, -5.999999999999991118, -77.53867513459483973 ) ) ;
#25815=( BOUNDED_CURVE ( )  B_SPLINE_CURVE ( 2, ( #17962, #10575, #6392, #5934, #17496, #3928, #4090, #12903, #1024 ),
 .UNSPECIFIED., .F., .T. ) 
 B_SPLINE_CURVE_WITH_KNOTS ( ( 3, 2, 2, 2, 3 ),
 ( 0.1138888888888888173, 0.1148148148148148140, 0.1166666666666666963, 0.1185185185185184675, 0.1194444444444444642 ),
 .UNSPECIFIED. ) 
 CURVE ( )  GEOMETRIC_REPRESENTATION_ITEM ( )  RATIONAL_B_SPLINE_CURVE ( ( 0.9330127018922194093, 0.9330127018922154125, 1.000000000000000000, 0.8660254037844388186, 1.000000000000000000, 0.8660254037844388186, 1.000000000000000000, 0.9330127018922154125, 0.9330127018922194093 ) ) 
 REPRESENTATION_ITEM ( '' )  );
#25816=DIRECTION ( 'NONE',  ( -7.147005652999508048E-36, 5.642372883946980038E-36, 1.000000000000000000 ) ) ;
#25818=CARTESIAN_POINT ( 'NONE',  ( 3.464101615137757051, -5.999999999999979572, -141.9136751345948255 ) ) ;
#25822=CARTESIAN_POINT ( 'NONE',  ( 5.412658773652712085, -3.125000000000086153, -141.0669872981078470 ) ) ;
#25826=ADVANCED_FACE ( 'NONE', ( #1100 ), #17271, .T. ) ;
#25827=CARTESIAN_POINT ( 'NONE',  ( 5.196152422706629359, -2.999999999999988898, -129.7886751345947971 ) ) ;
#25834=FACE_BOUND ( 'NONE', #5454, .T. ) ;
#25838=CARTESIAN_POINT ( 'NONE',  ( 5.196152422706629359, 3.000000000000002665, -149.0386751345948539 ) ) ;
#25841=CARTESIAN_POINT ( 'NONE',  ( 3.175426480543072749, 5.499999999999865885, -52.62500000000002842 ) ) ;
#25846=CARTESIAN_POINT ( 'NONE',  ( 3.608439182435180470, 6.249999999999982236, -103.1919872981078328 ) ) ;
#25847=CARTESIAN_POINT ( 'NONE',  ( -6.000000000000000888, 1.067854986875958443E-15, 7.560779664488942560E-35 ) ) ;
#25852=CARTESIAN_POINT ( 'NONE',  ( 4.763139720814407951, 2.750000000000002665, -141.2500000000000000 ) ) ;
#25854=VERTEX_POINT ( 'NONE', #22003 ) ;
#25855=CARTESIAN_POINT ( 'NONE',  ( -5.999999999999919176, 1.607695154586804565, -162.9033121635129646 ) ) ;
#25856=CARTESIAN_POINT ( 'NONE',  ( -3.175426480542816510, 5.499999999999865885, -65.87500000000002842 ) ) ;
#25857=( BOUNDED_CURVE ( )  B_SPLINE_CURVE ( 2, ( #1287, #18073, #24797, #6211, #3744, #3890, #13321, #13178, #22662 ),
 .UNSPECIFIED., .F., .F. ) 
 B_SPLINE_CURVE_WITH_KNOTS ( ( 3, 2, 2, 2, 3 ),
 ( 0.1361111111111110716, 0.1370370370370370683, 0.1388888888888888395, 0.1407407407407407218, 0.1416666666666667185 ),
 .UNSPECIFIED. ) 
 CURVE ( )  GEOMETRIC_REPRESENTATION_ITEM ( )  RATIONAL_B_SPLINE_CURVE ( ( 0.9330127018922194093, 0.9330127018922154125, 1.000000000000000000, 0.8660254037844388186, 1.000000000000000000, 0.8660254037844388186, 1.000000000000000000, 0.9330127018922154125, 0.9330127018922194093 ) ) 
 REPRESENTATION_ITEM ( '' )  );
#25859=DIRECTION ( 'NONE',  ( -7.147005652999508048E-36, 5.642372883946980038E-36, 1.000000000000000000 ) ) ;
#25860=CARTESIAN_POINT ( 'NONE',  ( -3.464101615137725076, 5.999999999999979572, -66.16367513459479710 ) ) ;
#25861=EDGE_CURVE ( 'NONE', #152, #12734, #5828, .T. ) ;
#25862=CARTESIAN_POINT ( 'NONE',  ( 2.775557561562891351E-14, -6.250000000000061284, -82.18301270189220986 ) ) ;
#25863=CARTESIAN_POINT ( 'NONE',  ( -3.464101615137757051, -5.999999999999979572, -113.6636751345948113 ) ) ;
#25867=CARTESIAN_POINT ( 'NONE',  ( 3.175426480543072749, -5.500000000000105693, -150.6250000000000284 ) ) ;
#25869=CARTESIAN_POINT ( 'NONE',  ( -3.608439182435052128, -6.250000000000110134, -164.8080127018922667 ) ) ;
#25870=CARTESIAN_POINT ( 'NONE',  ( -5.196152422706573404, -3.000000000000002665, -149.2113248654052313 ) ) ;
#25872=CARTESIAN_POINT ( 'NONE',  ( 4.763139720814407951, -2.749999999999988454, -78.50000000000001421 ) ) ;
#25873=CARTESIAN_POINT ( 'NONE',  ( 4.763139720814407951, 2.750000000000002665, -69.25000000000002842 ) ) ;
#25880=CARTESIAN_POINT ( 'NONE',  ( 0.000000000000000000, 0.000000000000000000, -200.0000000000000000 ) ) ;
#25886=CARTESIAN_POINT ( 'NONE',  ( 5.412658773652739619, 3.124999999999988898, -155.8169872981078470 ) ) ;
#25887=EDGE_LOOP ( 'NONE', ( #12649, #25141, #1321, #19540 ) ) ;
#25888=CARTESIAN_POINT ( 'NONE',  ( -6.350852961085760029, -1.281975124255709124E-13, -89.62500000000000000 ) ) ;
#25891=( BOUNDED_CURVE ( )  B_SPLINE_CURVE ( 2, ( #27182, #22139, #8772, #3984, #8458, #5993, #27333, #18159, #27474 ),
 .UNSPECIFIED., .F., .F. ) 
 B_SPLINE_CURVE_WITH_KNOTS ( ( 3, 2, 2, 2, 3 ),
 ( 0.1750000000000000167, 0.1759259259259259300, 0.1777777777777777846, 0.1796296296296296391, 0.1805555555555555525 ),
 .UNSPECIFIED. ) 
 CURVE ( )  GEOMETRIC_REPRESENTATION_ITEM ( )  RATIONAL_B_SPLINE_CURVE ( ( 0.9330127018922194093, 0.9330127018922204085, 1.000000000000000000, 0.8660254037844388186, 1.000000000000000000, 0.8660254037844388186, 1.000000000000000000, 0.9330127018922205195, 0.9330127018922196314 ) ) 
 REPRESENTATION_ITEM ( '' )  );
#25893=ORIENTED_EDGE ( 'NONE', *, *, #2889, .F. ) ;
#25895=CARTESIAN_POINT ( 'NONE',  ( 7.216878364870455975, -6.409875621278545621E-14, -47.30801270189223118 ) ) ;
#25896=( BOUNDED_CURVE ( )  B_SPLINE_CURVE ( 2, ( #28714, #14782, #24126, #12498, #14037, #9227, #2010, #11254, #18322 ),
 .UNSPECIFIED., .F., .F. ) 
 B_SPLINE_CURVE_WITH_KNOTS ( ( 3, 2, 2, 2, 3 ),
 ( 0.4916666666666666408, 0.4925925925925925819, 0.4944444444444444642, 0.4962962962962962910, 0.4972222222222222321 ),
 .UNSPECIFIED. ) 
 CURVE ( )  GEOMETRIC_REPRESENTATION_ITEM ( )  RATIONAL_B_SPLINE_CURVE ( ( 0.9330127018922194093, 0.9330127018922174109, 1.000000000000000000, 0.8660254037844388186, 1.000000000000000000, 0.8660254037844388186, 1.000000000000000000, 0.9330127018922194093, 0.9330127018922194093 ) ) 
 REPRESENTATION_ITEM ( '' )  );
#25897=CARTESIAN_POINT ( 'NONE',  ( -3.175426480542816066, 5.499999999999865885, -172.3750000000000568 ) ) ;
#25900=CARTESIAN_POINT ( 'NONE',  ( 6.350852961086080661, -9.614813431917819062E-14, -157.8750000000000000 ) ) ;
#25902=CARTESIAN_POINT ( 'NONE',  ( -4.763139720814407951, -2.750000000000016431, -103.0000000000000426 ) ) ;
#25906=CARTESIAN_POINT ( 'NONE',  ( -4.763139720814407951, 2.749999999999946709, -157.2500000000000000 ) ) ;
#25907=CARTESIAN_POINT ( 'NONE',  ( 3.175426480543072749, -5.500000000000105693, -90.62500000000001421 ) ) ;
#25914=CARTESIAN_POINT ( 'NONE',  ( 0.000000000000000000, 5.499999999999991118, -46.49999999999998579 ) ) ;
#25916=CARTESIAN_POINT ( 'NONE',  ( 6.000000000000000888, -3.330669073875464691E-16, -7.560779664488942560E-35 ) ) ;
#25923=ORIENTED_EDGE ( 'NONE', *, *, #17599, .T. ) ;
#25925=CARTESIAN_POINT ( 'NONE',  ( 3.175426480543072749, 5.499999999999865885, -117.1250000000000142 ) ) ;
#25928=CARTESIAN_POINT ( 'NONE',  ( -7.216878364870328078, 0.000000000000000000, -130.5580127018922383 ) ) ;
#25929=ORIENTED_EDGE ( 'NONE', *, *, #5311, .F. ) ;
#25931=CARTESIAN_POINT ( 'NONE',  ( 2.775557561562891351E-14, -6.250000000000061284, -168.3169872981078470 ) ) ;
#25934=EDGE_LOOP ( 'NONE', ( #113, #8924, #2862, #23077 ) ) ;
#25935=CARTESIAN_POINT ( 'NONE',  ( 3.464101615137852974, 5.999999999999884537, -95.83632486540517448 ) ) ;
#25937=FACE_OUTER_BOUND ( 'NONE', #14628, .T. ) ;
#25939=CARTESIAN_POINT ( 'NONE',  ( -3.608439182435115633, 6.249999999999965361, -180.3080127018922667 ) ) ;
#25944=CARTESIAN_POINT ( 'NONE',  ( -6.350852961085760029, -1.281975124255709124E-13, -110.6249999999999858 ) ) ;
#25954=ADVANCED_FACE ( 'NONE', ( #13282 ), #23240, .T. ) ;
#25957=VERTEX_POINT ( 'NONE', #29663 ) ;
#25959=CARTESIAN_POINT ( 'NONE',  ( -6.000000000000000888, 1.067854986875958443E-15, 7.560779664488942560E-35 ) ) ;
#25962=CARTESIAN_POINT ( 'NONE',  ( 5.196152422706629359, -2.999999999999988898, -141.7886751345947971 ) ) ;
#25965=EDGE_CURVE ( 'NONE', #12143, #20807, #14494, .T. ) ;
#25967=CARTESIAN_POINT ( 'NONE',  ( 5.412658773652739619, 3.124999999999988898, -142.3169872981078186 ) ) ;
#25969=EDGE_CURVE ( 'NONE', #7855, #8435, #25973, .T. ) ;
#25970=DIRECTION ( 'NONE',  ( 1.000000000000000000, -5.551115123125773458E-17, -1.260129944081490338E-35 ) ) ;
#25973=LINE ( 'NONE', #9707, #22572 ) ;
#25974=DIRECTION ( 'NONE',  ( 7.147005652999508048E-36, -5.642372883946980038E-36, -1.000000000000000000 ) ) ;
#25977=CARTESIAN_POINT ( 'NONE',  ( 6.000000000000000888, 1.743066579297358182E-13, -99.66367513459479710 ) ) ;
#25978=CARTESIAN_POINT ( 'NONE',  ( 5.196152422706629359, -2.999999999999988898, -160.7113248654052313 ) ) ;
#25980=CARTESIAN_POINT ( 'NONE',  ( 0.000000000000000000, -5.999999999999991118, -69.46132486540523132 ) ) ;
#25982=CARTESIAN_POINT ( 'NONE',  ( 6.000000000000103917, -1.607695154586573416, -142.6533121635129646 ) ) ;
#25984=CARTESIAN_POINT ( 'NONE',  ( 0.000000000000000000, 5.999999999999977796, -112.7886751345948397 ) ) ;
#25986=CARTESIAN_POINT ( 'NONE',  ( 3.464101615137757051, -5.999999999999979572, -106.8363248654052313 ) ) ;
#25987=CARTESIAN_POINT ( 'NONE',  ( 3.464101615137852974, 5.999999999999884537, -52.91367513459480421 ) ) ;
#25988=( BOUNDED_CURVE ( )  B_SPLINE_CURVE ( 2, ( #5470, #8397, #17803, #15505, #12898, #14878, #1018, #27121, #6093 ),
 .UNSPECIFIED., .F., .T. ) 
 B_SPLINE_CURVE_WITH_KNOTS ( ( 3, 2, 2, 2, 3 ),
 ( 0.8750000000000000000, 0.8759259259259258856, 0.8777777777777777679, 0.8796296296296296502, 0.8805555555555555358 ),
 .UNSPECIFIED. ) 
 CURVE ( )  GEOMETRIC_REPRESENTATION_ITEM ( )  RATIONAL_B_SPLINE_CURVE ( ( 0.9330127018922194093, 0.9330127018922194093, 1.000000000000000000, 0.8660254037844388186, 1.000000000000000000, 0.8660254037844388186, 1.000000000000000000, 0.9330127018922234061, 0.9330127018922194093 ) ) 
 REPRESENTATION_ITEM ( '' )  );
#25989=CARTESIAN_POINT ( 'NONE',  ( -5.999999999999963585, -1.487416814333745711E-14, -170.9136751345948255 ) ) ;
#25997=CARTESIAN_POINT ( 'NONE',  ( 3.175426480543072749, -5.500000000000105693, -128.1249999999999716 ) ) ;
#26001=CARTESIAN_POINT ( 'NONE',  ( 6.350852961086080661, -9.614813431917819062E-14, -67.87500000000002842 ) ) ;
#26002=CARTESIAN_POINT ( 'NONE',  ( 6.000000000000001776, 5.345404176511898156E-15, -179.1636751345948255 ) ) ;
#26004=CARTESIAN_POINT ( 'NONE',  ( -5.412658773652684552, -3.125000000000099920, -79.43301270189223828 ) ) ;
#26010=CARTESIAN_POINT ( 'NONE',  ( -6.350852961085760029, -1.281975124255709124E-13, -139.1250000000000000 ) ) ;
#26012=CARTESIAN_POINT ( 'NONE',  ( 7.216878364870455975, -6.409875621278545621E-14, -152.3080127018922099 ) ) ;
#26013=SURFACE_STYLE_USAGE ( .BOTH. , #28310 ) ;
#26015=CARTESIAN_POINT ( 'NONE',  ( 0.000000000000000000, 5.499999999999991118, -78.00000000000001421 ) ) ;
#26017=CARTESIAN_POINT ( 'NONE',  ( 6.350852961086080661, -9.614813431917819062E-14, -67.87500000000002842 ) ) ;
#26022=PLANE ( 'NONE',  #20214 ) ;
#26025=EDGE_CURVE ( 'NONE', #27786, #20871, #15299, .T. ) ;
#26027=CARTESIAN_POINT ( 'NONE',  ( 3.464101615137757051, -5.999999999999979572, -144.9136751345948255 ) ) ;
#26033=ADVANCED_FACE ( 'NONE', ( #5065 ), #23686, .T. ) ;
#26037=CARTESIAN_POINT ( 'NONE',  ( 3.608439182435180470, -6.249999999999997335, -154.6919872981078470 ) ) ;
#26038=ORIENTED_EDGE ( 'NONE', *, *, #24941, .F. ) ;
#26039=CARTESIAN_POINT ( 'NONE',  ( 0.000000000000000000, 5.499999999999991118, -91.50000000000002842 ) ) ;
#26041=CARTESIAN_POINT ( 'NONE',  ( 5.412658773652739619, 3.124999999999988898, -99.68301270189222407 ) ) ;
#26042=VERTEX_POINT ( 'NONE', #26266 ) ;
#26043=VECTOR ( 'NONE', #16435, 1000.000000000000000 ) ;
#26047=CARTESIAN_POINT ( 'NONE',  ( 4.380587382795412488, -10.09118633559234190, -20.89546095134608805 ) ) ;
#26048=CARTESIAN_POINT ( 'NONE',  ( -3.464101615137725076, 5.999999999999979572, -93.16367513459479710 ) ) ;
#26049=( NAMED_UNIT ( * ) PLANE_ANGLE_UNIT ( ) SI_UNIT ( $, .RADIAN. ) );
#26050=CARTESIAN_POINT ( 'NONE',  ( -3.175426480542816066, 5.499999999999865885, -175.3750000000000568 ) ) ;
#26051=CARTESIAN_POINT ( 'NONE',  ( -5.999999999999963585, 1.780251999655701777E-13, -57.83632486540521711 ) ) ;
#26052=CARTESIAN_POINT ( 'NONE',  ( 4.763139720814407951, -2.749999999999988454, -156.5000000000000284 ) ) ;
#26054=CARTESIAN_POINT ( 'NONE',  ( 3.175426480543072749, 5.499999999999865885, -102.1250000000000142 ) ) ;
#26056=CARTESIAN_POINT ( 'NONE',  ( -3.175426480542816510, -5.500000000000057732, -86.37500000000005684 ) ) ;
#26065=EDGE_CURVE ( 'NONE', #14802, #11050, #18633, .T. ) ;
#26067=DIRECTION ( 'NONE',  ( 1.000000000000000000, -5.551115123125773458E-17, -1.260129944081490338E-35 ) ) ;
#26069=VECTOR ( 'NONE', #4896, 1000.000000000000000 ) ;
#26071=ORIENTED_EDGE ( 'NONE', *, *, #26369, .T. ) ;
#26075=CARTESIAN_POINT ( 'NONE',  ( 3.175426480543072749, -5.500000000000105693, -113.1250000000000000 ) ) ;
#26077=CARTESIAN_POINT ( 'NONE',  ( 5.412658773652712085, -3.125000000000086153, -120.9330127018922667 ) ) ;
#26079=FACE_OUTER_BOUND ( 'NONE', #26366, .T. ) ;
#26080=CARTESIAN_POINT ( 'NONE',  ( 2.775557561562891351E-14, -6.250000000000061284, -159.3169872981078470 ) ) ;
#26086=CARTESIAN_POINT ( 'NONE',  ( -3.027755249632137158, 10.58056329815972241, -19.80527582512399931 ) ) ;
#26087=CARTESIAN_POINT ( 'NONE',  ( -5.999999999999963585, -1.487416814333745711E-14, -137.3363248654052313 ) ) ;
#26088=CARTESIAN_POINT ( 'NONE',  ( -3.175426480542816510, -5.500000000000057732, -180.8750000000000000 ) ) ;
#26091=CARTESIAN_POINT ( 'NONE',  ( 5.412658773652739619, 3.124999999999988898, -177.6830127018922383 ) ) ;
#26092=CARTESIAN_POINT ( 'NONE',  ( -3.464101615137725076, 5.999999999999979572, -76.08632486540520290 ) ) ;
#26094=CARTESIAN_POINT ( 'NONE',  ( -4.763139720814407951, -2.750000000000016431, -125.5000000000000568 ) ) ;
#26095=CARTESIAN_POINT ( 'NONE',  ( 6.000000000000000888, 1.607695154586715303, -159.5966878364870922 ) ) ;
#26096=CARTESIAN_POINT ( 'NONE',  ( 0.000000000000000000, 5.499999999999991118, -112.5000000000000426 ) ) ;
#26097=ORIENTED_EDGE ( 'NONE', *, *, #24781, .T. ) ;
#26099=LINE ( 'NONE', #7368, #25591 ) ;
#26100=CARTESIAN_POINT ( 'NONE',  ( 6.000000000000000888, -1.859271017917181981E-14, -136.5863248654051745 ) ) ;
#26101=CYLINDRICAL_SURFACE ( 'NONE', #5954, 6.000000000000000888 ) ;
#26102=EDGE_CURVE ( 'NONE', #18315, #21672, #8824, .T. ) ;
#26104=CARTESIAN_POINT ( 'NONE',  ( 6.000000000000000888, -1.607695154586752384, -126.1533121635130072 ) ) ;
#26105=CARTESIAN_POINT ( 'NONE',  ( -4.763139720814407951, 2.749999999999946709, -176.7500000000000284 ) ) ;
#26113=CARTESIAN_POINT ( 'NONE',  ( -7.216878364870328078, 0.000000000000000000, -137.1919872981078186 ) ) ;
#26114=CARTESIAN_POINT ( 'NONE',  ( -6.000000000000000888, 1.067854986875958443E-15, 7.560779664488942560E-35 ) ) ;
#26117=VERTEX_POINT ( 'NONE', #10155 ) ;
#26119=CARTESIAN_POINT ( 'NONE',  ( 0.000000000000000000, 0.000000000000000000, 0.000000000000000000 ) ) ;
#26120=CARTESIAN_POINT ( 'NONE',  ( -5.999999999999963585, -1.487416814333745711E-14, -92.33632486540518869 ) ) ;
#26126=EDGE_CURVE ( 'NONE', #16271, #29296, #15108, .T. ) ;
#26131=CARTESIAN_POINT ( 'NONE',  ( 6.000000000000000888, 1.743066579297358182E-13, -106.5863248654052313 ) ) ;
#26132=CARTESIAN_POINT ( 'NONE',  ( -5.999999999999963585, 1.780251999655701777E-13, -52.41367513459481842 ) ) ;
#26137=LINE ( 'NONE', #5234, #21328 ) ;
#26138=CARTESIAN_POINT ( 'NONE',  ( -7.216878364870328078, 0.000000000000000000, -101.1919872981078328 ) ) ;
#26139=CARTESIAN_POINT ( 'NONE',  ( -3.464101615137725076, 5.999999999999979572, -172.6636751345947687 ) ) ;
#26142=CARTESIAN_POINT ( 'NONE',  ( -4.763139720814407951, -2.750000000000016431, -133.0000000000000000 ) ) ;
#26144=VERTEX_POINT ( 'NONE', #24257 ) ;
#26145=CARTESIAN_POINT ( 'NONE',  ( -4.763139720814407951, -2.750000000000016431, -55.00000000000004974 ) ) ;
#26146=CARTESIAN_POINT ( 'NONE',  ( 6.000000000000000888, 1.743066579297358182E-13, -81.08632486540518869 ) ) ;
#26149=CARTESIAN_POINT ( 'NONE',  ( 5.412658773652712085, -3.125000000000086153, -83.43301270189223828 ) ) ;
#26150=DIRECTION ( 'NONE',  ( 1.000000000000000000, -5.551115123125773458E-17, -1.260129944081490338E-35 ) ) ;
#26151=ADVANCED_FACE ( 'NONE', ( #8119 ), #19381, .T. ) ;
#26155=( BOUNDED_CURVE ( )  B_SPLINE_CURVE ( 2, ( #26552, #453, #19520, #12327, #3055, #19219, #26404, #21673, #28694 ),
 .UNSPECIFIED., .F., .T. ) 
 B_SPLINE_CURVE_WITH_KNOTS ( ( 3, 2, 2, 2, 3 ),
 ( 0.2861111111111112049, 0.2870370370370370905, 0.2888888888888888618, 0.2907407407407407440, 0.2916666666666666297 ),
 .UNSPECIFIED. ) 
 CURVE ( )  GEOMETRIC_REPRESENTATION_ITEM ( )  RATIONAL_B_SPLINE_CURVE ( ( 0.9330127018922194093, 0.9330127018922234061, 1.000000000000000000, 0.8660254037844388186, 1.000000000000000000, 0.8660254037844388186, 1.000000000000000000, 0.9330127018922234061, 0.9330127018922194093 ) ) 
 REPRESENTATION_ITEM ( '' )  );
#26156=CARTESIAN_POINT ( 'NONE',  ( -4.763139720814407951, 2.749999999999946709, -142.2500000000000000 ) ) ;
#26157=CARTESIAN_POINT ( 'NONE',  ( -5.412658773652684552, -3.125000000000099920, -151.4330127018922383 ) ) ;
#26159=CARTESIAN_POINT ( 'NONE',  ( -3.175426480542816066, 5.499999999999865885, -73.37500000000000000 ) ) ;
#26162=CARTESIAN_POINT ( 'NONE',  ( 3.175426480543072749, 5.499999999999865885, -69.12500000000002842 ) ) ;
#26164=CARTESIAN_POINT ( 'NONE',  ( 6.000000000000000888, 1.607695154586715303, -54.01933756729742697 ) ) ;
#26169=CARTESIAN_POINT ( 'NONE',  ( 5.196152422706629359, 3.000000000000002665, -127.4613248654052313 ) ) ;
#26172=CARTESIAN_POINT ( 'NONE',  ( 6.000000000000026645, -1.607695154586707753, -144.7306624327026157 ) ) ;
#26173=VERTEX_POINT ( 'NONE', #24118 ) ;
#26177=CARTESIAN_POINT ( 'NONE',  ( 6.000000000000000000, 2.951592740943527306E-14, -154.5863248654052029 ) ) ;
#26179=ORIENTED_EDGE ( 'NONE', *, *, #1620, .T. ) ;
#26180=CARTESIAN_POINT ( 'NONE',  ( -3.608439182435052128, -6.250000000000110134, -153.4419872981078470 ) ) ;
#26182=CARTESIAN_POINT ( 'NONE',  ( -2.775557561562891351E-14, -5.500000000000115463, -83.25000000000004263 ) ) ;
#26183=CARTESIAN_POINT ( 'NONE',  ( 5.412658773652712085, -3.125000000000086153, -99.93301270189225249 ) ) ;
#26185=CARTESIAN_POINT ( 'NONE',  ( 0.000000000000000000, 5.999999999999977796, -147.2886751345948824 ) ) ;
#26186=EDGE_CURVE ( 'NONE', #22716, #6411, #12490, .T. ) ;
#26188=CARTESIAN_POINT ( 'NONE',  ( 6.000000000000000888, -1.859271017917181981E-14, -59.16367513459483263 ) ) ;
#26191=CARTESIAN_POINT ( 'NONE',  ( 3.175426480543072749, 5.499999999999865885, -160.6250000000000284 ) ) ;
#26192=CARTESIAN_POINT ( 'NONE',  ( -5.999999999999963585, 1.780251999655701777E-13, -60.83632486540522422 ) ) ;
#26193=CARTESIAN_POINT ( 'NONE',  ( -2.775557561562891351E-14, -5.500000000000115463, -152.2500000000000000 ) ) ;
#26195=CARTESIAN_POINT ( 'NONE',  ( -6.350852961085760029, -1.281975124255709124E-13, -92.62500000000001421 ) ) ;
#26198=CARTESIAN_POINT ( 'NONE',  ( -6.350852961085760029, -1.281975124255709124E-13, -92.62500000000001421 ) ) ;
#26201=CYLINDRICAL_SURFACE ( 'NONE', #3233, 6.000000000000000888 ) ;
#26208=CARTESIAN_POINT ( 'NONE',  ( 0.000000000000000000, 0.000000000000000000, 0.000000000000000000 ) ) ;
#26212=CARTESIAN_POINT ( 'NONE',  ( 4.763139720814407951, 2.750000000000002665, -114.2500000000000142 ) ) ;
#26214=CARTESIAN_POINT ( 'NONE',  ( 3.608439182435180470, -6.249999999999997335, -127.0580127018922525 ) ) ;
#26216=ORIENTED_EDGE ( 'NONE', *, *, #29723, .T. ) ;
#26217=CARTESIAN_POINT ( 'NONE',  ( -5.196152422706573404, -3.000000000000002665, -61.28867513459484684 ) ) ;
#26218=CARTESIAN_POINT ( 'NONE',  ( 3.608439182435180470, -6.249999999999997335, -159.1919872981078470 ) ) ;
#26223=CARTESIAN_POINT ( 'NONE',  ( -3.608439182435115633, 6.249999999999965361, -61.80801270189223828 ) ) ;
#26224=ORIENTED_EDGE ( 'NONE', *, *, #10188, .F. ) ;
#26226=EDGE_CURVE ( 'NONE', #12504, #11496, #15489, .T. ) ;
#26228=CARTESIAN_POINT ( 'NONE',  ( -6.000249633052390230, 9.219381998443786586, -24.80704692217342355 ) ) ;
#26230=CARTESIAN_POINT ( 'NONE',  ( -3.175426480542816510, -5.500000000000057732, -176.3750000000000284 ) ) ;
#26233=CARTESIAN_POINT ( 'NONE',  ( 5.412658773652712085, -3.125000000000086153, -176.4330127018922667 ) ) ;
#26236=CARTESIAN_POINT ( 'NONE',  ( 4.763139720814407951, -2.749999999999988454, -123.5000000000000568 ) ) ;
#26237=CARTESIAN_POINT ( 'NONE',  ( 6.000000000000000888, -1.859271017917181981E-14, -84.66367513459482552 ) ) ;
#26238=CARTESIAN_POINT ( 'NONE',  ( 6.350852961086080661, -9.614813431917819062E-14, -109.8750000000000426 ) ) ;
#26239=VECTOR ( 'NONE', #18625, 1000.000000000000000 ) ;
#26241=ORIENTED_EDGE ( 'NONE', *, *, #30327, .T. ) ;
#26244=DIRECTION ( 'NONE',  ( 1.000000000000000000, -5.551115123125774690E-17, 0.000000000000000000 ) ) ;
#26245=CARTESIAN_POINT ( 'NONE',  ( 3.464101615137757051, -5.999999999999979572, -136.8363248654052313 ) ) ;
#26247=ORIENTED_EDGE ( 'NONE', *, *, #13988, .T. ) ;
#26250=CARTESIAN_POINT ( 'NONE',  ( 4.763139720814407951, -2.749999999999988454, -177.5000000000000000 ) ) ;
#26252=FACE_OUTER_BOUND ( 'NONE', #5057, .T. ) ;
#26253=ORIENTED_EDGE ( 'NONE', *, *, #30040, .F. ) ;
#26259=VECTOR ( 'NONE', #1329, 1000.000000000000000 ) ;
#26260=CARTESIAN_POINT ( 'NONE',  ( 5.412658773652739619, 3.124999999999988898, -131.8169872981078186 ) ) ;
#26263=DIRECTION ( 'NONE',  ( -7.147005652999508048E-36, 5.642372883946980038E-36, 1.000000000000000000 ) ) ;
#26266=CARTESIAN_POINT ( 'NONE',  ( 6.000000000000000888, -1.859271017917181981E-14, -67.58632486540523132 ) ) ;
#26268=ADVANCED_FACE ( 'NONE', ( #15184 ), #26808, .T. ) ;
#26273=CARTESIAN_POINT ( 'NONE',  ( 0.000000000000000000, 0.000000000000000000, 0.000000000000000000 ) ) ;
#26275=CARTESIAN_POINT ( 'NONE',  ( -3.175426480542816510, 5.499999999999865885, -139.3750000000000568 ) ) ;
#26278=VERTEX_POINT ( 'NONE', #5475 ) ;
#26280=CARTESIAN_POINT ( 'NONE',  ( 5.196152422706629359, 3.000000000000002665, -53.03867513459481131 ) ) ;
#26282=CARTESIAN_POINT ( 'NONE',  ( 3.464101615137852974, 5.999999999999884537, -152.8363248654051745 ) ) ;
#26283=ORIENTED_EDGE ( 'NONE', *, *, #6647, .F. ) ;
#26286=CARTESIAN_POINT ( 'NONE',  ( -5.412658773652739619, 3.124999999999975131, -95.31698729810783277 ) ) ;
#26287=CARTESIAN_POINT ( 'NONE',  ( 6.000000000000000888, 1.743066579297358182E-13, -50.16367513459482552 ) ) ;
#26290=VECTOR ( 'NONE', #30102, 1000.000000000000000 ) ;
#26292=CARTESIAN_POINT ( 'NONE',  ( -3.175426480542816510, -5.500000000000057732, -131.3750000000000000 ) ) ;
#26293=ORIENTED_EDGE ( 'NONE', *, *, #10984, .T. ) ;
#26294=CARTESIAN_POINT ( 'NONE',  ( 4.763139720814407951, -2.749999999999988454, -59.00000000000004974 ) ) ;
#26296=DIRECTION ( 'NONE',  ( -7.147005652999508048E-36, 5.642372883946980038E-36, 1.000000000000000000 ) ) ;
#26297=CARTESIAN_POINT ( 'NONE',  ( 5.197786390520589883, 9.697480688945329774, -28.02189831943640996 ) ) ;
#26298=CARTESIAN_POINT ( 'NONE',  ( 7.216878364870455975, -6.409875621278545621E-14, -84.80801270189222407 ) ) ;
#26305=CARTESIAN_POINT ( 'NONE',  ( 4.763139720814407951, 2.750000000000002665, -136.7500000000000284 ) ) ;
#26307=CARTESIAN_POINT ( 'NONE',  ( -7.216878364870328078, 0.000000000000000000, -151.5580127018922099 ) ) ;
#26308=CARTESIAN_POINT ( 'NONE',  ( 5.196152422706629359, 3.000000000000002665, -158.9613248654052597 ) ) ;
#26310=CARTESIAN_POINT ( 'NONE',  ( 4.763139720814407951, -2.749999999999988454, -68.00000000000000000 ) ) ;
#26311=CARTESIAN_POINT ( 'NONE',  ( 4.763139720814407951, 2.750000000000002665, -63.25000000000002842 ) ) ;
#26315=CARTESIAN_POINT ( 'NONE',  ( -3.464101615137757051, -5.999999999999979572, -104.6636751345948539 ) ) ;
#26317=CARTESIAN_POINT ( 'NONE',  ( 5.196152422706629359, -2.999999999999988898, -144.7886751345948255 ) ) ;
#26318=ORIENTED_EDGE ( 'NONE', *, *, #24312, .F. ) ;
#26320=EDGE_CURVE ( 'NONE', #3131, #8715, #21790, .T. ) ;
#26323=CARTESIAN_POINT ( 'NONE',  ( 0.000000000000000000, -5.999999999999991118, -158.5386751345948539 ) ) ;
#26324=CARTESIAN_POINT ( 'NONE',  ( -3.175426480542816510, 5.499999999999865885, -179.8750000000000000 ) ) ;
#26325=CIRCLE ( 'NONE', #16086, 2.000000000000003109 ) ;
#26327=ORIENTED_EDGE ( 'NONE', *, *, #18747, .T. ) ;
#26329=CARTESIAN_POINT ( 'NONE',  ( -3.175426480542816510, 5.499999999999865885, -85.37500000000004263 ) ) ;
#26330=EDGE_CURVE ( 'NONE', #5324, #11924, #24676, .T. ) ;
#26331=CARTESIAN_POINT ( 'NONE',  ( 2.775557561562891351E-14, 6.250000000000033751, -99.43301270189225249 ) ) ;
#26339=VECTOR ( 'NONE', #8820, 1000.000000000000000 ) ;
#26341=CARTESIAN_POINT ( 'NONE',  ( -4.763139720814407951, 2.749999999999946709, -161.7500000000000568 ) ) ;
#26343=CARTESIAN_POINT ( 'NONE',  ( -2.775557561562891351E-14, -5.500000000000115463, -158.2500000000000000 ) ) ;
#26345=CARTESIAN_POINT ( 'NONE',  ( -2.775557561562891351E-14, -5.500000000000115463, -90.75000000000000000 ) ) ;
#26347=LINE ( 'NONE', #23479, #4941 ) ;
#26348=CARTESIAN_POINT ( 'NONE',  ( 3.175426480543072749, -5.500000000000105693, -92.12500000000001421 ) ) ;
#26350=CARTESIAN_POINT ( 'NONE',  ( 6.000000000000000888, 1.743066579297358182E-13, -65.16367513459479710 ) ) ;
#26355=DIRECTION ( 'NONE',  ( -7.147005652999508048E-36, 5.642372883946980038E-36, 1.000000000000000000 ) ) ;
#26359=VECTOR ( 'NONE', #21291, 1000.000000000000000 ) ;
#26364=ORIENTED_EDGE ( 'NONE', *, *, #25536, .T. ) ;
#26366=EDGE_LOOP ( 'NONE', ( #18480, #29306, #5604, #16590 ) ) ;
#26367=CARTESIAN_POINT ( 'NONE',  ( 0.000000000000000000, 5.499999999999991118, -105.0000000000000426 ) ) ;
#26369=EDGE_CURVE ( 'NONE', #13111, #11998, #18619, .T. ) ;
#26370=CARTESIAN_POINT ( 'NONE',  ( -3.608439182435052128, -6.250000000000110134, -119.8080127018922667 ) ) ;
#26372=CARTESIAN_POINT ( 'NONE',  ( 3.608439182435180470, -6.249999999999997335, -163.6919872981078754 ) ) ;
#26375=( BOUNDED_CURVE ( )  B_SPLINE_CURVE ( 2, ( #5220, #2772, #14923, #12199, #12047, #3208, #17240, #14634, #7682 ),
 .UNSPECIFIED., .F., .F. ) 
 B_SPLINE_CURVE_WITH_KNOTS ( ( 3, 2, 2, 2, 3 ),
 ( 0.3916666666666666075, 0.3925925925925926041, 0.3944444444444444864, 0.3962962962962962576, 0.3972222222222222543 ),
 .UNSPECIFIED. ) 
 CURVE ( )  GEOMETRIC_REPRESENTATION_ITEM ( )  RATIONAL_B_SPLINE_CURVE ( ( 0.9330127018922194093, 0.9330127018922154125, 1.000000000000000000, 0.8660254037844388186, 1.000000000000000000, 0.8660254037844388186, 1.000000000000000000, 0.9330127018922154125, 0.9330127018922194093 ) ) 
 REPRESENTATION_ITEM ( '' )  );
#26376=CARTESIAN_POINT ( 'NONE',  ( -5.412658773652684552, -3.125000000000099920, -58.43301270189227381 ) ) ;
#26378=CARTESIAN_POINT ( 'NONE',  ( -2.145494852022792998, 10.79031218954990479, -19.39330237445248528 ) ) ;
#26379=DIRECTION ( 'NONE',  ( -7.147005652999508048E-36, 5.642372883946980038E-36, 1.000000000000000000 ) ) ;
#26380=CARTESIAN_POINT ( 'NONE',  ( -5.196152422706573404, -3.000000000000002665, -150.7113248654052313 ) ) ;
#26384=CARTESIAN_POINT ( 'NONE',  ( 3.608439182435180470, -6.249999999999997335, -169.0580127018922383 ) ) ;
#26387=( BOUNDED_CURVE ( )  B_SPLINE_CURVE ( 2, ( #9034, #23334, #18422, #2277, #8295, #18730, #27743, #27899, #20147 ),
 .UNSPECIFIED., .F., .T. ) 
 B_SPLINE_CURVE_WITH_KNOTS ( ( 3, 2, 2, 2, 3 ),
 ( 0.1472222222222221988, 0.1481481481481481399, 0.1499999999999999944, 0.1518518518518518490, 0.1527777777777777901 ),
 .UNSPECIFIED. ) 
 CURVE ( )  GEOMETRIC_REPRESENTATION_ITEM ( )  RATIONAL_B_SPLINE_CURVE ( ( 0.9330127018922196314, 0.9330127018922185211, 1.000000000000000000, 0.8660254037844388186, 1.000000000000000000, 0.8660254037844388186, 1.000000000000000000, 0.9330127018922184101, 0.9330127018922194093 ) ) 
 REPRESENTATION_ITEM ( '' )  );
#26388=CARTESIAN_POINT ( 'NONE',  ( -4.763139720814407951, 2.749999999999946709, -116.7500000000000142 ) ) ;
#26389=CARTESIAN_POINT ( 'NONE',  ( -3.175426480542816510, 5.499999999999865885, -115.3750000000000000 ) ) ;
#26391=CARTESIAN_POINT ( 'NONE',  ( 0.000000000000000000, -5.999999999999991118, -131.5386751345948255 ) ) ;
#26392=VERTEX_POINT ( 'NONE', #4088 ) ;
#26394=CARTESIAN_POINT ( 'NONE',  ( 6.000000000000000888, -1.859271017917181981E-14, -109.5863248654052029 ) ) ;
#26395=ORIENTED_EDGE ( 'NONE', *, *, #5061, .T. ) ;
#26397=DIRECTION ( 'NONE',  ( -7.147005652999508048E-36, 5.642372883946980038E-36, 1.000000000000000000 ) ) ;
#26400=VERTEX_POINT ( 'NONE', #18258 ) ;
#26401=EDGE_CURVE ( 'NONE', #3499, #29376, #21741, .T. ) ;
#26402=VERTEX_POINT ( 'NONE', #13662 ) ;
#26404=CARTESIAN_POINT ( 'NONE',  ( 5.196152422706629359, 3.000000000000002665, -85.46132486540525974 ) ) ;
#26408=CARTESIAN_POINT ( 'NONE',  ( 5.412658773652712085, -3.125000000000086153, -133.5669872981078470 ) ) ;
#26412=ORIENTED_EDGE ( 'NONE', *, *, #2004, .T. ) ;
#26420=CARTESIAN_POINT ( 'NONE',  ( 6.000000000000000888, 7.762456499804235646E-14, -138.0863248654052029 ) ) ;
#26423=CARTESIAN_POINT ( 'NONE',  ( 4.763139720814407951, -2.749999999999988454, -134.0000000000000000 ) ) ;
#26424=DIRECTION ( 'NONE',  ( -7.147005652999508048E-36, 5.642372883946980038E-36, 1.000000000000000000 ) ) ;
#26425=ORIENTED_EDGE ( 'NONE', *, *, #24669, .T. ) ;
#26426=CARTESIAN_POINT ( 'NONE',  ( -2.775557561562891351E-14, -5.500000000000115463, -48.75000000000001421 ) ) ;
#26428=EDGE_LOOP ( 'NONE', ( #6726, #7734, #24828, #18734 ) ) ;
#26431=CARTESIAN_POINT ( 'NONE',  ( -7.216878364870328078, 0.000000000000000000, -92.19198729810779014 ) ) ;
#26432=ADVANCED_FACE ( 'NONE', ( #23005 ), #1948, .T. ) ;
#26439=CARTESIAN_POINT ( 'NONE',  ( -4.763139720814407951, 2.749999999999946709, -125.7500000000000284 ) ) ;
#26441=ORIENTED_EDGE ( 'NONE', *, *, #17425, .F. ) ;
#26442=CARTESIAN_POINT ( 'NONE',  ( 3.464101615137757051, -5.999999999999979572, -82.83632486540524553 ) ) ;
#26443=CARTESIAN_POINT ( 'NONE',  ( 0.000000000000000000, 5.499999999999991118, -61.50000000000000000 ) ) ;
#26444=VECTOR ( 'NONE', #656, 1000.000000000000000 ) ;
#26445=CARTESIAN_POINT ( 'NONE',  ( 0.000000000000000000, 0.000000000000000000, -43.99152654425658682 ) ) ;
#26446=CARTESIAN_POINT ( 'NONE',  ( -6.000000000000007105, -1.607695154586655129, -62.84668783648705670 ) ) ;
#26447=CARTESIAN_POINT ( 'NONE',  ( -5.412658773652739619, 3.124999999999975131, -82.68301270189226670 ) ) ;
#26450=CARTESIAN_POINT ( 'NONE',  ( 6.000000000000000888, -1.859271017917181981E-14, -168.0863248654052029 ) ) ;
#26452=CARTESIAN_POINT ( 'NONE',  ( 3.464101615137852974, 5.999999999999884537, -61.33632486540521001 ) ) ;
#26454=CARTESIAN_POINT ( 'NONE',  ( -3.175426480542816066, 5.499999999999865885, -143.8750000000000000 ) ) ;
#26456=CARTESIAN_POINT ( 'NONE',  ( -5.412658773652739619, 3.124999999999975131, -156.1830127018922667 ) ) ;
#26458=CARTESIAN_POINT ( 'NONE',  ( 0.000000000000000000, 5.499999999999991118, -69.00000000000000000 ) ) ;
#26459=CARTESIAN_POINT ( 'NONE',  ( 3.175426480543072749, -5.500000000000105693, -57.62500000000004974 ) ) ;
#26462=DIRECTION ( 'NONE',  ( 1.000000000000000000, -5.551115123125774074E-17, 0.000000000000000000 ) ) ;
#26463=CARTESIAN_POINT ( 'NONE',  ( -5.999999999999963585, 1.780251999655701777E-13, -104.9136751345948255 ) ) ;
#26468=AXIS2_PLACEMENT_3D ( 'NONE', #26700, #10614, #11193 ) ;
#26470=CARTESIAN_POINT ( 'NONE',  ( 0.000000000000000000, 5.499999999999991118, -178.5000000000000000 ) ) ;
#26473=CARTESIAN_POINT ( 'NONE',  ( -4.763139720814407951, -2.750000000000016431, -79.00000000000001421 ) ) ;
#26476=CARTESIAN_POINT ( 'NONE',  ( 0.000000000000000000, 0.000000000000000000, 0.000000000000000000 ) ) ;
#26479=CARTESIAN_POINT ( 'NONE',  ( -3.175426480542816066, 5.499999999999865885, -160.3750000000000000 ) ) ;
#26480=CARTESIAN_POINT ( 'NONE',  ( -5.999999999999919176, 1.607695154586804565, -161.4033121635129930 ) ) ;
#26481=CARTESIAN_POINT ( 'NONE',  ( -3.175426480542816510, 5.499999999999865885, -148.3750000000000568 ) ) ;
#26482=EDGE_CURVE ( 'NONE', #26042, #2096, #18255, .T. ) ;
#26483=DIRECTION ( 'NONE',  ( -7.147005652999508048E-36, 5.642372883946980038E-36, 1.000000000000000000 ) ) ;
#26484=CARTESIAN_POINT ( 'NONE',  ( 3.464101615137757051, -5.999999999999979572, -51.91367513459486105 ) ) ;
#26485=ADVANCED_FACE ( 'NONE', ( #23165 ), #21303, .T. ) ;
#26486=CARTESIAN_POINT ( 'NONE',  ( -3.175426480542816066, -5.500000000000057732, -93.87500000000002842 ) ) ;
#26488=CARTESIAN_POINT ( 'NONE',  ( -4.763139720814407951, -2.750000000000016431, -82.00000000000001421 ) ) ;
#26491=CARTESIAN_POINT ( 'NONE',  ( -5.196152422706601826, 2.999999999999975131, -143.4613248654052029 ) ) ;
#26494=FACE_OUTER_BOUND ( 'NONE', #25464, .T. ) ;
#26495=CARTESIAN_POINT ( 'NONE',  ( -5.196152422706601826, 2.999999999999975131, -72.03867513459482552 ) ) ;
#26496=ADVANCED_FACE ( 'NONE', ( #20852 ), #16126, .T. ) ;
#26502=CARTESIAN_POINT ( 'NONE',  ( 6.000000000000000888, 7.762456499804235646E-14, -143.1636751345948255 ) ) ;
#26503=CARTESIAN_POINT ( 'NONE',  ( 6.000000000000000888, 1.743066579297358182E-13, -81.08632486540518869 ) ) ;
#26507=( BOUNDED_CURVE ( )  B_SPLINE_CURVE ( 2, ( #28541, #23962, #7799, #12319, #26542, #17066, #24698, #10594, #22985 ),
 .UNSPECIFIED., .F., .F. ) 
 B_SPLINE_CURVE_WITH_KNOTS ( ( 3, 2, 2, 2, 3 ),
 ( 0.7361111111111111605, 0.7370370370370370461, 0.7388888888888889284, 0.7407407407407406996, 0.7416666666666666963 ),
 .UNSPECIFIED. ) 
 CURVE ( )  GEOMETRIC_REPRESENTATION_ITEM ( )  RATIONAL_B_SPLINE_CURVE ( ( 0.9330127018922194093, 0.9330127018922234061, 1.000000000000000000, 0.8660254037844388186, 1.000000000000000000, 0.8660254037844388186, 1.000000000000000000, 0.9330127018922154125, 0.9330127018922194093 ) ) 
 REPRESENTATION_ITEM ( '' )  );
#26508=AXIS2_PLACEMENT_3D ( 'NONE', #16132, #18267, #27578 ) ;
#26511=CARTESIAN_POINT ( 'NONE',  ( -2.775557561562891351E-14, -5.500000000000115463, -105.7500000000000142 ) ) ;
#26513=CARTESIAN_POINT ( 'NONE',  ( 5.412658773652739619, 3.124999999999988898, -126.6830127018922525 ) ) ;
#26515=ORIENTED_EDGE ( 'NONE', *, *, #14815, .F. ) ;
#26517=CARTESIAN_POINT ( 'NONE',  ( -7.216878364870328078, 0.000000000000000000, -161.1919872981078754 ) ) ;
#26520=CARTESIAN_POINT ( 'NONE',  ( -3.608439182435052128, -6.250000000000110134, -62.80801270189225249 ) ) ;
#26521=ORIENTED_EDGE ( 'NONE', *, *, #5351, .F. ) ;
#26522=CARTESIAN_POINT ( 'NONE',  ( -3.464101615137725076, 5.999999999999979572, -117.1636751345948255 ) ) ;
#26523=CARTESIAN_POINT ( 'NONE',  ( 5.196152422706629359, -2.999999999999988898, -132.2113248654052029 ) ) ;
#26525=CARTESIAN_POINT ( 'NONE',  ( -3.175426480542816510, -5.500000000000057732, -174.8750000000000284 ) ) ;
#26528=CARTESIAN_POINT ( 'NONE',  ( -7.216878364870328078, 0.000000000000000000, -169.5580127018922383 ) ) ;
#26530=EDGE_CURVE ( 'NONE', #19941, #15497, #27816, .T. ) ;
#26533=CARTESIAN_POINT ( 'NONE',  ( -6.350852961085760029, -1.281975124255709124E-13, -119.6250000000000426 ) ) ;
#26534=CARTESIAN_POINT ( 'NONE',  ( -5.196152422706601826, 2.999999999999975131, -84.03867513459483973 ) ) ;
#26535=CARTESIAN_POINT ( 'NONE',  ( -3.175426480542816510, -5.500000000000057732, -114.8749999999999858 ) ) ;
#26536=CARTESIAN_POINT ( 'NONE',  ( 5.196152422706629359, -2.999999999999988898, -131.2886751345948539 ) ) ;
#26539=CARTESIAN_POINT ( 'NONE',  ( 5.196152422706629359, -2.999999999999988898, -90.21132486540523132 ) ) ;
#26540=CARTESIAN_POINT ( 'NONE',  ( 5.196152422706629359, 3.000000000000002665, -109.4613248654052171 ) ) ;
#26541=EDGE_CURVE ( 'NONE', #26551, #23459, #21393, .T. ) ;
#26542=CARTESIAN_POINT ( 'NONE',  ( 0.000000000000000000, -5.999999999999991118, -145.9613248654052597 ) ) ;
#26546=CARTESIAN_POINT ( 'NONE',  ( 4.763139720814407951, 2.750000000000002665, -178.7500000000000284 ) ) ;
#26547=CARTESIAN_POINT ( 'NONE',  ( -5.412658773652684552, -3.125000000000099920, -84.56698729810784698 ) ) ;
#26549=ORIENTED_EDGE ( 'NONE', *, *, #9084, .F. ) ;
#26551=VERTEX_POINT ( 'NONE', #13820 ) ;
#26552=CARTESIAN_POINT ( 'NONE',  ( -5.999999999999963585, 1.780251999655701777E-13, -84.83632486540523132 ) ) ;
#26556=CARTESIAN_POINT ( 'NONE',  ( -5.999999999999963585, -1.487416814333745711E-14, -143.9136751345948255 ) ) ;
#26557=CARTESIAN_POINT ( 'NONE',  ( -3.608439182435052128, -6.250000000000110134, -133.9419872981078186 ) ) ;
#26560=FACE_OUTER_BOUND ( 'NONE', #6468, .T. ) ;
#26561=ORIENTED_EDGE ( 'NONE', *, *, #2428, .T. ) ;
#26563=CARTESIAN_POINT ( 'NONE',  ( -5.196152422706601826, 2.999999999999975131, -135.0386751345948824 ) ) ;
#26564=CARTESIAN_POINT ( 'NONE',  ( 0.000000000000000000, -5.999999999999991118, -139.0386751345948255 ) ) ;
#26567=DIRECTION ( 'NONE',  ( -7.147005652999508048E-36, 5.642372883946980038E-36, 1.000000000000000000 ) ) ;
#26568=DIRECTION ( 'NONE',  ( -7.147005652999508048E-36, 5.642372883946980038E-36, 1.000000000000000000 ) ) ;
#26572=CARTESIAN_POINT ( 'NONE',  ( 4.763139720814407951, 2.750000000000002665, -141.2500000000000000 ) ) ;
#26573=ORIENTED_EDGE ( 'NONE', *, *, #6480, .F. ) ;
#26574=CARTESIAN_POINT ( 'NONE',  ( -6.000000000000000888, 1.067854986875958443E-15, 7.560779664488942560E-35 ) ) ;
#26575=CARTESIAN_POINT ( 'NONE',  ( -3.175426480542816066, -5.500000000000057732, -47.37500000000000000 ) ) ;
#26576=CARTESIAN_POINT ( 'NONE',  ( -3.464101615137757051, -5.999999999999979572, -160.1636751345947687 ) ) ;
#26577=EDGE_CURVE ( 'NONE', #1984, #14122, #19583, .T. ) ;
#26581=CARTESIAN_POINT ( 'NONE',  ( -5.412658773652739619, 3.124999999999975131, -98.31698729810783277 ) ) ;
#26582=CARTESIAN_POINT ( 'NONE',  ( 5.196152422706629359, 3.000000000000002665, -173.0386751345947971 ) ) ;
#26589=CARTESIAN_POINT ( 'NONE',  ( -4.763139720814407951, -2.750000000000016431, -61.00000000000000000 ) ) ;
#26591=CYLINDRICAL_SURFACE ( 'NONE', #2439, 6.000000000000000888 ) ;
#26592=CARTESIAN_POINT ( 'NONE',  ( -5.999999999999963585, -1.487416814333745711E-14, -67.41367513459481131 ) ) ;
#26593=CARTESIAN_POINT ( 'NONE',  ( -5.412658773652684552, -3.125000000000099920, -73.43301270189222407 ) ) ;
#26595=CARTESIAN_POINT ( 'NONE',  ( 0.000000000000000000, 0.000000000000000000, 0.000000000000000000 ) ) ;
#26601=( GEOMETRIC_REPRESENTATION_CONTEXT ( 3 ) GLOBAL_UNCERTAINTY_ASSIGNED_CONTEXT ( ( #19266 ) ) GLOBAL_UNIT_ASSIGNED_CONTEXT ( ( #19158, #28186, #21459 ) ) REPRESENTATION_CONTEXT ( 'NONE', 'WORKASPACE' ) );
#26602=CARTESIAN_POINT ( 'NONE',  ( -3.175426480542816066, 5.499999999999865885, -142.3750000000000568 ) ) ;
#26603=CARTESIAN_POINT ( 'NONE',  ( 5.999999999999949374, 1.607695154586804565, -69.01933756729745539 ) ) ;
#26604=CARTESIAN_POINT ( 'NONE',  ( 2.775557561562891351E-14, 6.250000000000033751, -156.4330127018922383 ) ) ;
#26607=CARTESIAN_POINT ( 'NONE',  ( 3.175426480543072749, -5.500000000000105693, -72.62500000000005684 ) ) ;
#26608=CARTESIAN_POINT ( 'NONE',  ( 4.763139720814407951, 2.750000000000002665, -54.25000000000002132 ) ) ;
#26609=ORIENTED_EDGE ( 'NONE', *, *, #25239, .F. ) ;
#26612=CARTESIAN_POINT ( 'NONE',  ( -5.999999999999971578, 1.607695154586715303, -97.48066243270258724 ) ) ;
#26613=CARTESIAN_POINT ( 'NONE',  ( 6.000000000000000888, 1.743066579297358182E-13, -104.1636751345948397 ) ) ;
#26615=ORIENTED_EDGE ( 'NONE', *, *, #17989, .F. ) ;
#26620=CARTESIAN_POINT ( 'NONE',  ( 5.412658773652739619, 3.124999999999988898, -148.3169872981078186 ) ) ;
#26621=CARTESIAN_POINT ( 'NONE',  ( 3.175426480543072749, 5.499999999999865885, -84.12499999999997158 ) ) ;
#26623=CARTESIAN_POINT ( 'NONE',  ( 7.216878364870455975, -6.409875621278545621E-14, -98.30801270189222407 ) ) ;
#26625=CARTESIAN_POINT ( 'NONE',  ( 0.000000000000000000, 0.000000000000000000, 0.000000000000000000 ) ) ;
#26630=CARTESIAN_POINT ( 'NONE',  ( 0.000000000000000000, 5.499999999999991118, -163.5000000000000284 ) ) ;
#26631=CARTESIAN_POINT ( 'NONE',  ( -3.464101615137757051, -5.999999999999979572, -60.58632486540521001 ) ) ;
#26632=CARTESIAN_POINT ( 'NONE',  ( -4.763139720814407951, 2.749999999999946709, -148.2500000000000000 ) ) ;
#26635=CARTESIAN_POINT ( 'NONE',  ( 3.175426480543072749, 5.499999999999865885, -96.12500000000004263 ) ) ;
#26637=CARTESIAN_POINT ( 'NONE',  ( -3.175426480542816510, 5.499999999999865885, -82.37500000000002842 ) ) ;
#26639=CARTESIAN_POINT ( 'NONE',  ( -5.196152422706573404, -3.000000000000002665, -72.71132486540521711 ) ) ;
#26642=CARTESIAN_POINT ( 'NONE',  ( -5.196152422706601826, 2.999999999999975131, -128.4613248654051745 ) ) ;
#26643=CARTESIAN_POINT ( 'NONE',  ( 0.000000000000000000, 5.999999999999977796, -72.28867513459485394 ) ) ;
#26644=CARTESIAN_POINT ( 'NONE',  ( 5.999999999999949374, 1.607695154586804565, -78.59668783648706381 ) ) ;
#26645=VERTEX_POINT ( 'NONE', #19736 ) ;
#26647=DIRECTION ( 'NONE',  ( 1.000000000000000000, -5.551115123125773458E-17, -1.260129944081490338E-35 ) ) ;
#26652=CARTESIAN_POINT ( 'NONE',  ( 3.175426480543072749, -5.500000000000105693, -105.6250000000000142 ) ) ;
#26654=CARTESIAN_POINT ( 'NONE',  ( 5.412658773652712085, -3.125000000000086153, -125.4330127018922241 ) ) ;
#26656=CARTESIAN_POINT ( 'NONE',  ( -3.464101615137757051, -5.999999999999979572, -68.66367513459479710 ) ) ;
#26657=CARTESIAN_POINT ( 'NONE',  ( 7.216878364870455975, -6.409875621278545621E-14, -161.9419872981077901 ) ) ;
#26660=CARTESIAN_POINT ( 'NONE',  ( 3.608439182435180470, -6.249999999999997335, -59.55801270189223118 ) ) ;
#26661=ORIENTED_EDGE ( 'NONE', *, *, #1921, .F. ) ;
#26665=CARTESIAN_POINT ( 'NONE',  ( -5.195867772253099481, 9.698547982442537574, -21.97454809331925318 ) ) ;
#26667=CARTESIAN_POINT ( 'NONE',  ( -3.175426480542816510, -5.500000000000057732, -170.3750000000000568 ) ) ;
#26669=CARTESIAN_POINT ( 'NONE',  ( 6.000000000000000888, -1.859271017917181981E-14, -100.5863248654052171 ) ) ;
#26670=CARTESIAN_POINT ( 'NONE',  ( 3.608439182435180470, 6.249999999999982236, -165.5580127018922383 ) ) ;
#26673=CARTESIAN_POINT ( 'NONE',  ( -2.775557561562891351E-14, -5.500000000000115463, -113.2500000000000142 ) ) ;
#26675=( BOUNDED_CURVE ( )  B_SPLINE_CURVE ( 2, ( #5489, #20098, #15678, #24391, #24535, #3482, #27141, #26822, #13366 ),
 .UNSPECIFIED., .F., .T. ) 
 B_SPLINE_CURVE_WITH_KNOTS ( ( 3, 2, 2, 2, 3 ),
 ( 0.2805555555555555580, 0.2814814814814814437, 0.2833333333333333259, 0.2851851851851852082, 0.2861111111111112049 ),
 .UNSPECIFIED. ) 
 CURVE ( )  GEOMETRIC_REPRESENTATION_ITEM ( )  RATIONAL_B_SPLINE_CURVE ( ( 0.9330127018922194093, 0.9330127018922194093, 1.000000000000000000, 0.8660254037844388186, 1.000000000000000000, 0.8660254037844388186, 1.000000000000000000, 0.9330127018922154125, 0.9330127018922194093 ) ) 
 REPRESENTATION_ITEM ( '' )  );
#26676=CARTESIAN_POINT ( 'NONE',  ( 4.763139720814407951, 2.750000000000002665, -108.2500000000000142 ) ) ;
#26678=VERTEX_POINT ( 'NONE', #20047 ) ;
#26683=CARTESIAN_POINT ( 'NONE',  ( 5.196152422706629359, 3.000000000000002665, -65.96132486540523132 ) ) ;
#26684=CARTESIAN_POINT ( 'NONE',  ( -3.608439182435115633, 6.249999999999965361, -81.94198729810779014 ) ) ;
#26686=VERTEX_POINT ( 'NONE', #25232 ) ;
#26687=CARTESIAN_POINT ( 'NONE',  ( 0.000000000000000000, 0.000000000000000000, 0.000000000000000000 ) ) ;
#26688=ORIENTED_EDGE ( 'NONE', *, *, #11549, .F. ) ;
#26693=CARTESIAN_POINT ( 'NONE',  ( -7.216878364870328078, 0.000000000000000000, -129.6919872981078186 ) ) ;
#26694=CARTESIAN_POINT ( 'NONE',  ( -5.999999999999963585, 8.134310703387671600E-14, -135.8363248654052597 ) ) ;
#26695=CARTESIAN_POINT ( 'NONE',  ( 6.000000000000000888, -6.507448562710137091E-15, -175.5863248654052029 ) ) ;
#26696=ORIENTED_EDGE ( 'NONE', *, *, #14755, .T. ) ;
#26700=CARTESIAN_POINT ( 'NONE',  ( 0.000000000000000000, 0.000000000000000000, 0.000000000000000000 ) ) ;
#26702=CARTESIAN_POINT ( 'NONE',  ( -6.000000000000007105, -1.607695154586655129, -47.26933756729744829 ) ) ;
#26703=CARTESIAN_POINT ( 'NONE',  ( 2.775557561562891351E-14, -6.250000000000061284, -66.31698729810780435 ) ) ;
#26704=CARTESIAN_POINT ( 'NONE',  ( 7.216878364870455975, -6.409875621278545621E-14, -56.94198729810781145 ) ) ;
#26705=CARTESIAN_POINT ( 'NONE',  ( 5.196152422706629359, -2.999999999999988898, -128.2886751345948539 ) ) ;
#26708=CARTESIAN_POINT ( 'NONE',  ( -3.175426480542816510, -5.500000000000057732, -126.8749999999999858 ) ) ;
#26712=LINE ( 'NONE', #26574, #2829 ) ;
#26715=CARTESIAN_POINT ( 'NONE',  ( 6.000000000000000888, -1.859271017917181981E-14, -159.6636751345948539 ) ) ;
#26716=CARTESIAN_POINT ( 'NONE',  ( -5.999999999999963585, 1.780251999655701777E-13, -89.33632486540523132 ) ) ;
#26720=( BOUNDED_CURVE ( )  B_SPLINE_CURVE ( 2, ( #22166, #16830, #14957, #5099, #5402, #14525, #23864, #24009, #2804 ),
 .UNSPECIFIED., .F., .F. ) 
 B_SPLINE_CURVE_WITH_KNOTS ( ( 3, 2, 2, 2, 3 ),
 ( 0.7638888888888888395, 0.7648148148148148362, 0.7666666666666666075, 0.7685185185185184897, 0.7694444444444443754 ),
 .UNSPECIFIED. ) 
 CURVE ( )  GEOMETRIC_REPRESENTATION_ITEM ( )  RATIONAL_B_SPLINE_CURVE ( ( 0.9330127018922194093, 0.9330127018922154125, 1.000000000000000000, 0.8660254037844388186, 1.000000000000000000, 0.8660254037844388186, 1.000000000000000000, 0.9330127018922234061, 0.9330127018922194093 ) ) 
 REPRESENTATION_ITEM ( '' )  );
#26721=CARTESIAN_POINT ( 'NONE',  ( 3.608439182435180470, 6.249999999999982236, -92.69198729810779014 ) ) ;
#26728=ADVANCED_FACE ( 'NONE', ( #10534 ), #29393, .T. ) ;
#26731=CARTESIAN_POINT ( 'NONE',  ( -4.763139720814407951, 2.749999999999946709, -61.25000000000002842 ) ) ;
#26732=CARTESIAN_POINT ( 'NONE',  ( 0.000000000000000000, 5.999999999999977796, -69.28867513459479710 ) ) ;
#26733=CARTESIAN_POINT ( 'NONE',  ( 3.464101615137757051, -5.999999999999979572, -134.4136751345947971 ) ) ;
#26735=CARTESIAN_POINT ( 'NONE',  ( 2.775557561562891351E-14, -6.250000000000061284, -79.18301270189220986 ) ) ;
#26737=CARTESIAN_POINT ( 'NONE',  ( 6.000000000000000888, -1.607695154586752384, -168.1533121635130215 ) ) ;
#26739=CARTESIAN_POINT ( 'NONE',  ( 0.000000000000000000, -5.999999999999991118, -94.03867513459485394 ) ) ;
#26740=CARTESIAN_POINT ( 'NONE',  ( 4.763139720814407951, 2.750000000000002665, -132.2500000000000284 ) ) ;
#26741=VECTOR ( 'NONE', #19929, 1000.000000000000000 ) ;
#26742=CARTESIAN_POINT ( 'NONE',  ( 6.000000000000000888, 1.743066579297358182E-13, -74.16367513459482552 ) ) ;
#26745=CARTESIAN_POINT ( 'NONE',  ( 4.763139720814407951, -2.749999999999988454, -69.50000000000000000 ) ) ;
#26746=CARTESIAN_POINT ( 'NONE',  ( -6.350852961085760029, -1.281975124255709124E-13, -55.12500000000003553 ) ) ;
#26747=ORIENTED_EDGE ( 'NONE', *, *, #19463, .T. ) ;
#26751=AXIS2_PLACEMENT_3D ( 'NONE', #12680, #28904, #3406 ) ;
#26754=EDGE_LOOP ( 'NONE', ( #11857, #5835, #4158, #7989 ) ) ;
#26757=ADVANCED_FACE ( 'NONE', ( #17771 ), #22353, .T. ) ;
#26759=CARTESIAN_POINT ( 'NONE',  ( 4.763139720814407951, 2.750000000000002665, -145.7500000000000568 ) ) ;
#26761=CARTESIAN_POINT ( 'NONE',  ( 4.763139720814407951, 2.750000000000002665, -180.2500000000000284 ) ) ;
#26764=CARTESIAN_POINT ( 'NONE',  ( 5.412658773652739619, 3.124999999999988898, -145.3169872981078186 ) ) ;
#26765=CARTESIAN_POINT ( 'NONE',  ( 4.763139720814407951, -2.749999999999988454, -78.50000000000001421 ) ) ;
#26767=CARTESIAN_POINT ( 'NONE',  ( 3.608439182435180470, 6.249999999999982236, -95.05801270189226670 ) ) ;
#26768=CARTESIAN_POINT ( 'NONE',  ( -3.175426480542816510, 5.499999999999865885, -152.8749999999999716 ) ) ;
#26770=CARTESIAN_POINT ( 'NONE',  ( -5.196152422706573404, -3.000000000000002665, -96.71132486540523132 ) ) ;
#26771=CARTESIAN_POINT ( 'NONE',  ( 5.196152422706629359, -2.999999999999988898, -150.7886751345948255 ) ) ;
#26772=CARTESIAN_POINT ( 'NONE',  ( 5.196152422706629359, -2.999999999999988898, -90.78867513459488237 ) ) ;
#26775=CARTESIAN_POINT ( 'NONE',  ( -4.763139720814407951, 2.749999999999946709, -157.2500000000000000 ) ) ;
#26777=CARTESIAN_POINT ( 'NONE',  ( -6.350852961085760029, -1.281975124255709124E-13, -148.1250000000000284 ) ) ;
#26779=CARTESIAN_POINT ( 'NONE',  ( 0.000000000000000000, 5.499999999999991118, -94.50000000000002842 ) ) ;
#26781=CARTESIAN_POINT ( 'NONE',  ( 6.350852961086080661, -9.614813431917819062E-14, -84.37500000000005684 ) ) ;
#26787=CARTESIAN_POINT ( 'NONE',  ( -5.999999999999963585, -1.487416814333745711E-14, -124.4136751345948255 ) ) ;
#26789=CARTESIAN_POINT ( 'NONE',  ( 0.000000000000000000, 0.000000000000000000, 0.000000000000000000 ) ) ;
#26792=CARTESIAN_POINT ( 'NONE',  ( -5.999999999999962697, 3.323446944526963891E-14, -157.4136751345948539 ) ) ;
#26795=VERTEX_POINT ( 'NONE', #24640 ) ;
#26796=EDGE_CURVE ( 'NONE', #23369, #10419, #13015, .T. ) ;
#26798=CARTESIAN_POINT ( 'NONE',  ( -3.175426480542816510, 5.499999999999865885, -109.3750000000000284 ) ) ;
#26801=CARTESIAN_POINT ( 'NONE',  ( -7.216878364870328078, 0.000000000000000000, -112.5580127018922241 ) ) ;
#26803=CARTESIAN_POINT ( 'NONE',  ( -7.216878364870328078, 0.000000000000000000, -156.6919872981078186 ) ) ;
#26806=CARTESIAN_POINT ( 'NONE',  ( -3.608439182435115633, 6.249999999999965361, -54.30801270189220276 ) ) ;
#26807=ORIENTED_EDGE ( 'NONE', *, *, #12812, .T. ) ;
#26808=CYLINDRICAL_SURFACE ( 'NONE', #1453, 6.000000000000000888 ) ;
#26809=CARTESIAN_POINT ( 'NONE',  ( -5.999999999999963585, 8.134310703387671600E-14, -119.9136751345948397 ) ) ;
#26810=CARTESIAN_POINT ( 'NONE',  ( 6.000000000000052403, -1.607695154586662678, -166.6533121635129646 ) ) ;
#26811=EDGE_CURVE ( 'NONE', #84, #19051, #25857, .T. ) ;
#26812=CARTESIAN_POINT ( 'NONE',  ( 0.000000000000000000, 0.000000000000000000, 0.000000000000000000 ) ) ;
#26814=CARTESIAN_POINT ( 'NONE',  ( -3.175426480542816510, -5.500000000000057732, -168.8750000000000568 ) ) ;
#26816=CARTESIAN_POINT ( 'NONE',  ( -7.216878364870328078, 0.000000000000000000, -172.5580127018922383 ) ) ;
#26819=CARTESIAN_POINT ( 'NONE',  ( -4.763139720814407951, -2.750000000000016431, -116.5000000000000426 ) ) ;
#26820=CARTESIAN_POINT ( 'NONE',  ( 3.175426480543072749, 5.499999999999865885, -102.1250000000000142 ) ) ;
#26822=CARTESIAN_POINT ( 'NONE',  ( -6.000000000000007105, -1.607695154586655129, -84.76933756729746960 ) ) ;
#26823=ORIENTED_EDGE ( 'NONE', *, *, #12886, .F. ) ;
#26826=DIRECTION ( 'NONE',  ( -7.147005652999508048E-36, 5.642372883946980038E-36, 1.000000000000000000 ) ) ;
#26830=CARTESIAN_POINT ( 'NONE',  ( 6.350852961086080661, -9.614813431917819062E-14, -159.3750000000000284 ) ) ;
#26832=CARTESIAN_POINT ( 'NONE',  ( 7.216878364870455975, -6.409875621278545621E-14, -82.44198729810780435 ) ) ;
#26834=VERTEX_POINT ( 'NONE', #8229 ) ;
#26835=CYLINDRICAL_SURFACE ( 'NONE', #5160, 6.000000000000000888 ) ;
#26836=EDGE_CURVE ( 'NONE', #21222, #956, #22083, .T. ) ;
#26841=CARTESIAN_POINT ( 'NONE',  ( -3.608439182435115633, 6.249999999999965361, -136.8080127018922667 ) ) ;
#26842=ORIENTED_EDGE ( 'NONE', *, *, #23986, .T. ) ;
#26844=CARTESIAN_POINT ( 'NONE',  ( 3.608439182435180470, -6.249999999999997335, -130.6919872981078470 ) ) ;
#26845=FACE_OUTER_BOUND ( 'NONE', #29272, .T. ) ;
#26846=CARTESIAN_POINT ( 'NONE',  ( -4.763139720814407951, 2.749999999999946709, -173.7500000000000284 ) ) ;
#26847=CARTESIAN_POINT ( 'NONE',  ( -5.999999999999963585, 1.780251999655701777E-13, -49.41367513459484684 ) ) ;
#26852=FACE_OUTER_BOUND ( 'NONE', #23605, .T. ) ;
#26855=CARTESIAN_POINT ( 'NONE',  ( -5.196152422706601826, 2.999999999999975131, -90.03867513459485394 ) ) ;
#26856=CARTESIAN_POINT ( 'NONE',  ( 0.000000000000000000, -5.999999999999991118, -107.5386751345948113 ) ) ;
#26857=CARTESIAN_POINT ( 'NONE',  ( -3.608439182435052128, -6.250000000000110134, -67.94198729810780435 ) ) ;
#26858=CARTESIAN_POINT ( 'NONE',  ( 5.412658773652739619, 3.124999999999988898, -53.81698729810779724 ) ) ;
#26859=FACE_OUTER_BOUND ( 'NONE', #28658, .T. ) ;
#26863=CARTESIAN_POINT ( 'NONE',  ( -3.175426480542816510, -5.500000000000057732, -128.3750000000000000 ) ) ;
#26864=CARTESIAN_POINT ( 'NONE',  ( 6.000000000000000888, 1.607695154586715303, -167.0966878364870354 ) ) ;
#26866=VERTEX_POINT ( 'NONE', #22384 ) ;
#26867=CARTESIAN_POINT ( 'NONE',  ( 5.196152422706629359, -2.999999999999988898, -118.7113248654052597 ) ) ;
#26871=CARTESIAN_POINT ( 'NONE',  ( -6.000000000000000888, 1.067854986875958443E-15, 7.560779664488942560E-35 ) ) ;
#26872=CARTESIAN_POINT ( 'NONE',  ( 6.000000000000000000, 2.951592740943527306E-14, -161.1636751345949108 ) ) ;
#26875=FACE_OUTER_BOUND ( 'NONE', #1658, .T. ) ;
#26877=CARTESIAN_POINT ( 'NONE',  ( 3.608439182435180470, 6.249999999999982236, -98.69198729810781856 ) ) ;
#26878=CARTESIAN_POINT ( 'NONE',  ( -5.999999999999956479, -1.607695154586745057, -54.76933756729744829 ) ) ;
#26883=ORIENTED_EDGE ( 'NONE', *, *, #20517, .T. ) ;
#26886=CARTESIAN_POINT ( 'NONE',  ( 0.000000000000000000, 5.499999999999991118, -46.49999999999998579 ) ) ;
#26887=CARTESIAN_POINT ( 'NONE',  ( -5.999999999999956479, -1.607695154586745057, -59.84668783648706381 ) ) ;
#26888=CARTESIAN_POINT ( 'NONE',  ( 2.775557561562891351E-14, 6.250000000000033751, -73.93301270189223828 ) ) ;
#26889=CARTESIAN_POINT ( 'NONE',  ( 6.000000000000000888, -1.859271017917181981E-14, -172.5863248654052029 ) ) ;
#26892=CARTESIAN_POINT ( 'NONE',  ( -1.285375204280330350E-15, -10.49588505988223375, 1.184433945098074864E-34 ) ) ;
#26893=CARTESIAN_POINT ( 'NONE',  ( 5.196152422706629359, -2.999999999999988898, -152.2886751345948255 ) ) ;
#26895=CARTESIAN_POINT ( 'NONE',  ( -4.763139720814407951, -2.750000000000016431, -133.0000000000000000 ) ) ;
#26898=CARTESIAN_POINT ( 'NONE',  ( 5.412658773652712085, -3.125000000000086153, -147.9330127018922383 ) ) ;
#26899=CARTESIAN_POINT ( 'NONE',  ( 0.000000000000000000, 5.999999999999977796, -158.7113248654052313 ) ) ;
#26901=CARTESIAN_POINT ( 'NONE',  ( 0.000000000000000000, 5.499999999999991118, -61.50000000000000000 ) ) ;
#26902=CARTESIAN_POINT ( 'NONE',  ( 4.763139720814407951, 2.750000000000002665, -60.25000000000002842 ) ) ;
#26904=ORIENTED_EDGE ( 'NONE', *, *, #1371, .F. ) ;
#26907=CARTESIAN_POINT ( 'NONE',  ( 5.196152422706629359, -2.999999999999988898, -98.28867513459482552 ) ) ;
#26909=EDGE_CURVE ( 'NONE', #3013, #23373, #8073, .T. ) ;
#26911=ORIENTED_EDGE ( 'NONE', *, *, #26330, .F. ) ;
#26915=VECTOR ( 'NONE', #2651, 1000.000000000000000 ) ;
#26916=CARTESIAN_POINT ( 'NONE',  ( -3.175426480542816510, 5.499999999999865885, -142.3750000000000568 ) ) ;
#26918=CARTESIAN_POINT ( 'NONE',  ( -3.608439182435115633, 6.249999999999965361, -48.94198729810783988 ) ) ;
#26921=CARTESIAN_POINT ( 'NONE',  ( 3.608439182435180470, -6.249999999999997335, -148.6919872981078186 ) ) ;
#26922=CARTESIAN_POINT ( 'NONE',  ( 4.763139720814407951, 2.750000000000002665, -72.25000000000004263 ) ) ;
#26923=CARTESIAN_POINT ( 'NONE',  ( 2.775557561562891351E-14, 6.250000000000033751, -96.43301270189225249 ) ) ;
#26926=CARTESIAN_POINT ( 'NONE',  ( 6.000000000000000888, 1.743066579297358182E-13, -96.08632486540521711 ) ) ;
#26927=CYLINDRICAL_SURFACE ( 'NONE', #20424, 6.000000000000000888 ) ;
#26928=CARTESIAN_POINT ( 'NONE',  ( 5.196152422706629359, 3.000000000000002665, -98.96132486540520290 ) ) ;
#26931=CARTESIAN_POINT ( 'NONE',  ( -6.350852961085760029, -1.281975124255709124E-13, -157.1250000000000284 ) ) ;
#26933=CARTESIAN_POINT ( 'NONE',  ( 3.175426480543072749, -5.500000000000105693, -147.6250000000000284 ) ) ;
#26934=CARTESIAN_POINT ( 'NONE',  ( 5.999999999999949374, 1.607695154586804565, -77.09668783648706381 ) ) ;
#26935=CARTESIAN_POINT ( 'NONE',  ( -3.464101615137757051, -5.999999999999979572, -92.66367513459478289 ) ) ;
#26939=CARTESIAN_POINT ( 'NONE',  ( -4.763139720814407951, 2.749999999999946709, -83.74999999999998579 ) ) ;
#26940=CARTESIAN_POINT ( 'NONE',  ( -3.175426480542816510, -5.500000000000057732, -81.87500000000004263 ) ) ;
#26944=CARTESIAN_POINT ( 'NONE',  ( -5.999999999999963585, -1.487416814333745711E-14, -105.8363248654052313 ) ) ;
#26945=FACE_OUTER_BOUND ( 'NONE', #16317, .T. ) ;
#26951=CARTESIAN_POINT ( 'NONE',  ( -5.196152422706601826, 2.999999999999975131, -75.03867513459483973 ) ) ;
#26952=( BOUNDED_CURVE ( )  B_SPLINE_CURVE ( 2, ( #5156, #12281, #19609, #21769, #28799, #10251, #19470, #28950, #22065 ),
 .UNSPECIFIED., .F., .F. ) 
 B_SPLINE_CURVE_WITH_KNOTS ( ( 3, 2, 2, 2, 3 ),
 ( 0.2027777777777777235, 0.2037037037037037202, 0.2055555555555556024, 0.2074074074074073737, 0.2083333333333333703 ),
 .UNSPECIFIED. ) 
 CURVE ( )  GEOMETRIC_REPRESENTATION_ITEM ( )  RATIONAL_B_SPLINE_CURVE ( ( 0.9330127018922194093, 0.9330127018922154125, 1.000000000000000000, 0.8660254037844388186, 1.000000000000000000, 0.8660254037844388186, 1.000000000000000000, 0.9330127018922154125, 0.9330127018922194093 ) ) 
 REPRESENTATION_ITEM ( '' )  );
#26953=ORIENTED_EDGE ( 'NONE', *, *, #20101, .F. ) ;
#26954=CARTESIAN_POINT ( 'NONE',  ( -5.196152422706601826, 2.999999999999975131, -72.96132486540524553 ) ) ;
#26955=CARTESIAN_POINT ( 'NONE',  ( -6.000000000000007105, -1.607695154586655129, -79.34668783648702117 ) ) ;
#26956=CARTESIAN_POINT ( 'NONE',  ( -5.999999999999963585, -1.487416814333745711E-14, -101.3363248654052171 ) ) ;
#26957=ORIENTED_EDGE ( 'NONE', *, *, #15058, .T. ) ;
#26959=CARTESIAN_POINT ( 'NONE',  ( 0.000000000000000000, 5.499999999999991118, -97.50000000000002842 ) ) ;
#26961=CYLINDRICAL_SURFACE ( 'NONE', #7702, 6.000000000000000888 ) ;
#26962=CARTESIAN_POINT ( 'NONE',  ( -7.216878364870328078, 0.000000000000000000, -114.0580127018922241 ) ) ;
#26963=ORIENTED_EDGE ( 'NONE', *, *, #270, .F. ) ;
#26964=CARTESIAN_POINT ( 'NONE',  ( 3.464101615137852974, 5.999999999999884537, -91.91367513459485394 ) ) ;
#26966=CARTESIAN_POINT ( 'NONE',  ( 2.775557561562891351E-14, -6.250000000000061284, -55.18301270189224539 ) ) ;
#26971=CARTESIAN_POINT ( 'NONE',  ( 3.175426480543072749, 5.499999999999865885, -169.6250000000000000 ) ) ;
#26973=CARTESIAN_POINT ( 'NONE',  ( -3.464101615137725076, 5.999999999999979572, -107.5863248654051603 ) ) ;
#26974=CARTESIAN_POINT ( 'NONE',  ( 3.608439182435180470, -6.249999999999997335, -172.0580127018922383 ) ) ;
#26977=CARTESIAN_POINT ( 'NONE',  ( 4.763139720814407951, -2.749999999999988454, -114.5000000000000426 ) ) ;
#26979=ADVANCED_FACE ( 'NONE', ( #3922, #16121 ), #20378, .F. ) ;
#26980=CARTESIAN_POINT ( 'NONE',  ( 6.350852961086080661, -9.614813431917819062E-14, -108.3750000000000426 ) ) ;
#26981=CARTESIAN_POINT ( 'NONE',  ( -5.196152422706573404, -3.000000000000002665, -87.71132486540523132 ) ) ;
#26983=ORIENTED_EDGE ( 'NONE', *, *, #21062, .F. ) ;
#26987=DIRECTION ( 'NONE',  ( -7.147005652999508048E-36, 5.642372883946980038E-36, 1.000000000000000000 ) ) ;
#26990=ORIENTED_EDGE ( 'NONE', *, *, #25790, .F. ) ;
#26991=CARTESIAN_POINT ( 'NONE',  ( -6.350852961085760029, -1.281975124255709124E-13, -158.6250000000000284 ) ) ;
#26993=CARTESIAN_POINT ( 'NONE',  ( 3.608439182435180470, 6.249999999999982236, -82.19198729810780435 ) ) ;
#26998=VERTEX_POINT ( 'NONE', #29886 ) ;
#27001=( BOUNDED_CURVE ( )  B_SPLINE_CURVE ( 2, ( #23574, #2510, #28302, #5101, #21418, #19119, #7282, #16686, #4953 ),
 .UNSPECIFIED., .F., .F. ) 
 B_SPLINE_CURVE_WITH_KNOTS ( ( 3, 2, 2, 2, 3 ),
 ( 0.9583333333333333703, 0.9592592592592592560, 0.9611111111111111382, 0.9629629629629630205, 0.9638888888888889062 ),
 .UNSPECIFIED. ) 
 CURVE ( )  GEOMETRIC_REPRESENTATION_ITEM ( )  RATIONAL_B_SPLINE_CURVE ( ( 0.9330127018922194093, 0.9330127018922234061, 1.000000000000000000, 0.8660254037844388186, 1.000000000000000000, 0.8660254037844388186, 1.000000000000000000, 0.9330127018922194093, 0.9330127018922194093 ) ) 
 REPRESENTATION_ITEM ( '' )  );
#27002=CARTESIAN_POINT ( 'NONE',  ( 3.175426480543072749, 5.499999999999865885, -132.1250000000000284 ) ) ;
#27003=CARTESIAN_POINT ( 'NONE',  ( -3.608439182435115633, 6.249999999999965361, -139.8080127018922667 ) ) ;
#27004=ORIENTED_EDGE ( 'NONE', *, *, #4385, .F. ) ;
#27005=DIRECTION ( 'NONE',  ( -7.147005652999508048E-36, 5.642372883946980038E-36, 1.000000000000000000 ) ) ;
#27006=CARTESIAN_POINT ( 'NONE',  ( 7.216878364870455975, -6.409875621278545621E-14, -122.9419872981078043 ) ) ;
#27008=CARTESIAN_POINT ( 'NONE',  ( 0.000000000000000000, 5.499999999999991118, -169.4999999999999716 ) ) ;
#27015=CARTESIAN_POINT ( 'NONE',  ( -6.000000000000023093, 1.607695154586625819, -147.9033121635129930 ) ) ;
#27016=CARTESIAN_POINT ( 'NONE',  ( 6.000000000000000888, 7.762456499804234384E-14, -117.0863248654052171 ) ) ;
#27017=CARTESIAN_POINT ( 'NONE',  ( 6.000000000000000888, -1.859271017917181981E-14, -171.6636751345948539 ) ) ;
#27020=CARTESIAN_POINT ( 'NONE',  ( 5.412658773652712085, -3.125000000000086153, -64.56698729810783277 ) ) ;
#27021=CARTESIAN_POINT ( 'NONE',  ( 7.216878364870455975, -6.409875621278545621E-14, -55.44198729810780435 ) ) ;
#27023=DIRECTION ( 'NONE',  ( -7.147005652999508048E-36, 5.642372883946980038E-36, 1.000000000000000000 ) ) ;
#27025=CARTESIAN_POINT ( 'NONE',  ( 0.000000000000000000, 5.999999999999977796, -127.7886751345948539 ) ) ;
#27026=EDGE_CURVE ( 'NONE', #18475, #17985, #10888, .T. ) ;
#27027=CARTESIAN_POINT ( 'NONE',  ( -6.350852961085760029, -1.281975124255709124E-13, -130.1250000000000284 ) ) ;
#27028=ORIENTED_EDGE ( 'NONE', *, *, #6087, .F. ) ;
#27031=CARTESIAN_POINT ( 'NONE',  ( -5.999999999999962697, 3.323446944526963891E-14, -147.8363248654052313 ) ) ;
#27032=ORIENTED_EDGE ( 'NONE', *, *, #18028, .T. ) ;
#27035=CARTESIAN_POINT ( 'NONE',  ( 5.412658773652712085, -3.125000000000086153, -114.0669872981078186 ) ) ;
#27037=CARTESIAN_POINT ( 'NONE',  ( -5.196152422706601826, 2.999999999999975131, -90.96132486540520290 ) ) ;
#27039=AXIS2_PLACEMENT_3D ( 'NONE', #23959, #14607, #19073 ) ;
#27043=AXIS2_PLACEMENT_3D ( 'NONE', #7507, #16921, #28091 ) ;
#27045=CARTESIAN_POINT ( 'NONE',  ( -5.196152422706601826, 2.999999999999975131, -81.03867513459483973 ) ) ;
#27046=EDGE_CURVE ( 'NONE', #25773, #20871, #18406, .T. ) ;
#27047=CARTESIAN_POINT ( 'NONE',  ( -6.350852961085760029, -1.281975124255709124E-13, -47.62500000000000000 ) ) ;
#27048=CARTESIAN_POINT ( 'NONE',  ( -3.464101615137757051, -5.999999999999979572, -62.66367513459483973 ) ) ;
#27049=CARTESIAN_POINT ( 'NONE',  ( -5.999999999999919176, 1.607695154586804565, -61.48066243270261566 ) ) ;
#27050=CARTESIAN_POINT ( 'NONE',  ( 7.216878364870455975, -6.409875621278545621E-14, -78.80801270189225249 ) ) ;
#27053=VECTOR ( 'NONE', #8687, 1000.000000000000000 ) ;
#27054=SURFACE_SIDE_STYLE ('',( #13136 ) ) ;
#27057=ADVANCED_FACE ( 'NONE', ( #20243 ), #27723, .T. ) ;
#27058=CARTESIAN_POINT ( 'NONE',  ( -4.763139720814407951, 2.749999999999946709, -131.7500000000000284 ) ) ;
#27061=CARTESIAN_POINT ( 'NONE',  ( -3.464101615137725076, 5.999999999999979572, -178.0863248654052313 ) ) ;
#27062=ORIENTED_EDGE ( 'NONE', *, *, #10445, .F. ) ;
#27063=CARTESIAN_POINT ( 'NONE',  ( -3.175426480542816066, -5.500000000000057732, -59.37500000000005684 ) ) ;
#27065=CARTESIAN_POINT ( 'NONE',  ( 3.175426480543072749, -5.500000000000105693, -60.62500000000000000 ) ) ;
#27069=DIRECTION ( 'NONE',  ( 1.000000000000000000, -5.551115123125773458E-17, -1.260129944081490338E-35 ) ) ;
#27072=CARTESIAN_POINT ( 'NONE',  ( -6.000000000000007105, -1.607695154586655129, -49.34668783648707091 ) ) ;
#27073=ORIENTED_EDGE ( 'NONE', *, *, #1587, .T. ) ;
#27077=CARTESIAN_POINT ( 'NONE',  ( -4.763139720814407951, 2.749999999999946709, -146.7500000000000568 ) ) ;
#27078=CARTESIAN_POINT ( 'NONE',  ( 5.412658773652712085, -3.125000000000086153, -48.06698729810781856 ) ) ;
#27081=CARTESIAN_POINT ( 'NONE',  ( 3.608439182435180470, -6.249999999999997335, -145.6919872981078470 ) ) ;
#27082=EDGE_CURVE ( 'NONE', #8702, #567, #29547, .T. ) ;
#27083=CARTESIAN_POINT ( 'NONE',  ( -4.763139720814407951, -2.750000000000016431, -74.50000000000001421 ) ) ;
#27085=CARTESIAN_POINT ( 'NONE',  ( 2.775557561562891351E-14, -6.250000000000061284, -95.68301270189222407 ) ) ;
#27086=CARTESIAN_POINT ( 'NONE',  ( -2.693961096941767774, -10.67153403684355339, -19.62422301979501782 ) ) ;
#27088=FACE_OUTER_BOUND ( 'NONE', #20120, .T. ) ;
#27089=CARTESIAN_POINT ( 'NONE',  ( 0.000000000000000000, -5.999999999999991118, -86.53867513459483973 ) ) ;
#27090=EDGE_CURVE ( 'NONE', #23148, #5313, #11634, .T. ) ;
#27093=CARTESIAN_POINT ( 'NONE',  ( -3.175426480542816066, -5.500000000000057732, -158.3750000000000284 ) ) ;
#27095=CARTESIAN_POINT ( 'NONE',  ( 6.350852961086080661, -9.614813431917819062E-14, -148.8750000000000284 ) ) ;
#27096=CARTESIAN_POINT ( 'NONE',  ( -5.999999999999919176, 1.607695154586804565, -48.90331216351300725 ) ) ;
#27097=CARTESIAN_POINT ( 'NONE',  ( -6.350852961085760029, -1.281975124255709124E-13, -89.62500000000001421 ) ) ;
#27100=CARTESIAN_POINT ( 'NONE',  ( -3.175426480542816510, -5.500000000000057732, -83.37500000000004263 ) ) ;
#27102=CARTESIAN_POINT ( 'NONE',  ( 5.196152422706629359, -2.999999999999988898, -120.2113248654052029 ) ) ;
#27105=DIRECTION ( 'NONE',  ( 1.000000000000000000, -5.551115123125773458E-17, -1.260129944081490338E-35 ) ) ;
#27106=CARTESIAN_POINT ( 'NONE',  ( 0.000000000000000000, -5.999999999999991118, -165.4613248654052029 ) ) ;
#27108=CARTESIAN_POINT ( 'NONE',  ( 3.464101615137852974, 5.999999999999884537, -174.4136751345948255 ) ) ;
#27113=ORIENTED_EDGE ( 'NONE', *, *, #424, .T. ) ;
#27115=CARTESIAN_POINT ( 'NONE',  ( 6.350852961086080661, -9.614813431917819062E-14, -96.37499999999997158 ) ) ;
#27116=CARTESIAN_POINT ( 'NONE',  ( 6.000000000000000888, 1.743066579297358182E-13, -71.16367513459481131 ) ) ;
#27117=CARTESIAN_POINT ( 'NONE',  ( 2.775557561562891351E-14, 6.250000000000033751, -111.4330127018922099 ) ) ;
#27119=ORIENTED_EDGE ( 'NONE', *, *, #21156, .F. ) ;
#27120=DIRECTION ( 'NONE',  ( 1.000000000000000000, -5.551115123125773458E-17, -1.260129944081490338E-35 ) ) ;
#27121=CARTESIAN_POINT ( 'NONE',  ( -5.999999999999919176, 1.607695154586804565, -62.98066243270261566 ) ) ;
#27122=CARTESIAN_POINT ( 'NONE',  ( 5.412658773652739619, 3.124999999999988898, -51.68301270189223828 ) ) ;
#27123=ORIENTED_EDGE ( 'NONE', *, *, #9151, .T. ) ;
#27127=CARTESIAN_POINT ( 'NONE',  ( 5.196152422706629359, -2.999999999999988898, -119.2886751345948397 ) ) ;
#27129=CARTESIAN_POINT ( 'NONE',  ( 3.464101615137757051, -5.999999999999979572, -166.8363248654051745 ) ) ;
#27131=CARTESIAN_POINT ( 'NONE',  ( 4.763139720814407951, -2.749999999999988454, -173.0000000000000568 ) ) ;
#27134=CARTESIAN_POINT ( 'NONE',  ( 3.608439182435180470, 6.249999999999982236, -159.5580127018922667 ) ) ;
#27135=DIRECTION ( 'NONE',  ( -7.147005652999508048E-36, 5.642372883946980038E-36, 1.000000000000000000 ) ) ;
#27136=CARTESIAN_POINT ( 'NONE',  ( 4.763139720814407951, -2.749999999999988454, -107.0000000000000426 ) ) ;
#27138=CARTESIAN_POINT ( 'NONE',  ( -4.763139720814407951, -2.750000000000016431, -104.5000000000000426 ) ) ;
#27141=CARTESIAN_POINT ( 'NONE',  ( -5.196152422706573404, -3.000000000000002665, -84.71132486540523132 ) ) ;
#27142=ORIENTED_EDGE ( 'NONE', *, *, #3123, .F. ) ;
#27144=DIRECTION ( 'NONE',  ( -7.147005652999508048E-36, 5.642372883946980038E-36, 1.000000000000000000 ) ) ;
#27146=CARTESIAN_POINT ( 'NONE',  ( 0.000000000000000000, -5.999999999999991118, -133.9613248654052313 ) ) ;
#27148=CARTESIAN_POINT ( 'NONE',  ( -2.775557561562891351E-14, -5.500000000000115463, -158.2500000000000000 ) ) ;
#27149=CARTESIAN_POINT ( 'NONE',  ( 5.412658773652739619, 3.124999999999988898, -80.81698729810781856 ) ) ;
#27153=ORIENTED_EDGE ( 'NONE', *, *, #6435, .F. ) ;
#27157=CARTESIAN_POINT ( 'NONE',  ( -3.175426480542816510, -5.500000000000057732, -119.3750000000000284 ) ) ;
#27159=CARTESIAN_POINT ( 'NONE',  ( -3.608439182435115633, 6.249999999999965361, -138.3080127018922951 ) ) ;
#27160=CARTESIAN_POINT ( 'NONE',  ( 5.999999999999999112, 2.951592740943527306E-14, -161.1636751345949108 ) ) ;
#27161=CARTESIAN_POINT ( 'NONE',  ( 2.775557561562891351E-14, -6.250000000000061284, -126.3169872981078043 ) ) ;
#27163=CARTESIAN_POINT ( 'NONE',  ( 0.000000000000000000, 5.499999999999991118, -174.0000000000000568 ) ) ;
#27168=CARTESIAN_POINT ( 'NONE',  ( -5.999999999999963585, -1.487416814333745711E-14, -117.8363248654052313 ) ) ;
#27169=CARTESIAN_POINT ( 'NONE',  ( -5.999999999999963585, -1.487416814333745711E-14, -55.41367513459483973 ) ) ;
#27172=CARTESIAN_POINT ( 'NONE',  ( -5.412658773652684552, -3.125000000000099920, -68.06698729810783277 ) ) ;
#27173=CARTESIAN_POINT ( 'NONE',  ( 5.412658773652712085, -3.125000000000086153, -52.56698729810782567 ) ) ;
#27174=LINE ( 'NONE', #6145, #19004 ) ;
#27177=CARTESIAN_POINT ( 'NONE',  ( 3.464101615137852974, 5.999999999999884537, -74.83632486540521711 ) ) ;
#27179=CARTESIAN_POINT ( 'NONE',  ( -2.775557561562891351E-14, -5.500000000000115463, -132.7500000000000284 ) ) ;
#27180=CARTESIAN_POINT ( 'NONE',  ( 3.464101615137852974, 5.999999999999884537, -50.83632486540523132 ) ) ;
#27182=CARTESIAN_POINT ( 'NONE',  ( 5.999999999999999112, 2.951592740943527306E-14, -158.1636751345948539 ) ) ;
#27183=CARTESIAN_POINT ( 'NONE',  ( -3.464101615137725076, 5.999999999999979572, -119.5863248654052313 ) ) ;
#27186=ORIENTED_EDGE ( 'NONE', *, *, #28246, .T. ) ;
#27190=CARTESIAN_POINT ( 'NONE',  ( -7.216878364870328078, 0.000000000000000000, -117.6919872981078470 ) ) ;
#27191=CARTESIAN_POINT ( 'NONE',  ( -3.464101615137757051, -5.999999999999979572, -173.6636751345947687 ) ) ;
#27194=LINE ( 'NONE', #8940, #266 ) ;
#27196=CIRCLE ( 'NONE', #14096, 4.000000000000003553 ) ;
#27198=CARTESIAN_POINT ( 'NONE',  ( -4.763139720814407951, -2.750000000000016431, -53.49999999999999289 ) ) ;
#27200=CARTESIAN_POINT ( 'NONE',  ( 5.196152422706629359, 3.000000000000002665, -120.5386751345948255 ) ) ;
#27201=CARTESIAN_POINT ( 'NONE',  ( 6.000000000000000888, -1.859271017917181981E-14, -79.58632486540520290 ) ) ;
#27202=CARTESIAN_POINT ( 'NONE',  ( 3.608439182435180470, -6.249999999999997335, -77.55801270189225249 ) ) ;
#27205=DIRECTION ( 'NONE',  ( 1.000000000000000000, -5.551115123125773458E-17, -1.260129944081490338E-35 ) ) ;
#27206=( NAMED_UNIT ( * ) PLANE_ANGLE_UNIT ( ) SI_UNIT ( $, .RADIAN. ) );
#27209=DIRECTION ( 'NONE',  ( 1.000000000000000000, -5.551115123125773458E-17, -1.260129944081490338E-35 ) ) ;
#27211=CARTESIAN_POINT ( 'NONE',  ( -6.350852961085760029, -1.281975124255709124E-13, -134.6250000000000284 ) ) ;
#27212=DIRECTION ( 'NONE',  ( -7.147005652999508048E-36, 5.642372883946980038E-36, 1.000000000000000000 ) ) ;
#27213=VERTEX_POINT ( 'NONE', #2619 ) ;
#27214=CARTESIAN_POINT ( 'NONE',  ( 0.000000000000000000, 5.499999999999991118, -63.00000000000000000 ) ) ;
#27215=DIRECTION ( 'NONE',  ( 1.000000000000000000, -5.551115123125773458E-17, -1.260129944081490338E-35 ) ) ;
#27217=ORIENTED_EDGE ( 'NONE', *, *, #25761, .T. ) ;
#27220=DIRECTION ( 'NONE',  ( 1.000000000000000000, -5.551115123125773458E-17, -1.260129944081490338E-35 ) ) ;
#27221=EDGE_CURVE ( 'NONE', #25740, #1154, #3060, .T. ) ;
#27222=DIRECTION ( 'NONE',  ( -7.147005652999508048E-36, 5.642372883946980038E-36, 1.000000000000000000 ) ) ;
#27224=ORIENTED_EDGE ( 'NONE', *, *, #29154, .T. ) ;
#27227=ORIENTED_EDGE ( 'NONE', *, *, #6164, .F. ) ;
#27228=VECTOR ( 'NONE', #6650, 1000.000000000000000 ) ;
#27229=CARTESIAN_POINT ( 'NONE',  ( -4.763139720814407951, 2.749999999999946709, -142.2500000000000000 ) ) ;
#27233=CARTESIAN_POINT ( 'NONE',  ( -3.175426480542816510, -5.500000000000057732, -72.87500000000000000 ) ) ;
#27235=CARTESIAN_POINT ( 'NONE',  ( -3.608439182435052128, -6.250000000000110134, -95.80801270189220986 ) ) ;
#27240=CARTESIAN_POINT ( 'NONE',  ( 5.196152422706629359, -2.999999999999988898, -86.28867513459481131 ) ) ;
#27242=CARTESIAN_POINT ( 'NONE',  ( -3.175426480542816066, -5.500000000000057732, -156.8750000000000284 ) ) ;
#27243=CARTESIAN_POINT ( 'NONE',  ( -5.999999999999963585, -1.487416814333745711E-14, -117.8363248654052313 ) ) ;
#27246=CARTESIAN_POINT ( 'NONE',  ( 0.000000000000000000, 5.499999999999991118, -85.50000000000001421 ) ) ;
#27247=DIRECTION ( 'NONE',  ( -7.147005652999508048E-36, 5.642372883946980038E-36, 1.000000000000000000 ) ) ;
#27248=CARTESIAN_POINT ( 'NONE',  ( -3.175426480542816510, -5.500000000000057732, -72.87500000000000000 ) ) ;
#27252=EDGE_CURVE ( 'NONE', #27478, #20611, #23534, .T. ) ;
#27253=CARTESIAN_POINT ( 'NONE',  ( 6.000000000000000888, 5.577813053751546416E-15, -165.0863248654052029 ) ) ;
#27255=FACE_OUTER_BOUND ( 'NONE', #14216, .T. ) ;
#27258=CARTESIAN_POINT ( 'NONE',  ( -3.464101615137757051, -5.999999999999979572, -172.1636751345947687 ) ) ;
#27261=CARTESIAN_POINT ( 'NONE',  ( -5.630955349224697315, 2.071796769723730058, -179.9999999999999432 ) ) ;
#27264=CARTESIAN_POINT ( 'NONE',  ( 4.763139720814407951, 2.750000000000002665, -99.25000000000000000 ) ) ;
#27265=CARTESIAN_POINT ( 'NONE',  ( -6.000000000000007105, -1.607695154586655129, -89.84668783648706381 ) ) ;
#27266=CARTESIAN_POINT ( 'NONE',  ( -3.608439182435115633, 6.249999999999965361, -115.8080127018922383 ) ) ;
#27270=CARTESIAN_POINT ( 'NONE',  ( -5.999999999999963585, 1.780251999655701777E-13, -51.83632486540522422 ) ) ;
#27271=CARTESIAN_POINT ( 'NONE',  ( 5.412658773652739619, 3.124999999999988898, -48.68301270189223828 ) ) ;
#27274=CARTESIAN_POINT ( 'NONE',  ( -5.196152422706601826, 2.999999999999975131, -135.9613248654052313 ) ) ;
#27275=CARTESIAN_POINT ( 'NONE',  ( 3.175426480543072749, 5.499999999999865885, -160.6250000000000284 ) ) ;
#27279=CARTESIAN_POINT ( 'NONE',  ( 4.763139720814407951, -2.749999999999988454, -109.9999999999999858 ) ) ;
#27281=CARTESIAN_POINT ( 'NONE',  ( -3.175426480542816510, -5.500000000000057732, -104.3750000000000142 ) ) ;
#27282=CARTESIAN_POINT ( 'NONE',  ( 5.999999999999999112, 2.951592740943527306E-14, -152.1636751345948255 ) ) ;
#27283=( NAMED_UNIT ( * ) PLANE_ANGLE_UNIT ( ) SI_UNIT ( $, .RADIAN. ) );
#27284=CARTESIAN_POINT ( 'NONE',  ( 3.464101615137852974, 5.999999999999884537, -145.3363248654052029 ) ) ;
#27292=VECTOR ( 'NONE', #18787, 1000.000000000000000 ) ;
#27293=CARTESIAN_POINT ( 'NONE',  ( 5.412658773652712085, -3.125000000000086153, -88.56698729810786119 ) ) ;
#27294=CARTESIAN_POINT ( 'NONE',  ( 0.000000000000000000, -5.999999999999991118, -103.0386751345948539 ) ) ;
#27298=CARTESIAN_POINT ( 'NONE',  ( 6.000000000000000888, 1.743066579297358182E-13, -75.08632486540521711 ) ) ;
#27300=CARTESIAN_POINT ( 'NONE',  ( -3.175426480542816510, -5.500000000000057732, -150.8750000000000000 ) ) ;
#27302=VERTEX_POINT ( 'NONE', #6133 ) ;
#27304=CARTESIAN_POINT ( 'NONE',  ( 4.763139720814407951, 2.750000000000002665, -121.7500000000000284 ) ) ;
#27305=( BOUNDED_CURVE ( )  B_SPLINE_CURVE ( 2, ( #26188, #7315, #12263, #14558, #16722, #21604, #14422, #9929, #23758 ),
 .UNSPECIFIED., .F., .F. ) 
 B_SPLINE_CURVE_WITH_KNOTS ( ( 3, 2, 2, 2, 3 ),
 ( 0.9083333333333333259, 0.9092592592592592116, 0.9111111111111110938, 0.9129629629629629761, 0.9138888888888888618 ),
 .UNSPECIFIED. ) 
 CURVE ( )  GEOMETRIC_REPRESENTATION_ITEM ( )  RATIONAL_B_SPLINE_CURVE ( ( 0.9330127018922194093, 0.9330127018922194093, 1.000000000000000000, 0.8660254037844388186, 1.000000000000000000, 0.8660254037844388186, 1.000000000000000000, 0.9330127018922234061, 0.9330127018922194093 ) ) 
 REPRESENTATION_ITEM ( '' )  );
#27306=CARTESIAN_POINT ( 'NONE',  ( -7.216878364870328078, 0.000000000000000000, -141.0580127018922099 ) ) ;
#27308=CARTESIAN_POINT ( 'NONE',  ( 0.000000000000000000, 5.999999999999977796, -57.28867513459484684 ) ) ;
#27309=CARTESIAN_POINT ( 'NONE',  ( -3.608439182435115633, 6.249999999999965361, -122.4419872981077901 ) ) ;
#27310=CARTESIAN_POINT ( 'NONE',  ( 2.775557561562891351E-14, 6.250000000000033751, -175.0669872981078186 ) ) ;
#27312=CARTESIAN_POINT ( 'NONE',  ( -3.175426480542816510, -5.500000000000057732, -173.3750000000000284 ) ) ;
#27315=ORIENTED_EDGE ( 'NONE', *, *, #3715, .F. ) ;
#27319=CARTESIAN_POINT ( 'NONE',  ( -5.999999999999919176, 1.607695154586804565, -89.98066243270262987 ) ) ;
#27320=AXIS2_PLACEMENT_3D ( 'NONE', #19304, #28492, #5137 ) ;
#27324=CARTESIAN_POINT ( 'NONE',  ( 2.775557561562891351E-14, -6.250000000000061284, -70.81698729810781856 ) ) ;
#27325=CARTESIAN_POINT ( 'NONE',  ( 2.775557561562891351E-14, 6.250000000000033751, -55.06698729810782567 ) ) ;
#27327=CARTESIAN_POINT ( 'NONE',  ( 6.350852961086080661, -9.614813431917819062E-14, -52.87500000000002132 ) ) ;
#27329=CARTESIAN_POINT ( 'NONE',  ( 6.000000000000000888, 7.762456499804234384E-14, -123.0863248654052313 ) ) ;
#27330=CARTESIAN_POINT ( 'NONE',  ( -3.175426480542816510, -5.500000000000057732, -132.8750000000000284 ) ) ;
#27332=ORIENTED_EDGE ( 'NONE', *, *, #8544, .F. ) ;
#27333=CARTESIAN_POINT ( 'NONE',  ( -5.196152422706601826, 2.999999999999975131, -157.5386751345948539 ) ) ;
#27334=EDGE_CURVE ( 'NONE', #1801, #25259, #28435, .T. ) ;
#27340=LINE ( 'NONE', #25036, #15987 ) ;
#27341=CARTESIAN_POINT ( 'NONE',  ( 6.000000000000001776, 5.345404176511898156E-15, -178.5863248654052313 ) ) ;
#27342=CARTESIAN_POINT ( 'NONE',  ( 3.608439182435180470, 6.249999999999982236, -118.1919872981078328 ) ) ;
#27343=CARTESIAN_POINT ( 'NONE',  ( -5.999999999999964473, 9.063946212346262433E-15, -173.9136751345948255 ) ) ;
#27344=ADVANCED_FACE ( 'NONE', ( #26845 ), #6292, .T. ) ;
#27346=ORIENTED_EDGE ( 'NONE', *, *, #19615, .T. ) ;
#27350=ORIENTED_EDGE ( 'NONE', *, *, #13203, .F. ) ;
#27351=CARTESIAN_POINT ( 'NONE',  ( 3.175426480543072749, -5.500000000000105693, -48.62500000000000711 ) ) ;
#27353=CARTESIAN_POINT ( 'NONE',  ( -5.196152422706601826, 2.999999999999975131, -61.53867513459482552 ) ) ;
#27354=CARTESIAN_POINT ( 'NONE',  ( -7.216878364870328078, 0.000000000000000000, -67.55801270189226670 ) ) ;
#27357=CARTESIAN_POINT ( 'NONE',  ( -5.196152422706601826, 2.999999999999975131, -177.0386751345948255 ) ) ;
#27358=CARTESIAN_POINT ( 'NONE',  ( 6.000000000000052403, -1.607695154586662678, -66.73066243270258724 ) ) ;
#27359=CARTESIAN_POINT ( 'NONE',  ( 3.175426480543072749, 5.499999999999865885, -133.6250000000000284 ) ) ;
#27360=CARTESIAN_POINT ( 'NONE',  ( 3.608439182435180470, 6.249999999999982236, -147.5580127018922667 ) ) ;
#27361=DIRECTION ( 'NONE',  ( -7.147005652999508048E-36, 5.642372883946980038E-36, 1.000000000000000000 ) ) ;
#27362=ORIENTED_EDGE ( 'NONE', *, *, #25536, .F. ) ;
#27364=CARTESIAN_POINT ( 'NONE',  ( 4.763139720814407951, 2.750000000000002665, -66.25000000000002842 ) ) ;
#27366=DIRECTION ( 'NONE',  ( -7.147005652999508048E-36, 5.642372883946980038E-36, 1.000000000000000000 ) ) ;
#27367=EDGE_CURVE ( 'NONE', #15456, #3196, #15266, .T. ) ;
#27368=CARTESIAN_POINT ( 'NONE',  ( 0.000000000000000000, -5.999999999999991118, -163.0386751345947971 ) ) ;
#27369=ORIENTED_EDGE ( 'NONE', *, *, #27367, .T. ) ;
#27372=CARTESIAN_POINT ( 'NONE',  ( 0.000000000000000000, 0.000000000000000000, 0.000000000000000000 ) ) ;
#27374=VERTEX_POINT ( 'NONE', #10965 ) ;
#27378=CARTESIAN_POINT ( 'NONE',  ( -2.775557561562891351E-14, -5.500000000000115463, -146.2500000000000000 ) ) ;
#27382=CARTESIAN_POINT ( 'NONE',  ( -3.175426480542816510, 5.499999999999865885, -70.37500000000004263 ) ) ;
#27385=LINE ( 'NONE', #15468, #17737 ) ;
#27386=FACE_OUTER_BOUND ( 'NONE', #15607, .T. ) ;
#27389=CARTESIAN_POINT ( 'NONE',  ( 0.000000000000000000, 5.499999999999991118, -156.0000000000000284 ) ) ;
#27391=CARTESIAN_POINT ( 'NONE',  ( 0.000000000000000000, 5.999999999999977796, -49.21132486540524553 ) ) ;
#27392=CARTESIAN_POINT ( 'NONE',  ( 3.175426480543072749, 5.499999999999865885, -87.12500000000000000 ) ) ;
#27394=CARTESIAN_POINT ( 'NONE',  ( -4.763139720814407951, 2.749999999999946709, -70.25000000000002842 ) ) ;
#27397=CARTESIAN_POINT ( 'NONE',  ( -3.464101615137757051, -5.999999999999979572, -120.5863248654052313 ) ) ;
#27399=CARTESIAN_POINT ( 'NONE',  ( 3.464101615137852974, 5.999999999999884537, -106.3363248654052313 ) ) ;
#27400=CARTESIAN_POINT ( 'NONE',  ( -3.464101615137757051, -5.999999999999979572, -175.1636751345947403 ) ) ;
#27403=CARTESIAN_POINT ( 'NONE',  ( -5.196152422706601826, 2.999999999999975131, -94.53867513459479710 ) ) ;
#27405=FACE_OUTER_BOUND ( 'NONE', #8909, .T. ) ;
#27406=ORIENTED_EDGE ( 'NONE', *, *, #19031, .T. ) ;
#27410=CARTESIAN_POINT ( 'NONE',  ( 6.000000000000000888, 1.743066579297358182E-13, -55.58632486540519579 ) ) ;
#27411=ORIENTED_EDGE ( 'NONE', *, *, #14553, .T. ) ;
#27413=CARTESIAN_POINT ( 'NONE',  ( -4.763139720814407951, 2.749999999999946709, -94.25000000000000000 ) ) ;
#27415=CARTESIAN_POINT ( 'NONE',  ( -3.608439182435115633, 6.249999999999965361, -111.3080127018922241 ) ) ;
#27417=CARTESIAN_POINT ( 'NONE',  ( -3.464101615137757051, -5.999999999999979572, -124.1636751345947829 ) ) ;
#27420=EDGE_CURVE ( 'NONE', #14683, #15286, #21033, .T. ) ;
#27421=CARTESIAN_POINT ( 'NONE',  ( 7.216878364870455975, -6.409875621278545621E-14, -53.30801270189225960 ) ) ;
#27422=ORIENTED_EDGE ( 'NONE', *, *, #1371, .T. ) ;
#27423=CARTESIAN_POINT ( 'NONE',  ( 5.999999999999988454, 1.607695154586737729, -153.5966878364870638 ) ) ;
#27427=CARTESIAN_POINT ( 'NONE',  ( -3.175426480542816510, -5.500000000000057732, -164.3750000000000568 ) ) ;
#27431=CARTESIAN_POINT ( 'NONE',  ( 5.196152422706629359, -2.999999999999988898, -165.7886751345948255 ) ) ;
#27432=CARTESIAN_POINT ( 'NONE',  ( -6.350852961085760029, -1.281975124255709124E-13, -100.1250000000000568 ) ) ;
#27433=CARTESIAN_POINT ( 'NONE',  ( 5.196152422706629359, -2.999999999999988898, -81.78867513459486815 ) ) ;
#27439=CARTESIAN_POINT ( 'NONE',  ( -3.608439182435052128, -6.250000000000110134, -90.44198729810783277 ) ) ;
#27441=CARTESIAN_POINT ( 'NONE',  ( 6.000000000000052403, -1.607695154586662678, -96.73066243270258724 ) ) ;
#27442=ORIENTED_EDGE ( 'NONE', *, *, #9360, .T. ) ;
#27443=CARTESIAN_POINT ( 'NONE',  ( 6.000000000000000888, 1.743066579297358182E-13, -65.16367513459479710 ) ) ;
#27445=ORIENTED_EDGE ( 'NONE', *, *, #14978, .F. ) ;
#27447=CARTESIAN_POINT ( 'NONE',  ( -3.175426480542816510, 5.499999999999865885, -118.3750000000000142 ) ) ;
#27448=CARTESIAN_POINT ( 'NONE',  ( 2.775557561562891351E-14, -6.250000000000061284, -140.6830127018922099 ) ) ;
#27451=CARTESIAN_POINT ( 'NONE',  ( 5.412658773652712085, -3.125000000000086153, -126.0669872981078328 ) ) ;
#27452=CARTESIAN_POINT ( 'NONE',  ( -5.412658773652684552, -3.125000000000099920, -177.5669872981078186 ) ) ;
#27453=FACE_OUTER_BOUND ( 'NONE', #11649, .T. ) ;
#27456=CARTESIAN_POINT ( 'NONE',  ( 5.999999999999949374, 1.607695154586804565, -148.5193375672974696 ) ) ;
#27461=CARTESIAN_POINT ( 'NONE',  ( -3.608439182435115633, 6.249999999999965361, -72.94198729810781856 ) ) ;
#27462=CARTESIAN_POINT ( 'NONE',  ( 2.775557561562891351E-14, 6.250000000000033751, -59.56698729810783277 ) ) ;
#27464=CARTESIAN_POINT ( 'NONE',  ( 0.000000000000000000, 5.499999999999991118, -48.00000000000004263 ) ) ;
#27466=CARTESIAN_POINT ( 'NONE',  ( 0.000000000000000000, -5.999999999999991118, -47.53867513459481131 ) ) ;
#27468=EDGE_CURVE ( 'NONE', #2682, #10812, #25486, .T. ) ;
#27469=CARTESIAN_POINT ( 'NONE',  ( -4.763139720814407951, -2.750000000000016431, -119.5000000000000568 ) ) ;
#27471=CARTESIAN_POINT ( 'NONE',  ( 6.000000000000000888, 7.762456499804234384E-14, -138.6636751345948255 ) ) ;
#27474=CARTESIAN_POINT ( 'NONE',  ( -5.999999999999962697, 3.323446944526963891E-14, -157.4136751345948539 ) ) ;
#27476=CARTESIAN_POINT ( 'NONE',  ( -5.999999999999963585, -1.487416814333745711E-14, -96.83632486540520290 ) ) ;
#27478=VERTEX_POINT ( 'NONE', #18788 ) ;
#27482=CARTESIAN_POINT ( 'NONE',  ( -3.608439182435052128, -6.250000000000110134, -115.9419872981078328 ) ) ;
#27500=CARTESIAN_POINT ( 'NONE',  ( 6.000000000000000888, -1.607695154586752384, -79.65331216351296462 ) ) ;
#27501=CARTESIAN_POINT ( 'NONE',  ( -5.412658773652684552, -3.125000000000099920, -68.93301270189222407 ) ) ;
#27502=AXIS2_PLACEMENT_3D ( 'NONE', #13884, #9381, #4149 ) ;
#27506=CARTESIAN_POINT ( 'NONE',  ( -5.999999999999968026, -1.607695154586722186, -155.8466878364870070 ) ) ;
#27508=CARTESIAN_POINT ( 'NONE',  ( 3.175426480543072749, -5.500000000000105693, -122.1250000000000426 ) ) ;
#27511=ORIENTED_EDGE ( 'NONE', *, *, #9293, .T. ) ;
#27513=CARTESIAN_POINT ( 'NONE',  ( 3.175426480543072749, -5.500000000000105693, -65.12500000000001421 ) ) ;
#27514=CARTESIAN_POINT ( 'NONE',  ( -5.999999999999956479, -1.607695154586745057, -154.3466878364870638 ) ) ;
#27515=CARTESIAN_POINT ( 'NONE',  ( 6.000000000000052403, -1.607695154586662678, -76.65331216351299304 ) ) ;
#27516=CARTESIAN_POINT ( 'NONE',  ( -3.464101615137757051, -5.999999999999979572, -163.1636751345947687 ) ) ;
#27526=CARTESIAN_POINT ( 'NONE',  ( -2.775557561562891351E-14, -5.500000000000115463, -140.2500000000000000 ) ) ;
#27529=CARTESIAN_POINT ( 'NONE',  ( 3.175426480543072749, 5.499999999999865885, -73.62500000000005684 ) ) ;
#27532=DIRECTION ( 'NONE',  ( -7.147005652999508048E-36, 5.642372883946980038E-36, 1.000000000000000000 ) ) ;
#27534=CARTESIAN_POINT ( 'NONE',  ( -1.965048709171653751, -10.82948053518398979, -19.31713205297533520 ) ) ;
#27535=CARTESIAN_POINT ( 'NONE',  ( 6.000000000000000888, 1.743066579297358182E-13, -83.16367513459481131 ) ) ;
#27540=CARTESIAN_POINT ( 'NONE',  ( -6.350852961085760029, -1.281975124255709124E-13, -149.6250000000000284 ) ) ;
#27543=CARTESIAN_POINT ( 'NONE',  ( -2.775557561562891351E-14, -5.500000000000115463, -86.25000000000004263 ) ) ;
#27544=CYLINDRICAL_SURFACE ( 'NONE', #18925, 6.000000000000000888 ) ;
#27545=CARTESIAN_POINT ( 'NONE',  ( 4.763139720814407951, -2.749999999999988454, -75.50000000000001421 ) ) ;
#27553=CARTESIAN_POINT ( 'NONE',  ( 5.999999999999949374, 1.607695154586804565, -139.5193375672973843 ) ) ;
#27554=ORIENTED_EDGE ( 'NONE', *, *, #11968, .T. ) ;
#27556=AXIS2_PLACEMENT_3D ( 'NONE', #12525, #29049, #17422 ) ;
#27557=CYLINDRICAL_SURFACE ( 'NONE', #1342, 6.000000000000000888 ) ;
#27558=ORIENTED_EDGE ( 'NONE', *, *, #9647, .F. ) ;
#27559=ORIENTED_EDGE ( 'NONE', *, *, #28511, .T. ) ;
#27560=ORIENTED_EDGE ( 'NONE', *, *, #11975, .T. ) ;
#27561=CARTESIAN_POINT ( 'NONE',  ( -6.350852961085760029, -1.281975124255709124E-13, -97.12500000000004263 ) ) ;
#27562=CARTESIAN_POINT ( 'NONE',  ( 0.000000000000000000, 5.999999999999977796, -96.28867513459482552 ) ) ;
#27563=ADVANCED_FACE ( 'NONE', ( #12626 ), #5062, .T. ) ;
#27564=CARTESIAN_POINT ( 'NONE',  ( 2.775557561562891351E-14, 6.250000000000033751, -109.9330127018922667 ) ) ;
#27565=ORIENTED_EDGE ( 'NONE', *, *, #19693, .T. ) ;
#27568=CARTESIAN_POINT ( 'NONE',  ( -4.763139720814407951, 2.749999999999946709, -164.7500000000000000 ) ) ;
#27569=CARTESIAN_POINT ( 'NONE',  ( -5.999999999999963585, -1.487416814333745711E-14, -106.4136751345948113 ) ) ;
#27571=CARTESIAN_POINT ( 'NONE',  ( 3.464101615137852974, 5.999999999999884537, -160.3363248654052313 ) ) ;
#27572=( BOUNDED_CURVE ( )  B_SPLINE_CURVE ( 2, ( #20270, #24856, #20565, #16148, #8893, #4419, #1812, #9042, #27443 ),
 .UNSPECIFIED., .F., .T. ) 
 B_SPLINE_CURVE_WITH_KNOTS ( ( 3, 2, 2, 2, 3 ),
 ( 0.8583333333333332815, 0.8592592592592592782, 0.8611111111111111605, 0.8629629629629629317, 0.8638888888888889284 ),
 .UNSPECIFIED. ) 
 CURVE ( )  GEOMETRIC_REPRESENTATION_ITEM ( )  RATIONAL_B_SPLINE_CURVE ( ( 0.9330127018922194093, 0.9330127018922154125, 1.000000000000000000, 0.8660254037844388186, 1.000000000000000000, 0.8660254037844388186, 1.000000000000000000, 0.9330127018922154125, 0.9330127018922194093 ) ) 
 REPRESENTATION_ITEM ( '' )  );
#27574=CARTESIAN_POINT ( 'NONE',  ( 4.763139720814407951, 2.750000000000002665, -162.2500000000000000 ) ) ;
#27576=CARTESIAN_POINT ( 'NONE',  ( 4.763139720814407951, 2.750000000000002665, -111.2500000000000142 ) ) ;
#27578=DIRECTION ( 'NONE',  ( 1.000000000000000000, -5.551115123125774074E-17, 0.000000000000000000 ) ) ;
#27579=CARTESIAN_POINT ( 'NONE',  ( 0.000000000000000000, 5.499999999999991118, -100.5000000000000284 ) ) ;
#27580=COLOUR_RGB ( '', 0.72549020, 0.75294118, 0.79215686) ;
#27582=CARTESIAN_POINT ( 'NONE',  ( -6.000000000000000888, 1.067854986875958443E-15, 7.560779664488942560E-35 ) ) ;
#27587=CARTESIAN_POINT ( 'NONE',  ( 6.000000000000000888, -1.859271017917181981E-14, -130.5863248654052313 ) ) ;
#27590=ORIENTED_EDGE ( 'NONE', *, *, #17989, .T. ) ;
#27591=CARTESIAN_POINT ( 'NONE',  ( 6.000000000000000888, -3.330669073875464691E-16, -7.560779664488942560E-35 ) ) ;
#27594=CARTESIAN_POINT ( 'NONE',  ( -5.412658773652739619, 3.124999999999975131, -86.31698729810783277 ) ) ;
#27596=CARTESIAN_POINT ( 'NONE',  ( -1.581364418632495106, 10.89278420593271157, -30.80148057605384793 ) ) ;
#27599=ORIENTED_EDGE ( 'NONE', *, *, #2389, .F. ) ;
#27600=CARTESIAN_POINT ( 'NONE',  ( 6.350852961086080661, -9.614813431917819062E-14, -121.8750000000000426 ) ) ;
#27603=EDGE_CURVE ( 'NONE', #20871, #12019, #15766, .T. ) ;
#27604=CARTESIAN_POINT ( 'NONE',  ( 3.608439182435180470, -6.249999999999997335, -131.5580127018922383 ) ) ;
#27607=CARTESIAN_POINT ( 'NONE',  ( -3.608439182435052128, -6.250000000000110134, -123.4419872981078043 ) ) ;
#27608=CARTESIAN_POINT ( 'NONE',  ( 3.608439182435180470, -6.249999999999997335, -178.6919872981078470 ) ) ;
#27611=ORIENTED_EDGE ( 'NONE', *, *, #13141, .T. ) ;
#27616=( BOUNDED_CURVE ( )  B_SPLINE_CURVE ( 2, ( #26889, #13133, #15269, #17726, #3394, #12821, #20169, #22163, #24598 ),
 .UNSPECIFIED., .F., .T. ) 
 B_SPLINE_CURVE_WITH_KNOTS ( ( 3, 2, 2, 2, 3 ),
 ( 0.9361111111111111160, 0.9370370370370370017, 0.9388888888888888840, 0.9407407407407407662, 0.9416666666666666519 ),
 .UNSPECIFIED. ) 
 CURVE ( )  GEOMETRIC_REPRESENTATION_ITEM ( )  RATIONAL_B_SPLINE_CURVE ( ( 0.9330127018922194093, 0.9330127018922194093, 1.000000000000000000, 0.8660254037844388186, 1.000000000000000000, 0.8660254037844388186, 1.000000000000000000, 0.9330127018922234061, 0.9330127018922194093 ) ) 
 REPRESENTATION_ITEM ( '' )  );
#27617=CARTESIAN_POINT ( 'NONE',  ( 5.196152422706629359, -2.999999999999988898, -150.2113248654052313 ) ) ;
#27619=CARTESIAN_POINT ( 'NONE',  ( 5.412658773652712085, -3.125000000000086153, -72.06698729810784698 ) ) ;
#27620=CARTESIAN_POINT ( 'NONE',  ( 7.216878364870455975, -6.409875621278545621E-14, -58.44198729810781856 ) ) ;
#27621=CARTESIAN_POINT ( 'NONE',  ( 0.000000000000000000, -5.999999999999991118, -170.5386751345947971 ) ) ;
#27622=CARTESIAN_POINT ( 'NONE',  ( 4.763139720814407951, -2.749999999999988454, -48.49999999999998579 ) ) ;
#27624=CARTESIAN_POINT ( 'NONE',  ( 4.763139720814407951, -2.749999999999988454, -122.0000000000000000 ) ) ;
#27627=EDGE_LOOP ( 'NONE', ( #13802, #13045, #9043, #13912 ) ) ;
#27629=( BOUNDED_CURVE ( )  B_SPLINE_CURVE ( 2, ( #4119, #13240, #22880, #22583, #27308, #19052, #25465, #18591, #23648 ),
 .UNSPECIFIED., .F., .F. ) 
 B_SPLINE_CURVE_WITH_KNOTS ( ( 3, 2, 2, 2, 3 ),
 ( 0.9194444444444445086, 0.9203703703703703942, 0.9222222222222222765, 0.9240740740740740478, 0.9249999999999999334 ),
 .UNSPECIFIED. ) 
 CURVE ( )  GEOMETRIC_REPRESENTATION_ITEM ( )  RATIONAL_B_SPLINE_CURVE ( ( 0.9330127018922194093, 0.9330127018922234061, 1.000000000000000000, 0.8660254037844388186, 1.000000000000000000, 0.8660254037844388186, 1.000000000000000000, 0.9330127018922234061, 0.9330127018922194093 ) ) 
 REPRESENTATION_ITEM ( '' )  );
#27635=CARTESIAN_POINT ( 'NONE',  ( 6.000000000000000000, 2.951592740943527306E-14, -164.1636751345948824 ) ) ;
#27637=EDGE_CURVE ( 'NONE', #11496, #21299, #6662, .T. ) ;
#27638=CARTESIAN_POINT ( 'NONE',  ( 2.775557561562891351E-14, 6.250000000000033751, -116.5669872981078328 ) ) ;
#27639=CARTESIAN_POINT ( 'NONE',  ( -5.999999999999963585, 1.780251999655701777E-13, -107.9136751345948397 ) ) ;
#27645=ADVANCED_FACE ( 'NONE', ( #26560 ), #3062, .T. ) ;
#27646=CARTESIAN_POINT ( 'NONE',  ( -5.412658773652739619, 3.124999999999975131, -50.31698729810785409 ) ) ;
#27647=VERTEX_POINT ( 'NONE', #28859 ) ;
#27648=CARTESIAN_POINT ( 'NONE',  ( -5.412658773652684552, -3.125000000000099920, -144.5669872981077901 ) ) ;
#27655=CARTESIAN_POINT ( 'NONE',  ( 5.412658773652739619, 3.124999999999988898, -63.68301270189225249 ) ) ;
#27659=CARTESIAN_POINT ( 'NONE',  ( -5.999999999999963585, -1.487416814333745711E-14, -170.3363248654052313 ) ) ;
#27662=CARTESIAN_POINT ( 'NONE',  ( -3.175426480542816066, -5.500000000000057732, -123.8749999999999858 ) ) ;
#27663=DIRECTION ( 'NONE',  ( 1.000000000000000000, -5.551115123125773458E-17, -1.260129944081490338E-35 ) ) ;
#27664=CARTESIAN_POINT ( 'NONE',  ( -3.608439182435115633, 6.249999999999965361, -144.3080127018922383 ) ) ;
#27668=CARTESIAN_POINT ( 'NONE',  ( -3.175426480542816066, -5.500000000000057732, -54.87500000000003553 ) ) ;
#27669=CYLINDRICAL_SURFACE ( 'NONE', #6063, 4.000000000000004441 ) ;
#27670=CARTESIAN_POINT ( 'NONE',  ( -3.464101615137725076, 5.999999999999979572, -172.0863248654052029 ) ) ;
#27671=( BOUNDED_CURVE ( )  B_SPLINE_CURVE ( 2, ( #21348, #9673, #19063, #26092, #5032, #433, #9822, #19198, #28527 ),
 .UNSPECIFIED., .F., .T. ) 
 B_SPLINE_CURVE_WITH_KNOTS ( ( 3, 2, 2, 2, 3 ),
 ( 0.2194444444444444420, 0.2203703703703703276, 0.2222222222222222099, 0.2240740740740740922, 0.2249999999999999778 ),
 .UNSPECIFIED. ) 
 CURVE ( )  GEOMETRIC_REPRESENTATION_ITEM ( )  RATIONAL_B_SPLINE_CURVE ( ( 0.9330127018922194093, 0.9330127018922194093, 1.000000000000000000, 0.8660254037844388186, 1.000000000000000000, 0.8660254037844388186, 1.000000000000000000, 0.9330127018922234061, 0.9330127018922194093 ) ) 
 REPRESENTATION_ITEM ( '' )  );
#27672=CARTESIAN_POINT ( 'NONE',  ( -5.999999999999962697, 3.323446944526963891E-14, -163.4136751345948539 ) ) ;
#27676=EDGE_CURVE ( 'NONE', #22801, #10034, #19087, .T. ) ;
#27677=CARTESIAN_POINT ( 'NONE',  ( -6.000000000000000888, 1.067854986875958443E-15, 7.560779664488942560E-35 ) ) ;
#27681=CARTESIAN_POINT ( 'NONE',  ( 3.175426480543072749, -5.500000000000105693, -140.1250000000000000 ) ) ;
#27684=CARTESIAN_POINT ( 'NONE',  ( 3.175426480543072749, 5.499999999999865885, -66.12500000000002842 ) ) ;
#27686=CARTESIAN_POINT ( 'NONE',  ( -5.999999999999963585, -1.487416814333745711E-14, -139.4136751345948255 ) ) ;
#27687=CARTESIAN_POINT ( 'NONE',  ( 0.000000000000000000, 0.000000000000000000, 0.000000000000000000 ) ) ;
#27691=CARTESIAN_POINT ( 'NONE',  ( 3.175426480543072749, 5.499999999999865885, -151.6250000000000284 ) ) ;
#27693=CARTESIAN_POINT ( 'NONE',  ( -2.775557561562891351E-14, -5.500000000000115463, -141.7500000000000568 ) ) ;
#27694=CARTESIAN_POINT ( 'NONE',  ( -5.412658773652739619, 3.124999999999975131, -163.6830127018922383 ) ) ;
#27696=CARTESIAN_POINT ( 'NONE',  ( 6.350852961086080661, -9.614813431917819062E-14, -79.87500000000001421 ) ) ;
#27697=CARTESIAN_POINT ( 'NONE',  ( 0.000000000000000000, 0.000000000000000000, 0.000000000000000000 ) ) ;
#27698=CARTESIAN_POINT ( 'NONE',  ( -3.175426480542816510, 5.499999999999865885, -76.37500000000001421 ) ) ;
#27699=CARTESIAN_POINT ( 'NONE',  ( 0.000000000000000000, -5.999999999999991118, -74.53867513459483973 ) ) ;
#27700=VECTOR ( 'NONE', #27247, 1000.000000000000000 ) ;
#27703=CARTESIAN_POINT ( 'NONE',  ( -3.464101615137757051, -5.999999999999979572, -71.66367513459481131 ) ) ;
#27705=AXIS2_PLACEMENT_3D ( 'NONE', #21626, #26355, #5306 ) ;
#27706=CARTESIAN_POINT ( 'NONE',  ( -5.999999999999963585, 8.134310703387671600E-14, -145.4136751345948539 ) ) ;
#27707=EDGE_CURVE ( 'NONE', #25500, #21299, #17997, .T. ) ;
#27709=CARTESIAN_POINT ( 'NONE',  ( -5.999999999999963585, 1.780251999655701777E-13, -83.91367513459482552 ) ) ;
#27714=DIRECTION ( 'NONE',  ( 1.000000000000000000, -5.551115123125773458E-17, -1.260129944081490338E-35 ) ) ;
#27715=ORIENTED_EDGE ( 'NONE', *, *, #873, .F. ) ;
#27718=VECTOR ( 'NONE', #15379, 1000.000000000000000 ) ;
#27719=ORIENTED_EDGE ( 'NONE', *, *, #9291, .F. ) ;
#27720=CARTESIAN_POINT ( 'NONE',  ( -4.763139720814407951, 2.749999999999946709, -92.75000000000000000 ) ) ;
#27721=CARTESIAN_POINT ( 'NONE',  ( -5.412658773652684552, -3.125000000000099920, -103.4330127018922525 ) ) ;
#27723=CYLINDRICAL_SURFACE ( 'NONE', #7853, 6.000000000000000888 ) ;
#27726=CARTESIAN_POINT ( 'NONE',  ( -3.175426480542816510, 5.499999999999865885, -164.8750000000000568 ) ) ;
#27727=CARTESIAN_POINT ( 'NONE',  ( 3.679869817085056116, -10.37177793260014091, -29.75506555745400306 ) ) ;
#27731=CARTESIAN_POINT ( 'NONE',  ( -4.763139720814407951, 2.749999999999946709, -169.2500000000000000 ) ) ;
#27732=CARTESIAN_POINT ( 'NONE',  ( 6.000000000000000000, 2.951592740943527306E-14, -158.1636751345948539 ) ) ;
#27733=CARTESIAN_POINT ( 'NONE',  ( -2.775557561562891351E-14, -5.500000000000115463, -161.2500000000000000 ) ) ;
#27735=CARTESIAN_POINT ( 'NONE',  ( -6.350852961085760029, -1.281975124255709124E-13, -104.6250000000000142 ) ) ;
#27737=CARTESIAN_POINT ( 'NONE',  ( -5.999999999999963585, -1.487416814333745711E-14, -166.4136751345948539 ) ) ;
#27738=CARTESIAN_POINT ( 'NONE',  ( -2.775557561562891351E-14, -5.500000000000115463, -93.75000000000000000 ) ) ;
#27743=CARTESIAN_POINT ( 'NONE',  ( 5.196152422706629359, -2.999999999999988898, -161.2886751345948255 ) ) ;
#27746=EDGE_CURVE ( 'NONE', #25123, #13073, #2363, .T. ) ;
#27747=ORIENTED_EDGE ( 'NONE', *, *, #603, .F. ) ;
#27749=VECTOR ( 'NONE', #29530, 1000.000000000000000 ) ;
#27750=CARTESIAN_POINT ( 'NONE',  ( -7.216878364870328078, 0.000000000000000000, -90.69198729810784698 ) ) ;
#27753=ORIENTED_EDGE ( 'NONE', *, *, #2463, .F. ) ;
#27755=CARTESIAN_POINT ( 'NONE',  ( 6.350852961086080661, -9.614813431917819062E-14, -123.3749999999999858 ) ) ;
#27758=CARTESIAN_POINT ( 'NONE',  ( -5.412658773652684552, -3.125000000000099920, -127.4330127018922241 ) ) ;
#27760=ORIENTED_EDGE ( 'NONE', *, *, #16516, .T. ) ;
#27761=DIRECTION ( 'NONE',  ( 1.000000000000000000, -5.551115123125773458E-17, -1.260129944081490338E-35 ) ) ;
#27762=CARTESIAN_POINT ( 'NONE',  ( 7.216878364870455975, -6.409875621278545621E-14, -166.4419872981078186 ) ) ;
#27763=CARTESIAN_POINT ( 'NONE',  ( 5.412658773652712085, -3.125000000000086153, -178.5669872981078186 ) ) ;
#27769=CARTESIAN_POINT ( 'NONE',  ( -5.196152422706601826, 2.999999999999975131, -54.03867513459481842 ) ) ;
#27770=CARTESIAN_POINT ( 'NONE',  ( 2.308094007029174666, 5.188356418777920531, -180.0000000000000000 ) ) ;
#27771=CARTESIAN_POINT ( 'NONE',  ( 5.196152422706629359, 3.000000000000002665, -137.0386751345948255 ) ) ;
#27772=CARTESIAN_POINT ( 'NONE',  ( -10.00000000000001421, 1.779758311459933302E-15, -43.99152654425658682 ) ) ;
#27773=CARTESIAN_POINT ( 'NONE',  ( 3.608439182435180470, -6.249999999999997335, -73.69198729810783277 ) ) ;
#27774=CARTESIAN_POINT ( 'NONE',  ( 7.216878364870455975, -6.409875621278545621E-14, -62.94198729810783277 ) ) ;
#27776=CARTESIAN_POINT ( 'NONE',  ( -4.763139720814407951, -2.750000000000016431, -47.49999999999998579 ) ) ;
#27778=CARTESIAN_POINT ( 'NONE',  ( 6.000000000000052403, -1.607695154586662678, -153.1533121635129646 ) ) ;
#27779=CARTESIAN_POINT ( 'NONE',  ( 3.464101615137852974, 5.999999999999884537, -159.4136751345947687 ) ) ;
#27780=CARTESIAN_POINT ( 'NONE',  ( -4.763139720814407951, -2.750000000000016431, -124.0000000000000000 ) ) ;
#27781=CARTESIAN_POINT ( 'NONE',  ( 6.000000000000000888, -1.859271017917181981E-14, -166.5863248654052029 ) ) ;
#27784=CARTESIAN_POINT ( 'NONE',  ( -5.196152422706601826, 2.999999999999975131, -105.0386751345948539 ) ) ;
#27786=VERTEX_POINT ( 'NONE', #17686 ) ;
#27791=CARTESIAN_POINT ( 'NONE',  ( 7.216878364870455975, -6.409875621278545621E-14, -107.9419872981078043 ) ) ;
#27794=VECTOR ( 'NONE', #3571, 1000.000000000000000 ) ;
#27795=ORIENTED_EDGE ( 'NONE', *, *, #4385, .T. ) ;
#27799=CARTESIAN_POINT ( 'NONE',  ( 5.412658773652739619, 3.124999999999988898, -140.8169872981078186 ) ) ;
#27802=VECTOR ( 'NONE', #14256, 1000.000000000000000 ) ;
#27806=CARTESIAN_POINT ( 'NONE',  ( 2.775557561562891351E-14, -6.250000000000061284, -70.18301270189225249 ) ) ;
#27809=CARTESIAN_POINT ( 'NONE',  ( 3.464101615137757051, -5.999999999999979572, -69.91367513459481131 ) ) ;
#27811=CARTESIAN_POINT ( 'NONE',  ( 5.999999999999993783, 1.607695154586726627, -165.5966878364870354 ) ) ;
#27816=( BOUNDED_CURVE ( )  B_SPLINE_CURVE ( 2, ( #16573, #7008, #2263, #21011, #25429, #26048, #28340, #11668, #30357 ),
 .UNSPECIFIED., .F., .F. ) 
 B_SPLINE_CURVE_WITH_KNOTS ( ( 3, 2, 2, 2, 3 ),
 ( 0.6527777777777777901, 0.6537037037037036757, 0.6555555555555555580, 0.6574074074074074403, 0.6583333333333333259 ),
 .UNSPECIFIED. ) 
 CURVE ( )  GEOMETRIC_REPRESENTATION_ITEM ( )  RATIONAL_B_SPLINE_CURVE ( ( 0.9330127018922194093, 0.9330127018922194093, 1.000000000000000000, 0.8660254037844388186, 1.000000000000000000, 0.8660254037844388186, 1.000000000000000000, 0.9330127018922194093, 0.9330127018922194093 ) ) 
 REPRESENTATION_ITEM ( '' )  );
#27817=CARTESIAN_POINT ( 'NONE',  ( 0.000000000000000000, 5.499999999999991118, -123.0000000000000000 ) ) ;
#27820=CARTESIAN_POINT ( 'NONE',  ( 7.216878364870455975, -6.409875621278545621E-14, -146.3080127018922667 ) ) ;
#27823=CARTESIAN_POINT ( 'NONE',  ( 4.763139720814407951, -2.749999999999988454, -53.00000000000004974 ) ) ;
#27824=EDGE_CURVE ( 'NONE', #3063, #6123, #5461, .T. ) ;
#27825=CARTESIAN_POINT ( 'NONE',  ( -5.999999999999919176, 1.607695154586804565, -171.9033121635130215 ) ) ;
#27826=EDGE_CURVE ( 'NONE', #14122, #17549, #1678, .T. ) ;
#27827=CARTESIAN_POINT ( 'NONE',  ( 0.000000000000000000, -5.999999999999991118, -163.9613248654052597 ) ) ;
#27836=CARTESIAN_POINT ( 'NONE',  ( -3.175426480542816510, -5.500000000000057732, -135.8750000000000284 ) ) ;
#27839=ORIENTED_EDGE ( 'NONE', *, *, #13022, .T. ) ;
#27840=CARTESIAN_POINT ( 'NONE',  ( -2.775557561562891351E-14, -5.500000000000115463, -68.25000000000002842 ) ) ;
#27844=EDGE_CURVE ( 'NONE', #4876, #4112, #4282, .T. ) ;
#27849=CARTESIAN_POINT ( 'NONE',  ( -3.175426480542816066, 5.499999999999865885, -146.8750000000000284 ) ) ;
#27850=DIRECTION ( 'NONE',  ( 1.000000000000000000, -5.551115123125774074E-17, 0.000000000000000000 ) ) ;
#27851=CARTESIAN_POINT ( 'NONE',  ( 3.175426480543072749, 5.499999999999865885, -139.6250000000000000 ) ) ;
#27852=CARTESIAN_POINT ( 'NONE',  ( 2.775557561562891351E-14, 6.250000000000033751, -162.4330127018922667 ) ) ;
#27853=CARTESIAN_POINT ( 'NONE',  ( 0.000000000000000000, 0.000000000000000000, 0.000000000000000000 ) ) ;
#27854=CARTESIAN_POINT ( 'NONE',  ( 4.763139720814407951, 2.750000000000002665, -81.25000000000004263 ) ) ;
#27855=ADVANCED_FACE ( 'NONE', ( #27453 ), #8755, .F. ) ;
#27856=CARTESIAN_POINT ( 'NONE',  ( 4.763139720814407951, 2.750000000000002665, -72.25000000000004263 ) ) ;
#27858=ADVANCED_FACE ( 'NONE', ( #16160 ), #23755, .T. ) ;
#27859=CARTESIAN_POINT ( 'NONE',  ( -6.000000000000007105, -1.607695154586655129, -120.7693375672974412 ) ) ;
#27872=CARTESIAN_POINT ( 'NONE',  ( 3.464101615137757051, -5.999999999999979572, -108.9136751345947971 ) ) ;
#27874=CARTESIAN_POINT ( 'NONE',  ( 3.175426480543072749, -5.500000000000105693, -153.6250000000000568 ) ) ;
#27879=CARTESIAN_POINT ( 'NONE',  ( 3.175426480543072749, -5.500000000000105693, -86.12500000000000000 ) ) ;
#27880=CARTESIAN_POINT ( 'NONE',  ( -5.412658773652739619, 3.124999999999975131, -106.6830127018922383 ) ) ;
#27881=CARTESIAN_POINT ( 'NONE',  ( 4.767949350811410802, 9.915884935901873476, -28.66271918150854958 ) ) ;
#27884=CARTESIAN_POINT ( 'NONE',  ( 3.608439182435180470, -6.249999999999997335, -47.55801270189223828 ) ) ;
#27887=CARTESIAN_POINT ( 'NONE',  ( -3.175426480542816066, -5.500000000000057732, -168.8750000000000568 ) ) ;
#27888=CARTESIAN_POINT ( 'NONE',  ( -6.000000000000000888, 1.067854986875958443E-15, 7.560779664488942560E-35 ) ) ;
#27889=CARTESIAN_POINT ( 'NONE',  ( 4.763139720814407951, 2.750000000000002665, -165.2500000000000000 ) ) ;
#27891=CARTESIAN_POINT ( 'NONE',  ( -3.175426480542816066, 5.499999999999865885, -104.8750000000000142 ) ) ;
#27892=CARTESIAN_POINT ( 'NONE',  ( 6.000000000000000888, 7.762456499804234384E-14, -122.1636751345948397 ) ) ;
#27894=CARTESIAN_POINT ( 'NONE',  ( -4.763139720814407951, 2.749999999999946709, -100.2500000000000000 ) ) ;
#27896=ORIENTED_EDGE ( 'NONE', *, *, #12275, .T. ) ;
#27899=CARTESIAN_POINT ( 'NONE',  ( 6.000000000000014211, -1.607695154586730180, -161.2306624327026157 ) ) ;
#27901=CARTESIAN_POINT ( 'NONE',  ( 3.464101615137757051, -5.999999999999979572, -85.83632486540520290 ) ) ;
#27904=ORIENTED_EDGE ( 'NONE', *, *, #19615, .F. ) ;
#27907=CARTESIAN_POINT ( 'NONE',  ( 3.175426480543072749, -5.500000000000105693, -111.6249999999999858 ) ) ;
#27908=AXIS2_PLACEMENT_3D ( 'NONE', #3461, #24967, #1161 ) ;
#27910=CARTESIAN_POINT ( 'NONE',  ( -3.608439182435052128, -6.250000000000110134, -133.3080127018922667 ) ) ;
#27914=CARTESIAN_POINT ( 'NONE',  ( -3.608439182435052128, -6.250000000000110134, -169.9419872981078470 ) ) ;
#27915=CARTESIAN_POINT ( 'NONE',  ( -3.608439182435115633, 6.249999999999965361, -174.9419872981078470 ) ) ;
#27919=CARTESIAN_POINT ( 'NONE',  ( -5.999999999999957367, 1.607695154586737507, -163.4806624327025588 ) ) ;
#27921=CARTESIAN_POINT ( 'NONE',  ( -6.000000000000000888, 1.067854986875958443E-15, 7.560779664488942560E-35 ) ) ;
#27922=CARTESIAN_POINT ( 'NONE',  ( -5.196152422706601826, 2.999999999999975131, -132.9613248654052313 ) ) ;
#27925=CARTESIAN_POINT ( 'NONE',  ( -5.412658773652739619, 3.124999999999975131, -75.81698729810781856 ) ) ;
#27926=CARTESIAN_POINT ( 'NONE',  ( -5.412658773652684552, -3.125000000000099920, -59.06698729810783277 ) ) ;
#27927=CARTESIAN_POINT ( 'NONE',  ( 2.775557561562891351E-14, -6.250000000000061284, -181.1830127018922383 ) ) ;
#27929=DIRECTION ( 'NONE',  ( 1.000000000000000000, -5.551115123125773458E-17, -1.260129944081490338E-35 ) ) ;
#27930=CARTESIAN_POINT ( 'NONE',  ( 5.196152422706629359, -2.999999999999988898, -53.28867513459483973 ) ) ;
#27931=CARTESIAN_POINT ( 'NONE',  ( -3.175426480542816510, -5.500000000000057732, -117.8750000000000142 ) ) ;
#27941=CARTESIAN_POINT ( 'NONE',  ( -3.608439182435052128, -6.250000000000110134, -108.4419872981078043 ) ) ;
#27943=( BOUNDED_CURVE ( )  B_SPLINE_CURVE ( 2, ( #1663, #22111, #1191, #19951, #24854, #24545, #11057, #17981, #12924 ),
 .UNSPECIFIED., .F., .T. ) 
 B_SPLINE_CURVE_WITH_KNOTS ( ( 3, 2, 2, 2, 3 ),
 ( 0.6138888888888889284, 0.6148148148148148140, 0.6166666666666666963, 0.6185185185185184675, 0.6194444444444444642 ),
 .UNSPECIFIED. ) 
 CURVE ( )  GEOMETRIC_REPRESENTATION_ITEM ( )  RATIONAL_B_SPLINE_CURVE ( ( 0.9330127018922194093, 0.9330127018922234061, 1.000000000000000000, 0.8660254037844388186, 1.000000000000000000, 0.8660254037844388186, 1.000000000000000000, 0.9330127018922154125, 0.9330127018922194093 ) ) 
 REPRESENTATION_ITEM ( '' )  );
#27948=CARTESIAN_POINT ( 'NONE',  ( -3.608439182435115633, 6.249999999999965361, -135.9419872981077901 ) ) ;
#27950=CARTESIAN_POINT ( 'NONE',  ( 6.000000000000000888, -1.607695154586752384, -93.15331216351302146 ) ) ;
#27951=VECTOR ( 'NONE', #10001, 1000.000000000000000 ) ;
#27955=CARTESIAN_POINT ( 'NONE',  ( 5.412658773652712085, -3.125000000000086153, -60.93301270189221697 ) ) ;
#27959=DIRECTION ( 'NONE',  ( 1.000000000000000000, -5.551115123125773458E-17, -1.260129944081490338E-35 ) ) ;
#27960=CARTESIAN_POINT ( 'NONE',  ( 0.000000000000000000, 5.999999999999977796, -165.2886751345948824 ) ) ;
#27964=CARTESIAN_POINT ( 'NONE',  ( 5.196152422706629359, -2.999999999999988898, -94.71132486540523132 ) ) ;
#27965=CARTESIAN_POINT ( 'NONE',  ( 0.000000000000000000, 5.499999999999991118, -127.5000000000000568 ) ) ;
#27967=CARTESIAN_POINT ( 'NONE',  ( 2.775557561562891351E-14, 6.250000000000033751, -145.9330127018922383 ) ) ;
#27969=CARTESIAN_POINT ( 'NONE',  ( 3.464101615137852974, 5.999999999999884537, -142.9136751345948255 ) ) ;
#27970=ORIENTED_EDGE ( 'NONE', *, *, #21101, .F. ) ;
#27971=CARTESIAN_POINT ( 'NONE',  ( 6.350852961086080661, -9.614813431917819062E-14, -51.37500000000002132 ) ) ;
#27972=CARTESIAN_POINT ( 'NONE',  ( 0.000000000000000000, 0.000000000000000000, 0.000000000000000000 ) ) ;
#27974=CARTESIAN_POINT ( 'NONE',  ( 3.464101615137757051, -5.999999999999979572, -178.8363248654052029 ) ) ;
#27975=ORIENTED_EDGE ( 'NONE', *, *, #17846, .T. ) ;
#27978=CARTESIAN_POINT ( 'NONE',  ( 2.775557561562891351E-14, -6.250000000000061284, -100.8169872981078470 ) ) ;
#27985=CARTESIAN_POINT ( 'NONE',  ( 3.175426480543072749, 5.499999999999865885, -141.1250000000000000 ) ) ;
#27987=VERTEX_POINT ( 'NONE', #19593 ) ;
#27988=ORIENTED_EDGE ( 'NONE', *, *, #5104, .T. ) ;
#27989=CARTESIAN_POINT ( 'NONE',  ( -2.775557561562891351E-14, -5.500000000000115463, -65.25000000000002842 ) ) ;
#27992=CARTESIAN_POINT ( 'NONE',  ( -5.999999999999956479, -1.607695154586745057, -124.3466878364870496 ) ) ;
#27993=CARTESIAN_POINT ( 'NONE',  ( 2.775557561562891351E-14, 6.250000000000033751, -88.93301270189223828 ) ) ;
#27994=EDGE_CURVE ( 'NONE', #18584, #4636, #8630, .T. ) ;
#27996=CARTESIAN_POINT ( 'NONE',  ( -5.999999999999956479, -1.607695154586745057, -113.8466878364870496 ) ) ;
#27999=CARTESIAN_POINT ( 'NONE',  ( 6.000000000000000888, 1.743066579297358182E-13, -86.16367513459481131 ) ) ;
#28001=CARTESIAN_POINT ( 'NONE',  ( -4.763139720814407951, -2.750000000000016431, -149.5000000000000284 ) ) ;
#28003=CARTESIAN_POINT ( 'NONE',  ( -4.763139720814407951, -2.750000000000016431, -140.5000000000000000 ) ) ;
#28004=VECTOR ( 'NONE', #9504, 1000.000000000000000 ) ;
#28005=CARTESIAN_POINT ( 'NONE',  ( 2.775557561562891351E-14, 6.250000000000033751, -159.4330127018922383 ) ) ;
#28007=CARTESIAN_POINT ( 'NONE',  ( -3.175426480542816066, -5.500000000000057732, -77.37500000000001421 ) ) ;
#28008=CARTESIAN_POINT ( 'NONE',  ( 3.175426480543072749, 5.499999999999865885, -67.62500000000002842 ) ) ;
#28009=CARTESIAN_POINT ( 'NONE',  ( -5.999999999999956479, -1.607695154586745057, -88.34668783648706381 ) ) ;
#28016=DIRECTION ( 'NONE',  ( -7.147005652999508048E-36, 5.642372883946980038E-36, 1.000000000000000000 ) ) ;
#28018=CARTESIAN_POINT ( 'NONE',  ( -5.999999999999963585, 1.780251999655701777E-13, -98.33632486540520290 ) ) ;
#28019=VERTEX_POINT ( 'NONE', #537 ) ;
#28024=CARTESIAN_POINT ( 'NONE',  ( 10.00000000000001421, -5.551115123125781716E-16, -44.99152654425658682 ) ) ;
#28027=ORIENTED_EDGE ( 'NONE', *, *, #25800, .F. ) ;
#28028=CARTESIAN_POINT ( 'NONE',  ( 3.175426480543072749, -5.500000000000105693, -89.12500000000000000 ) ) ;
#28030=( BOUNDED_CURVE ( )  B_SPLINE_CURVE ( 2, ( #26944, #10867, #11016, #20223, #8689, #27399, #6364, #24950, #29573 ),
 .UNSPECIFIED., .F., .T. ) 
 B_SPLINE_CURVE_WITH_KNOTS ( ( 3, 2, 2, 2, 3 ),
 ( 0.4416666666666666519, 0.4425925925925925375, 0.4444444444444444198, 0.4462962962962963021, 0.4472222222222221877 ),
 .UNSPECIFIED. ) 
 CURVE ( )  GEOMETRIC_REPRESENTATION_ITEM ( )  RATIONAL_B_SPLINE_CURVE ( ( 0.9330127018922194093, 0.9330127018922194093, 1.000000000000000000, 0.8660254037844388186, 1.000000000000000000, 0.8660254037844388186, 1.000000000000000000, 0.9330127018922234061, 0.9330127018922194093 ) ) 
 REPRESENTATION_ITEM ( '' )  );
#28031=CARTESIAN_POINT ( 'NONE',  ( 2.775557561562891351E-14, -6.250000000000061284, -110.6830127018922383 ) ) ;
#28034=CARTESIAN_POINT ( 'NONE',  ( 5.681812044562478903, 9.420575401947205663, -23.03339967402430943 ) ) ;
#28037=CARTESIAN_POINT ( 'NONE',  ( -5.196152422706573404, -3.000000000000002665, -63.71132486540520290 ) ) ;
#28039=CARTESIAN_POINT ( 'NONE',  ( 0.000000000000000000, 0.000000000000000000, 0.000000000000000000 ) ) ;
#28040=CARTESIAN_POINT ( 'NONE',  ( -4.763139720814407951, -2.750000000000016431, -175.0000000000000568 ) ) ;
#28043=CARTESIAN_POINT ( 'NONE',  ( 3.175426480543072749, 5.499999999999865885, -153.1250000000000284 ) ) ;
#28045=VECTOR ( 'NONE', #5070, 1000.000000000000000 ) ;
#28047=CARTESIAN_POINT ( 'NONE',  ( -5.999999999999919176, 1.607695154586804565, -86.98066243270262987 ) ) ;
#28048=CARTESIAN_POINT ( 'NONE',  ( 0.000000000000000000, 5.499999999999991118, -94.50000000000002842 ) ) ;
#28050=ORIENTED_EDGE ( 'NONE', *, *, #22793, .T. ) ;
#28055=CARTESIAN_POINT ( 'NONE',  ( 6.000000000000000888, 1.743066579297358182E-13, -50.16367513459482552 ) ) ;
#28056=VERTEX_POINT ( 'NONE', #29080 ) ;
#28057=CARTESIAN_POINT ( 'NONE',  ( 6.000000000000000888, -3.330669073875464691E-16, -7.560779664488942560E-35 ) ) ;
#28058=FACE_OUTER_BOUND ( 'NONE', #7810, .T. ) ;
#28060=EDGE_CURVE ( 'NONE', #9068, #29150, #23187, .T. ) ;
#28063=CARTESIAN_POINT ( 'NONE',  ( -6.000000000000007105, -1.607695154586655129, -53.26933756729743408 ) ) ;
#28065=ORIENTED_EDGE ( 'NONE', *, *, #7994, .T. ) ;
#28066=CARTESIAN_POINT ( 'NONE',  ( 4.763139720814407951, 2.750000000000002665, -111.2500000000000142 ) ) ;
#28068=ADVANCED_FACE ( 'NONE', ( #12259 ), #8192, .T. ) ;
#28069=CARTESIAN_POINT ( 'NONE',  ( 2.775557561562891351E-14, -6.250000000000061284, -133.1830127018922667 ) ) ;
#28072=CARTESIAN_POINT ( 'NONE',  ( -3.608439182435115633, 6.249999999999965361, -167.4419872981078186 ) ) ;
#28077=DIRECTION ( 'NONE',  ( 1.000000000000000000, -5.551115123125773458E-17, -1.260129944081490338E-35 ) ) ;
#28078=CARTESIAN_POINT ( 'NONE',  ( 3.175426480543072749, 5.499999999999865885, -180.1250000000000000 ) ) ;
#28080=CARTESIAN_POINT ( 'NONE',  ( -3.608439182435052128, -6.250000000000110134, -179.8080127018922383 ) ) ;
#28081=CARTESIAN_POINT ( 'NONE',  ( 3.464101615137757051, -5.999999999999979572, -111.3363248654051745 ) ) ;
#28084=CARTESIAN_POINT ( 'NONE',  ( 6.350852961086080661, -9.614813431917819062E-14, -123.3749999999999858 ) ) ;
#28085=LINE ( 'NONE', #23804, #6812 ) ;
#28086=CARTESIAN_POINT ( 'NONE',  ( -5.196152422706601826, 2.999999999999975131, -153.9613248654052597 ) ) ;
#28091=DIRECTION ( 'NONE',  ( 1.000000000000000000, -5.551115123125773458E-17, -1.260129944081490338E-35 ) ) ;
#28095=CARTESIAN_POINT ( 'NONE',  ( 5.412658773652712085, -3.125000000000086153, -108.0669872981078186 ) ) ;
#28099=EDGE_CURVE ( 'NONE', #26686, #2098, #18372, .T. ) ;
#28100=CARTESIAN_POINT ( 'NONE',  ( -5.999999999999962697, 3.323446944526963891E-14, -148.4136751345948255 ) ) ;
#28102=ORIENTED_EDGE ( 'NONE', *, *, #25346, .F. ) ;
#28105=VERTEX_POINT ( 'NONE', #29853 ) ;
#28106=CARTESIAN_POINT ( 'NONE',  ( -7.216878364870328078, 0.000000000000000000, -141.6919872981078186 ) ) ;
#28109=CARTESIAN_POINT ( 'NONE',  ( -3.464101615137757051, -5.999999999999979572, -93.58632486540523132 ) ) ;
#28111=CARTESIAN_POINT ( 'NONE',  ( -6.000000000000000888, 1.067854986875958443E-15, 7.560779664488942560E-35 ) ) ;
#28113=CARTESIAN_POINT ( 'NONE',  ( 7.216878364870455975, -6.409875621278545621E-14, -59.30801270189222407 ) ) ;
#28114=DIRECTION ( 'NONE',  ( 1.000000000000000000, -5.551115123125773458E-17, -1.260129944081490338E-35 ) ) ;
#28118=CARTESIAN_POINT ( 'NONE',  ( -6.000000000000007105, -1.607695154586655129, -161.2693375672974696 ) ) ;
#28119=CARTESIAN_POINT ( 'NONE',  ( -5.999999999999982236, -1.607695154586700426, -146.8466878364870070 ) ) ;
#28122=CARTESIAN_POINT ( 'NONE',  ( 3.464101615137852974, 5.999999999999884537, -113.8363248654051745 ) ) ;
#28124=( BOUNDED_CURVE ( )  B_SPLINE_CURVE ( 2, ( #19385, #2921, #23543, #7683, #2482, #17091, #9862, #19236, #29014 ),
 .UNSPECIFIED., .F., .F. ) 
 B_SPLINE_CURVE_WITH_KNOTS ( ( 3, 2, 2, 2, 3 ),
 ( 0.6916666666666666519, 0.6925925925925926485, 0.6944444444444444198, 0.6962962962962963021, 0.6972222222222221877 ),
 .UNSPECIFIED. ) 
 CURVE ( )  GEOMETRIC_REPRESENTATION_ITEM ( )  RATIONAL_B_SPLINE_CURVE ( ( 0.9330127018922194093, 0.9330127018922154125, 1.000000000000000000, 0.8660254037844388186, 1.000000000000000000, 0.8660254037844388186, 1.000000000000000000, 0.9330127018922234061, 0.9330127018922194093 ) ) 
 REPRESENTATION_ITEM ( '' )  );
#28127=VERTEX_POINT ( 'NONE', #27686 ) ;
#28128=CARTESIAN_POINT ( 'NONE',  ( 6.350852961086080661, -9.614813431917819062E-14, -54.37500000000003553 ) ) ;
#28131=CARTESIAN_POINT ( 'NONE',  ( -6.000000000000007105, -1.607695154586655129, -179.2693375672974696 ) ) ;
#28132=ORIENTED_EDGE ( 'NONE', *, *, #28158, .T. ) ;
#28136=CARTESIAN_POINT ( 'NONE',  ( 5.412658773652739619, 3.124999999999988898, -104.8169872981078470 ) ) ;
#28137=DIRECTION ( 'NONE',  ( 1.000000000000000000, -5.551115123125773458E-17, -1.260129944081490338E-35 ) ) ;
#28140=ORIENTED_EDGE ( 'NONE', *, *, #565, .T. ) ;
#28142=CARTESIAN_POINT ( 'NONE',  ( -4.763139720814407951, 2.749999999999946709, -136.2499999999999716 ) ) ;
#28144=CARTESIAN_POINT ( 'NONE',  ( 3.175426480543072749, -5.500000000000105693, -65.12500000000001421 ) ) ;
#28145=CARTESIAN_POINT ( 'NONE',  ( -5.999999999999963585, 8.134310703387671600E-14, -115.4136751345948397 ) ) ;
#28146=CARTESIAN_POINT ( 'NONE',  ( 3.464101615137852974, 5.999999999999884537, -66.41367513459485394 ) ) ;
#28147=CARTESIAN_POINT ( 'NONE',  ( 2.775557561562891351E-14, -6.250000000000061284, -83.68301270189226670 ) ) ;
#28148=CARTESIAN_POINT ( 'NONE',  ( -5.999999999999956479, -1.607695154586745057, -101.2693375672974554 ) ) ;
#28153=CARTESIAN_POINT ( 'NONE',  ( -4.763139720814407951, -2.750000000000016431, -148.0000000000000284 ) ) ;
#28155=CARTESIAN_POINT ( 'NONE',  ( 2.775557561562891351E-14, 6.250000000000033751, -160.9330127018922667 ) ) ;
#28156=CARTESIAN_POINT ( 'NONE',  ( 5.196152422706629359, -2.999999999999988898, -148.7113248654052313 ) ) ;
#28157=CARTESIAN_POINT ( 'NONE',  ( 5.999999999999949374, 1.607695154586804565, -49.51933756729743408 ) ) ;
#28158=EDGE_CURVE ( 'NONE', #19684, #6844, #12341, .T. ) ;
#28159=CARTESIAN_POINT ( 'NONE',  ( -2.775557561562891351E-14, -5.500000000000115463, -77.25000000000004263 ) ) ;
#28161=CARTESIAN_POINT ( 'NONE',  ( -2.775557561562891351E-14, -5.500000000000115463, -62.25000000000002842 ) ) ;
#28165=CARTESIAN_POINT ( 'NONE',  ( -6.000000000000060396, -1.607695154586566089, -144.7693375672974696 ) ) ;
#28168=CARTESIAN_POINT ( 'NONE',  ( -5.999999999999962697, 3.323446944526963260E-14, -147.8363248654052313 ) ) ;
#28170=CARTESIAN_POINT ( 'NONE',  ( -5.196152422706573404, -3.000000000000002665, -98.21132486540523132 ) ) ;
#28176=ORIENTED_EDGE ( 'NONE', *, *, #11751, .T. ) ;
#28178=ORIENTED_EDGE ( 'NONE', *, *, #9401, .T. ) ;
#28179=CARTESIAN_POINT ( 'NONE',  ( 4.763139720814407951, 2.750000000000002665, -90.25000000000005684 ) ) ;
#28181=EDGE_LOOP ( 'NONE', ( #9954, #2433, #14610, #1343 ) ) ;
#28184=CARTESIAN_POINT ( 'NONE',  ( 4.763139720814407951, 2.750000000000002665, -165.2500000000000000 ) ) ;
#28186=( NAMED_UNIT ( * ) PLANE_ANGLE_UNIT ( ) SI_UNIT ( $, .RADIAN. ) );
#28187=CARTESIAN_POINT ( 'NONE',  ( -4.763139720814407951, 2.749999999999946709, -172.2500000000000000 ) ) ;
#28189=CARTESIAN_POINT ( 'NONE',  ( -3.175426480542816510, 5.499999999999865885, -152.8749999999999716 ) ) ;
#28193=CARTESIAN_POINT ( 'NONE',  ( -4.763139720814407951, -2.750000000000016431, -100.0000000000000284 ) ) ;
#28196=CARTESIAN_POINT ( 'NONE',  ( 0.000000000000000000, 5.499999999999991118, -154.5000000000000284 ) ) ;
#28197=CARTESIAN_POINT ( 'NONE',  ( -4.763139720814407951, 2.749999999999946709, -86.75000000000000000 ) ) ;
#28200=ORIENTED_EDGE ( 'NONE', *, *, #1608, .T. ) ;
#28205=EDGE_CURVE ( 'NONE', #9697, #3256, #27385, .T. ) ;
#28206=CARTESIAN_POINT ( 'NONE',  ( -3.464101615137757051, -5.999999999999979572, -86.08632486540520290 ) ) ;
#28207=ORIENTED_EDGE ( 'NONE', *, *, #2191, .T. ) ;
#28209=CARTESIAN_POINT ( 'NONE',  ( 0.000000000000000000, 0.000000000000000000, 0.000000000000000000 ) ) ;
#28213=ORIENTED_EDGE ( 'NONE', *, *, #3679, .F. ) ;
#28219=AXIS2_PLACEMENT_3D ( 'NONE', #18089, #17790, #8214 ) ;
#28220=CARTESIAN_POINT ( 'NONE',  ( -3.175426480542816510, 5.499999999999865885, -115.3750000000000000 ) ) ;
#28222=CARTESIAN_POINT ( 'NONE',  ( -5.412658773652739619, 3.124999999999975131, -129.1830127018922667 ) ) ;
#28224=CARTESIAN_POINT ( 'NONE',  ( -5.412658773652739619, 3.124999999999975131, -167.3169872981078470 ) ) ;
#28231=CARTESIAN_POINT ( 'NONE',  ( -4.763139720814407951, -2.750000000000016431, -179.5000000000000000 ) ) ;
#28233=CARTESIAN_POINT ( 'NONE',  ( 2.775557561562891351E-14, -6.250000000000061284, -178.1830127018922383 ) ) ;
#28236=DIRECTION ( 'NONE',  ( -7.147005652999508048E-36, 5.642372883946980038E-36, 1.000000000000000000 ) ) ;
#28237=CARTESIAN_POINT ( 'NONE',  ( -5.999999999999963585, -1.487416814333745711E-14, -122.9136751345948255 ) ) ;
#28238=CARTESIAN_POINT ( 'NONE',  ( 4.763139720814407951, 2.750000000000002665, -111.2500000000000142 ) ) ;
#28241=ORIENTED_EDGE ( 'NONE', *, *, #16101, .F. ) ;
#28246=EDGE_CURVE ( 'NONE', #18017, #28127, #11817, .T. ) ;
#28247=EDGE_CURVE ( 'NONE', #19083, #23968, #11074, .T. ) ;
#28251=DIRECTION ( 'NONE',  ( -7.147005652999508048E-36, 5.642372883946980038E-36, 1.000000000000000000 ) ) ;
#28252=CARTESIAN_POINT ( 'NONE',  ( 5.196152422706629359, -2.999999999999988898, -95.28867513459482552 ) ) ;
#28254=EDGE_LOOP ( 'NONE', ( #9273, #20884, #28684, #20948, #18465 ) ) ;
#28259=CARTESIAN_POINT ( 'NONE',  ( -3.608439182435115633, 6.249999999999965361, -140.4419872981078470 ) ) ;
#28260=FACE_OUTER_BOUND ( 'NONE', #2362, .T. ) ;
#28267=CARTESIAN_POINT ( 'NONE',  ( 6.000000000000052403, -1.607695154586662678, -69.73066243270262987 ) ) ;
#28268=CARTESIAN_POINT ( 'NONE',  ( -5.196152422706601826, 2.999999999999975131, -146.4613248654052029 ) ) ;
#28274=VERTEX_POINT ( 'NONE', #30164 ) ;
#28276=CARTESIAN_POINT ( 'NONE',  ( 6.350852961086080661, -9.614813431917819062E-14, -48.37500000000000711 ) ) ;
#28277=CARTESIAN_POINT ( 'NONE',  ( 6.000000000000000888, 1.743066579297358182E-13, -53.16367513459481131 ) ) ;
#28279=CARTESIAN_POINT ( 'NONE',  ( 0.000000000000000000, 5.999999999999977796, -79.21132486540521711 ) ) ;
#28280=CARTESIAN_POINT ( 'NONE',  ( 5.999999999999999112, 2.951592740943527306E-14, -163.5863248654052313 ) ) ;
#28281=VERTEX_POINT ( 'NONE', #9127 ) ;
#28284=CARTESIAN_POINT ( 'NONE',  ( -3.608439182435115633, 6.249999999999965361, -101.4419872981078328 ) ) ;
#28290=AXIS2_PLACEMENT_3D ( 'NONE', #25105, #26826, #8097 ) ;
#28291=CARTESIAN_POINT ( 'NONE',  ( -4.763139720814407951, -2.750000000000016431, -131.5000000000000000 ) ) ;
#28293=CARTESIAN_POINT ( 'NONE',  ( 6.000000000000000888, 1.743066579297358182E-13, -81.66367513459481131 ) ) ;
#28294=CARTESIAN_POINT ( 'NONE',  ( 0.000000000000000000, 5.499999999999991118, -63.00000000000000000 ) ) ;
#28296=( BOUNDED_CURVE ( )  B_SPLINE_CURVE ( 2, ( #27253, #8057, #7911, #15488, #27106, #5751, #24498, #13032, #24812 ),
 .UNSPECIFIED., .F., .F. ) 
 B_SPLINE_CURVE_WITH_KNOTS ( ( 3, 2, 2, 2, 3 ),
 ( 0.8805555555555555358, 0.8814814814814815325, 0.8833333333333333037, 0.8851851851851851860, 0.8861111111111110716 ),
 .UNSPECIFIED. ) 
 CURVE ( )  GEOMETRIC_REPRESENTATION_ITEM ( )  RATIONAL_B_SPLINE_CURVE ( ( 0.9330127018922194093, 0.9330127018922154125, 1.000000000000000000, 0.8660254037844388186, 1.000000000000000000, 0.8660254037844388186, 1.000000000000000000, 0.9330127018922234061, 0.9330127018922194093 ) ) 
 REPRESENTATION_ITEM ( '' )  );
#28297=CARTESIAN_POINT ( 'NONE',  ( 5.412658773652712085, -3.125000000000086153, -86.43301270189223828 ) ) ;
#28298=LINE ( 'NONE', #659, #2518 ) ;
#28302=CARTESIAN_POINT ( 'NONE',  ( 5.196152422706629359, -2.999999999999988898, -175.7113248654052029 ) ) ;
#28306=( BOUNDED_CURVE ( )  B_SPLINE_CURVE ( 2, ( #24281, #14510, #19694, #5536, #484, #3381, #3228, #17260, #26287 ),
 .UNSPECIFIED., .F., .T. ) 
 B_SPLINE_CURVE_WITH_KNOTS ( ( 3, 2, 2, 2, 3 ),
 ( 0.9694444444444444420, 0.9703703703703703276, 0.9722222222222222099, 0.9740740740740740922, 0.9750000000000000888 ),
 .UNSPECIFIED. ) 
 CURVE ( )  GEOMETRIC_REPRESENTATION_ITEM ( )  RATIONAL_B_SPLINE_CURVE ( ( 0.9330127018922194093, 0.9330127018922194093, 1.000000000000000000, 0.8660254037844388186, 1.000000000000000000, 0.8660254037844388186, 1.000000000000000000, 0.9330127018922154125, 0.9330127018922194093 ) ) 
 REPRESENTATION_ITEM ( '' )  );
#28307=CARTESIAN_POINT ( 'NONE',  ( -6.350852961085760029, -1.281975124255709124E-13, -137.6250000000000568 ) ) ;
#28309=CARTESIAN_POINT ( 'NONE',  ( 7.216878364870455975, -6.409875621278545621E-14, -156.8080127018922667 ) ) ;
#28310=SURFACE_SIDE_STYLE ('',( #9750 ) ) ;
#28311=CARTESIAN_POINT ( 'NONE',  ( -5.999999999999963585, 1.780251999655701777E-13, -73.41367513459483973 ) ) ;
#28312=CARTESIAN_POINT ( 'NONE',  ( -3.175426480542816066, -5.500000000000057732, -81.87500000000002842 ) ) ;
#28314=CARTESIAN_POINT ( 'NONE',  ( -3.464101615137725076, 5.999999999999979572, -114.1636751345948113 ) ) ;
#28316=CARTESIAN_POINT ( 'NONE',  ( -4.763139720814407951, -2.750000000000016431, -68.50000000000000000 ) ) ;
#28317=CARTESIAN_POINT ( 'NONE',  ( -5.196152422706573404, -3.000000000000002665, -148.2886751345948824 ) ) ;
#28320=DIRECTION ( 'NONE',  ( -7.147005652999508048E-36, 5.642372883946980038E-36, 1.000000000000000000 ) ) ;
#28322=CARTESIAN_POINT ( 'NONE',  ( 0.000000000000000000, -5.999999999999991118, -145.0386751345948539 ) ) ;
#28327=CARTESIAN_POINT ( 'NONE',  ( 6.000000000000000888, -3.330669073875464691E-16, -7.560779664488942560E-35 ) ) ;
#28328=VECTOR ( 'NONE', #4229, 1000.000000000000000 ) ;
#28332=CARTESIAN_POINT ( 'NONE',  ( 0.000000000000000000, 5.499999999999991118, -87.00000000000002842 ) ) ;
#28334=CARTESIAN_POINT ( 'NONE',  ( 7.216878364870455975, -6.409875621278545621E-14, -99.80801270189222407 ) ) ;
#28335=VERTEX_POINT ( 'NONE', #7280 ) ;
#28337=CARTESIAN_POINT ( 'NONE',  ( -3.175426480542816510, -5.500000000000057732, -167.3750000000000568 ) ) ;
#28340=CARTESIAN_POINT ( 'NONE',  ( -5.196152422706601826, 2.999999999999975131, -93.03867513459485394 ) ) ;
#28343=CARTESIAN_POINT ( 'NONE',  ( -4.763139720814407951, -2.750000000000016431, -158.5000000000000284 ) ) ;
#28345=CARTESIAN_POINT ( 'NONE',  ( -6.350852961085760029, -1.281975124255709124E-13, -103.1250000000000142 ) ) ;
#28346=CARTESIAN_POINT ( 'NONE',  ( 3.464101615137852974, 5.999999999999884537, -59.83632486540521001 ) ) ;
#28347=CARTESIAN_POINT ( 'NONE',  ( -4.763139720814407951, 2.749999999999946709, -155.7500000000000568 ) ) ;
#28348=CARTESIAN_POINT ( 'NONE',  ( 0.000000000000000000, 5.499999999999991118, -93.00000000000002842 ) ) ;
#28360=VERTEX_POINT ( 'NONE', #10498 ) ;
#28362=EDGE_LOOP ( 'NONE', ( #4544, #18500, #27719 ) ) ;
#28364=CARTESIAN_POINT ( 'NONE',  ( -4.763139720814407951, 2.749999999999946709, -112.2500000000000142 ) ) ;
#28366=CARTESIAN_POINT ( 'NONE',  ( 2.775557561562891351E-14, 6.250000000000033751, -120.4330127018922099 ) ) ;
#28368=ORIENTED_EDGE ( 'NONE', *, *, #12482, .T. ) ;
#28370=CARTESIAN_POINT ( 'NONE',  ( 7.216878364870455975, -6.409875621278545621E-14, -172.4419872981078470 ) ) ;
#28373=VERTEX_POINT ( 'NONE', #5552 ) ;
#28374=EDGE_CURVE ( 'NONE', #16705, #3266, #14239, .T. ) ;
#28377=CARTESIAN_POINT ( 'NONE',  ( -4.763139720814407951, 2.749999999999946709, -178.2500000000000284 ) ) ;
#28379=CARTESIAN_POINT ( 'NONE',  ( 5.412658773652739619, 3.124999999999988898, -173.1830127018922383 ) ) ;
#28381=CARTESIAN_POINT ( 'NONE',  ( -5.196152422706573404, -3.000000000000002665, -101.7886751345948255 ) ) ;
#28384=CARTESIAN_POINT ( 'NONE',  ( -6.350852961085760029, -1.281975124255709124E-13, -115.1250000000000000 ) ) ;
#28385=CARTESIAN_POINT ( 'NONE',  ( -5.999999999999963585, -1.487416814333745711E-14, -165.8363248654052029 ) ) ;
#28387=ORIENTED_EDGE ( 'NONE', *, *, #15058, .F. ) ;
#28389=CARTESIAN_POINT ( 'NONE',  ( 6.000000000000000888, -3.330669073875464691E-16, -7.560779664488942560E-35 ) ) ;
#28390=CARTESIAN_POINT ( 'NONE',  ( 0.000000000000000000, 5.999999999999977796, -109.2113248654051887 ) ) ;
#28392=( BOUNDED_CURVE ( )  B_SPLINE_CURVE ( 2, ( #24602, #3399, #8017, #17123, #7717, #1251, #26893, #15274, #10660 ),
 .UNSPECIFIED., .F., .T. ) 
 B_SPLINE_CURVE_WITH_KNOTS ( ( 3, 2, 2, 2, 3 ),
 ( 0.2138888888888888784, 0.2148148148148148195, 0.2166666666666666741, 0.2185185185185185286, 0.2194444444444444697 ),
 .UNSPECIFIED. ) 
 CURVE ( )  GEOMETRIC_REPRESENTATION_ITEM ( )  RATIONAL_B_SPLINE_CURVE ( ( 0.9330127018922196314, 0.9330127018922185211, 1.000000000000000000, 0.8660254037844388186, 1.000000000000000000, 0.8660254037844388186, 1.000000000000000000, 0.9330127018922184101, 0.9330127018922194093 ) ) 
 REPRESENTATION_ITEM ( '' )  );
#28393=ORIENTED_EDGE ( 'NONE', *, *, #8773, .F. ) ;
#28394=CARTESIAN_POINT ( 'NONE',  ( -5.999999999999963585, 1.780251999655701777E-13, -98.91367513459483973 ) ) ;
#28395=CARTESIAN_POINT ( 'NONE',  ( 3.175426480543072749, -5.500000000000105693, -177.6250000000000284 ) ) ;
#28398=CARTESIAN_POINT ( 'NONE',  ( 5.196152422706629359, -2.999999999999988898, -77.28867513459481131 ) ) ;
#28401=ORIENTED_EDGE ( 'NONE', *, *, #24850, .T. ) ;
#28403=CARTESIAN_POINT ( 'NONE',  ( -5.999999999999944933, 1.607695154586759934, -140.9806624327026157 ) ) ;
#28405=ADVANCED_FACE ( 'NONE', ( #8016 ), #16975, .T. ) ;
#28406=CARTESIAN_POINT ( 'NONE',  ( -5.412658773652739619, 3.124999999999975131, -138.8169872981078186 ) ) ;
#28407=CARTESIAN_POINT ( 'NONE',  ( 0.000000000000000000, 0.000000000000000000, 0.000000000000000000 ) ) ;
#28408=CARTESIAN_POINT ( 'NONE',  ( 11.00000000000001599, -6.106226635438360972E-16, -1.386142938489641429E-34 ) ) ;
#28410=CARTESIAN_POINT ( 'NONE',  ( -6.000000000000000888, 1.067854986875958443E-15, 7.560779664488942560E-35 ) ) ;
#28413=ADVANCED_FACE ( 'NONE', ( #22008 ), #17122, .T. ) ;
#28415=CARTESIAN_POINT ( 'NONE',  ( 3.464101615137757051, -5.999999999999979572, -119.4136751345948397 ) ) ;
#28416=CARTESIAN_POINT ( 'NONE',  ( 3.464101615137852974, 5.999999999999884537, -92.83632486540514606 ) ) ;
#28419=( LENGTH_UNIT ( ) NAMED_UNIT ( * ) SI_UNIT ( .MILLI., .METRE. ) );
#28425=CARTESIAN_POINT ( 'NONE',  ( -4.763139720814407951, -2.750000000000016431, -50.49999999999998579 ) ) ;
#28426=CARTESIAN_POINT ( 'NONE',  ( -5.999999999999956479, -1.607695154586745057, -133.3466878364870354 ) ) ;
#28428=ORIENTED_EDGE ( 'NONE', *, *, #21100, .T. ) ;
#28431=CARTESIAN_POINT ( 'NONE',  ( -5.412658773652739619, 3.124999999999975131, -102.8169872981078470 ) ) ;
#28435=( BOUNDED_CURVE ( )  B_SPLINE_CURVE ( 2, ( #10775, #1064, #17683, #29004, #5505, #7969, #20123, #14913, #26694 ),
 .UNSPECIFIED., .F., .F. ) 
 B_SPLINE_CURVE_WITH_KNOTS ( ( 3, 2, 2, 2, 3 ),
 ( 0.6583333333333333259, 0.6592592592592592116, 0.6611111111111110938, 0.6629629629629629761, 0.6638888888888889728 ),
 .UNSPECIFIED. ) 
 CURVE ( )  GEOMETRIC_REPRESENTATION_ITEM ( )  RATIONAL_B_SPLINE_CURVE ( ( 0.9330127018922194093, 0.9330127018922194093, 1.000000000000000000, 0.8660254037844388186, 1.000000000000000000, 0.8660254037844388186, 1.000000000000000000, 0.9330127018922114157, 0.9330127018922194093 ) ) 
 REPRESENTATION_ITEM ( '' )  );
#28438=CARTESIAN_POINT ( 'NONE',  ( -3.175426480542816510, 5.499999999999865885, -131.8750000000000000 ) ) ;
#28440=ORIENTED_EDGE ( 'NONE', *, *, #24185, .T. ) ;
#28442=CARTESIAN_POINT ( 'NONE',  ( -2.775557561562891351E-14, -5.500000000000115463, -56.25000000000002132 ) ) ;
#28443=LINE ( 'NONE', #16826, #820 ) ;
#28445=EDGE_CURVE ( 'NONE', #2534, #4196, #26720, .T. ) ;
#28446=CARTESIAN_POINT ( 'NONE',  ( -5.412658773652684552, -3.125000000000099920, -85.43301270189223828 ) ) ;
#28452=CARTESIAN_POINT ( 'NONE',  ( 6.000000000000000888, -1.859271017917181981E-14, -110.1636751345948397 ) ) ;
#28454=CARTESIAN_POINT ( 'NONE',  ( -2.775557561562891351E-14, -5.500000000000115463, -140.2500000000000000 ) ) ;
#28455=CARTESIAN_POINT ( 'NONE',  ( -5.999999999999956479, -1.607695154586745057, -105.7693375672974696 ) ) ;
#28456=CARTESIAN_POINT ( 'NONE',  ( -3.608439182435115633, 6.249999999999965361, -154.8080127018922383 ) ) ;
#28457=CARTESIAN_POINT ( 'NONE',  ( 6.000000000000000000, -3.330669073875464198E-16, -180.0000000000000568 ) ) ;
#28459=CARTESIAN_POINT ( 'NONE',  ( -2.775557561562891351E-14, -5.500000000000115463, -68.25000000000002842 ) ) ;
#28462=CARTESIAN_POINT ( 'NONE',  ( -4.763139720814407951, 2.749999999999946709, -67.25000000000002842 ) ) ;
#28464=CYLINDRICAL_SURFACE ( 'NONE', #13054, 6.000000000000000888 ) ;
#28468=CARTESIAN_POINT ( 'NONE',  ( 6.000000000000000888, -1.859271017917181981E-14, -147.0863248654052313 ) ) ;
#28469=DIRECTION ( 'NONE',  ( -7.147005652999508048E-36, 5.642372883946980038E-36, 1.000000000000000000 ) ) ;
#28470=AXIS2_PLACEMENT_3D ( 'NONE', #9443, #16541, #11778 ) ;
#28477=( BOUNDED_CURVE ( )  B_SPLINE_CURVE ( 2, ( #16548, #6975, #28156, #2380, #63, #7126, #25870, #23580, #2517 ),
 .UNSPECIFIED., .F., .T. ) 
 B_SPLINE_CURVE_WITH_KNOTS ( ( 3, 2, 2, 2, 3 ),
 ( 0.7583333333333333037, 0.7592592592592593004, 0.7611111111111110716, 0.7629629629629629539, 0.7638888888888888395 ),
 .UNSPECIFIED. ) 
 CURVE ( )  GEOMETRIC_REPRESENTATION_ITEM ( )  RATIONAL_B_SPLINE_CURVE ( ( 0.9330127018922194093, 0.9330127018922154125, 1.000000000000000000, 0.8660254037844388186, 1.000000000000000000, 0.8660254037844388186, 1.000000000000000000, 0.9330127018922234061, 0.9330127018922194093 ) ) 
 REPRESENTATION_ITEM ( '' )  );
#28478=EDGE_CURVE ( 'NONE', #16758, #18552, #7560, .T. ) ;
#28479=CARTESIAN_POINT ( 'NONE',  ( 0.000000000000000000, 5.999999999999977796, -64.21132486540520290 ) ) ;
#28480=CARTESIAN_POINT ( 'NONE',  ( -6.350852961085760029, -1.281975124255709124E-13, -179.6250000000000284 ) ) ;
#28482=CARTESIAN_POINT ( 'NONE',  ( 2.775557561562891351E-14, 6.250000000000033751, -154.0669872981078470 ) ) ;
#28483=ORIENTED_EDGE ( 'NONE', *, *, #1328, .F. ) ;
#28484=CARTESIAN_POINT ( 'NONE',  ( 4.763139720814407951, 2.750000000000002665, -79.74999999999998579 ) ) ;
#28486=( BOUNDED_CURVE ( )  B_SPLINE_CURVE ( 2, ( #20676, #18386, #11328, #27703, #13637, #19650, #6525, #5644, #3489 ),
 .UNSPECIFIED., .F., .T. ) 
 B_SPLINE_CURVE_WITH_KNOTS ( ( 3, 2, 2, 2, 3 ),
 ( 0.8138888888888888840, 0.8148148148148147696, 0.8166666666666666519, 0.8185185185185185341, 0.8194444444444445308 ),
 .UNSPECIFIED. ) 
 CURVE ( )  GEOMETRIC_REPRESENTATION_ITEM ( )  RATIONAL_B_SPLINE_CURVE ( ( 0.9330127018922194093, 0.9330127018922194093, 1.000000000000000000, 0.8660254037844388186, 1.000000000000000000, 0.8660254037844388186, 1.000000000000000000, 0.9330127018922154125, 0.9330127018922194093 ) ) 
 REPRESENTATION_ITEM ( '' )  );
#28489=CARTESIAN_POINT ( 'NONE',  ( -5.196152422706601826, 2.999999999999975131, -147.0386751345948539 ) ) ;
#28492=DIRECTION ( 'NONE',  ( -7.147005652999508048E-36, 5.642372883946980038E-36, 1.000000000000000000 ) ) ;
#28494=CARTESIAN_POINT ( 'NONE',  ( 4.763139720814407951, 2.750000000000002665, -160.7500000000000568 ) ) ;
#28495=CARTESIAN_POINT ( 'NONE',  ( 3.464101615137852974, 5.999999999999884537, -161.8363248654052313 ) ) ;
#28496=CARTESIAN_POINT ( 'NONE',  ( -4.763139720814407951, -2.750000000000016431, -155.5000000000000284 ) ) ;
#28498=CARTESIAN_POINT ( 'NONE',  ( 6.350852961086080661, -9.614813431917819062E-14, -91.87500000000001421 ) ) ;
#28500=CARTESIAN_POINT ( 'NONE',  ( -6.350852961085760029, -1.281975124255709124E-13, -86.62499999999998579 ) ) ;
#28505=CARTESIAN_POINT ( 'NONE',  ( -5.999999999999963585, 8.134310703387671600E-14, -119.3363248654052455 ) ) ;
#28507=CARTESIAN_POINT ( 'NONE',  ( 0.000000000000000000, 5.999999999999977796, -178.7886751345948539 ) ) ;
#28508=CYLINDRICAL_SURFACE ( 'NONE', #10881, 6.000000000000000888 ) ;
#28511=EDGE_CURVE ( 'NONE', #567, #6844, #5255, .T. ) ;
#28512=CARTESIAN_POINT ( 'NONE',  ( -3.175426480542816510, 5.499999999999865885, -110.8750000000000426 ) ) ;
#28514=CARTESIAN_POINT ( 'NONE',  ( 2.775557561562891351E-14, -6.250000000000061284, -127.1830127018922525 ) ) ;
#28516=CARTESIAN_POINT ( 'NONE',  ( 3.464101615137757051, -5.999999999999979572, -68.41367513459479710 ) ) ;
#28517=CARTESIAN_POINT ( 'NONE',  ( 3.608439182435180470, -6.249999999999997335, -160.6919872981078470 ) ) ;
#28519=( BOUNDED_CURVE ( )  B_SPLINE_CURVE ( 2, ( #29785, #29160, #8123, #24565, #26856, #5815, #5982, #15232, #3516 ),
 .UNSPECIFIED., .F., .F. ) 
 B_SPLINE_CURVE_WITH_KNOTS ( ( 3, 2, 2, 2, 3 ),
 ( 0.5472222222222221655, 0.5481481481481481621, 0.5500000000000000444, 0.5518518518518518157, 0.5527777777777778123 ),
 .UNSPECIFIED. ) 
 CURVE ( )  GEOMETRIC_REPRESENTATION_ITEM ( )  RATIONAL_B_SPLINE_CURVE ( ( 0.9330127018922194093, 0.9330127018922154125, 1.000000000000000000, 0.8660254037844388186, 1.000000000000000000, 0.8660254037844388186, 1.000000000000000000, 0.9330127018922154125, 0.9330127018922194093 ) ) 
 REPRESENTATION_ITEM ( '' )  );
#28522=CARTESIAN_POINT ( 'NONE',  ( -5.196152422706573404, -3.000000000000002665, -132.7113248654052597 ) ) ;
#28523=CARTESIAN_POINT ( 'NONE',  ( 0.000000000000000000, 5.499999999999991118, -177.0000000000000568 ) ) ;
#28525=CARTESIAN_POINT ( 'NONE',  ( 6.000000000000000888, -1.607695154586752384, -168.7306624327026157 ) ) ;
#28526=CARTESIAN_POINT ( 'NONE',  ( 3.608439182435180470, -6.249999999999997335, -179.5580127018922383 ) ) ;
#28527=CARTESIAN_POINT ( 'NONE',  ( 6.000000000000000888, 1.743066579297358182E-13, -76.58632486540521711 ) ) ;
#28529=CARTESIAN_POINT ( 'NONE',  ( -4.763139720814407951, -2.750000000000016431, -127.0000000000000000 ) ) ;
#28531=CARTESIAN_POINT ( 'NONE',  ( 3.175426480543072749, -5.500000000000105693, -110.1249999999999858 ) ) ;
#28534=ORIENTED_EDGE ( 'NONE', *, *, #7037, .F. ) ;
#28537=ADVANCED_FACE ( 'NONE', ( #28898 ), #24296, .T. ) ;
#28538=DIRECTION ( 'NONE',  ( -7.147005652999508048E-36, 5.642372883946980038E-36, 1.000000000000000000 ) ) ;
#28539=DIRECTION ( 'NONE',  ( -7.147005652999508048E-36, 5.642372883946980038E-36, 1.000000000000000000 ) ) ;
#28541=CARTESIAN_POINT ( 'NONE',  ( 6.000000000000000888, -1.859271017917181981E-14, -145.5863248654052029 ) ) ;
#28542=VERTEX_POINT ( 'NONE', #22778 ) ;
#28543=CARTESIAN_POINT ( 'NONE',  ( -4.763139720814407951, -2.750000000000016431, -178.0000000000000568 ) ) ;
#28546=EDGE_LOOP ( 'NONE', ( #6186, #18816, #3303, #27332 ) ) ;
#28547=CARTESIAN_POINT ( 'NONE',  ( 3.464101615137757051, -5.999999999999979572, -95.41367513459479710 ) ) ;
#28549=VERTEX_POINT ( 'NONE', #8320 ) ;
#28550=AXIS2_PLACEMENT_3D ( 'NONE', #15435, #22314, #1246 ) ;
#28553=CARTESIAN_POINT ( 'NONE',  ( -5.412658773652739619, 3.124999999999975131, -129.8169872981078186 ) ) ;
#28554=DIRECTION ( 'NONE',  ( -7.147005652999508048E-36, 5.642372883946980038E-36, 1.000000000000000000 ) ) ;
#28556=CARTESIAN_POINT ( 'NONE',  ( 0.000000000000000000, 0.000000000000000000, 0.000000000000000000 ) ) ;
#28557=EDGE_LOOP ( 'NONE', ( #21854, #8332, #21439, #14084 ) ) ;
#28559=CARTESIAN_POINT ( 'NONE',  ( 6.000000000000026645, -1.607695154586707753, -129.7306624327025872 ) ) ;
#28563=LINE ( 'NONE', #10160, #8994 ) ;
#28564=( NAMED_UNIT ( * ) SI_UNIT ( $, .STERADIAN. ) SOLID_ANGLE_UNIT ( ) );
#28567=CARTESIAN_POINT ( 'NONE',  ( -4.763139720814407951, 2.749999999999946709, -137.7500000000000284 ) ) ;
#28573=CYLINDRICAL_SURFACE ( 'NONE', #8520, 6.000000000000000888 ) ;
#28574=CARTESIAN_POINT ( 'NONE',  ( 5.196152422706629359, 3.000000000000002665, -79.46132486540524553 ) ) ;
#28576=CARTESIAN_POINT ( 'NONE',  ( 0.000000000000000000, 5.999999999999977796, -152.7113248654052313 ) ) ;
#28580=CARTESIAN_POINT ( 'NONE',  ( 3.608439182435180470, 6.249999999999982236, -94.19198729810779014 ) ) ;
#28581=CARTESIAN_POINT ( 'NONE',  ( -5.999999999999963585, 1.780251999655701777E-13, -78.83632486540523132 ) ) ;
#28585=CARTESIAN_POINT ( 'NONE',  ( 3.175426480543072749, 5.499999999999865885, -129.1250000000000284 ) ) ;
#28588=CARTESIAN_POINT ( 'NONE',  ( 3.175426480543072749, -5.500000000000105693, -59.12499999999999289 ) ) ;
#28591=CARTESIAN_POINT ( 'NONE',  ( -3.608439182435052128, -6.250000000000110134, -85.30801270189222407 ) ) ;
#28592=CARTESIAN_POINT ( 'NONE',  ( 6.000000000000000888, -1.859271017917181981E-14, -169.5863248654052029 ) ) ;
#28596=CARTESIAN_POINT ( 'NONE',  ( -4.763139720814407951, 2.749999999999946709, -143.7500000000000568 ) ) ;
#28597=CARTESIAN_POINT ( 'NONE',  ( 6.000000000000000888, -3.330669073875464691E-16, -7.560779664488942560E-35 ) ) ;
#28598=CARTESIAN_POINT ( 'NONE',  ( 2.775557561562891351E-14, -6.250000000000061284, -155.6830127018922099 ) ) ;
#28599=CARTESIAN_POINT ( 'NONE',  ( -5.196152422706601826, 2.999999999999975131, -158.4613248654052029 ) ) ;
#28600=CARTESIAN_POINT ( 'NONE',  ( 3.464101615137852974, 5.999999999999884537, -51.41367513459485394 ) ) ;
#28601=ADVANCED_FACE ( 'NONE', ( #18186 ), #1872, .T. ) ;
#28602=CARTESIAN_POINT ( 'NONE',  ( -6.350852961085760029, -1.281975124255709124E-13, -71.62500000000005684 ) ) ;
#28603=CARTESIAN_POINT ( 'NONE',  ( 3.175426480543072749, 5.499999999999865885, -64.62500000000001421 ) ) ;
#28605=AXIS2_PLACEMENT_3D ( 'NONE', #24647, #22522, #1455 ) ;
#28611=CARTESIAN_POINT ( 'NONE',  ( 3.464101615137757051, -5.999999999999979572, -88.83632486540521711 ) ) ;
#28612=EDGE_CURVE ( 'NONE', #10004, #22416, #18731, .T. ) ;
#28613=ORIENTED_EDGE ( 'NONE', *, *, #7508, .F. ) ;
#28616=CARTESIAN_POINT ( 'NONE',  ( 0.000000000000000000, 0.000000000000000000, 0.000000000000000000 ) ) ;
#28617=CARTESIAN_POINT ( 'NONE',  ( -3.608439182435052128, -6.250000000000110134, -46.94198729810782567 ) ) ;
#28620=CARTESIAN_POINT ( 'NONE',  ( -2.775557561562891351E-14, -5.500000000000115463, -78.74999999999998579 ) ) ;
#28621=CARTESIAN_POINT ( 'NONE',  ( -3.608439182435052128, -6.250000000000110134, -101.8080127018922241 ) ) ;
#28622=ORIENTED_EDGE ( 'NONE', *, *, #23310, .T. ) ;
#28627=CARTESIAN_POINT ( 'NONE',  ( 4.763139720814407951, 2.750000000000002665, -162.2500000000000000 ) ) ;
#28628=CARTESIAN_POINT ( 'NONE',  ( 6.000000000000000888, -1.859271017917181981E-14, -80.16367513459481131 ) ) ;
#28629=CARTESIAN_POINT ( 'NONE',  ( -4.763139720814407951, -2.750000000000016431, -157.0000000000000284 ) ) ;
#28633=CARTESIAN_POINT ( 'NONE',  ( -6.350852961085760029, -1.281975124255709124E-13, -91.12500000000001421 ) ) ;
#28634=CARTESIAN_POINT ( 'NONE',  ( 3.464101615137852974, 5.999999999999884537, -125.8363248654051887 ) ) ;
#28635=CARTESIAN_POINT ( 'NONE',  ( -5.999999999999971578, 1.607695154586715303, -59.40331216351300014 ) ) ;
#28637=CARTESIAN_POINT ( 'NONE',  ( 3.175426480543072749, 5.499999999999865885, -93.12500000000002842 ) ) ;
#28638=FACE_OUTER_BOUND ( 'NONE', #6312, .T. ) ;
#28640=CARTESIAN_POINT ( 'NONE',  ( 6.000000000000000888, -1.859271017917181981E-14, -72.08632486540521711 ) ) ;
#28645=CARTESIAN_POINT ( 'NONE',  ( 5.196152422706629359, 3.000000000000002665, -72.53867513459482552 ) ) ;
#28647=( BOUNDED_CURVE ( )  B_SPLINE_CURVE ( 2, ( #23736, #514, #24580, #5833, #21134, #29030, #71, #28165, #7135 ),
 .UNSPECIFIED., .F., .T. ) 
 B_SPLINE_CURVE_WITH_KNOTS ( ( 3, 2, 2, 2, 3 ),
 ( 0.7249999999999999778, 0.7259259259259258634, 0.7277777777777778567, 0.7296296296296296280, 0.7305555555555556246 ),
 .UNSPECIFIED. ) 
 CURVE ( )  GEOMETRIC_REPRESENTATION_ITEM ( )  RATIONAL_B_SPLINE_CURVE ( ( 0.9330127018922194093, 0.9330127018922194093, 1.000000000000000000, 0.8660254037844388186, 1.000000000000000000, 0.8660254037844388186, 1.000000000000000000, 0.9330127018922114157, 0.9330127018922194093 ) ) 
 REPRESENTATION_ITEM ( '' )  );
#28648=ORIENTED_EDGE ( 'NONE', *, *, #28948, .F. ) ;
#28652=( BOUNDED_CURVE ( )  B_SPLINE_CURVE ( 2, ( #20799, #16518, #18355, #21245, #18962, #25689, #11755, #16666, #18806 ),
 .UNSPECIFIED., .F., .T. ) 
 B_SPLINE_CURVE_WITH_KNOTS ( ( 3, 2, 2, 2, 3 ),
 ( 0.7805555555555555580, 0.7814814814814814437, 0.7833333333333333259, 0.7851851851851852082, 0.7861111111111110938 ),
 .UNSPECIFIED. ) 
 CURVE ( )  GEOMETRIC_REPRESENTATION_ITEM ( )  RATIONAL_B_SPLINE_CURVE ( ( 0.9330127018922194093, 0.9330127018922194093, 1.000000000000000000, 0.8660254037844388186, 1.000000000000000000, 0.8660254037844388186, 1.000000000000000000, 0.9330127018922194093, 0.9330127018922194093 ) ) 
 REPRESENTATION_ITEM ( '' )  );
#28654=CARTESIAN_POINT ( 'NONE',  ( -3.175426480542816510, -5.500000000000057732, -105.8750000000000284 ) ) ;
#28656=CARTESIAN_POINT ( 'NONE',  ( 0.000000000000000000, 5.499999999999991118, -150.0000000000000284 ) ) ;
#28657=CARTESIAN_POINT ( 'NONE',  ( 3.608439182435180470, 6.249999999999982236, -125.0580127018921957 ) ) ;
#28658=EDGE_LOOP ( 'NONE', ( #14197, #23817, #13273, #15622 ) ) ;
#28659=CARTESIAN_POINT ( 'NONE',  ( 2.775557561562891351E-14, 6.250000000000033751, -161.5669872981078186 ) ) ;
#28663=CARTESIAN_POINT ( 'NONE',  ( 2.775557561562891351E-14, -6.250000000000061284, -56.68301270189224539 ) ) ;
#28664=ORIENTED_EDGE ( 'NONE', *, *, #424, .F. ) ;
#28665=CARTESIAN_POINT ( 'NONE',  ( 0.000000000000000000, -5.999999999999991118, -132.4613248654051745 ) ) ;
#28666=CARTESIAN_POINT ( 'NONE',  ( 6.000000000000000888, -3.330669073875464691E-16, -7.560779664488942560E-35 ) ) ;
#28667=CARTESIAN_POINT ( 'NONE',  ( 0.000000000000000000, 5.499999999999991118, -178.5000000000000000 ) ) ;
#28669=CARTESIAN_POINT ( 'NONE',  ( -5.196152422706573404, -3.000000000000002665, -169.2886751345948255 ) ) ;
#28670=CARTESIAN_POINT ( 'NONE',  ( -3.608439182435115633, 6.249999999999965361, -178.8080127018922667 ) ) ;
#28673=ADVANCED_FACE ( 'NONE', ( #4015 ), #2616, .F. ) ;
#28674=CARTESIAN_POINT ( 'NONE',  ( -5.999999999999983125, 1.067854986875956076E-15, -44.99152654425658682 ) ) ;
#28675=EDGE_CURVE ( 'NONE', #9700, #17985, #15006, .T. ) ;
#28676=CARTESIAN_POINT ( 'NONE',  ( 3.175426480543072749, -5.500000000000105693, -111.6249999999999858 ) ) ;
#28677=CARTESIAN_POINT ( 'NONE',  ( -3.464101615137725076, 5.999999999999979572, -142.6636751345948255 ) ) ;
#28679=CARTESIAN_POINT ( 'NONE',  ( -5.196152422706601826, 2.999999999999975131, -88.53867513459483973 ) ) ;
#28683=CARTESIAN_POINT ( 'NONE',  ( -3.464101615137757051, -5.999999999999979572, -56.08632486540518158 ) ) ;
#28684=ORIENTED_EDGE ( 'NONE', *, *, #17804, .F. ) ;
#28686=CARTESIAN_POINT ( 'NONE',  ( 0.000000000000000000, 5.499999999999991118, -180.0000000000000568 ) ) ;
#28690=VERTEX_POINT ( 'NONE', #16205 ) ;
#28693=ORIENTED_EDGE ( 'NONE', *, *, #22809, .T. ) ;
#28694=CARTESIAN_POINT ( 'NONE',  ( 6.000000000000000888, 1.743066579297358182E-13, -85.58632486540523132 ) ) ;
#28698=CARTESIAN_POINT ( 'NONE',  ( -5.412658773652684552, -3.125000000000099920, -134.0669872981078470 ) ) ;
#28700=CARTESIAN_POINT ( 'NONE',  ( 0.000000000000000000, 5.999999999999977796, -130.7886751345947971 ) ) ;
#28706=LINE ( 'NONE', #7528, #11802 ) ;
#28709=LINE ( 'NONE', #10009, #3476 ) ;
#28711=CARTESIAN_POINT ( 'NONE',  ( 0.000000000000000000, 0.000000000000000000, 0.000000000000000000 ) ) ;
#28714=CARTESIAN_POINT ( 'NONE',  ( -5.999999999999963585, 8.134310703387671600E-14, -115.4136751345948397 ) ) ;
#28716=CARTESIAN_POINT ( 'NONE',  ( 3.175426480543072749, -5.500000000000105693, -135.6250000000000000 ) ) ;
#28717=CYLINDRICAL_SURFACE ( 'NONE', #18621, 6.000000000000000888 ) ;
#28718=ORIENTED_EDGE ( 'NONE', *, *, #8908, .F. ) ;
#28720=CARTESIAN_POINT ( 'NONE',  ( 6.000000000000000888, 1.607695154586715303, -88.51933756729746960 ) ) ;
#28721=LINE ( 'NONE', #26871, #649 ) ;
#28722=CARTESIAN_POINT ( 'NONE',  ( -5.196152422706573404, -3.000000000000002665, -164.2113248654052313 ) ) ;
#28723=ORIENTED_EDGE ( 'NONE', *, *, #20751, .F. ) ;
#28726=CARTESIAN_POINT ( 'NONE',  ( -3.608439182435115633, 6.249999999999965361, -92.44198729810784698 ) ) ;
#28727=CARTESIAN_POINT ( 'NONE',  ( -6.000000000000007105, -1.607695154586655129, -78.76933756729745539 ) ) ;
#28733=CARTESIAN_POINT ( 'NONE',  ( 3.175426480543072749, 5.499999999999865885, -126.1250000000000426 ) ) ;
#28734=EDGE_CURVE ( 'NONE', #9152, #2251, #12078, .T. ) ;
#28736=EDGE_CURVE ( 'NONE', #29376, #23842, #6557, .T. ) ;
#28737=CARTESIAN_POINT ( 'NONE',  ( 4.763139720814407951, 2.750000000000002665, -60.25000000000002842 ) ) ;
#28738=DIRECTION ( 'NONE',  ( 1.000000000000000000, -5.551115123125773458E-17, -1.260129944081490338E-35 ) ) ;
#28739=CARTESIAN_POINT ( 'NONE',  ( 6.000000000000000888, -3.330669073875464691E-16, -7.560779664488942560E-35 ) ) ;
#28740=CARTESIAN_POINT ( 'NONE',  ( 5.960408494996782380, 9.245657484109267799, -25.79492440527508990 ) ) ;
#28741=CARTESIAN_POINT ( 'NONE',  ( -3.608439182435115633, 6.249999999999965361, -81.30801270189226670 ) ) ;
#28742=( BOUNDED_CURVE ( )  B_SPLINE_CURVE ( 2, ( #290, #26095, #20750, #27779, #11710, #6754, #23213, #9370, #30249 ),
 .UNSPECIFIED., .F., .T. ) 
 B_SPLINE_CURVE_WITH_KNOTS ( ( 3, 2, 2, 2, 3 ),
 ( 0.1638888888888888895, 0.1648148148148148029, 0.1666666666666666574, 0.1685185185185185119, 0.1694444444444444253 ),
 .UNSPECIFIED. ) 
 CURVE ( )  GEOMETRIC_REPRESENTATION_ITEM ( )  RATIONAL_B_SPLINE_CURVE ( ( 0.9330127018922194093, 0.9330127018922194093, 1.000000000000000000, 0.8660254037844388186, 1.000000000000000000, 0.8660254037844388186, 1.000000000000000000, 0.9330127018922205195, 0.9330127018922196314 ) ) 
 REPRESENTATION_ITEM ( '' )  );
#28743=CARTESIAN_POINT ( 'NONE',  ( 0.000000000000000000, -5.999999999999991118, -100.9613248654052171 ) ) ;
#28744=CARTESIAN_POINT ( 'NONE',  ( -3.464101615137725076, 5.999999999999979572, -169.0863248654052029 ) ) ;
#28750=ADVANCED_FACE ( 'NONE', ( #30285 ), #7089, .T. ) ;
#28751=CARTESIAN_POINT ( 'NONE',  ( 3.175426480543072749, 5.499999999999865885, -139.6250000000000000 ) ) ;
#28753=CARTESIAN_POINT ( 'NONE',  ( 5.412658773652712085, -3.125000000000086153, -155.4330127018922383 ) ) ;
#28754=CARTESIAN_POINT ( 'NONE',  ( -5.196152422706601826, 2.999999999999975131, -101.4613248654052171 ) ) ;
#28755=CARTESIAN_POINT ( 'NONE',  ( -3.464101615137725076, 5.999999999999979572, -67.08632486540523132 ) ) ;
#28756=CARTESIAN_POINT ( 'NONE',  ( -4.763139720814407951, 2.749999999999946709, -73.25000000000004263 ) ) ;
#28757=CARTESIAN_POINT ( 'NONE',  ( 3.175426480543072749, 5.499999999999865885, -54.12500000000003553 ) ) ;
#28761=CARTESIAN_POINT ( 'NONE',  ( 6.000000000000000888, 1.607695154586715303, -127.5193375672974412 ) ) ;
#28763=FACE_OUTER_BOUND ( 'NONE', #4302, .T. ) ;
#28767=DIRECTION ( 'NONE',  ( 1.000000000000000000, -5.551115123125774074E-17, 0.000000000000000000 ) ) ;
#28769=CARTESIAN_POINT ( 'NONE',  ( 4.763139720814407951, -2.749999999999988454, -180.5000000000000000 ) ) ;
#28772=ADVANCED_FACE ( 'NONE', ( #18638 ), #29973, .T. ) ;
#28773=CARTESIAN_POINT ( 'NONE',  ( 3.175426480543072749, -5.500000000000105693, -83.12500000000004263 ) ) ;
#28774=CARTESIAN_POINT ( 'NONE',  ( 3.608439182435180470, 6.249999999999982236, -99.55801270189222407 ) ) ;
#28775=AXIS2_PLACEMENT_3D ( 'NONE', #12450, #7641, #14170 ) ;
#28777=CARTESIAN_POINT ( 'NONE',  ( -5.999999999999963585, -1.487416814333745711E-14, -96.83632486540520290 ) ) ;
#28778=CARTESIAN_POINT ( 'NONE',  ( -5.999999999999963585, 1.780251999655701777E-13, -100.4136751345948255 ) ) ;
#28781=VECTOR ( 'NONE', #9569, 1000.000000000000000 ) ;
#28785=CARTESIAN_POINT ( 'NONE',  ( -2.775557561562891351E-14, -5.500000000000115463, -164.2500000000000000 ) ) ;
#28786=CARTESIAN_POINT ( 'NONE',  ( 6.000000000000000888, -1.859271017917181981E-14, -58.58632486540521001 ) ) ;
#28787=CARTESIAN_POINT ( 'NONE',  ( 0.000000000000000000, 5.499999999999991118, -145.5000000000000284 ) ) ;
#28788=FACE_OUTER_BOUND ( 'NONE', #22074, .T. ) ;
#28789=CARTESIAN_POINT ( 'NONE',  ( 6.000000000000052403, -1.607695154586662678, -103.6533121635130072 ) ) ;
#28791=CARTESIAN_POINT ( 'NONE',  ( -3.175426480542816066, -5.500000000000057732, -92.37500000000002842 ) ) ;
#28793=CARTESIAN_POINT ( 'NONE',  ( 4.763139720814407951, -2.749999999999988454, -80.00000000000001421 ) ) ;
#28795=DIRECTION ( 'NONE',  ( 1.000000000000000000, -5.551115123125773458E-17, -1.260129944081490338E-35 ) ) ;
#28799=CARTESIAN_POINT ( 'NONE',  ( 0.000000000000000000, -5.999999999999991118, -73.96132486540524553 ) ) ;
#28801=ORIENTED_EDGE ( 'NONE', *, *, #28445, .T. ) ;
#28802=CARTESIAN_POINT ( 'NONE',  ( -5.196152422706601826, 2.999999999999975131, -178.5386751345948824 ) ) ;
#28803=CARTESIAN_POINT ( 'NONE',  ( 0.000000000000000000, -5.999999999999991118, -79.03867513459483973 ) ) ;
#28810=CARTESIAN_POINT ( 'NONE',  ( -3.175426480542816510, 5.499999999999865885, -101.8750000000000000 ) ) ;
#28812=CARTESIAN_POINT ( 'NONE',  ( 2.775557561562891351E-14, 6.250000000000033751, -123.4330127018922241 ) ) ;
#28814=CARTESIAN_POINT ( 'NONE',  ( -5.999999999999963585, 1.780251999655701777E-13, -61.41367513459483973 ) ) ;
#28815=CARTESIAN_POINT ( 'NONE',  ( 5.412658773652739619, 3.124999999999988898, -158.8169872981078470 ) ) ;
#28817=AXIS2_PLACEMENT_3D ( 'NONE', #17331, #854, #26647 ) ;
#28819=CARTESIAN_POINT ( 'NONE',  ( 5.412658773652739619, 3.124999999999988898, -56.18301270189224539 ) ) ;
#28820=VERTEX_POINT ( 'NONE', #16804 ) ;
#28822=CARTESIAN_POINT ( 'NONE',  ( -5.676437577760642839, 9.422458200488973645, -23.04620489006168782 ) ) ;
#28823=CARTESIAN_POINT ( 'NONE',  ( -5.999999999999919176, 1.607695154586804565, -137.4033121635130215 ) ) ;
#28824=CARTESIAN_POINT ( 'NONE',  ( -3.175426480542816510, 5.499999999999865885, -167.8750000000000568 ) ) ;
#28826=CARTESIAN_POINT ( 'NONE',  ( 5.196152422706629359, -2.999999999999988898, -112.7113248654052455 ) ) ;
#28827=CARTESIAN_POINT ( 'NONE',  ( 5.412658773652712085, -3.125000000000086153, -165.9330127018922099 ) ) ;
#28830=CARTESIAN_POINT ( 'NONE',  ( 0.000000000000000000, 5.499999999999991118, -118.5000000000000568 ) ) ;
#28831=CARTESIAN_POINT ( 'NONE',  ( -5.999999999999963585, 1.780251999655701777E-13, -83.91367513459482552 ) ) ;
#28833=CARTESIAN_POINT ( 'NONE',  ( 4.763139720814407951, 2.750000000000002665, -114.2500000000000142 ) ) ;
#28835=DIRECTION ( 'NONE',  ( 1.000000000000000000, -5.551115123125773458E-17, -1.260129944081490338E-35 ) ) ;
#28836=CARTESIAN_POINT ( 'NONE',  ( -5.999999999999919176, 1.607695154586804565, -100.4806624327025872 ) ) ;
#28837=ORIENTED_EDGE ( 'NONE', *, *, #4974, .T. ) ;
#28839=CARTESIAN_POINT ( 'NONE',  ( 5.196152422706629359, 3.000000000000002665, -168.5386751345947971 ) ) ;
#28840=( BOUNDED_CURVE ( )  B_SPLINE_CURVE ( 2, ( #4955, #13291, #10348, #17279, #26739, #3401, #20009, #8020, #1570 ),
 .UNSPECIFIED., .F., .T. ) 
 B_SPLINE_CURVE_WITH_KNOTS ( ( 3, 2, 2, 2, 3 ),
 ( 0.6472222222222221433, 0.6481481481481481399, 0.6500000000000000222, 0.6518518518518519045, 0.6527777777777777901 ),
 .UNSPECIFIED. ) 
 CURVE ( )  GEOMETRIC_REPRESENTATION_ITEM ( )  RATIONAL_B_SPLINE_CURVE ( ( 0.9330127018922194093, 0.9330127018922154125, 1.000000000000000000, 0.8660254037844388186, 1.000000000000000000, 0.8660254037844388186, 1.000000000000000000, 0.9330127018922194093, 0.9330127018922194093 ) ) 
 REPRESENTATION_ITEM ( '' )  );
#28841=CARTESIAN_POINT ( 'NONE',  ( -3.464101615137725076, 5.999999999999979572, -86.58632486540520290 ) ) ;
#28842=ORIENTED_EDGE ( 'NONE', *, *, #16510, .F. ) ;
#28845=CARTESIAN_POINT ( 'NONE',  ( 5.412658773652739619, 3.124999999999988898, -82.31698729810781856 ) ) ;
#28847=ORIENTED_EDGE ( 'NONE', *, *, #15951, .F. ) ;
#28848=CARTESIAN_POINT ( 'NONE',  ( 0.000000000000000000, 5.999999999999977796, -144.2886751345948824 ) ) ;
#28851=ORIENTED_EDGE ( 'NONE', *, *, #6714, .T. ) ;
#28854=EDGE_CURVE ( 'NONE', #28019, #13234, #26375, .T. ) ;
#28857=CARTESIAN_POINT ( 'NONE',  ( 2.775557561562891351E-14, 6.250000000000033751, -128.5669872981078470 ) ) ;
#28858=CARTESIAN_POINT ( 'NONE',  ( -5.196152422706601826, 2.999999999999975131, -49.53867513459481131 ) ) ;
#28859=CARTESIAN_POINT ( 'NONE',  ( 6.000000000000000888, 1.743066579297358182E-13, -90.66367513459483973 ) ) ;
#28862=CARTESIAN_POINT ( 'NONE',  ( -5.196152422706573404, -3.000000000000002665, -139.2886751345948539 ) ) ;
#28863=DIRECTION ( 'NONE',  ( 1.000000000000000000, -5.551115123125773458E-17, -1.260129944081490338E-35 ) ) ;
#28865=CARTESIAN_POINT ( 'NONE',  ( 0.000000000000000000, 0.000000000000000000, 0.000000000000000000 ) ) ;
#28866=CARTESIAN_POINT ( 'NONE',  ( -4.000000000000004441, 7.119033245839730840E-16, 5.040519776325966696E-35 ) ) ;
#28867=CYLINDRICAL_SURFACE ( 'NONE', #29247, 6.000000000000000888 ) ;
#28868=CARTESIAN_POINT ( 'NONE',  ( 0.000000000000000000, 0.000000000000000000, 0.000000000000000000 ) ) ;
#28870=CARTESIAN_POINT ( 'NONE',  ( 0.000000000000000000, 0.000000000000000000, 0.000000000000000000 ) ) ;
#28871=CARTESIAN_POINT ( 'NONE',  ( -3.175426480542816510, -5.500000000000057732, -137.3750000000000568 ) ) ;
#28872=CARTESIAN_POINT ( 'NONE',  ( 0.000000000000000000, 0.000000000000000000, 0.000000000000000000 ) ) ;
#28874=CARTESIAN_POINT ( 'NONE',  ( 4.763139720814407951, 2.750000000000002665, -48.25000000000001421 ) ) ;
#28880=APPLICATION_CONTEXT ( 'automotive_design' ) ;
#28881=CARTESIAN_POINT ( 'NONE',  ( -5.412658773652684552, -3.125000000000099920, -95.06698729810780435 ) ) ;
#28882=DIRECTION ( 'NONE',  ( -7.147005652999508048E-36, 5.642372883946980038E-36, 1.000000000000000000 ) ) ;
#28885=CARTESIAN_POINT ( 'NONE',  ( 6.000000000000000888, 1.743066579297358182E-13, -78.08632486540520290 ) ) ;
#28886=CARTESIAN_POINT ( 'NONE',  ( -3.175426480542816510, -5.500000000000057732, -132.8750000000000284 ) ) ;
#28888=EDGE_LOOP ( 'NONE', ( #21361, #28393, #14157, #15882 ) ) ;
#28889=ORIENTED_EDGE ( 'NONE', *, *, #17953, .T. ) ;
#28891=CARTESIAN_POINT ( 'NONE',  ( 3.175426480543072749, 5.499999999999865885, -60.12499999999999289 ) ) ;
#28892=AXIS2_PLACEMENT_3D ( 'NONE', #6013, #19845, #29193 ) ;
#28893=CARTESIAN_POINT ( 'NONE',  ( -3.464101615137725076, 5.999999999999979572, -69.16367513459479710 ) ) ;
#28894=CARTESIAN_POINT ( 'NONE',  ( 0.000000000000000000, -5.999999999999991118, -134.5386751345948255 ) ) ;
#28895=CARTESIAN_POINT ( 'NONE',  ( 2.511346088335001170, 10.71107091704333847, -30.45263927933801540 ) ) ;
#28896=CARTESIAN_POINT ( 'NONE',  ( 3.608439182435180470, -6.249999999999997335, -73.05801270189222407 ) ) ;
#28897=VECTOR ( 'NONE', #18229, 1000.000000000000000 ) ;
#28898=FACE_OUTER_BOUND ( 'NONE', #25785, .T. ) ;
#28901=CARTESIAN_POINT ( 'NONE',  ( 3.175426480543072749, -5.500000000000105693, -143.1250000000000000 ) ) ;
#28903=CARTESIAN_POINT ( 'NONE',  ( -3.608439182435052128, -6.250000000000110134, -152.8080127018922099 ) ) ;
#28904=DIRECTION ( 'NONE',  ( -7.147005652999508048E-36, 5.642372883946980038E-36, 1.000000000000000000 ) ) ;
#28905=CARTESIAN_POINT ( 'NONE',  ( -5.196152422706601826, 2.999999999999975131, -66.96132486540523132 ) ) ;
#28906=CARTESIAN_POINT ( 'NONE',  ( 0.000000000000000000, 5.499999999999991118, -73.50000000000001421 ) ) ;
#28907=CARTESIAN_POINT ( 'NONE',  ( 5.999999999999949374, 1.607695154586804565, -86.09668783648704959 ) ) ;
#28908=CARTESIAN_POINT ( 'NONE',  ( 4.763139720814407951, -2.749999999999988454, -60.50000000000000000 ) ) ;
#28912=DIRECTION ( 'NONE',  ( 1.000000000000000000, -5.551115123125774074E-17, -1.260129944081490070E-35 ) ) ;
#28914=DIRECTION ( 'NONE',  ( 1.000000000000000000, -5.551115123125773458E-17, -1.260129944081490338E-35 ) ) ;
#28919=LINE ( 'NONE', #22338, #27794 ) ;
#28924=CARTESIAN_POINT ( 'NONE',  ( -5.412658773652684552, -3.125000000000099920, -47.06698729810781856 ) ) ;
#28926=CARTESIAN_POINT ( 'NONE',  ( 2.775557561562891351E-14, -6.250000000000061284, -148.8169872981078186 ) ) ;
#28928=CARTESIAN_POINT ( 'NONE',  ( 3.175426480543072749, 5.499999999999865885, -78.12500000000001421 ) ) ;
#28929=CARTESIAN_POINT ( 'NONE',  ( -3.608439182435115633, 6.249999999999965361, -94.80801270189219565 ) ) ;
#28930=CARTESIAN_POINT ( 'NONE',  ( 5.999999999999998224, 1.607695154586720854, -176.0966878364870070 ) ) ;
#28935=CARTESIAN_POINT ( 'NONE',  ( 6.000000000000000888, -1.607695154586752384, -58.65331216351298593 ) ) ;
#28937=AXIS2_PLACEMENT_3D ( 'NONE', #6814, #11311, #25230 ) ;
#28938=CARTESIAN_POINT ( 'NONE',  ( 3.175426480543072749, 5.499999999999865885, -165.1250000000000000 ) ) ;
#28939=CARTESIAN_POINT ( 'NONE',  ( 6.000000000000000888, 1.743066579297358182E-13, -60.08632486540520290 ) ) ;
#28940=CARTESIAN_POINT ( 'NONE',  ( 4.763139720814407951, 2.750000000000002665, -145.7500000000000568 ) ) ;
#28943=CARTESIAN_POINT ( 'NONE',  ( -4.763139720814407951, 2.749999999999946709, -97.25000000000000000 ) ) ;
#28944=CARTESIAN_POINT ( 'NONE',  ( 3.175426480543072749, -5.500000000000105693, -81.62500000000002842 ) ) ;
#28945=CARTESIAN_POINT ( 'NONE',  ( -5.999999999999962697, 3.323446944526963891E-14, -159.8363248654052597 ) ) ;
#28946=CYLINDRICAL_SURFACE ( 'NONE', #6637, 6.000000000000000888 ) ;
#28948=EDGE_CURVE ( 'NONE', #3793, #16482, #28709, .T. ) ;
#28950=CARTESIAN_POINT ( 'NONE',  ( -6.000000000000007105, -1.607695154586655129, -74.26933756729742697 ) ) ;
#28952=ORIENTED_EDGE ( 'NONE', *, *, #21062, .T. ) ;
#28954=CYLINDRICAL_SURFACE ( 'NONE', #22427, 11.00000000000001599 ) ;
#28955=CARTESIAN_POINT ( 'NONE',  ( -3.464101615137757051, -5.999999999999979572, -79.16367513459483973 ) ) ;
#28958=ADVANCED_FACE ( 'NONE', ( #17090 ), #29013, .T. ) ;
#28960=ORIENTED_EDGE ( 'NONE', *, *, #23760, .T. ) ;
#28963=CARTESIAN_POINT ( 'NONE',  ( -3.175426480542816510, 5.499999999999865885, -106.3750000000000284 ) ) ;
#28965=CARTESIAN_POINT ( 'NONE',  ( -5.412658773652684552, -3.125000000000099920, -124.4330127018922241 ) ) ;
#28967=CARTESIAN_POINT ( 'NONE',  ( 5.412658773652739619, 3.124999999999988898, -163.3169872981078470 ) ) ;
#28969=VECTOR ( 'NONE', #19828, 1000.000000000000000 ) ;
#28970=CARTESIAN_POINT ( 'NONE',  ( -5.412658773652684552, -3.125000000000099920, -62.93301270189222407 ) ) ;
#28972=CARTESIAN_POINT ( 'NONE',  ( 6.000000000000000888, -3.330669073875464691E-16, -7.560779664488942560E-35 ) ) ;
#28974=CARTESIAN_POINT ( 'NONE',  ( -5.841785975170636469, 9.320713607846746740, -23.61690496628341407 ) ) ;
#28975=CARTESIAN_POINT ( 'NONE',  ( -4.763139720814407951, 2.749999999999946709, -167.7500000000000000 ) ) ;
#28977=CARTESIAN_POINT ( 'NONE',  ( -5.999999999999963585, 9.296355089585909904E-15, -169.4136751345948539 ) ) ;
#28978=CARTESIAN_POINT ( 'NONE',  ( 2.775557561562891351E-14, 6.250000000000033751, -172.9330127018922099 ) ) ;
#28982=CARTESIAN_POINT ( 'NONE',  ( -2.775557561562891351E-14, -5.500000000000115463, -117.7500000000000284 ) ) ;
#28984=CARTESIAN_POINT ( 'NONE',  ( -2.775557561562891351E-14, -5.500000000000115463, -102.7500000000000142 ) ) ;
#28985=CARTESIAN_POINT ( 'NONE',  ( -5.196152422706573404, -3.000000000000002665, -131.7886751345947971 ) ) ;
#28986=EDGE_LOOP ( 'NONE', ( #23529, #17941, #17950, #6005, #17524 ) ) ;
#28988=CARTESIAN_POINT ( 'NONE',  ( 0.000000000000000000, 0.000000000000000000, 0.000000000000000000 ) ) ;
#28991=CARTESIAN_POINT ( 'NONE',  ( 3.464101615137852974, 5.999999999999884537, -86.83632486540520290 ) ) ;
#28992=CARTESIAN_POINT ( 'NONE',  ( 6.000000000000000888, -1.859271017917181981E-14, -126.6636751345948397 ) ) ;
#28993=CARTESIAN_POINT ( 'NONE',  ( 2.775557561562891351E-14, -6.250000000000061284, -78.31698729810781856 ) ) ;
#28994=CYLINDRICAL_SURFACE ( 'NONE', #19996, 6.000000000000000888 ) ;
#29000=AXIS2_PLACEMENT_3D ( 'NONE', #6141, #15555, #28077 ) ;
#29003=CARTESIAN_POINT ( 'NONE',  ( -3.608439182435115633, 6.249999999999965361, -132.9419872981078186 ) ) ;
#29004=CARTESIAN_POINT ( 'NONE',  ( 3.464101615137757051, -5.999999999999979572, -135.3363248654052313 ) ) ;
#29005=CARTESIAN_POINT ( 'NONE',  ( 0.000000000000000000, -5.999999999999991118, -167.5386751345948539 ) ) ;
#29009=CARTESIAN_POINT ( 'NONE',  ( -6.000000000000000888, 1.067854986875958443E-15, 7.560779664488942560E-35 ) ) ;
#29011=CARTESIAN_POINT ( 'NONE',  ( 5.999999999999949374, 1.607695154586804565, -57.01933756729742697 ) ) ;
#29013=CYLINDRICAL_SURFACE ( 'NONE', #20685, 6.000000000000000888 ) ;
#29014=CARTESIAN_POINT ( 'NONE',  ( -5.999999999999963585, 8.134310703387671600E-14, -140.3363248654052313 ) ) ;
#29015=CARTESIAN_POINT ( 'NONE',  ( 5.412658773652712085, -3.125000000000086153, -69.06698729810784698 ) ) ;
#29017=CARTESIAN_POINT ( 'NONE',  ( -5.412658773652684552, -3.125000000000099920, -51.56698729810782567 ) ) ;
#29018=CARTESIAN_POINT ( 'NONE',  ( 0.000000000000000000, 0.000000000000000000, 0.000000000000000000 ) ) ;
#29021=CARTESIAN_POINT ( 'NONE',  ( -5.999999999999919176, 1.607695154586804565, -74.40331216351303567 ) ) ;
#29022=CARTESIAN_POINT ( 'NONE',  ( 4.763139720814407951, -2.749999999999988454, -126.5000000000000568 ) ) ;
#29025=EDGE_CURVE ( 'NONE', #15666, #2682, #20117, .T. ) ;
#29030=CARTESIAN_POINT ( 'NONE',  ( -3.464101615137757051, -5.999999999999979572, -144.5863248654052029 ) ) ;
#29036=CARTESIAN_POINT ( 'NONE',  ( 5.412658773652739619, 3.124999999999988898, -92.81698729810783277 ) ) ;
#29039=LINE ( 'NONE', #28327, #2813 ) ;
#29042=ORIENTED_EDGE ( 'NONE', *, *, #7345, .F. ) ;
#29043=CARTESIAN_POINT ( 'NONE',  ( -5.196152422706573404, -3.000000000000002665, -138.7113248654052029 ) ) ;
#29044=CARTESIAN_POINT ( 'NONE',  ( -3.175426480542816510, -5.500000000000057732, -56.37500000000004263 ) ) ;
#29046=CARTESIAN_POINT ( 'NONE',  ( -5.999999999999963585, 8.134310703387671600E-14, -116.3363248654052313 ) ) ;
#29048=CARTESIAN_POINT ( 'NONE',  ( -3.608439182435052128, -6.250000000000110134, -79.30801270189226670 ) ) ;
#29049=DIRECTION ( 'NONE',  ( -7.147005652999508048E-36, 5.642372883946980038E-36, 1.000000000000000000 ) ) ;
#29052=CARTESIAN_POINT ( 'NONE',  ( 5.196152422706629359, 3.000000000000002665, -80.03867513459483973 ) ) ;
#29055=CARTESIAN_POINT ( 'NONE',  ( -2.775557561562891351E-14, -5.500000000000115463, -134.2500000000000284 ) ) ;
#29057=CARTESIAN_POINT ( 'NONE',  ( -5.999999999999962697, 3.323446944526963891E-14, -152.3363248654052313 ) ) ;
#29059=CARTESIAN_POINT ( 'NONE',  ( 6.350852961086080661, -9.614813431917819062E-14, -73.87500000000000000 ) ) ;
#29060=CARTESIAN_POINT ( 'NONE',  ( 0.000000000000000000, 5.499999999999991118, -60.00000000000005684 ) ) ;
#29069=ORIENTED_EDGE ( 'NONE', *, *, #7947, .T. ) ;
#29072=CARTESIAN_POINT ( 'NONE',  ( -6.000000000000007105, -1.607695154586655129, -102.7693375672974270 ) ) ;
#29073=CARTESIAN_POINT ( 'NONE',  ( 4.763139720814407951, -2.749999999999988454, -179.0000000000000568 ) ) ;
#29075=ORIENTED_EDGE ( 'NONE', *, *, #1434, .T. ) ;
#29076=CARTESIAN_POINT ( 'NONE',  ( 2.775557561562891351E-14, -6.250000000000061284, -145.8169872981078186 ) ) ;
#29077=CARTESIAN_POINT ( 'NONE',  ( -6.350852961085760029, -1.281975124255709124E-13, -80.62500000000004263 ) ) ;
#29079=CARTESIAN_POINT ( 'NONE',  ( -5.412658773652739619, 3.124999999999975131, -94.68301270189222407 ) ) ;
#29080=CARTESIAN_POINT ( 'NONE',  ( 6.000000000000000888, -1.859271017917181981E-14, -105.6636751345948397 ) ) ;
#29082=CARTESIAN_POINT ( 'NONE',  ( 0.000000000000000000, -5.999999999999991118, -151.0386751345948539 ) ) ;
#29085=CARTESIAN_POINT ( 'NONE',  ( 6.350852961086080661, -9.614813431917819062E-14, -163.8750000000000568 ) ) ;
#29087=CARTESIAN_POINT ( 'NONE',  ( -3.175426480542816510, 5.499999999999865885, -146.8750000000000284 ) ) ;
#29088=LINE ( 'NONE', #8049, #19395 ) ;
#29089=CARTESIAN_POINT ( 'NONE',  ( 3.175426480543072749, 5.499999999999865885, -93.12500000000002842 ) ) ;
#29091=CARTESIAN_POINT ( 'NONE',  ( -4.763139720814407951, 2.749999999999946709, -80.74999999999998579 ) ) ;
#29094=CARTESIAN_POINT ( 'NONE',  ( 5.999999999999949374, 1.607695154586804565, -65.09668783648702117 ) ) ;
#29097=CARTESIAN_POINT ( 'NONE',  ( 0.000000000000000000, 5.999999999999977796, -124.7886751345948539 ) ) ;
#29099=CARTESIAN_POINT ( 'NONE',  ( -5.999999999999919176, 1.607695154586804565, -74.98066243270262987 ) ) ;
#29100=( BOUNDED_CURVE ( )  B_SPLINE_CURVE ( 2, ( #16192, #2174, #9232, #16641, #18781, #25818, #25962, #7078, #23678 ),
 .UNSPECIFIED., .F., .T. ) 
 B_SPLINE_CURVE_WITH_KNOTS ( ( 3, 2, 2, 2, 3 ),
 ( 0.2916666666666666297, 0.2925925925925925708, 0.2944444444444444531, 0.2962962962962962798, 0.2972222222222222210 ),
 .UNSPECIFIED. ) 
 CURVE ( )  GEOMETRIC_REPRESENTATION_ITEM ( )  RATIONAL_B_SPLINE_CURVE ( ( 0.9330127018922194093, 0.9330127018922174109, 1.000000000000000000, 0.8660254037844388186, 1.000000000000000000, 0.8660254037844388186, 1.000000000000000000, 0.9330127018922194093, 0.9330127018922194093 ) ) 
 REPRESENTATION_ITEM ( '' )  );
#29101=ORIENTED_EDGE ( 'NONE', *, *, #12403, .F. ) ;
#29102=CARTESIAN_POINT ( 'NONE',  ( 6.000000000000000888, 1.743066579297358182E-13, -91.58632486540523132 ) ) ;
#29104=CARTESIAN_POINT ( 'NONE',  ( 5.196152422706629359, 3.000000000000002665, -83.03867513459483973 ) ) ;
#29106=ORIENTED_EDGE ( 'NONE', *, *, #12207, .F. ) ;
#29109=CARTESIAN_POINT ( 'NONE',  ( -3.175426480542816510, 5.499999999999865885, -104.8750000000000142 ) ) ;
#29111=CARTESIAN_POINT ( 'NONE',  ( -3.608439182435052128, -6.250000000000110134, -116.8080127018922383 ) ) ;
#29113=CARTESIAN_POINT ( 'NONE',  ( -5.999999999999919176, 1.607695154586804565, -110.9806624327025872 ) ) ;
#29114=CARTESIAN_POINT ( 'NONE',  ( 2.775557561562891351E-14, 6.250000000000033751, -157.0669872981078754 ) ) ;
#29117=EDGE_CURVE ( 'NONE', #29147, #4124, #5377, .T. ) ;
#29118=CARTESIAN_POINT ( 'NONE',  ( 2.775557561562891351E-14, -6.250000000000061284, -52.18301270189223828 ) ) ;
#29121=DIRECTION ( 'NONE',  ( -7.147005652999508048E-36, 5.642372883946980038E-36, 1.000000000000000000 ) ) ;
#29123=DIRECTION ( 'NONE',  ( 1.000000000000000000, -5.551115123125773458E-17, -1.260129944081490338E-35 ) ) ;
#29124=CARTESIAN_POINT ( 'NONE',  ( -3.175426480542816510, 5.499999999999865885, -173.8750000000000000 ) ) ;
#29127=CARTESIAN_POINT ( 'NONE',  ( -5.412658773652739619, 3.124999999999975131, -165.1830127018922383 ) ) ;
#29128=CARTESIAN_POINT ( 'NONE',  ( 6.000000000000000888, 1.743066579297358182E-13, -48.66367513459482552 ) ) ;
#29130=CARTESIAN_POINT ( 'NONE',  ( -6.350852961085760029, -1.281975124255709124E-13, -116.6250000000000000 ) ) ;
#29132=EDGE_CURVE ( 'NONE', #7780, #9966, #8531, .T. ) ;
#29133=CARTESIAN_POINT ( 'NONE',  ( 4.763139720814407951, -2.749999999999988454, -105.5000000000000426 ) ) ;
#29135=ORIENTED_EDGE ( 'NONE', *, *, #1328, .T. ) ;
#29139=CARTESIAN_POINT ( 'NONE',  ( 6.000000000000000000, 2.951592740943527306E-14, -150.0863248654052029 ) ) ;
#29140=ORIENTED_EDGE ( 'NONE', *, *, #3740, .T. ) ;
#29141=CARTESIAN_POINT ( 'NONE',  ( -3.175426480542816510, -5.500000000000057732, -159.8750000000000284 ) ) ;
#29143=CARTESIAN_POINT ( 'NONE',  ( -5.412658773652739619, 3.124999999999975131, -83.31698729810781856 ) ) ;
#29145=ORIENTED_EDGE ( 'NONE', *, *, #1467, .T. ) ;
#29147=VERTEX_POINT ( 'NONE', #19814 ) ;
#29149=CARTESIAN_POINT ( 'NONE',  ( -7.216878364870328078, 0.000000000000000000, -138.0580127018922099 ) ) ;
#29150=VERTEX_POINT ( 'NONE', #1683 ) ;
#29151=CARTESIAN_POINT ( 'NONE',  ( 7.216878364870455975, -6.409875621278545621E-14, -130.4419872981078470 ) ) ;
#29154=EDGE_CURVE ( 'NONE', #7308, #27374, #28519, .T. ) ;
#29157=CARTESIAN_POINT ( 'NONE',  ( 6.000000000000000888, 1.607695154586715303, -135.5966878364870354 ) ) ;
#29158=CARTESIAN_POINT ( 'NONE',  ( 3.464101615137852974, 5.999999999999884537, -148.3363248654051461 ) ) ;
#29159=CARTESIAN_POINT ( 'NONE',  ( -5.999999999999919176, 1.607695154586804565, -56.40331216351302857 ) ) ;
#29160=CARTESIAN_POINT ( 'NONE',  ( -6.000000000000007105, -1.607695154586655129, -107.8466878364870354 ) ) ;
#29162=CARTESIAN_POINT ( 'NONE',  ( -3.608439182435052128, -6.250000000000110134, -69.44198729810781856 ) ) ;
#29164=CARTESIAN_POINT ( 'NONE',  ( -5.999999999999963585, 1.780251999655701777E-13, -64.41367513459483973 ) ) ;
#29165=CARTESIAN_POINT ( 'NONE',  ( 0.000000000000000000, 5.999999999999977796, -103.2113248654052455 ) ) ;
#29166=CARTESIAN_POINT ( 'NONE',  ( 6.000000000000000888, 1.743066579297358182E-13, -98.16367513459481131 ) ) ;
#29168=CARTESIAN_POINT ( 'NONE',  ( -3.175426480542816510, 5.499999999999865885, -127.3750000000000000 ) ) ;
#29169=ADVANCED_FACE ( 'NONE', ( #24724 ), #13100, .T. ) ;
#29173=ORIENTED_EDGE ( 'NONE', *, *, #16847, .F. ) ;
#29178=CARTESIAN_POINT ( 'NONE',  ( 6.000000000000000888, 1.743066579297358182E-13, -102.0863248654051887 ) ) ;
#29179=ORIENTED_EDGE ( 'NONE', *, *, #5791, .T. ) ;
#29182=CARTESIAN_POINT ( 'NONE',  ( 2.775557561562891351E-14, -6.250000000000061284, -99.31698729810783277 ) ) ;
#29186=( BOUNDED_CURVE ( )  B_SPLINE_CURVE ( 2, ( #24595, #29664, #15900, #3545, #24760, #3700, #27353, #27049, #22926 ),
 .UNSPECIFIED., .F., .F. ) 
 B_SPLINE_CURVE_WITH_KNOTS ( ( 3, 2, 2, 2, 3 ),
 ( 0.8861111111111111827, 0.8870370370370370683, 0.8888888888888888395, 0.8907407407407407218, 0.8916666666666666075 ),
 .UNSPECIFIED. ) 
 CURVE ( )  GEOMETRIC_REPRESENTATION_ITEM ( )  RATIONAL_B_SPLINE_CURVE ( ( 0.9330127018922194093, 0.9330127018922234061, 1.000000000000000000, 0.8660254037844388186, 1.000000000000000000, 0.8660254037844388186, 1.000000000000000000, 0.9330127018922234061, 0.9330127018922194093 ) ) 
 REPRESENTATION_ITEM ( '' )  );
#29187=ORIENTED_EDGE ( 'NONE', *, *, #16469, .T. ) ;
#29189=CARTESIAN_POINT ( 'NONE',  ( 0.000000000000000000, -5.999999999999991118, -82.96132486540518869 ) ) ;
#29190=CARTESIAN_POINT ( 'NONE',  ( -3.175426480542816510, 5.499999999999865885, -52.37500000000002842 ) ) ;
#29193=DIRECTION ( 'NONE',  ( 1.000000000000000000, -5.551115123125773458E-17, -1.260129944081490338E-35 ) ) ;
#29194=CARTESIAN_POINT ( 'NONE',  ( 5.412658773652739619, 3.124999999999988898, -77.18301270189220986 ) ) ;
#29195=DIRECTION ( 'NONE',  ( 1.000000000000000000, -5.551115123125773458E-17, -1.260129944081490338E-35 ) ) ;
#29198=( LENGTH_UNIT ( ) NAMED_UNIT ( * ) SI_UNIT ( .MILLI., .METRE. ) );
#29200=CARTESIAN_POINT ( 'NONE',  ( 0.000000000000000000, 0.000000000000000000, 0.000000000000000000 ) ) ;
#29202=CARTESIAN_POINT ( 'NONE',  ( -3.175426480542816066, 5.499999999999865885, -128.8750000000000284 ) ) ;
#29204=CARTESIAN_POINT ( 'NONE',  ( -3.464101615137725076, 5.999999999999979572, -101.5863248654052029 ) ) ;
#29206=CARTESIAN_POINT ( 'NONE',  ( -6.350852961085760029, -1.281975124255709124E-13, -61.12500000000000000 ) ) ;
#29208=CARTESIAN_POINT ( 'NONE',  ( 4.763139720814407951, -2.749999999999988454, -59.00000000000004974 ) ) ;
#29213=VECTOR ( 'NONE', #15915, 1000.000000000000000 ) ;
#29216=ORIENTED_EDGE ( 'NONE', *, *, #16516, .F. ) ;
#29220=EDGE_LOOP ( 'NONE', ( #23421, #24666, #24239, #16458 ) ) ;
#29221=CARTESIAN_POINT ( 'NONE',  ( -6.350852961085760029, -1.281975124255709124E-13, -148.1250000000000284 ) ) ;
#29224=CARTESIAN_POINT ( 'NONE',  ( -3.608439182435052128, -6.250000000000110134, -147.4419872981078470 ) ) ;
#29225=CARTESIAN_POINT ( 'NONE',  ( -4.763139720814407951, -2.750000000000016431, -73.00000000000001421 ) ) ;
#29228=EDGE_CURVE ( 'NONE', #4337, #2765, #1250, .T. ) ;
#29229=CARTESIAN_POINT ( 'NONE',  ( -7.216878364870328078, 0.000000000000000000, -91.55801270189225249 ) ) ;
#29232=CARTESIAN_POINT ( 'NONE',  ( -3.464101615137725076, 5.999999999999979572, -98.58632486540518869 ) ) ;
#29233=DIRECTION ( 'NONE',  ( 1.000000000000000000, -5.551115123125773458E-17, -1.260129944081490338E-35 ) ) ;
#29234=CARTESIAN_POINT ( 'NONE',  ( -6.350852961085760029, -1.281975124255709124E-13, -158.6250000000000284 ) ) ;
#29236=CARTESIAN_POINT ( 'NONE',  ( -4.763139720814407951, 2.749999999999946709, -146.7500000000000568 ) ) ;
#29237=CARTESIAN_POINT ( 'NONE',  ( 3.464101615137852974, 5.999999999999884537, -76.91367513459478289 ) ) ;
#29239=CARTESIAN_POINT ( 'NONE',  ( 4.763139720814407951, -2.749999999999988454, -86.00000000000001421 ) ) ;
#29242=CARTESIAN_POINT ( 'NONE',  ( -4.763139720814407951, 2.749999999999946709, -85.25000000000004263 ) ) ;
#29244=LINE ( 'NONE', #22366, #28897 ) ;
#29245=CARTESIAN_POINT ( 'NONE',  ( -3.464101615137757051, -5.999999999999979572, -108.5863248654051887 ) ) ;
#29247=AXIS2_PLACEMENT_3D ( 'NONE', #28711, #3072, #23981 ) ;
#29248=CARTESIAN_POINT ( 'NONE',  ( -3.464101615137757051, -5.999999999999979572, -149.6636751345947971 ) ) ;
#29252=CARTESIAN_POINT ( 'NONE',  ( -5.196152422706601826, 2.999999999999975131, -138.9613248654052313 ) ) ;
#29253=ORIENTED_EDGE ( 'NONE', *, *, #8455, .T. ) ;
#29255=( NAMED_UNIT ( * ) PLANE_ANGLE_UNIT ( ) SI_UNIT ( $, .RADIAN. ) );
#29259=CARTESIAN_POINT ( 'NONE',  ( -5.196152422706573404, -3.000000000000002665, -116.2113248654052029 ) ) ;
#29263=CARTESIAN_POINT ( 'NONE',  ( -4.763139720814407951, 2.749999999999946709, -104.7500000000000142 ) ) ;
#29266=CARTESIAN_POINT ( 'NONE',  ( -5.412658773652684552, -3.125000000000099920, -116.9330127018922667 ) ) ;
#29268=LINE ( 'NONE', #24829, #14705 ) ;
#29271=CARTESIAN_POINT ( 'NONE',  ( 7.216878364870455975, -6.409875621278545621E-14, -54.80801270189220986 ) ) ;
#29272=EDGE_LOOP ( 'NONE', ( #29739, #18091, #7669, #7175, #17961, #13338, #10377, #24362, #6495, #7775, #23985, #17254, #17972, #13855, #30193, #2435, #19794, #5924, #14506, #5275, #29135, #2442, #4929, #3818, #9050, #16220, #23779, #5283, #13977, #11380, #7270, #14832, #12099, #20105, #22252, #26696, #25923, #3157, #6416, #20407, #5355, #13918, #24785, #29546, #3510, #21749, #13227, #10067, #4719, #28851, #4489, #19260, #24966, #21784, #2489, #12583, #6281, #1504, #26425, #27839, #1274, #21141, #5205, #9653, #13163, #19555, #27560, #15375, #26293, #11465, #20372, #22432, #19446, #2543, #17028, #26216, #4193, #18100, #29075, #12283, #11346, #13536, #23016, #25136, #425, #3308, #1849, #9312, #12888, #25075, #28440, #607, #18329, #18242, #26327, #21480, #27565, #19980, #30216, #4769, #29658, #27590, #25499, #580, #24882, #3676, #6196, #24926, #2687, #3343, #18623, #10481, #16965, #11252, #19633, #24322, #24736, #29511, #25189, #21986, #24960, #16162, #11220, #30037, #6090, #23032, #5232, #21145, #6455, #27073, #18297, #30067, #14450, #8790, #28050, #27795, #6082, #13202, #28801, #19047, #22461, #3044, #9802, #17454, #6707, #2395, #6120, #5054, #30313, #26247, #27406, #23067, #23663, #10451, #27123, #5961, #1110, #19756, #4542, #16862, #10599, #22941, #22112, #19878, #21450, #11061, #21372, #13439, #10848, #8967, #23277, #1308, #11714, #23943, #7924, #19076, #28401, #13239, #14230, #30342, #14332, #8815 ) ) ;
#29273=CARTESIAN_POINT ( 'NONE',  ( 0.000000000000000000, 5.999999999999977796, -167.7113248654051745 ) ) ;
#29274=CARTESIAN_POINT ( 'NONE',  ( -3.464101615137757051, -5.999999999999979572, -119.6636751345947829 ) ) ;
#29277=CARTESIAN_POINT ( 'NONE',  ( -2.775557561562891351E-14, -5.500000000000115463, -173.2500000000000284 ) ) ;
#29280=CARTESIAN_POINT ( 'NONE',  ( 2.775557561562891351E-14, -6.250000000000061284, -170.6830127018922383 ) ) ;
#29282=CARTESIAN_POINT ( 'NONE',  ( 3.175426480543072749, -5.500000000000105693, -114.6250000000000000 ) ) ;
#29284=CARTESIAN_POINT ( 'NONE',  ( 3.175426480543072749, -5.500000000000105693, -104.1250000000000142 ) ) ;
#29287=CARTESIAN_POINT ( 'NONE',  ( 5.196152422706629359, -2.999999999999988898, -87.21132486540523132 ) ) ;
#29288=LINE ( 'NONE', #27582, #19585 ) ;
#29290=EDGE_LOOP ( 'NONE', ( #17752, #1201, #8393, #25620 ) ) ;
#29296=VERTEX_POINT ( 'NONE', #14016 ) ;
#29297=CARTESIAN_POINT ( 'NONE',  ( 4.763139720814407951, -2.749999999999988454, -161.0000000000000284 ) ) ;
#29300=EDGE_CURVE ( 'NONE', #17631, #956, #4401, .T. ) ;
#29301=CARTESIAN_POINT ( 'NONE',  ( 5.412658773652712085, -3.125000000000086153, -81.06698729810779014 ) ) ;
#29305=VECTOR ( 'NONE', #5827, 1000.000000000000000 ) ;
#29306=ORIENTED_EDGE ( 'NONE', *, *, #10950, .T. ) ;
#29307=ORIENTED_EDGE ( 'NONE', *, *, #30327, .F. ) ;
#29310=VERTEX_POINT ( 'NONE', #21048 ) ;
#29311=CARTESIAN_POINT ( 'NONE',  ( 5.412658773652739619, 3.124999999999988898, -122.8169872981078612 ) ) ;
#29312=CARTESIAN_POINT ( 'NONE',  ( -4.763139720814407951, 2.749999999999946709, -169.2500000000000000 ) ) ;
#29313=CARTESIAN_POINT ( 'NONE',  ( 6.000000000000000888, -1.607695154586752384, -167.2306624327026157 ) ) ;
#29315=EDGE_LOOP ( 'NONE', ( #13418, #4147, #28241, #24678 ) ) ;
#29317=CARTESIAN_POINT ( 'NONE',  ( 0.000000000000000000, 5.999999999999977796, -163.7886751345948255 ) ) ;
#29318=CARTESIAN_POINT ( 'NONE',  ( 0.000000000000000000, 5.999999999999977796, -56.71132486540520290 ) ) ;
#29320=CARTESIAN_POINT ( 'NONE',  ( 3.464101615137757051, -5.999999999999979572, -54.91367513459480421 ) ) ;
#29323=CARTESIAN_POINT ( 'NONE',  ( -3.608439182435115633, 6.249999999999965361, -65.44198729810786119 ) ) ;
#29324=CARTESIAN_POINT ( 'NONE',  ( -3.608439182435052128, -6.250000000000110134, -57.44198729810781856 ) ) ;
#29325=CARTESIAN_POINT ( 'NONE',  ( 5.196152422706629359, -2.999999999999988898, -120.7886751345948539 ) ) ;
#29328=CARTESIAN_POINT ( 'NONE',  ( 6.000000000000000888, -1.859271017917181981E-14, -120.6636751345948255 ) ) ;
#29329=CARTESIAN_POINT ( 'NONE',  ( -6.350852961085760029, -1.281975124255709124E-13, -131.6250000000000284 ) ) ;
#29331=CARTESIAN_POINT ( 'NONE',  ( -5.999999999999963585, -1.487416814333745711E-14, -166.4136751345948539 ) ) ;
#29334=CARTESIAN_POINT ( 'NONE',  ( -5.999999999999963585, 0.000000000000000000, -179.9136751345948255 ) ) ;
#29335=CARTESIAN_POINT ( 'NONE',  ( 6.000000000000000000, 2.951592740943527306E-14, -155.1636751345948539 ) ) ;
#29341=CARTESIAN_POINT ( 'NONE',  ( 2.775557561562891351E-14, 6.250000000000033751, -118.0669872981078328 ) ) ;
#29342=CARTESIAN_POINT ( 'NONE',  ( 6.000000000000000888, -1.607695154586752384, -173.2306624327026441 ) ) ;
#29350=CARTESIAN_POINT ( 'NONE',  ( 4.763139720814407951, 2.750000000000002665, -49.75000000000001421 ) ) ;
#29352=CARTESIAN_POINT ( 'NONE',  ( 0.000000000000000000, -5.999999999999991118, -59.53867513459481842 ) ) ;
#29353=DIRECTION ( 'NONE',  ( -7.147005652999508048E-36, 5.642372883946980038E-36, 1.000000000000000000 ) ) ;
#29354=CARTESIAN_POINT ( 'NONE',  ( 3.608439182435180470, 6.249999999999982236, -75.55801270189225249 ) ) ;
#29357=DIRECTION ( 'NONE',  ( 1.000000000000000000, -5.551115123125773458E-17, -1.260129944081490338E-35 ) ) ;
#29360=CARTESIAN_POINT ( 'NONE',  ( -5.196152422706601826, 2.999999999999975131, -104.4613248654052171 ) ) ;
#29361=CARTESIAN_POINT ( 'NONE',  ( 3.175426480543072749, 5.499999999999865885, -132.1250000000000284 ) ) ;
#29365=CARTESIAN_POINT ( 'NONE',  ( 4.763139720814407951, -2.749999999999988454, -65.00000000000000000 ) ) ;
#29366=CARTESIAN_POINT ( 'NONE',  ( -4.763139720814407951, -2.750000000000016431, -58.00000000000004974 ) ) ;
#29368=ORIENTED_EDGE ( 'NONE', *, *, #2547, .F. ) ;
#29373=EDGE_CURVE ( 'NONE', #22801, #25470, #3995, .T. ) ;
#29374=DIRECTION ( 'NONE',  ( -7.147005652999508048E-36, 5.642372883946980038E-36, 1.000000000000000000 ) ) ;
#29376=VERTEX_POINT ( 'NONE', #10273 ) ;
#29377=CARTESIAN_POINT ( 'NONE',  ( -5.999999999999956479, -1.607695154586745057, -122.2693375672974128 ) ) ;
#29380=CARTESIAN_POINT ( 'NONE',  ( 0.000000000000000000, 5.499999999999991118, -148.5000000000000284 ) ) ;
#29382=CARTESIAN_POINT ( 'NONE',  ( 7.216878364870455975, -6.409875621278545621E-14, -47.94198729810783277 ) ) ;
#29385=CARTESIAN_POINT ( 'NONE',  ( 2.775557561562891351E-14, -6.250000000000061284, -150.3169872981078186 ) ) ;
#29386=CARTESIAN_POINT ( 'NONE',  ( -3.175426480542816510, 5.499999999999865885, -73.37500000000000000 ) ) ;
#29387=CARTESIAN_POINT ( 'NONE',  ( 5.412658773652739619, 3.124999999999988898, -96.68301270189222407 ) ) ;
#29388=CARTESIAN_POINT ( 'NONE',  ( -4.763139720814407951, -2.750000000000016431, -152.5000000000000284 ) ) ;
#29389=CARTESIAN_POINT ( 'NONE',  ( -5.196552517144552574, -9.698180938751621127, -21.97571210926416541 ) ) ;
#29390=DIRECTION ( 'NONE',  ( -7.147005652999508048E-36, 5.642372883946980038E-36, 1.000000000000000000 ) ) ;
#29391=FACE_OUTER_BOUND ( 'NONE', #6696, .T. ) ;
#29392=CARTESIAN_POINT ( 'NONE',  ( -6.000000000000007105, -1.607695154586655129, -91.34668783648704959 ) ) ;
#29393=CYLINDRICAL_SURFACE ( 'NONE', #1946, 6.000000000000000888 ) ;
#29394=CARTESIAN_POINT ( 'NONE',  ( -4.763139720814407951, 2.749999999999946709, -158.7500000000000568 ) ) ;
#29395=CARTESIAN_POINT ( 'NONE',  ( -3.175426480542816510, 5.499999999999865885, -145.3750000000000000 ) ) ;
#29397=UNCERTAINTY_MEASURE_WITH_UNIT (LENGTH_MEASURE( 1.000000000000000082E-05 ), #18830, 'distance_accuracy_value', 'NONE');
#29399=CARTESIAN_POINT ( 'NONE',  ( -4.763139720814407951, -2.750000000000016431, -89.50000000000002842 ) ) ;
#29401=CARTESIAN_POINT ( 'NONE',  ( 3.175426480543072749, 5.499999999999865885, -81.12500000000002842 ) ) ;
#29406=CARTESIAN_POINT ( 'NONE',  ( 6.000000000000000888, -1.859271017917181981E-14, -125.1636751345948397 ) ) ;
#29407=EDGE_CURVE ( 'NONE', #21222, #24216, #10720, .T. ) ;
#29409=CARTESIAN_POINT ( 'NONE',  ( 6.000000000000000888, -3.330669073875464691E-16, -7.560779664488942560E-35 ) ) ;
#29412=CARTESIAN_POINT ( 'NONE',  ( 5.999999999999949374, 1.607695154586804565, -91.51933756729745539 ) ) ;
#29413=CARTESIAN_POINT ( 'NONE',  ( 5.999999999999949374, 1.607695154586804565, -73.51933756729744118 ) ) ;
#29419=CARTESIAN_POINT ( 'NONE',  ( 3.175426480543072749, -5.500000000000105693, -95.12500000000002842 ) ) ;
#29421=CARTESIAN_POINT ( 'NONE',  ( 5.412658773652739619, 3.124999999999988898, -111.6830127018922383 ) ) ;
#29423=CYLINDRICAL_SURFACE ( 'NONE', #27908, 6.000000000000000888 ) ;
#29427=CARTESIAN_POINT ( 'NONE',  ( -3.608439182435052128, -6.250000000000110134, -52.30801270189225249 ) ) ;
#29428=EDGE_LOOP ( 'NONE', ( #26953, #6698, #12766, #26983 ) ) ;
#29430=CARTESIAN_POINT ( 'NONE',  ( 6.000000000000000888, -1.859271017917181981E-14, -136.5863248654051745 ) ) ;
#29432=CARTESIAN_POINT ( 'NONE',  ( -4.763139720814407951, -2.750000000000016431, -173.5000000000000000 ) ) ;
#29435=CARTESIAN_POINT ( 'NONE',  ( -7.216878364870328078, 0.000000000000000000, -159.0580127018922383 ) ) ;
#29436=CARTESIAN_POINT ( 'NONE',  ( -3.464101615137725076, 5.999999999999979572, -48.16367513459483973 ) ) ;
#29437=CARTESIAN_POINT ( 'NONE',  ( -4.763139720814407951, 2.749999999999946709, -106.2500000000000142 ) ) ;
#29439=CARTESIAN_POINT ( 'NONE',  ( -4.763139720814407951, 2.749999999999946709, -107.7500000000000142 ) ) ;
#29440=CARTESIAN_POINT ( 'NONE',  ( 5.196152422706629359, 3.000000000000002665, -152.0386751345948539 ) ) ;
#29442=CARTESIAN_POINT ( 'NONE',  ( 5.196152422706629359, 3.000000000000002665, -145.4613248654052029 ) ) ;
#29444=CARTESIAN_POINT ( 'NONE',  ( 3.464101615137757051, -5.999999999999979572, -90.33632486540521711 ) ) ;
#29447=ADVANCED_FACE ( 'NONE', ( #7204 ), #14460, .T. ) ;
#29448=ORIENTED_EDGE ( 'NONE', *, *, #3740, .F. ) ;
#29449=CARTESIAN_POINT ( 'NONE',  ( 0.000000000000000000, 5.499999999999991118, -160.5000000000000284 ) ) ;
#29450=CARTESIAN_POINT ( 'NONE',  ( 0.000000000000000000, 5.999999999999977796, -65.71132486540520290 ) ) ;
#29452=CARTESIAN_POINT ( 'NONE',  ( 2.775557561562891351E-14, -6.250000000000061284, -82.81698729810781856 ) ) ;
#29455=CARTESIAN_POINT ( 'NONE',  ( 6.000000000000000888, -1.859271017917181981E-14, -125.1636751345948397 ) ) ;
#29456=CIRCLE ( 'NONE', #17727, 6.000000000000009770 ) ;
#29460=CARTESIAN_POINT ( 'NONE',  ( 3.175426480543072749, -5.500000000000105693, -122.1250000000000284 ) ) ;
#29462=CARTESIAN_POINT ( 'NONE',  ( 5.412658773652739619, 3.124999999999988898, -135.6830127018922667 ) ) ;
#29465=CARTESIAN_POINT ( 'NONE',  ( 5.412658773652712085, -3.125000000000086153, -120.0669872981078328 ) ) ;
#29466=CARTESIAN_POINT ( 'NONE',  ( 3.175426480543072749, -5.500000000000105693, -174.6250000000000284 ) ) ;
#29469=CARTESIAN_POINT ( 'NONE',  ( -5.196152422706601826, 2.999999999999975131, -47.46132486540521711 ) ) ;
#29473=FACE_OUTER_BOUND ( 'NONE', #10408, .T. ) ;
#29476=CARTESIAN_POINT ( 'NONE',  ( 5.196152422706629359, -2.999999999999988898, -54.78867513459484684 ) ) ;
#29478=CARTESIAN_POINT ( 'NONE',  ( -5.196152422706573404, -3.000000000000002665, -47.21132486540524553 ) ) ;
#29480=CARTESIAN_POINT ( 'NONE',  ( -3.608439182435052128, -6.250000000000110134, -66.44198729810784698 ) ) ;
#29481=CARTESIAN_POINT ( 'NONE',  ( -5.412658773652739619, 3.124999999999975131, -56.31698729810785409 ) ) ;
#29482=EDGE_CURVE ( 'NONE', #24216, #17631, #2590, .T. ) ;
#29484=CARTESIAN_POINT ( 'NONE',  ( -6.000000000000007105, -1.607695154586655129, -64.34668783648703538 ) ) ;
#29487=CARTESIAN_POINT ( 'NONE',  ( -4.763139720814407951, 2.749999999999946709, -125.7500000000000284 ) ) ;
#29489=AXIS2_PLACEMENT_3D ( 'NONE', #3400, #8482, #27209 ) ;
#29490=ORIENTED_EDGE ( 'NONE', *, *, #15461, .F. ) ;
#29491=CARTESIAN_POINT ( 'NONE',  ( -5.999999999999963585, 8.134310703387671600E-14, -119.3363248654052455 ) ) ;
#29493=CARTESIAN_POINT ( 'NONE',  ( 0.000000000000000000, 5.999999999999977796, -97.21132486540517448 ) ) ;
#29499=DIRECTION ( 'NONE',  ( 1.000000000000000000, -5.551115123125773458E-17, -1.260129944081490338E-35 ) ) ;
#29501=CARTESIAN_POINT ( 'NONE',  ( 5.412658773652712085, -3.125000000000086153, -112.5669872981078186 ) ) ;
#29506=ORIENTED_EDGE ( 'NONE', *, *, #7474, .T. ) ;
#29507=VERTEX_POINT ( 'NONE', #12305 ) ;
#29511=ORIENTED_EDGE ( 'NONE', *, *, #20597, .T. ) ;
#29513=CARTESIAN_POINT ( 'NONE',  ( 3.175426480543072749, -5.500000000000105693, -50.12500000000001421 ) ) ;
#29516=CARTESIAN_POINT ( 'NONE',  ( -7.216878364870328078, 0.000000000000000000, -76.55801270189223828 ) ) ;
#29520=CARTESIAN_POINT ( 'NONE',  ( 0.000000000000000000, 5.999999999999977796, -177.2886751345948539 ) ) ;
#29526=LINE ( 'NONE', #2038, #10866 ) ;
#29527=CARTESIAN_POINT ( 'NONE',  ( -4.763139720814407951, 2.749999999999946709, -130.2500000000000284 ) ) ;
#29528=CARTESIAN_POINT ( 'NONE',  ( -5.196152422706601826, 2.999999999999975131, -68.46132486540523132 ) ) ;
#29529=CARTESIAN_POINT ( 'NONE',  ( 2.775557561562891351E-14, -6.250000000000061284, -146.6830127018922099 ) ) ;
#29530=DIRECTION ( 'NONE',  ( -7.147005652999508048E-36, 5.642372883946980038E-36, 1.000000000000000000 ) ) ;
#29531=CARTESIAN_POINT ( 'NONE',  ( 5.196152422706629359, 3.000000000000002665, -178.4613248654052313 ) ) ;
#29534=CARTESIAN_POINT ( 'NONE',  ( -4.763139720814407951, -2.750000000000016431, -64.00000000000000000 ) ) ;
#29542=CARTESIAN_POINT ( 'NONE',  ( 3.464101615137757051, -5.999999999999979572, -48.91367513459484684 ) ) ;
#29543=ORIENTED_EDGE ( 'NONE', *, *, #6216, .T. ) ;
#29546=ORIENTED_EDGE ( 'NONE', *, *, #4895, .T. ) ;
#29547=B_SPLINE_CURVE_WITH_KNOTS ( 'NONE', 3,
 ( #13503, #22843, #20537, #8867, #18860, #22004, #7860, #21860, #2951, #16569, #9163, #5548, #9318, #24005, #24153, #28034, #16278, #92, #12367, #18556, #28740, #19560, #7004, #25596, #26297, #27881, #7712, #21717, #805, #11815, #23466, #12523, #28895, #25745, #16423, #4692, #21153, #5252 ),
 .UNSPECIFIED., .F., .F.,
 ( 4, 2, 2, 2, 2, 2, 2, 2, 2, 2, 2, 2, 2, 2, 2, 2, 2, 2, 4 ),
 ( 0.01915730813553682965, 0.01975454893833632555, 0.02035178974113582145, 0.02154627134673480979, 0.02274075295233380159, 0.02393523455793278992, 0.02512971616353178173, 0.02632419776913077353, 0.02751867937472976533, 0.02871316098032875713, 0.02990764258592774893, 0.03110212419152673727, 0.03229660579712572560, 0.03349108740272471740, 0.03468556900832370227, 0.03528280981112319470, 0.03588005061392269407, 0.03707453221952168587, 0.03826901382512067074 ),
 .UNSPECIFIED. ) ;
#29548=CARTESIAN_POINT ( 'NONE',  ( -2.775557561562891351E-14, -5.500000000000115463, -141.7500000000000568 ) ) ;
#29549=CARTESIAN_POINT ( 'NONE',  ( 3.608439182435180470, 6.249999999999982236, -47.69198729810783277 ) ) ;
#29551=ORIENTED_EDGE ( 'NONE', *, *, #11975, .F. ) ;
#29552=CARTESIAN_POINT ( 'NONE',  ( -3.175426480542816510, -5.500000000000057732, -75.87500000000001421 ) ) ;
#29554=CARTESIAN_POINT ( 'NONE',  ( -5.412658773652739619, 3.124999999999975131, -96.18301270189222407 ) ) ;
#29556=CARTESIAN_POINT ( 'NONE',  ( -2.687256737965178832, -10.66819377212465447, -30.36813770228164699 ) ) ;
#29558=CARTESIAN_POINT ( 'NONE',  ( 5.999999999999999112, 2.951592740943527306E-14, -150.6636751345948539 ) ) ;
#29561=CARTESIAN_POINT ( 'NONE',  ( -2.775557561562891351E-14, -5.500000000000115463, -158.2500000000000000 ) ) ;
#29562=DIRECTION ( 'NONE',  ( 1.000000000000000000, -5.551115123125773458E-17, -1.260129944081490338E-35 ) ) ;
#29563=CARTESIAN_POINT ( 'NONE',  ( -3.106370373191974732, 4.832402510093865899, -180.0000000000000853 ) ) ;
#29564=CARTESIAN_POINT ( 'NONE',  ( 3.175426480543072749, 5.499999999999865885, -85.62500000000000000 ) ) ;
#29566=ADVANCED_FACE ( 'NONE', ( #13059 ), #12750, .T. ) ;
#29567=CARTESIAN_POINT ( 'NONE',  ( 4.763139720814407951, -2.749999999999988454, -74.00000000000001421 ) ) ;
#29568=( BOUNDED_CURVE ( )  B_SPLINE_CURVE ( 2, ( #19350, #17354, #21650, #5185, #12600, #17203, #2886, #21504, #26669 ),
 .UNSPECIFIED., .F., .T. ) 
 B_SPLINE_CURVE_WITH_KNOTS ( ( 3, 2, 2, 2, 3 ),
 ( 0.3972222222222222543, 0.3981481481481481399, 0.4000000000000000222, 0.4018518518518519045, 0.4027777777777777901 ),
 .UNSPECIFIED. ) 
 CURVE ( )  GEOMETRIC_REPRESENTATION_ITEM ( )  RATIONAL_B_SPLINE_CURVE ( ( 0.9330127018922194093, 0.9330127018922234061, 1.000000000000000000, 0.8660254037844388186, 1.000000000000000000, 0.8660254037844388186, 1.000000000000000000, 0.9330127018922194093, 0.9330127018922194093 ) ) 
 REPRESENTATION_ITEM ( '' )  );
#29571=CYLINDRICAL_SURFACE ( 'NONE', #21694, 6.000000000000000888 ) ;
#29573=CARTESIAN_POINT ( 'NONE',  ( 6.000000000000000888, 1.743066579297358182E-13, -106.5863248654052313 ) ) ;
#29575=CARTESIAN_POINT ( 'NONE',  ( 3.464101615137852974, 5.999999999999884537, -124.9136751345948113 ) ) ;
#29580=DIRECTION ( 'NONE',  ( -7.147005652999508048E-36, 5.642372883946980038E-36, 1.000000000000000000 ) ) ;
#29581=CARTESIAN_POINT ( 'NONE',  ( 6.000000000000000888, -1.607695154586752384, -171.7306624327026157 ) ) ;
#29585=CARTESIAN_POINT ( 'NONE',  ( 0.000000000000000000, 5.499999999999991118, -96.00000000000002842 ) ) ;
#29587=CARTESIAN_POINT ( 'NONE',  ( 6.000000000000000888, -3.330669073875464691E-16, -7.560779664488942560E-35 ) ) ;
#29588=CARTESIAN_POINT ( 'NONE',  ( 2.775557561562891351E-14, -6.250000000000061284, -118.1830127018922383 ) ) ;
#29590=CARTESIAN_POINT ( 'NONE',  ( 5.196152422706629359, 3.000000000000002665, -94.46132486540520290 ) ) ;
#29594=CARTESIAN_POINT ( 'NONE',  ( 2.775557561562891351E-14, -6.250000000000061284, -53.68301270189223828 ) ) ;
#29597=EDGE_CURVE ( 'NONE', #4074, #7068, #3322, .T. ) ;
#29598=CARTESIAN_POINT ( 'NONE',  ( 6.350852961086080661, -9.614813431917819062E-14, -162.3750000000000284 ) ) ;
#29600=CARTESIAN_POINT ( 'NONE',  ( 6.000000000000052403, -1.607695154586662678, -157.6533121635129362 ) ) ;
#29601=CARTESIAN_POINT ( 'NONE',  ( 6.350852961086080661, -9.614813431917819062E-14, -111.3750000000000426 ) ) ;
#29603=CARTESIAN_POINT ( 'NONE',  ( -2.775557561562891351E-14, -5.500000000000115463, -104.2500000000000142 ) ) ;
#29605=CARTESIAN_POINT ( 'NONE',  ( 5.196152422706629359, 3.000000000000002665, -118.4613248654052313 ) ) ;
#29610=CARTESIAN_POINT ( 'NONE',  ( -5.196152422706573404, -3.000000000000002665, -134.2113248654052029 ) ) ;
#29611=CARTESIAN_POINT ( 'NONE',  ( -3.175426480542816510, 5.499999999999865885, -158.8750000000000000 ) ) ;
#29614=CARTESIAN_POINT ( 'NONE',  ( 2.775557561562891351E-14, -6.250000000000061284, -88.81698729810783277 ) ) ;
#29615=ORIENTED_EDGE ( 'NONE', *, *, #16341, .F. ) ;
#29616=CARTESIAN_POINT ( 'NONE',  ( 0.000000000000000000, 0.000000000000000000, 0.000000000000000000 ) ) ;
#29617=ORIENTED_EDGE ( 'NONE', *, *, #24664, .F. ) ;
#29619=CARTESIAN_POINT ( 'NONE',  ( -2.775557561562891351E-14, -5.500000000000115463, -119.2500000000000284 ) ) ;
#29620=CARTESIAN_POINT ( 'NONE',  ( -3.608439182435052128, -6.250000000000110134, -142.3080127018922667 ) ) ;
#29623=CARTESIAN_POINT ( 'NONE',  ( 2.775557561562891351E-14, -6.250000000000061284, -124.8169872981078612 ) ) ;
#29624=CARTESIAN_POINT ( 'NONE',  ( 2.775557561562891351E-14, -6.250000000000061284, -177.3169872981078470 ) ) ;
#29625=CARTESIAN_POINT ( 'NONE',  ( 4.763139720814407951, -2.749999999999988454, -174.5000000000000000 ) ) ;
#29630=DIRECTION ( 'NONE',  ( 1.000000000000000000, -5.551115123125773458E-17, -1.260129944081490338E-35 ) ) ;
#29632=CARTESIAN_POINT ( 'NONE',  ( -5.999999999999963585, -1.487416814333745711E-14, -170.9136751345948255 ) ) ;
#29634=CARTESIAN_POINT ( 'NONE',  ( -3.608439182435115633, 6.249999999999965361, -71.44198729810781856 ) ) ;
#29635=CARTESIAN_POINT ( 'NONE',  ( -5.412658773652739619, 3.124999999999975131, -57.81698729810780435 ) ) ;
#29636=CARTESIAN_POINT ( 'NONE',  ( 0.000000000000000000, 0.000000000000000000, 0.000000000000000000 ) ) ;
#29637=CARTESIAN_POINT ( 'NONE',  ( -4.763139720814407951, -2.750000000000016431, -49.00000000000004263 ) ) ;
#29640=CARTESIAN_POINT ( 'NONE',  ( 3.175426480543072749, 5.499999999999865885, -132.1250000000000284 ) ) ;
#29641=CARTESIAN_POINT ( 'NONE',  ( -5.999999999999963585, 1.780251999655701777E-13, -85.41367513459483973 ) ) ;
#29642=ORIENTED_EDGE ( 'NONE', *, *, #1174, .T. ) ;
#29645=CARTESIAN_POINT ( 'NONE',  ( -5.999999999999963585, -1.487416814333745711E-14, -50.91367513459483973 ) ) ;
#29650=CARTESIAN_POINT ( 'NONE',  ( 5.412658773652739619, 3.124999999999988898, -113.8169872981078470 ) ) ;
#29653=CARTESIAN_POINT ( 'NONE',  ( 6.000000000000000888, -3.330669073875464691E-16, -7.560779664488942560E-35 ) ) ;
#29658=ORIENTED_EDGE ( 'NONE', *, *, #21742, .T. ) ;
#29661=CARTESIAN_POINT ( 'NONE',  ( 3.175426480543072749, 5.499999999999865885, -49.62500000000001421 ) ) ;
#29663=CARTESIAN_POINT ( 'NONE',  ( 6.000000000000000888, -1.859271017917181981E-14, -141.6636751345948255 ) ) ;
#29664=CARTESIAN_POINT ( 'NONE',  ( 5.999999999999949374, 1.607695154586804565, -62.09668783648702117 ) ) ;
#29665=CARTESIAN_POINT ( 'NONE',  ( -3.608439182435052128, -6.250000000000110134, -70.30801270189220986 ) ) ;
#29670=DIRECTION ( 'NONE',  ( -7.147005652999508048E-36, 5.642372883946980038E-36, 1.000000000000000000 ) ) ;
#29673=CARTESIAN_POINT ( 'NONE',  ( 5.196152422706629359, 3.000000000000002665, -115.4613248654052171 ) ) ;
#29674=CARTESIAN_POINT ( 'NONE',  ( -4.763139720814407951, 2.749999999999946709, -134.7500000000000284 ) ) ;
#29677=CARTESIAN_POINT ( 'NONE',  ( 3.175426480543072749, -5.500000000000105693, -63.62500000000001421 ) ) ;
#29678=DIRECTION ( 'NONE',  ( -7.147005652999508048E-36, 5.642372883946980038E-36, 1.000000000000000000 ) ) ;
#29679=CARTESIAN_POINT ( 'NONE',  ( 6.000000000000000888, -1.859271017917181981E-14, -172.5863248654052029 ) ) ;
#29680=CARTESIAN_POINT ( 'NONE',  ( -5.999999999999964473, 9.063946212346262433E-15, -174.8363248654052313 ) ) ;
#29692=CARTESIAN_POINT ( 'NONE',  ( -4.763139720814407951, 2.749999999999946709, -148.2500000000000000 ) ) ;
#29695=ORIENTED_EDGE ( 'NONE', *, *, #19184, .T. ) ;
#29696=CARTESIAN_POINT ( 'NONE',  ( -6.350852961085760029, -1.281975124255709124E-13, -71.62500000000005684 ) ) ;
#29698=CARTESIAN_POINT ( 'NONE',  ( -5.412658773652684552, -3.125000000000099920, -89.93301270189223828 ) ) ;
#29703=CARTESIAN_POINT ( 'NONE',  ( 0.000000000000000000, 5.999999999999977796, -46.78867513459483973 ) ) ;
#29707=CARTESIAN_POINT ( 'NONE',  ( 6.350852961086080661, -9.614813431917819062E-14, -157.8750000000000284 ) ) ;
#29708=CARTESIAN_POINT ( 'NONE',  ( -6.000000000000000888, 1.067854986875958443E-15, 7.560779664488942560E-35 ) ) ;
#29709=CARTESIAN_POINT ( 'NONE',  ( -5.196152422706601826, 2.999999999999975131, -48.96132486540521711 ) ) ;
#29711=CARTESIAN_POINT ( 'NONE',  ( 3.175426480543072749, 5.499999999999865885, -90.12500000000001421 ) ) ;
#29712=CARTESIAN_POINT ( 'NONE',  ( 4.763139720814407951, 2.750000000000002665, -70.75000000000002842 ) ) ;
#29713=DIRECTION ( 'NONE',  ( -7.147005652999508048E-36, 5.642372883946980038E-36, 1.000000000000000000 ) ) ;
#29716=CARTESIAN_POINT ( 'NONE',  ( 3.464101615137852974, 5.999999999999884537, -118.9136751345948397 ) ) ;
#29718=LINE ( 'NONE', #15490, #4653 ) ;
#29723=EDGE_CURVE ( 'NONE', #20406, #21808, #15003, .T. ) ;
#29724=FACE_OUTER_BOUND ( 'NONE', #30379, .T. ) ;
#29728=CARTESIAN_POINT ( 'NONE',  ( 0.000000000000000000, 5.499999999999991118, -94.50000000000002842 ) ) ;
#29729=CARTESIAN_POINT ( 'NONE',  ( 3.464101615137852974, 5.999999999999884537, -96.41367513459479710 ) ) ;
#29731=CARTESIAN_POINT ( 'NONE',  ( 2.775557561562891351E-14, 6.250000000000033751, -112.9330127018922667 ) ) ;
#29738=CARTESIAN_POINT ( 'NONE',  ( 2.775557561562891351E-14, -6.250000000000061284, -49.18301270189223828 ) ) ;
#29739=ORIENTED_EDGE ( 'NONE', *, *, #22885, .T. ) ;
#29742=CARTESIAN_POINT ( 'NONE',  ( -5.999999999999866773, 1.607695154586893826, -135.9033121635129930 ) ) ;
#29743=CARTESIAN_POINT ( 'NONE',  ( 4.763139720814407951, -2.749999999999988454, -164.0000000000000284 ) ) ;
#29746=CARTESIAN_POINT ( 'NONE',  ( 3.175426480543072749, 5.499999999999865885, -108.1250000000000284 ) ) ;
#29748=CARTESIAN_POINT ( 'NONE',  ( -5.999999999999956479, -1.607695154586745057, -122.8466878364870496 ) ) ;
#29749=CARTESIAN_POINT ( 'NONE',  ( 6.350852961086080661, -9.614813431917819062E-14, -99.37499999999998579 ) ) ;
#29750=CARTESIAN_POINT ( 'NONE',  ( -3.464101615137757051, -5.999999999999979572, -112.1636751345948113 ) ) ;
#29751=CARTESIAN_POINT ( 'NONE',  ( -6.000000000000007105, -1.607695154586655129, -82.34668783648702117 ) ) ;
#29755=CARTESIAN_POINT ( 'NONE',  ( 0.000000000000000000, 0.000000000000000000, 0.000000000000000000 ) ) ;
#29759=CARTESIAN_POINT ( 'NONE',  ( 2.775557561562891351E-14, -6.250000000000061284, -87.31698729810783277 ) ) ;
#29760=ADVANCED_FACE ( 'NONE', ( #14413 ), #969, .T. ) ;
#29762=ORIENTED_EDGE ( 'NONE', *, *, #3301, .T. ) ;
#29768=VERTEX_POINT ( 'NONE', #26177 ) ;
#29770=CARTESIAN_POINT ( 'NONE',  ( 4.763139720814407951, -2.749999999999988454, -119.0000000000000000 ) ) ;
#29771=EDGE_CURVE ( 'NONE', #9697, #84, #7538, .T. ) ;
#29772=CARTESIAN_POINT ( 'NONE',  ( -5.412658773652739619, 3.124999999999975131, -139.6830127018922099 ) ) ;
#29774=CARTESIAN_POINT ( 'NONE',  ( 2.775557561562891351E-14, 6.250000000000033751, -119.5669872981078328 ) ) ;
#29775=CARTESIAN_POINT ( 'NONE',  ( -3.608439182435115633, 6.249999999999965361, -176.4419872981078470 ) ) ;
#29777=CARTESIAN_POINT ( 'NONE',  ( 0.000000000000000000, 5.499999999999991118, -172.5000000000000000 ) ) ;
#29778=CARTESIAN_POINT ( 'NONE',  ( -5.999999999999962697, 3.323446944526963891E-14, -151.4136751345948255 ) ) ;
#29779=CARTESIAN_POINT ( 'NONE',  ( 6.000000000000000888, -1.859271017917181981E-14, -147.6636751345948255 ) ) ;
#29784=AXIS2_PLACEMENT_3D ( 'NONE', #26476, #11974, #7597 ) ;
#29785=CARTESIAN_POINT ( 'NONE',  ( -5.999999999999963585, 1.780251999655701777E-13, -107.9136751345948397 ) ) ;
#29786=CARTESIAN_POINT ( 'NONE',  ( 6.000000000000052403, -1.607695154586662678, -150.1533121635129646 ) ) ;
#29787=CARTESIAN_POINT ( 'NONE',  ( 2.775557561562891351E-14, -6.250000000000061284, -75.31698729810781856 ) ) ;
#29788=CARTESIAN_POINT ( 'NONE',  ( 5.412658773652739619, 3.124999999999988898, -59.81698729810780435 ) ) ;
#29789=CARTESIAN_POINT ( 'NONE',  ( 0.000000000000000000, 5.999999999999977796, -110.7113248654052455 ) ) ;
#29790=CARTESIAN_POINT ( 'NONE',  ( 3.175426480543072749, -5.500000000000105693, -51.62500000000001421 ) ) ;
#29793=CARTESIAN_POINT ( 'NONE',  ( -3.175426480542816510, -5.500000000000057732, -122.3749999999999716 ) ) ;
#29794=ORIENTED_EDGE ( 'NONE', *, *, #22328, .F. ) ;
#29795=CARTESIAN_POINT ( 'NONE',  ( 5.196152422706629359, 3.000000000000002665, -132.5386751345948255 ) ) ;
#29796=( BOUNDED_CURVE ( )  B_SPLINE_CURVE ( 2, ( #8711, #13933, #1322, #19922, #10887, #12896, #1632, #6240, #10734 ),
 .UNSPECIFIED., .F., .F. ) 
 B_SPLINE_CURVE_WITH_KNOTS ( ( 3, 2, 2, 2, 3 ),
 ( 0.6972222222222221877, 0.6981481481481481843, 0.6999999999999999556, 0.7018518518518518379, 0.7027777777777777235 ),
 .UNSPECIFIED. ) 
 CURVE ( )  GEOMETRIC_REPRESENTATION_ITEM ( )  RATIONAL_B_SPLINE_CURVE ( ( 0.9330127018922194093, 0.9330127018922154125, 1.000000000000000000, 0.8660254037844388186, 1.000000000000000000, 0.8660254037844388186, 1.000000000000000000, 0.9330127018922234061, 0.9330127018922194093 ) ) 
 REPRESENTATION_ITEM ( '' )  );
#29797=CARTESIAN_POINT ( 'NONE',  ( 3.464101615137852974, 5.999999999999884537, -105.4136751345947971 ) ) ;
#29798=DIRECTION ( 'NONE',  ( -7.147005652999508048E-36, 5.642372883946980038E-36, 1.000000000000000000 ) ) ;
#29803=CARTESIAN_POINT ( 'NONE',  ( 5.412658773652739619, 3.124999999999988898, -116.8169872981078612 ) ) ;
#29804=EDGE_CURVE ( 'NONE', #2708, #8939, #10717, .T. ) ;
#29805=CARTESIAN_POINT ( 'NONE',  ( 3.464101615137757051, -5.999999999999979572, -109.8363248654051745 ) ) ;
#29816=CARTESIAN_POINT ( 'NONE',  ( -3.175426480542816510, 5.499999999999865885, -49.37500000000000711 ) ) ;
#29820=CARTESIAN_POINT ( 'NONE',  ( -3.608439182435052128, -6.250000000000110134, -64.30801270189225249 ) ) ;
#29822=CARTESIAN_POINT ( 'NONE',  ( 5.196152422706629359, 3.000000000000002665, -177.5386751345948255 ) ) ;
#29823=FILL_AREA_STYLE ('',( #17891 ) ) ;
#29824=CARTESIAN_POINT ( 'NONE',  ( -5.196152422706601826, 2.999999999999975131, -165.0386751345947971 ) ) ;
#29828=CARTESIAN_POINT ( 'NONE',  ( -3.175426480542816066, 5.499999999999865885, -122.8749999999999716 ) ) ;
#29829=DIRECTION ( 'NONE',  ( -7.147005652999508048E-36, 5.642372883946980038E-36, 1.000000000000000000 ) ) ;
#29830=CARTESIAN_POINT ( 'NONE',  ( -5.412658773652739619, 3.124999999999975131, -145.6830127018922099 ) ) ;
#29833=CARTESIAN_POINT ( 'NONE',  ( 3.175426480543072749, 5.499999999999865885, -64.62500000000001421 ) ) ;
#29835=CARTESIAN_POINT ( 'NONE',  ( 3.464101615137852974, 5.999999999999884537, -172.3363248654052029 ) ) ;
#29837=VERTEX_POINT ( 'NONE', #13431 ) ;
#29841=LINE ( 'NONE', #6801, #4266 ) ;
#29844=DIRECTION ( 'NONE',  ( -7.147005652999508048E-36, 5.642372883946980038E-36, 1.000000000000000000 ) ) ;
#29846=CARTESIAN_POINT ( 'NONE',  ( 3.175426480543072749, 5.499999999999865885, -142.6250000000000000 ) ) ;
#29847=ORIENTED_EDGE ( 'NONE', *, *, #17380, .F. ) ;
#29849=VERTEX_POINT ( 'NONE', #18185 ) ;
#29850=CARTESIAN_POINT ( 'NONE',  ( -3.175426480542816510, -5.500000000000057732, -74.37500000000000000 ) ) ;
#29852=CARTESIAN_POINT ( 'NONE',  ( 2.775557561562891351E-14, 6.250000000000033751, -87.43301270189223828 ) ) ;
#29853=CARTESIAN_POINT ( 'NONE',  ( 6.000000000000000888, 1.743066579297358182E-13, -111.0863248654051887 ) ) ;
#29855=DIRECTION ( 'NONE',  ( 1.000000000000000000, -5.551115123125773458E-17, -1.260129944081490338E-35 ) ) ;
#29858=CARTESIAN_POINT ( 'NONE',  ( 0.000000000000000000, 5.499999999999991118, -153.0000000000000284 ) ) ;
#29860=CARTESIAN_POINT ( 'NONE',  ( 5.196152422706629359, 3.000000000000002665, -49.46132486540521711 ) ) ;
#29861=ADVANCED_FACE ( 'NONE', ( #15746 ), #8319, .T. ) ;
#29862=CARTESIAN_POINT ( 'NONE',  ( -3.175426480542816066, -5.500000000000057732, -87.87500000000000000 ) ) ;
#29864=CARTESIAN_POINT ( 'NONE',  ( 4.763139720814407951, -2.749999999999988454, -71.00000000000001421 ) ) ;
#29865=CARTESIAN_POINT ( 'NONE',  ( -5.999999999999963585, 9.296355089585909904E-15, -164.3363248654052313 ) ) ;
#29868=CARTESIAN_POINT ( 'NONE',  ( 3.464101615137757051, -5.999999999999979572, -149.4136751345947687 ) ) ;
#29873=CARTESIAN_POINT ( 'NONE',  ( -5.999999999999963585, -1.487416814333745711E-14, -137.3363248654052313 ) ) ;
#29879=CARTESIAN_POINT ( 'NONE',  ( 3.464101615137852974, 5.999999999999884537, -157.3363248654051745 ) ) ;
#29881=ORIENTED_EDGE ( 'NONE', *, *, #12482, .F. ) ;
#29882=CARTESIAN_POINT ( 'NONE',  ( 4.763139720814407951, 2.750000000000002665, -100.7500000000000000 ) ) ;
#29883=CARTESIAN_POINT ( 'NONE',  ( 6.000000000000000888, 1.743066579297358182E-13, -96.66367513459479710 ) ) ;
#29884=CARTESIAN_POINT ( 'NONE',  ( -7.216878364870328078, 0.000000000000000000, -109.5580127018922099 ) ) ;
#29886=CARTESIAN_POINT ( 'NONE',  ( -5.999999999999963585, -1.487416814333745711E-14, -50.33632486540523843 ) ) ;
#29887=CARTESIAN_POINT ( 'NONE',  ( 6.000000000000026645, -1.607695154586707753, -143.2306624327025872 ) ) ;
#29888=CARTESIAN_POINT ( 'NONE',  ( 5.196152422706629359, -2.999999999999988898, -63.21132486540520290 ) ) ;
#29889=AXIS2_PLACEMENT_3D ( 'NONE', #11583, #13426, #20316 ) ;
#29891=CARTESIAN_POINT ( 'NONE',  ( 3.464101615137852974, 5.999999999999884537, -153.4136751345947971 ) ) ;
#29892=( GEOMETRIC_REPRESENTATION_CONTEXT ( 3 ) GLOBAL_UNCERTAINTY_ASSIGNED_CONTEXT ( ( #3592 ) ) GLOBAL_UNIT_ASSIGNED_CONTEXT ( ( #15981, #27283, #17658 ) ) REPRESENTATION_CONTEXT ( 'NONE', 'WORKASPACE' ) );
#29894=CARTESIAN_POINT ( 'NONE',  ( 0.000000000000000000, 5.499999999999991118, -159.0000000000000284 ) ) ;
#29897=VECTOR ( 'NONE', #12942, 1000.000000000000000 ) ;
#29899=CARTESIAN_POINT ( 'NONE',  ( -4.763139720814407951, 2.749999999999946709, -107.7500000000000142 ) ) ;
#29901=CARTESIAN_POINT ( 'NONE',  ( -4.763139720814407951, -2.750000000000016431, -97.00000000000002842 ) ) ;
#29908=ADVANCED_FACE ( 'NONE', ( #25203 ), #22777, .T. ) ;
#29911=DIRECTION ( 'NONE',  ( -7.147005652999508048E-36, 5.642372883946980038E-36, 1.000000000000000000 ) ) ;
#29913=CARTESIAN_POINT ( 'NONE',  ( 7.216878364870455975, -6.409875621278545621E-14, -86.94198729810781856 ) ) ;
#29914=VECTOR ( 'NONE', #28554, 1000.000000000000000 ) ;
#29916=DIRECTION ( 'NONE',  ( -7.147005652999508048E-36, 5.642372883946980038E-36, 1.000000000000000000 ) ) ;
#29920=CARTESIAN_POINT ( 'NONE',  ( 4.763139720814407951, 2.750000000000002665, -118.7500000000000284 ) ) ;
#29923=CARTESIAN_POINT ( 'NONE',  ( 5.412658773652739619, 3.124999999999988898, -128.1830127018922383 ) ) ;
#29924=ORIENTED_EDGE ( 'NONE', *, *, #25685, .F. ) ;
#29925=CARTESIAN_POINT ( 'NONE',  ( -5.196152422706601826, 2.999999999999975131, -160.5386751345948539 ) ) ;
#29926=CARTESIAN_POINT ( 'NONE',  ( -7.216878364870328078, 0.000000000000000000, -122.1919872981078043 ) ) ;
#29927=CARTESIAN_POINT ( 'NONE',  ( -3.608439182435052128, -6.250000000000110134, -174.4419872981078754 ) ) ;
#29930=CARTESIAN_POINT ( 'NONE',  ( -5.999999999999962697, 3.323446944526963891E-14, -163.4136751345948539 ) ) ;
#29931=CARTESIAN_POINT ( 'NONE',  ( 0.000000000000000000, 5.999999999999977796, -90.28867513459482552 ) ) ;
#29935=CARTESIAN_POINT ( 'NONE',  ( 7.216878364870455975, -6.409875621278545621E-14, -76.44198729810783277 ) ) ;
#29936=CARTESIAN_POINT ( 'NONE',  ( 7.216878364870455975, -6.409875621278545621E-14, -59.94198729810782567 ) ) ;
#29937=CARTESIAN_POINT ( 'NONE',  ( -5.196152422706573404, -3.000000000000002665, -170.7886751345948255 ) ) ;
#29938=CARTESIAN_POINT ( 'NONE',  ( 2.775557561562891351E-14, 6.250000000000033751, -181.9330127018922099 ) ) ;
#29940=EDGE_CURVE ( 'NONE', #7050, #8787, #3397, .T. ) ;
#29942=CARTESIAN_POINT ( 'NONE',  ( -2.775557561562891351E-14, -5.500000000000115463, -122.2500000000000284 ) ) ;
#29943=CARTESIAN_POINT ( 'NONE',  ( -5.999999999999944933, 1.607695154586759934, -145.4806624327026441 ) ) ;
#29946=CARTESIAN_POINT ( 'NONE',  ( 0.000000000000000000, 5.999999999999977796, -105.2886751345948397 ) ) ;
#29947=DIRECTION ( 'NONE',  ( -7.147005652999508048E-36, 5.642372883946980038E-36, 1.000000000000000000 ) ) ;
#29948=EDGE_CURVE ( 'NONE', #8787, #124, #9894, .T. ) ;
#29954=CARTESIAN_POINT ( 'NONE',  ( 3.608439182435180470, 6.249999999999982236, -113.6919872981078186 ) ) ;
#29955=CARTESIAN_POINT ( 'NONE',  ( -5.196152422706573404, -3.000000000000002665, -110.2113248654051887 ) ) ;
#29956=CARTESIAN_POINT ( 'NONE',  ( -5.999999999999963585, -1.487416814333745711E-14, -87.83632486540521711 ) ) ;
#29957=VERTEX_POINT ( 'NONE', #6319 ) ;
#29958=ORIENTED_EDGE ( 'NONE', *, *, #19530, .T. ) ;
#29959=LINE ( 'NONE', #13733, #23338 ) ;
#29964=CARTESIAN_POINT ( 'NONE',  ( 5.412658773652712085, -3.125000000000086153, -144.0669872981078470 ) ) ;
#29970=CARTESIAN_POINT ( 'NONE',  ( 7.216878364870455975, -6.409875621278545621E-14, -63.80801270189225249 ) ) ;
#29972=CARTESIAN_POINT ( 'NONE',  ( -5.196152422706601826, 2.999999999999975131, -102.0386751345948539 ) ) ;
#29973=CYLINDRICAL_SURFACE ( 'NONE', #11392, 6.000000000000000888 ) ;
#29977=EDGE_CURVE ( 'NONE', #1984, #16378, #17574, .T. ) ;
#29979=ADVANCED_FACE ( 'NONE', ( #22473 ), #24907, .T. ) ;
#29980=CARTESIAN_POINT ( 'NONE',  ( -4.763139720814407951, 2.749999999999946709, -124.2500000000000284 ) ) ;
#29981=CARTESIAN_POINT ( 'NONE',  ( 0.000000000000000000, 0.000000000000000000, 0.000000000000000000 ) ) ;
#29982=CARTESIAN_POINT ( 'NONE',  ( 2.775557561562891351E-14, 6.250000000000033751, -144.4330127018922383 ) ) ;
#29985=ORIENTED_EDGE ( 'NONE', *, *, #24748, .F. ) ;
#29986=AXIS2_PLACEMENT_3D ( 'NONE', #26625, #17007, #7746 ) ;
#29987=CARTESIAN_POINT ( 'NONE',  ( -6.350852961085760029, -1.281975124255709124E-13, -52.12500000000002842 ) ) ;
#29988=FACE_OUTER_BOUND ( 'NONE', #20616, .T. ) ;
#29989=CARTESIAN_POINT ( 'NONE',  ( -5.196152422706601826, 2.999999999999975131, -69.96132486540524553 ) ) ;
#29994=LINE ( 'NONE', #27677, #11159 ) ;
#29997=CARTESIAN_POINT ( 'NONE',  ( 4.763139720814407951, -2.749999999999988454, -135.5000000000000000 ) ) ;
#30002=CARTESIAN_POINT ( 'NONE',  ( -6.350852961085760029, -1.281975124255709124E-13, -62.62500000000001421 ) ) ;
#30003=VECTOR ( 'NONE', #26379, 1000.000000000000000 ) ;
#30005=CARTESIAN_POINT ( 'NONE',  ( 5.412658773652739619, 3.124999999999988898, -87.68301270189226670 ) ) ;
#30006=EDGE_LOOP ( 'NONE', ( #18435, #28200, #7962, #21643 ) ) ;
#30008=CYLINDRICAL_SURFACE ( 'NONE', #15769, 6.000000000000000888 ) ;
#30010=DIRECTION ( 'NONE',  ( 1.000000000000000000, -5.551115123125773458E-17, -1.260129944081490338E-35 ) ) ;
#30012=PRODUCT_CONTEXT ( 'NONE', #28880, 'mechanical' ) ;
#30013=( BOUNDED_CURVE ( )  B_SPLINE_CURVE ( 2, ( #3877, #1273, #10686, #20030, #24316, #13308, #7885, #29377, #22029 ),
 .UNSPECIFIED., .F., .T. ) 
 B_SPLINE_CURVE_WITH_KNOTS ( ( 3, 2, 2, 2, 3 ),
 ( 0.5583333333333333481, 0.5592592592592592338, 0.5611111111111111160, 0.5629629629629628873, 0.5638888888888888840 ),
 .UNSPECIFIED. ) 
 CURVE ( )  GEOMETRIC_REPRESENTATION_ITEM ( )  RATIONAL_B_SPLINE_CURVE ( ( 0.9330127018922194093, 0.9330127018922234061, 1.000000000000000000, 0.8660254037844388186, 1.000000000000000000, 0.8660254037844388186, 1.000000000000000000, 0.9330127018922194093, 0.9330127018922194093 ) ) 
 REPRESENTATION_ITEM ( '' )  );
#30015=CARTESIAN_POINT ( 'NONE',  ( 0.000000000000000000, 5.499999999999991118, -147.0000000000000284 ) ) ;
#30017=CARTESIAN_POINT ( 'NONE',  ( -5.412658773652739619, 3.124999999999975131, -159.1830127018922667 ) ) ;
#30019=CARTESIAN_POINT ( 'NONE',  ( 6.000000000000000888, -3.330669073875464691E-16, -7.560779664488942560E-35 ) ) ;
#30020=PRODUCT ( 'Clamp rod', 'Clamp rod', '', ( #30012 ) ) ;
#30021=CARTESIAN_POINT ( 'NONE',  ( -6.350852961085760029, -1.281975124255709124E-13, -80.62500000000001421 ) ) ;
#30022=CARTESIAN_POINT ( 'NONE',  ( -5.999999999999963585, 1.780251999655701777E-13, -65.91367513459482552 ) ) ;
#30023=CARTESIAN_POINT ( 'NONE',  ( 0.000000000000000000, 5.499999999999991118, -72.00000000000001421 ) ) ;
#30024=CARTESIAN_POINT ( 'NONE',  ( -3.464101615137757051, -5.999999999999979572, -74.66367513459483973 ) ) ;
#30026=CARTESIAN_POINT ( 'NONE',  ( -5.999999999999904965, -1.607695154586834541, -114.7693375672974412 ) ) ;
#30028=CARTESIAN_POINT ( 'NONE',  ( -5.999999999999963585, -1.487416814333745711E-14, -76.41367513459481131 ) ) ;
#30032=CARTESIAN_POINT ( 'NONE',  ( 0.000000000000000000, -5.999999999999991118, -97.96132486540520290 ) ) ;
#30037=ORIENTED_EDGE ( 'NONE', *, *, #6689, .T. ) ;
#30039=ORIENTED_EDGE ( 'NONE', *, *, #3756, .T. ) ;
#30040=EDGE_CURVE ( 'NONE', #11659, #5958, #13061, .T. ) ;
#30041=CARTESIAN_POINT ( 'NONE',  ( -3.175426480542816510, -5.500000000000057732, -96.87499999999997158 ) ) ;
#30042=CARTESIAN_POINT ( 'NONE',  ( -7.216878364870328078, 0.000000000000000000, -103.5580127018922383 ) ) ;
#30044=DIRECTION ( 'NONE',  ( 1.260129944081490070E-35, 5.642372883946978702E-36, 1.000000000000000000 ) ) ;
#30045=CARTESIAN_POINT ( 'NONE',  ( -5.999999999999963585, -1.487416814333745711E-14, -143.9136751345948255 ) ) ;
#30046=CARTESIAN_POINT ( 'NONE',  ( 4.763139720814407951, -2.749999999999988454, -162.5000000000000284 ) ) ;
#30051=CARTESIAN_POINT ( 'NONE',  ( -4.763139720814407951, -2.750000000000016431, -170.4999999999999716 ) ) ;
#30053=CARTESIAN_POINT ( 'NONE',  ( 6.350852961086080661, -9.614813431917819062E-14, -166.8750000000000568 ) ) ;
#30055=CARTESIAN_POINT ( 'NONE',  ( -4.763139720814407951, -2.750000000000016431, -108.9999999999999858 ) ) ;
#30056=CARTESIAN_POINT ( 'NONE',  ( 3.464101615137757051, -5.999999999999979572, -122.4136751345947971 ) ) ;
#30057=CARTESIAN_POINT ( 'NONE',  ( -6.350852961085760029, -1.281975124255709124E-13, -94.12500000000004263 ) ) ;
#30067=ORIENTED_EDGE ( 'NONE', *, *, #20488, .T. ) ;
#30070=CARTESIAN_POINT ( 'NONE',  ( -7.216878364870328078, 0.000000000000000000, -89.19198729810783277 ) ) ;
#30078=CARTESIAN_POINT ( 'NONE',  ( -4.763139720814407951, -2.750000000000016431, -124.0000000000000000 ) ) ;
#30080=CARTESIAN_POINT ( 'NONE',  ( -3.608439182435115633, 6.249999999999965361, -132.3080127018922383 ) ) ;
#30083=CARTESIAN_POINT ( 'NONE',  ( 5.412658773652739619, 3.124999999999988898, -167.8169872981077901 ) ) ;
#30084=CARTESIAN_POINT ( 'NONE',  ( -3.608439182435115633, 6.249999999999965361, -173.4419872981078470 ) ) ;
#30089=EDGE_CURVE ( 'NONE', #18552, #856, #15335, .T. ) ;
#30090=DIRECTION ( 'NONE',  ( 1.000000000000000000, -5.551115123125773458E-17, -1.260129944081490338E-35 ) ) ;
#30095=CARTESIAN_POINT ( 'NONE',  ( -3.608439182435052128, -6.250000000000110134, -76.94198729810784698 ) ) ;
#30096=CARTESIAN_POINT ( 'NONE',  ( 5.412658773652739619, 3.124999999999988898, -61.31698729810780435 ) ) ;
#30097=CARTESIAN_POINT ( 'NONE',  ( -2.775557561562891351E-14, -5.500000000000115463, -51.75000000000002132 ) ) ;
#30099=DIRECTION ( 'NONE',  ( 0.000000000000000000, 0.000000000000000000, -1.000000000000000000 ) ) ;
#30100=CARTESIAN_POINT ( 'NONE',  ( -6.000000000000007105, -1.607695154586655129, -53.84668783648703538 ) ) ;
#30101=CARTESIAN_POINT ( 'NONE',  ( -4.763139720814407951, -2.750000000000016431, -118.0000000000000000 ) ) ;
#30102=DIRECTION ( 'NONE',  ( -7.147005652999508048E-36, 5.642372883946980038E-36, 1.000000000000000000 ) ) ;
#30107=FACE_OUTER_BOUND ( 'NONE', #18749, .T. ) ;
#30112=CARTESIAN_POINT ( 'NONE',  ( 7.216878364870455975, -6.409875621278545621E-14, -110.9419872981078186 ) ) ;
#30113=CARTESIAN_POINT ( 'NONE',  ( 6.000000000000000888, -6.507448562710137091E-15, -176.1636751345947971 ) ) ;
#30116=ORIENTED_EDGE ( 'NONE', *, *, #30294, .T. ) ;
#30121=ORIENTED_EDGE ( 'NONE', *, *, #6262, .T. ) ;
#30122=CARTESIAN_POINT ( 'NONE',  ( 2.775557561562891351E-14, -6.250000000000061284, -136.8169872981078186 ) ) ;
#30124=CARTESIAN_POINT ( 'NONE',  ( 5.196152422706629359, 3.000000000000002665, -151.4613248654052029 ) ) ;
#30126=CARTESIAN_POINT ( 'NONE',  ( 0.000000000000000000, 5.999999999999977796, -120.2886751345948539 ) ) ;
#30128=CARTESIAN_POINT ( 'NONE',  ( 2.775557561562891351E-14, -6.250000000000061284, -67.18301270189225249 ) ) ;
#30129=EDGE_CURVE ( 'NONE', #3793, #11265, #6741, .T. ) ;
#30132=CARTESIAN_POINT ( 'NONE',  ( -5.999999999999963585, 1.780251999655701777E-13, -73.41367513459483973 ) ) ;
#30133=DIRECTION ( 'NONE',  ( -7.147005652999508048E-36, 5.642372883946980038E-36, 1.000000000000000000 ) ) ;
#30135=CARTESIAN_POINT ( 'NONE',  ( -3.464101615137757051, -5.999999999999979572, -67.16367513459479710 ) ) ;
#30138=CARTESIAN_POINT ( 'NONE',  ( 3.175426480543072749, -5.500000000000105693, -126.6249999999999858 ) ) ;
#30140=CARTESIAN_POINT ( 'NONE',  ( 3.608439182435180470, -6.249999999999997335, -145.0580127018922383 ) ) ;
#30143=EDGE_LOOP ( 'NONE', ( #15410, #15614, #22079, #10963 ) ) ;
#30144=CARTESIAN_POINT ( 'NONE',  ( 4.763139720814407951, -2.749999999999988454, -51.49999999999999289 ) ) ;
#30146=CARTESIAN_POINT ( 'NONE',  ( -5.999999999999963585, 1.780251999655701777E-13, -69.83632486540523132 ) ) ;
#30147=CARTESIAN_POINT ( 'NONE',  ( 6.000000000000000888, -3.330669073875464691E-16, -7.560779664488942560E-35 ) ) ;
#30148=ORIENTED_EDGE ( 'NONE', *, *, #3229, .T. ) ;
#30151=CARTESIAN_POINT ( 'NONE',  ( -5.999999999999971578, 1.607695154586715303, -176.4033121635129930 ) ) ;
#30155=ADVANCED_FACE ( 'NONE', ( #13744 ), #177, .T. ) ;
#30156=CARTESIAN_POINT ( 'NONE',  ( 3.175426480543072749, -5.500000000000105693, -137.1250000000000568 ) ) ;
#30159=ORIENTED_EDGE ( 'NONE', *, *, #19742, .T. ) ;
#30160=CARTESIAN_POINT ( 'NONE',  ( -6.350852961085760029, -1.281975124255709124E-13, -68.62500000000004263 ) ) ;
#30161=EDGE_CURVE ( 'NONE', #3569, #12154, #19319, .T. ) ;
#30162=CARTESIAN_POINT ( 'NONE',  ( -5.412658773652739619, 3.124999999999975131, -88.68301270189226670 ) ) ;
#30163=ORIENTED_EDGE ( 'NONE', *, *, #28612, .T. ) ;
#30164=CARTESIAN_POINT ( 'NONE',  ( -11.00000000000000000, 1.957734142605923910E-15, -14.99152654425661702 ) ) ;
#30168=CARTESIAN_POINT ( 'NONE',  ( 4.763139720814407951, 2.750000000000002665, -147.2500000000000000 ) ) ;
#30171=CARTESIAN_POINT ( 'NONE',  ( 7.216878364870455975, -6.409875621278545621E-14, -159.8080127018922667 ) ) ;
#30172=PRESENTATION_STYLE_ASSIGNMENT (( #26013 ) ) ;
#30173=CARTESIAN_POINT ( 'NONE',  ( 3.464101615137852974, 5.999999999999884537, -89.83632486540521711 ) ) ;
#30174=CARTESIAN_POINT ( 'NONE',  ( -4.763139720814407951, -2.750000000000016431, -76.00000000000001421 ) ) ;
#30176=CARTESIAN_POINT ( 'NONE',  ( -4.763139720814407951, 2.749999999999946709, -76.25000000000004263 ) ) ;
#30183=LINE ( 'NONE', #75, #30278 ) ;
#30188=CARTESIAN_POINT ( 'NONE',  ( 0.000000000000000000, -5.999999999999991118, -157.0386751345948539 ) ) ;
#30190=CARTESIAN_POINT ( 'NONE',  ( -4.763139720814407951, 2.749999999999946709, -154.2500000000000000 ) ) ;
#30193=ORIENTED_EDGE ( 'NONE', *, *, #873, .T. ) ;
#30194=ORIENTED_EDGE ( 'NONE', *, *, #11654, .T. ) ;
#30195=EDGE_CURVE ( 'NONE', #12734, #11750, #23455, .T. ) ;
#30197=ORIENTED_EDGE ( 'NONE', *, *, #29940, .T. ) ;
#30198=CARTESIAN_POINT ( 'NONE',  ( -3.175426480542816510, -5.500000000000057732, -87.87500000000000000 ) ) ;
#30199=( BOUNDED_CURVE ( )  B_SPLINE_CURVE ( 2, ( #8217, #20234, #26954, #22373, #17943, #3304, #12883, #29413, #22220 ),
 .UNSPECIFIED., .F., .T. ) 
 B_SPLINE_CURVE_WITH_KNOTS ( ( 3, 2, 2, 2, 3 ),
 ( 0.1972222222222222987, 0.1981481481481481843, 0.1999999999999999556, 0.2018518518518518379, 0.2027777777777777235 ),
 .UNSPECIFIED. ) 
 CURVE ( )  GEOMETRIC_REPRESENTATION_ITEM ( )  RATIONAL_B_SPLINE_CURVE ( ( 0.9330127018922194093, 0.9330127018922234061, 1.000000000000000000, 0.8660254037844388186, 1.000000000000000000, 0.8660254037844388186, 1.000000000000000000, 0.9330127018922234061, 0.9330127018922194093 ) ) 
 REPRESENTATION_ITEM ( '' )  );
#30200=CARTESIAN_POINT ( 'NONE',  ( -5.412658773652739619, 3.124999999999975131, -109.6830127018922383 ) ) ;
#30203=CARTESIAN_POINT ( 'NONE',  ( 4.763139720814407951, -2.749999999999988454, -165.4999999999999716 ) ) ;
#30206=CARTESIAN_POINT ( 'NONE',  ( 6.000000000000000888, -1.859271017917181981E-14, -47.16367513459483263 ) ) ;
#30208=CARTESIAN_POINT ( 'NONE',  ( -6.350852961085760029, -1.281975124255709124E-13, -173.6250000000000284 ) ) ;
#30209=CARTESIAN_POINT ( 'NONE',  ( -2.775557561562891351E-14, -5.500000000000115463, -164.2500000000000000 ) ) ;
#30211=CARTESIAN_POINT ( 'NONE',  ( -6.350852961085760029, -1.281975124255709124E-13, -101.6250000000000000 ) ) ;
#30212=CARTESIAN_POINT ( 'NONE',  ( -3.175426480542816510, -5.500000000000057732, -98.37500000000000000 ) ) ;
#30216=ORIENTED_EDGE ( 'NONE', *, *, #1965, .T. ) ;
#30219=CARTESIAN_POINT ( 'NONE',  ( -6.000000000000000888, 1.067854986875958443E-15, 7.560779664488942560E-35 ) ) ;
#30222=EDGE_LOOP ( 'NONE', ( #8729, #13699, #10558, #21246 ) ) ;
#30225=CARTESIAN_POINT ( 'NONE',  ( 0.000000000000000000, 0.000000000000000000, -200.0000000000000000 ) ) ;
#30226=VERTEX_POINT ( 'NONE', #1167 ) ;
#30227=CARTESIAN_POINT ( 'NONE',  ( -5.999999999999963585, 1.780251999655701777E-13, -79.41367513459482552 ) ) ;
#30229=ORIENTED_EDGE ( 'NONE', *, *, #7994, .F. ) ;
#30231=ORIENTED_EDGE ( 'NONE', *, *, #23781, .F. ) ;
#30232=CARTESIAN_POINT ( 'NONE',  ( 4.763139720814407951, 2.750000000000002665, -112.7500000000000142 ) ) ;
#30234=CARTESIAN_POINT ( 'NONE',  ( 2.775557561562891351E-14, -6.250000000000061284, -131.6830127018922667 ) ) ;
#30237=CARTESIAN_POINT ( 'NONE',  ( 5.412658773652739619, 3.124999999999988898, -169.3169872981078470 ) ) ;
#30238=CARTESIAN_POINT ( 'NONE',  ( 3.608439182435180470, -6.249999999999997335, -177.1919872981078470 ) ) ;
#30239=VERTEX_POINT ( 'NONE', #24376 ) ;
#30245=CARTESIAN_POINT ( 'NONE',  ( -5.412658773652739619, 3.124999999999975131, -62.31698729810780435 ) ) ;
#30246=CARTESIAN_POINT ( 'NONE',  ( -2.775557561562891351E-14, -5.500000000000115463, -53.25000000000002132 ) ) ;
#30247=CARTESIAN_POINT ( 'NONE',  ( 0.000000000000000000, -5.999999999999991118, -111.4613248654052171 ) ) ;
#30248=CARTESIAN_POINT ( 'NONE',  ( 6.000000000000000888, 1.743066579297358182E-13, -51.66367513459483263 ) ) ;
#30249=CARTESIAN_POINT ( 'NONE',  ( -5.999999999999962697, 3.323446944526963891E-14, -158.9136751345947971 ) ) ;
#30250=CARTESIAN_POINT ( 'NONE',  ( -4.763139720814407951, 2.749999999999946709, -124.2500000000000284 ) ) ;
#30258=DIRECTION ( 'NONE',  ( -7.147005652999508048E-36, 5.642372883946980038E-36, 1.000000000000000000 ) ) ;
#30262=DIRECTION ( 'NONE',  ( -7.147005652999508048E-36, 5.642372883946980038E-36, 1.000000000000000000 ) ) ;
#30263=CARTESIAN_POINT ( 'NONE',  ( -3.608439182435115633, 6.249999999999965361, -110.4419872981078186 ) ) ;
#30268=VERTEX_POINT ( 'NONE', #19773 ) ;
#30273=CARTESIAN_POINT ( 'NONE',  ( 3.608439182435180470, -6.249999999999997335, -136.6919872981078470 ) ) ;
#30275=AXIS2_PLACEMENT_3D ( 'NONE', #28407, #16647, #25970 ) ;
#30278=VECTOR ( 'NONE', #28016, 1000.000000000000000 ) ;
#30282=CARTESIAN_POINT ( 'NONE',  ( 5.412658773652739619, 3.124999999999988898, -66.68301270189225249 ) ) ;
#30285=FACE_OUTER_BOUND ( 'NONE', #17489, .T. ) ;
#30286=LINE ( 'NONE', #28866, #15380 ) ;
#30290=CARTESIAN_POINT ( 'NONE',  ( 0.000000000000000000, 5.499999999999991118, -124.5000000000000568 ) ) ;
#30292=CARTESIAN_POINT ( 'NONE',  ( 0.000000000000000000, 5.999999999999977796, -148.7886751345948255 ) ) ;
#30294=EDGE_CURVE ( 'NONE', #16705, #4423, #17646, .T. ) ;
#30295=CARTESIAN_POINT ( 'NONE',  ( 0.000000000000000000, 5.499999999999991118, -58.50000000000000000 ) ) ;
#30296=CARTESIAN_POINT ( 'NONE',  ( -5.196152422706601826, 2.999999999999975131, -120.9613248654052313 ) ) ;
#30297=( BOUNDED_CURVE ( )  B_SPLINE_CURVE ( 2, ( #16788, #310, #13893, #4766, #9698, #14193, #19081, #28403, #7381 ),
 .UNSPECIFIED., .F., .T. ) 
 B_SPLINE_CURVE_WITH_KNOTS ( ( 3, 2, 2, 2, 3 ),
 ( 0.2972222222222222210, 0.2981481481481481621, 0.2999999999999999889, 0.3018518518518518712, 0.3027777777777777568 ),
 .UNSPECIFIED. ) 
 CURVE ( )  GEOMETRIC_REPRESENTATION_ITEM ( )  RATIONAL_B_SPLINE_CURVE ( ( 0.9330127018922194093, 0.9330127018922194093, 1.000000000000000000, 0.8660254037844388186, 1.000000000000000000, 0.8660254037844388186, 1.000000000000000000, 0.9330127018922214077, 0.9330127018922194093 ) ) 
 REPRESENTATION_ITEM ( '' )  );
#30303=CARTESIAN_POINT ( 'NONE',  ( 2.775557561562891351E-14, -6.250000000000061284, -103.8169872981078470 ) ) ;
#30305=AXIS2_PLACEMENT_3D ( 'NONE', #18930, #28251, #7227 ) ;
#30306=EDGE_CURVE ( 'NONE', #2399, #341, #8234, .T. ) ;
#30309=CARTESIAN_POINT ( 'NONE',  ( 3.175426480543072749, 5.499999999999865885, -138.1250000000000284 ) ) ;
#30310=ORIENTED_EDGE ( 'NONE', *, *, #26836, .T. ) ;
#30313=ORIENTED_EDGE ( 'NONE', *, *, #3123, .T. ) ;
#30314=CARTESIAN_POINT ( 'NONE',  ( 3.175426480543072749, 5.499999999999865885, -69.12500000000002842 ) ) ;
#30315=CARTESIAN_POINT ( 'NONE',  ( 6.000000000000000888, -3.330669073875464691E-16, -7.560779664488942560E-35 ) ) ;
#30316=CARTESIAN_POINT ( 'NONE',  ( -5.196152422706573404, -3.000000000000002665, -124.2886751345948539 ) ) ;
#30317=CARTESIAN_POINT ( 'NONE',  ( 2.775557561562891351E-14, -6.250000000000061284, -88.18301270189220986 ) ) ;
#30320=CARTESIAN_POINT ( 'NONE',  ( -5.999999999999965361, 1.068766945199469465, -179.9582070906448052 ) ) ;
#30322=CARTESIAN_POINT ( 'NONE',  ( 3.175426480543072749, -5.500000000000105693, -149.1250000000000284 ) ) ;
#30323=LINE ( 'NONE', #4208, #3015 ) ;
#30324=CARTESIAN_POINT ( 'NONE',  ( 4.763139720814407951, 2.750000000000002665, -135.2500000000000284 ) ) ;
#30325=CARTESIAN_POINT ( 'NONE',  ( 7.216878364870455975, -6.409875621278545621E-14, -162.8080127018922667 ) ) ;
#30326=CARTESIAN_POINT ( 'NONE',  ( -2.910268709469100014E-14, -10.99999999999998224, -14.99152654425661702 ) ) ;
#30327=EDGE_CURVE ( 'NONE', #3967, #17636, #24220, .T. ) ;
#30328=CARTESIAN_POINT ( 'NONE',  ( 3.175426480543072749, 5.499999999999865885, -79.62500000000002842 ) ) ;
#30329=CARTESIAN_POINT ( 'NONE',  ( 5.196152422706629359, -2.999999999999988898, -140.2886751345948539 ) ) ;
#30331=CARTESIAN_POINT ( 'NONE',  ( 3.175426480543072749, -5.500000000000105693, -63.62500000000001421 ) ) ;
#30333=CARTESIAN_POINT ( 'NONE',  ( 6.000000000000052403, -1.607695154586662678, -87.73066243270261566 ) ) ;
#30339=CARTESIAN_POINT ( 'NONE',  ( -5.196152422706573404, -3.000000000000002665, -98.78867513459482552 ) ) ;
#30342=ORIENTED_EDGE ( 'NONE', *, *, #11945, .F. ) ;
#30346=CARTESIAN_POINT ( 'NONE',  ( 3.464101615137757051, -5.999999999999979572, -84.91367513459481131 ) ) ;
#30348=ORIENTED_EDGE ( 'NONE', *, *, #29300, .T. ) ;
#30349=ORIENTED_EDGE ( 'NONE', *, *, #21507, .T. ) ;
#30350=CARTESIAN_POINT ( 'NONE',  ( -3.175426480542816510, -5.500000000000057732, -89.37500000000001421 ) ) ;
#30351=CARTESIAN_POINT ( 'NONE',  ( -3.608439182435052128, -6.250000000000110134, -104.8080127018922383 ) ) ;
#30357=CARTESIAN_POINT ( 'NONE',  ( -5.999999999999963585, -1.487416814333745711E-14, -92.91367513459482552 ) ) ;
#30358=CARTESIAN_POINT ( 'NONE',  ( 3.175426480543072749, 5.499999999999865885, -174.1250000000000284 ) ) ;
#30360=CARTESIAN_POINT ( 'NONE',  ( -4.763139720814407951, -2.750000000000016431, -152.5000000000000284 ) ) ;
#30363=CARTESIAN_POINT ( 'NONE',  ( 4.763139720814407951, -2.749999999999988454, -102.5000000000000284 ) ) ;
#30365=ADVANCED_FACE ( 'NONE', ( #13664 ), #1949, .T. ) ;
#30366=CARTESIAN_POINT ( 'NONE',  ( 6.350852961086080661, -9.614813431917819062E-14, -94.87500000000004263 ) ) ;
#30372=CARTESIAN_POINT ( 'NONE',  ( -3.464101615137725076, 5.999999999999979572, -130.0863248654052029 ) ) ;
#30374=DIRECTION ( 'NONE',  ( -7.147005652999508048E-36, 5.642372883946980038E-36, 1.000000000000000000 ) ) ;
#30376=DIRECTION ( 'NONE',  ( -7.147005652999508048E-36, 5.642372883946980038E-36, 1.000000000000000000 ) ) ;
#30379=EDGE_LOOP ( 'NONE', ( #22578, #15101, #8594, #21148 ) ) ;
#30380=DIRECTION ( 'NONE',  ( 1.000000000000000000, -5.551115123125774074E-17, 0.000000000000000000 ) ) ;
#30381=( BOUNDED_CURVE ( )  B_SPLINE_CURVE ( 2, ( #22374, #26955, #5757, #28955, #28803, #24207, #17332, #10725, #1002 ),
 .UNSPECIFIED., .F., .T. ) 
 B_SPLINE_CURVE_WITH_KNOTS ( ( 3, 2, 2, 2, 3 ),
 ( 0.7583333333333333037, 0.7592592592592593004, 0.7611111111111110716, 0.7629629629629629539, 0.7638888888888889506 ),
 .UNSPECIFIED. ) 
 CURVE ( )  GEOMETRIC_REPRESENTATION_ITEM ( )  RATIONAL_B_SPLINE_CURVE ( ( 0.9330127018922194093, 0.9330127018922154125, 1.000000000000000000, 0.8660254037844388186, 1.000000000000000000, 0.8660254037844388186, 1.000000000000000000, 0.9330127018922154125, 0.9330127018922194093 ) ) 
 REPRESENTATION_ITEM ( '' )  );
#30384=ORIENTED_EDGE ( 'NONE', *, *, #16101, .T. ) ;
#30385=CARTESIAN_POINT ( 'NONE',  ( -6.350852961085760029, -1.281975124255709124E-13, -112.1249999999999858 ) ) ;
#30387=CARTESIAN_POINT ( 'NONE',  ( -7.216878364870328078, 0.000000000000000000, -133.5580127018922667 ) ) ;
#30390=CONICAL_SURFACE ( 'NONE', #22059, 1000.000000000000682, 0.7853981633974479459 ) ;
#30391=CARTESIAN_POINT ( 'NONE',  ( -3.608439182435115633, 6.249999999999965361, -170.4419872981078186 ) ) ;
#30394=ORIENTED_EDGE ( 'NONE', *, *, #12545, .T. ) ;
#30395=FACE_OUTER_BOUND ( 'NONE', #24170, .T. ) ;
#30399=CARTESIAN_POINT ( 'NONE',  ( -7.216878364870328078, 0.000000000000000000, -175.5580127018922667 ) ) ;
#30403=CARTESIAN_POINT ( 'NONE',  ( -2.775557561562891351E-14, -5.500000000000115463, -123.7500000000000284 ) ) ;
#30405=CARTESIAN_POINT ( 'NONE',  ( 5.196152422706629359, 3.000000000000002665, -146.0386751345948539 ) ) ;
#30408=CARTESIAN_POINT ( 'NONE',  ( 6.000000000000000888, -1.859271017917181981E-14, -72.08632486540521711 ) ) ;
#30411=CYLINDRICAL_SURFACE ( 'NONE', #27043, 6.000000000000000888 ) ;
#30414=CARTESIAN_POINT ( 'NONE',  ( 6.000000000000000888, -1.859271017917181981E-14, -135.0863248654052029 ) ) ;
#30415=CARTESIAN_POINT ( 'NONE',  ( 6.000000000000000888, -1.859271017917181981E-14, -159.0863248654052029 ) ) ;
ENDSEC;
END-ISO-10303-21;
